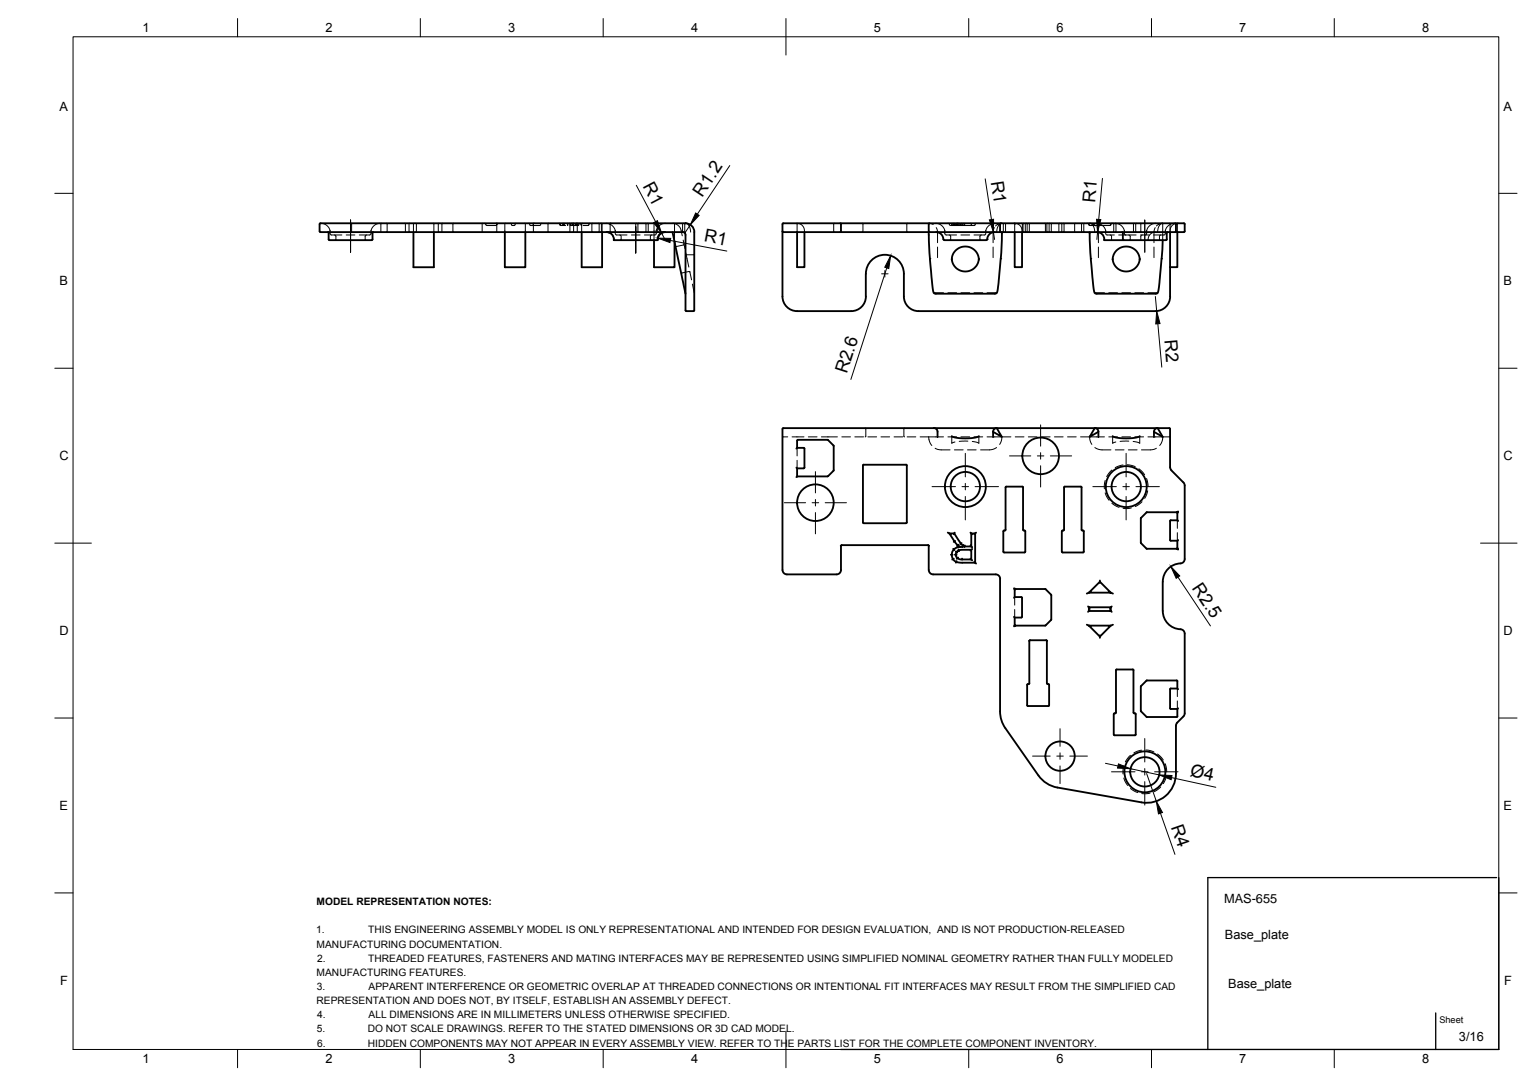
ISO-10303-21;
HEADER;
FILE_DESCRIPTION((''),'2;1');
FILE_NAME('Base_Plate.step','2026-10-09T11:34:15-07:00',(''),(''),'','','');
FILE_SCHEMA (('AUTOMOTIVE_DESIGN { 1 0 10303 214 3 1 1 }'));
ENDSEC;
DATA;
#10=MECHANICAL_DESIGN_GEOMETRIC_PRESENTATION_REPRESENTATION('',(#630),#117170);
#171=ELLIPSE('',#50166,0.169705627484765,0.12) ;
#172=ELLIPSE('',#50168,0.169705627484778,0.12) ;
#173=ELLIPSE('',#50175,0.249814202663062,0.12) ;
#174=ELLIPSE('',#50177,0.136899613896297,0.12) ;
#175=ELLIPSE('',#50182,0.169705627484765,0.12) ;
#176=ELLIPSE('',#50184,0.169705627484778,0.12) ;
#177=ELLIPSE('',#50186,0.169705627484765,0.12) ;
#178=ELLIPSE('',#50188,0.169705627484778,0.12) ;
#179=ELLIPSE('',#50195,0.169705627484765,0.12) ;
#180=ELLIPSE('',#50197,0.169705627484765,0.12) ;
#181=ELLIPSE('',#50201,0.169705627484779,0.12) ;
#182=ELLIPSE('',#50202,0.31357511157033,0.12) ;
#183=ELLIPSE('',#50204,0.313575111570327,0.12) ;
#184=ELLIPSE('',#50210,0.169705627484784,0.12) ;
#185=ELLIPSE('',#50211,0.169705627484784,0.12) ;
#186=ELLIPSE('',#50213,0.169705627484765,0.12) ;
#187=ELLIPSE('',#50215,0.169705627484753,0.12) ;
#188=ELLIPSE('',#50221,0.313575111570327,0.12) ;
#189=ELLIPSE('',#50222,0.169705627484779,0.12) ;
#190=ELLIPSE('',#50224,0.31357511157033,0.12) ;
#191=ELLIPSE('',#50230,0.249814202663065,0.12) ;
#192=ELLIPSE('',#50233,0.136899613896321,0.12) ;
#193=ELLIPSE('',#50235,0.169705627484778,0.12) ;
#194=ELLIPSE('',#50236,0.169705627484778,0.12) ;
#195=ELLIPSE('',#50238,0.169705627484765,0.12) ;
#196=ELLIPSE('',#50240,0.169705627484778,0.12) ;
#197=ELLIPSE('',#50250,1.73726470137952,1.7) ;
#198=ELLIPSE('',#50251,1.73726470137952,1.7) ;
#199=ELLIPSE('',#50254,1.73726470137952,1.7) ;
#200=ELLIPSE('',#50255,1.73726470137952,1.7) ;
#201=ELLIPSE('',#50326,0.313575111570335,0.12) ;
#202=ELLIPSE('',#50327,0.169705627484762,0.12) ;
#203=ELLIPSE('',#50329,0.313575111570314,0.12) ;
#204=ELLIPSE('',#50333,0.169705627484778,0.12) ;
#205=ELLIPSE('',#50334,0.169705627484778,0.12) ;
#206=ELLIPSE('',#50336,0.169705627484765,0.12) ;
#207=ELLIPSE('',#50338,0.169705627484778,0.12) ;
#208=ELLIPSE('',#50342,0.169705627484779,0.12) ;
#209=ELLIPSE('',#50343,0.313575111570343,0.12) ;
#210=ELLIPSE('',#50345,0.313575111570327,0.12) ;
#211=ELLIPSE('',#50371,1.73726470137952,1.7) ;
#212=ELLIPSE('',#50372,1.73726470137952,1.7) ;
#213=ELLIPSE('',#50373,1.73726470137952,1.7) ;
#214=ELLIPSE('',#50374,1.73726470137952,1.7) ;
#215=ELLIPSE('',#50520,4.854121959737,1.) ;
#216=ELLIPSE('',#50521,4.854121959737,1.) ;
#217=ELLIPSE('',#50535,4.854121959737,1.) ;
#218=ELLIPSE('',#50536,4.854121959737,1.) ;
#219=ELLIPSE('',#50561,8.2520073315529,1.7) ;
#220=ELLIPSE('',#50562,8.2520073315529,1.7) ;
#221=ELLIPSE('',#50563,8.2520073315529,1.7) ;
#222=ELLIPSE('',#50564,8.2520073315529,1.7) ;
#223=ELLIPSE('',#50565,0.707106781186556,0.5) ;
#224=ELLIPSE('',#50571,0.509901951359303,0.0999999999999979) ;
#225=ELLIPSE('',#50645,0.223606797749974,0.0999999999999979) ;
#226=ELLIPSE('',#50646,0.223606797749982,0.0999999999999979) ;
#227=ELLIPSE('',#50648,0.141421356237297,0.1) ;
#228=ELLIPSE('',#50651,0.223606797749982,0.100000000000002) ;
#229=ELLIPSE('',#50652,0.223606797749974,0.0999999999999979) ;
#230=ELLIPSE('',#50660,0.1414213562373,0.1) ;
#231=ELLIPSE('',#50779,0.223606797749974,0.0999999999999934) ;
#232=ELLIPSE('',#50780,0.223606797749982,0.0999999999999979) ;
#233=ELLIPSE('',#50783,0.223606797749982,0.0999999999999979) ;
#234=ELLIPSE('',#50784,0.223606797749974,0.100000000000002) ;
#235=ELLIPSE('',#51163,1.38924439894499,1.2) ;
#236=ELLIPSE('',#51164,1.38924439894499,1.2) ;
#237=ELLIPSE('',#51210,0.141421356237297,0.1) ;
#238=ELLIPSE('',#51222,0.141421356237292,0.1) ;
#239=ELLIPSE('',#51349,0.141421356237297,0.1) ;
#240=ELLIPSE('',#51361,0.141421356237292,0.1) ;
#241=ELLIPSE('',#51463,0.141421356237297,0.1) ;
#242=ELLIPSE('',#51475,0.141421356237292,0.1) ;
#243=ELLIPSE('',#51481,0.141421356237297,0.1) ;
#244=ELLIPSE('',#51631,1.38924439894499,1.2) ;
#245=ELLIPSE('',#51632,1.38924439894498,1.2) ;
#246=ELLIPSE('',#51634,1.38924439894498,1.2) ;
#247=ELLIPSE('',#51635,1.38924439894498,1.2) ;
#248=ELLIPSE('',#51636,1.38924439894499,1.2) ;
#249=ELLIPSE('',#51637,1.38924439894499,1.2) ;
#250=ELLIPSE('',#51639,1.38924439894499,1.2) ;
#251=ELLIPSE('',#51640,1.38924439894499,1.2) ;
#252=ELLIPSE('',#51641,1.38924439894498,1.2) ;
#253=ELLIPSE('',#51642,1.38924439894498,1.2) ;
#254=ELLIPSE('',#51644,1.38924439894498,1.20000000000001) ;
#255=ELLIPSE('',#51645,1.38924439894498,1.20000000000001) ;
#256=ELLIPSE('',#51650,0.614889130379839,0.499999999999998) ;
#257=ELLIPSE('',#51654,0.614889130379839,0.499999999999998) ;
#258=ELLIPSE('',#51660,0.614889130379839,0.499999999999998) ;
#259=ELLIPSE('',#51664,0.614889130379841,0.499999999999998) ;
#260=ELLIPSE('',#51673,4.7762432936358,0.499999999999998) ;
#261=ELLIPSE('',#51675,4.7762432936358,0.499999999999998) ;
#262=ELLIPSE('',#51683,4.7762432936358,0.499999999999998) ;
#263=ELLIPSE('',#51706,4.7762432936358,0.499999999999998) ;
#588=SHAPE_REPRESENTATION_RELATIONSHIP('SRR','None',#117243,#609) ;
#609=ADVANCED_BREP_SHAPE_REPRESENTATION('',(#651),#117151) ;
#630=STYLED_ITEM('',(#117355),#651) ;
#651=MANIFOLD_SOLID_BREP('Body1',#49059) ;
#679=FACE_BOUND('',#14322,.T.) ;
#680=FACE_BOUND('',#14408,.T.) ;
#681=FACE_BOUND('',#14409,.T.) ;
#682=FACE_BOUND('',#14410,.T.) ;
#683=FACE_BOUND('',#14411,.T.) ;
#684=FACE_BOUND('',#14412,.T.) ;
#685=FACE_BOUND('',#14413,.T.) ;
#686=FACE_BOUND('',#14414,.T.) ;
#687=FACE_BOUND('',#14415,.T.) ;
#688=FACE_BOUND('',#14416,.T.) ;
#689=FACE_BOUND('',#14417,.T.) ;
#690=FACE_BOUND('',#14418,.T.) ;
#691=FACE_BOUND('',#14419,.T.) ;
#692=FACE_BOUND('',#14420,.T.) ;
#693=FACE_BOUND('',#14421,.T.) ;
#694=FACE_BOUND('',#14422,.T.) ;
#695=FACE_BOUND('',#14423,.T.) ;
#696=FACE_BOUND('',#14424,.T.) ;
#697=FACE_BOUND('',#14425,.T.) ;
#698=FACE_BOUND('',#14447,.T.) ;
#699=FACE_BOUND('',#14453,.T.) ;
#700=FACE_BOUND('',#14454,.T.) ;
#701=FACE_BOUND('',#14455,.T.) ;
#702=FACE_BOUND('',#14456,.T.) ;
#703=FACE_BOUND('',#14457,.T.) ;
#704=FACE_BOUND('',#14458,.T.) ;
#705=FACE_BOUND('',#14459,.T.) ;
#706=FACE_BOUND('',#14460,.T.) ;
#707=FACE_BOUND('',#14461,.T.) ;
#708=FACE_BOUND('',#14462,.T.) ;
#709=FACE_BOUND('',#14463,.T.) ;
#710=FACE_BOUND('',#14464,.T.) ;
#711=FACE_BOUND('',#14465,.T.) ;
#712=FACE_BOUND('',#14466,.T.) ;
#713=FACE_BOUND('',#14496,.T.) ;
#714=FACE_BOUND('',#14502,.T.) ;
#715=FACE_BOUND('',#14505,.T.) ;
#716=FACE_BOUND('',#14509,.T.) ;
#717=FACE_BOUND('',#14512,.T.) ;
#718=FACE_BOUND('',#15017,.T.) ;
#719=FACE_BOUND('',#15025,.T.) ;
#720=FACE_BOUND('',#15032,.T.) ;
#721=FACE_BOUND('',#15038,.T.) ;
#998=B_SPLINE_CURVE_WITH_KNOTS('',3,(#79250,#79251,#79252,#79253,#79254,
#79255,#79256,#79257,#79258,#79259),.UNSPECIFIED.,.F.,.F.,(4,2,2,2,4),(-0.000984424941950333,
0.,0.0304393222729151,0.0604225486602068,0.0620633422654789),
 .UNSPECIFIED.) ;
#999=B_SPLINE_CURVE_WITH_KNOTS('',3,(#79261,#79262,#79263,#79264,#79265,
#79266,#79267,#79268,#79269,#79270,#79271,#79272,#79273,#79274),
 .UNSPECIFIED.,.F.,.F.,(4,2,2,2,2,2,4),(-8.82336995782881E-5,0.,0.00475115835790631,
0.00873436624242474,0.0121992039700031,0.0140206649989405,0.0158413354962278),
 .UNSPECIFIED.) ;
#1000=B_SPLINE_CURVE_WITH_KNOTS('',3,(#79276,#79277,#79278,#79279,#79280,
#79281,#79282,#79283,#79284,#79285,#79286,#79287,#79288,#79289,#79290,#79291,
#79292,#79293,#79294,#79295,#79296,#79297,#79298,#79299,#79300,#79301,#79302,
#79303,#79304,#79305,#79306,#79307,#79308,#79309),.UNSPECIFIED.,.F.,.F.,
(4,3,3,3,3,3,3,3,3,3,3,4),(-0.0604222015446389,-0.0550499926507643,-0.0493561418638026,
-0.0430468116754606,-0.0361516451437183,-0.0304393667102573,-0.0296323735440378,
-0.0222243385537494,-0.0158108328697019,-0.00982069491557987,-0.00433261667194647,
-2.33582884381498E-7),.UNSPECIFIED.) ;
#1001=B_SPLINE_CURVE_WITH_KNOTS('',3,(#79310,#79311,#79312,#79313,#79314,
#79315,#79316,#79317,#79318,#79319,#79320,#79321,#79322,#79323),
 .UNSPECIFIED.,.F.,.F.,(4,2,2,2,2,2,4),(-0.0211454388250223,-0.0210285224813978,
-0.0147156589259276,-0.00942919902689826,-0.00482563543048829,-0.00241277839740307,
0.),.UNSPECIFIED.) ;
#1002=B_SPLINE_CURVE_WITH_KNOTS('',3,(#79366,#79367,#79368,#79369,#79370,
#79371),.UNSPECIFIED.,.F.,.F.,(4,2,4),(-0.0604383125048107,-0.0340909276764841,
-5.87690718515846E-9),.UNSPECIFIED.) ;
#1003=B_SPLINE_CURVE_WITH_KNOTS('',3,(#79373,#79374,#79375,#79376,#79377,
#79378,#79379,#79380,#79381,#79382,#79383,#79384,#79385,#79386,#79387,#79388,
#79389,#79390,#79391,#79392,#79393,#79394,#79395,#79396,#79397),
 .UNSPECIFIED.,.F.,.F.,(4,3,3,3,3,3,3,3,4),(0.,0.142857141665404,0.284233095225632,
0.427830830943624,0.571428566661616,0.709082623356265,0.846526517857094,
0.983993345114335,1.00000000203212),.UNSPECIFIED.) ;
#1004=B_SPLINE_CURVE_WITH_KNOTS('',3,(#79399,#79400,#79401,#79402,#79403,
#79404,#79405,#79406),.UNSPECIFIED.,.F.,.F.,(4,2,2,4),(-6.37514627733282E-5,
0.0340909276764841,0.0604383336928468,0.061399226101535),.UNSPECIFIED.) ;
#1005=B_SPLINE_CURVE_WITH_KNOTS('',3,(#79407,#79408,#79409,#79410,#79411,
#79412,#79413,#79414,#79415,#79416,#79417,#79418,#79419,#79420),
 .UNSPECIFIED.,.F.,.F.,(4,2,2,2,2,2,4),(-0.0211453713160809,-0.0210284730514246,
-0.0147152918429848,-0.00942861499076061,-0.00482456947936517,-0.00241227801516162,
0.),.UNSPECIFIED.) ;
#1006=B_SPLINE_CURVE_WITH_KNOTS('',3,(#79472,#79473,#79474,#79475,#79476,
#79477,#79478,#79479,#79480,#79481),.UNSPECIFIED.,.F.,.F.,(4,2,2,2,4),(-0.0016406621045341,
0.,0.032656775096122,0.0751675585986371,0.0752925833074644),
 .UNSPECIFIED.) ;
#1007=B_SPLINE_CURVE_WITH_KNOTS('',3,(#79483,#79484,#79485,#79486,#79487,
#79488,#79489,#79490,#79491,#79492,#79493,#79494,#79495,#79496,#79497,#79498,
#79499,#79500,#79501,#79502,#79503,#79504,#79505,#79506),.UNSPECIFIED.,
 .F.,.F.,(4,2,2,2,2,2,2,2,2,2,2,4),(-0.0405465275427285,-0.0399836298810584,
-0.0342707961683927,-0.0296950430028694,-0.0224465576618196,-0.012906803650382,
-0.0107060635347755,-0.00880130672328058,-0.00614814155262501,-0.00435008553811397,
-0.00226833765470988,0.),.UNSPECIFIED.) ;
#1008=B_SPLINE_CURVE_WITH_KNOTS('',3,(#79507,#79508,#79509,#79510,#79511,
#79512,#79513,#79514,#79515,#79516,#79517,#79518,#79519,#79520,#79521,#79522,
#79523,#79524,#79525,#79526,#79527,#79528,#79529,#79530,#79531,#79532,#79533,
#79534,#79535,#79536,#79537,#79538,#79539,#79540),.UNSPECIFIED.,.F.,.F.,
(4,3,3,3,3,3,3,3,3,3,3,4),(-0.0751671270593557,-0.0670063003644427,-0.058330620968889,
-0.0493174041305417,-0.0396504587769834,-0.032656775096122,-0.0326552412924559,
-0.0240593424052777,-0.0160879007308648,-0.00858318314202981,-0.00158464448525019,
-1.06159176561375E-7),.UNSPECIFIED.) ;
#1009=B_SPLINE_CURVE_WITH_KNOTS('',3,(#79607,#79608,#79609,#79610,#79611,
#79612),.UNSPECIFIED.,.F.,.F.,(4,2,4),(-0.0457309983059805,-0.0235600635035843,
-3.22828420435411E-7),.UNSPECIFIED.) ;
#1010=B_SPLINE_CURVE_WITH_KNOTS('',3,(#79614,#79615,#79616,#79617,#79618,
#79619,#79620,#79621,#79622,#79623),.UNSPECIFIED.,.F.,.F.,(4,2,2,2,4),(-0.00096080851771424,
0.,0.0235600635035843,0.0457311162964727,0.0467303873666823),
 .UNSPECIFIED.) ;
#1011=B_SPLINE_CURVE_WITH_KNOTS('',3,(#79624,#79625,#79626,#79627,#79628,
#79629,#79630,#79631,#79632,#79633,#79634,#79635,#79636,#79637),
 .UNSPECIFIED.,.F.,.F.,(4,2,2,2,2,2,4),(-8.774851074935E-5,0.,0.00473869223690591,
0.00870703996733189,0.0121629886280889,0.0139740750814815,0.0157851260614204),
 .UNSPECIFIED.) ;
#1012=B_SPLINE_CURVE_WITH_KNOTS('',3,(#79688,#79689,#79690,#79691,#79692,
#79693,#79694,#79695,#79696,#79697,#79698,#79699,#79700,#79701,#79702,#79703,
#79704,#79705,#79706,#79707,#79708,#79709,#79710,#79711,#79712,#79713,#79714,
#79715),.UNSPECIFIED.,.F.,.F.,(4,3,3,3,3,3,3,3,3,4),(-0.0432143735368821,
-0.0386255934136773,-0.0334465535042506,-0.027720164402335,-0.0217199035575619,
-0.0210041587704275,-0.0147723605623817,-0.00929676450395368,-0.00452143288898869,
-8.08181800291421E-8),.UNSPECIFIED.) ;
#1013=B_SPLINE_CURVE_WITH_KNOTS('',3,(#79716,#79717,#79718,#79719,#79720,
#79721,#79722,#79723,#79724,#79725),.UNSPECIFIED.,.F.,.F.,(4,2,2,2,4),(-0.000999294135844071,
0.,0.0217198699392343,0.0432144526123464,0.0441989132427654),
 .UNSPECIFIED.) ;
#1014=B_SPLINE_CURVE_WITH_KNOTS('',3,(#79752,#79753,#79754,#79755,#79756,
#79757),.UNSPECIFIED.,.F.,.F.,(4,2,4),(1.8183290160026E-14,0.0307388136698783,
0.0544948017664183),.UNSPECIFIED.) ;
#1015=B_SPLINE_CURVE_WITH_KNOTS('',3,(#79763,#79764,#79765,#79766,#79767,
#79768,#79769,#79770),.UNSPECIFIED.,.F.,.F.,(4,2,2,4),(-0.000903812556791651,
0.,0.0126332411015006,0.0312371936251197),.UNSPECIFIED.) ;
#1016=B_SPLINE_CURVE_WITH_KNOTS('',3,(#79772,#79773,#79774,#79775,#79776,
#79777,#79778,#79779,#79780,#79781),.UNSPECIFIED.,.F.,.F.,(4,2,2,2,4),(-0.000668949496694549,
0.,0.0150950300818429,0.0294213468333971,0.0303251295908459),
 .UNSPECIFIED.) ;
#1017=B_SPLINE_CURVE_WITH_KNOTS('',3,(#79783,#79784,#79785,#79786,#79787,
#79788,#79789,#79790,#79791,#79792),.UNSPECIFIED.,.F.,.F.,(4,2,2,2,4),(-0.00020740379149845,
0.,0.0232646742763639,0.0410522705936588,0.041721226167804),
 .UNSPECIFIED.) ;
#1018=B_SPLINE_CURVE_WITH_KNOTS('',3,(#79794,#79795,#79796,#79797,#79798,
#79799,#79800,#79801),.UNSPECIFIED.,.F.,.F.,(4,2,2,4),(-4.75212523545475E-5,
0.0386336727204952,0.0678747004384468,0.0680821984481714),.UNSPECIFIED.) ;
#1019=B_SPLINE_CURVE_WITH_KNOTS('',3,(#79809,#79810,#79811,#79812,#79813,
#79814),.UNSPECIFIED.,.F.,.F.,(4,2,4),(0.000722157276979357,0.0318468005485353,
0.0667305959449343),.UNSPECIFIED.) ;
#1020=B_SPLINE_CURVE_WITH_KNOTS('',3,(#79816,#79817,#79818,#79819,#79820,
#79821,#79822,#79823),.UNSPECIFIED.,.F.,.F.,(4,2,2,4),(-0.0369647188766498,
0.,0.0196661092474417,0.0345442295414817),.UNSPECIFIED.) ;
#1021=B_SPLINE_CURVE_WITH_KNOTS('',3,(#79825,#79826,#79827,#79828,#79829,
#79830,#79831,#79832),.UNSPECIFIED.,.F.,.F.,(4,2,2,4),(0.00145417557171005,
0.0398009040484053,0.0884506599106943,0.125182168962163),.UNSPECIFIED.) ;
#1022=B_SPLINE_CURVE_WITH_KNOTS('',3,(#79834,#79835,#79836,#79837,#79838,
#79839,#79840,#79841),.UNSPECIFIED.,.F.,.F.,(4,1,2,1,4),(0.000848899917498889,
0.021868453247988,0.0364474220799808,0.0505556257289287,0.070263889237609),
 .UNSPECIFIED.) ;
#1023=B_SPLINE_CURVE_WITH_KNOTS('',3,(#79843,#79844,#79845,#79846,#79847,
#79848),.UNSPECIFIED.,.F.,.F.,(4,2,4),(0.000832214192100071,0.0289083223985083,
0.0574703491509667),.UNSPECIFIED.) ;
#1024=B_SPLINE_CURVE_WITH_KNOTS('',3,(#79850,#79851,#79852,#79853,#79854,
#79855,#79856,#79857),.UNSPECIFIED.,.F.,.F.,(4,1,2,1,4),(0.00109423153353252,
0.0104867604235457,0.0262169010588733,0.0371127510104888,0.052624276685899),
 .UNSPECIFIED.) ;
#1025=B_SPLINE_CURVE_WITH_KNOTS('',3,(#79859,#79860,#79861,#79862,#79863,
#79864),.UNSPECIFIED.,.F.,.F.,(4,2,4),(4.70742900094273E-5,0.0453812948763195,
0.0781603595086036),.UNSPECIFIED.) ;
#1026=B_SPLINE_CURVE_WITH_KNOTS('',3,(#79877,#79878,#79879,#79880,#79881,
#79882,#79883,#79884,#79885,#79886,#79887,#79888,#79889,#79890,#79891,#79892,
#79893,#79894,#79895,#79896,#79897,#79898),.UNSPECIFIED.,.F.,.F.,(4,2,2,
2,2,2,2,2,2,2,4),(-0.0189100268387207,-0.0188225261357837,-0.0160937127726661,
-0.0140628523915856,-0.0113357098457601,-0.010804126006901,-0.00937481072638454,
-0.00663134068272864,-0.00468727656071559,-0.00196623445923168,0.),
 .UNSPECIFIED.) ;
#1027=B_SPLINE_CURVE_WITH_KNOTS('',3,(#79905,#79906,#79907,#79908,#79909,
#79910,#79911,#79912,#79913,#79914,#79915,#79916,#79917,#79918,#79919,#79920,
#79921,#79922,#79923,#79924,#79925,#79926),.UNSPECIFIED.,.F.,.F.,(4,2,2,
2,2,2,2,2,2,2,4),(-0.0189091510353225,-0.0188216583950064,-0.0160930867214601,
-0.0140631747980082,-0.0113361362872527,-0.010803887239561,-0.00937541792678878,
-0.00663206984589378,-0.00468769926487486,-0.00196659271288638,0.),
 .UNSPECIFIED.) ;
#1028=B_SPLINE_CURVE_WITH_KNOTS('',3,(#79969,#79970,#79971,#79972,#79973,
#79974,#79975,#79976,#79977,#79978,#79979,#79980,#79981,#79982,#79983,#79984,
#79985,#79986,#79987,#79988,#79989,#79990,#79991,#79992,#79993,#79994,#79995,
#79996,#79997,#79998,#79999,#80000,#80001,#80002),.UNSPECIFIED.,.F.,.F.,
(4,3,3,3,3,3,3,3,3,3,3,4),(-0.0189104384936197,-0.0188229339990635,-0.0160940759188526,
-0.0140627008849462,-0.011335536637837,-0.0108042382537074,-0.00937452533081662,
-0.00663104829102613,-0.00468707787444879,-0.00196605255282242,-9.10972545172394E-5,
0.),.UNSPECIFIED.) ;
#1029=B_SPLINE_CURVE_WITH_KNOTS('',3,(#80003,#80004,#80005,#80006,#80007,
#80008),.UNSPECIFIED.,.F.,.F.,(4,2,4),(-0.0678747004384468,-0.0386336727204952,
9.931359662603E-16),.UNSPECIFIED.) ;
#1030=B_SPLINE_CURVE_WITH_KNOTS('',3,(#80060,#80061,#80062,#80063,#80064,
#80065,#80066,#80067,#80068,#80069,#80070,#80071,#80072,#80073,#80074,#80075,
#80076,#80077,#80078,#80079,#80080,#80081,#80082,#80083,#80084,#80085,#80086,
#80087,#80088,#80089,#80090,#80091,#80092,#80093),.UNSPECIFIED.,.F.,.F.,
(4,3,3,3,3,3,3,3,3,3,3,4),(-0.0189231987523393,-0.0188355768250839,-0.016103896315164,
-0.0140579962341654,-0.0113294935982673,-0.0108077177394999,-0.00936568511698275,
-0.00662104306256861,-0.00468092840563795,-0.00196078713666773,-0.000132076778823899,
0.),.UNSPECIFIED.) ;
#1031=B_SPLINE_CURVE_WITH_KNOTS('',3,(#80094,#80095,#80096,#80097,#80098,
#80099,#80100,#80101,#80102,#80103,#80104,#80105,#80106,#80107,#80108,#80109,
#80110,#80111,#80112,#80113,#80114,#80115,#80116,#80117,#80118),
 .UNSPECIFIED.,.F.,.F.,(4,3,3,3,3,3,3,3,4),(-0.041052254598462,-0.0353947710294345,
-0.0290069620103994,-0.0232649417665907,-0.0232646742763639,-0.0157599768214883,
-0.00879512539945639,-0.00239829329457513,-6.62284045196766E-9),
 .UNSPECIFIED.) ;
#1032=B_SPLINE_CURVE_WITH_KNOTS('',3,(#80151,#80152,#80153,#80154,#80155,
#80156),.UNSPECIFIED.,.F.,.F.,(4,2,4),(-0.0792555822118552,-0.0453812948763195,
2.08166817117217E-17),.UNSPECIFIED.) ;
#1033=B_SPLINE_CURVE_WITH_KNOTS('',3,(#80158,#80159,#80160,#80161,#80162,
#80163,#80164,#80165,#80166,#80167,#80168,#80169,#80170,#80171),
 .UNSPECIFIED.,.F.,.F.,(4,2,2,2,2,2,4),(-8.7816797165505E-5,0.,0.00473925006253047,
0.00870923522712718,0.0121658095680286,0.0139774248519991,0.0157888885985204),
 .UNSPECIFIED.) ;
#1034=B_SPLINE_CURVE_WITH_KNOTS('',3,(#80223,#80224,#80225,#80226,#80227,
#80228,#80229,#80230,#80231,#80232,#80233,#80234,#80235,#80236,#80237,#80238,
#80239,#80240,#80241,#80242,#80243,#80244,#80245,#80246,#80247,#80248,#80249,
#80250,#80251,#80252,#80253,#80254,#80255,#80256),.UNSPECIFIED.,.F.,.F.,
(4,3,3,3,3,3,3,3,3,3,3,4),(-8.77394398539964E-5,0.,0.00273498567989683,
0.00479398440821394,0.00752394270229122,0.00803717040806658,0.00949060351895224,
0.0122365053916693,0.0141734575442573,0.0168931630703535,0.0187358978034301,
0.0188493460956781),.UNSPECIFIED.) ;
#1035=B_SPLINE_CURVE_WITH_KNOTS('',3,(#80257,#80258,#80259,#80260,#80261,
#80262),.UNSPECIFIED.,.F.,.F.,(4,2,4),(-0.029421301615743,-0.0150950300818429,
-3.73770280713704E-8),.UNSPECIFIED.) ;
#1036=B_SPLINE_CURVE_WITH_KNOTS('',3,(#80309,#80310,#80311,#80312,#80313,
#80314,#80315,#80316,#80317,#80318,#80319,#80320,#80321,#80322,#80323,#80324,
#80325,#80326,#80327,#80328,#80329,#80330),.UNSPECIFIED.,.F.,.F.,(4,3,3,
3,3,3,3,4),(-0.0312400832992503,-0.0246244522927767,-0.0173572943526231,
-0.0126332423749213,-0.011908506553527,-0.00595425844831785,-0.000527709717726606,
-1.03431087073348E-8),.UNSPECIFIED.) ;
#1037=B_SPLINE_CURVE_WITH_KNOTS('',3,(#80386,#80387,#80388,#80389,#80390,
#80391,#80392,#80393),.UNSPECIFIED.,.F.,.F.,(4,1,2,1,4),(-0.0534565259379121,
-0.0371127510104888,-0.0262169010588733,-0.0104867604235457,6.07153216596483E-15),
 .UNSPECIFIED.) ;
#1038=B_SPLINE_CURVE_WITH_KNOTS('',3,(#80394,#80395,#80396,#80397,#80398,
#80399,#80400,#80401,#80402,#80403,#80404,#80405,#80406,#80407,#80408,#80409,
#80410,#80411,#80412,#80413,#80414,#80415,#80416,#80417,#80418,#80419,#80420,
#80421,#80422,#80423,#80424,#80425,#80426,#80427),.UNSPECIFIED.,.F.,.F.,
(4,3,3,3,3,3,3,3,3,3,3,4),(-0.0189309682305329,-0.0188432744075911,-0.0161088065138652,
-0.0140551360522483,-0.0113261441011701,-0.0108100283879569,-0.0108098271232967,
-0.00936033610026891,-0.00661505228534929,-0.00467721248496698,-0.00195726652153048,
0.),.UNSPECIFIED.) ;
#1039=B_SPLINE_CURVE_WITH_KNOTS('',3,(#80459,#80460,#80461,#80462,#80463,
#80464,#80465,#80466,#80467,#80468,#80469,#80470,#80471,#80472,#80473,#80474,
#80475,#80476,#80477,#80478,#80479,#80480,#80481,#80482,#80483,#80484,#80485,
#80486,#80487,#80488,#80489,#80490,#80491,#80492,#80493,#80494,#80495,#80496,
#80497,#80498),.UNSPECIFIED.,.F.,.F.,(4,3,3,3,3,3,3,3,3,3,3,3,3,4),(-0.0583191426684248,
-0.0515202234042521,-0.0455591618953523,-0.0399214617427771,-0.034414844098878,
-0.0316615352769285,-0.0302848808659537,-0.0294521489819769,-0.028908226454979,
-0.0238511390677379,-0.0185352795979771,-0.0127504766938683,-0.00631797168678906,
1.19054072156493E-14),.UNSPECIFIED.) ;
#1040=B_SPLINE_CURVE_WITH_KNOTS('',3,(#80499,#80500,#80501,#80502,#80503,
#80504,#80505,#80506,#80507,#80508,#80509,#80510,#80511,#80512,#80513,#80514,
#80515,#80516,#80517,#80518,#80519,#80520,#80521,#80522,#80523,#80524,#80525,
#80526,#80527,#80528,#80529,#80530,#80531,#80532),.UNSPECIFIED.,.F.,.F.,
(4,3,3,3,3,3,3,3,3,3,3,4),(-8.77110797273226E-5,0.,0.00273520643559201,
0.00478983254758793,0.00751988059915136,0.0080349187065388,0.00803514813958154,
0.00948541104957732,0.0122325784356822,0.0141688418023582,0.0168884919204612,
0.0188461231184326),.UNSPECIFIED.) ;
#1041=B_SPLINE_CURVE_WITH_KNOTS('',3,(#80574,#80575,#80576,#80577,#80578,
#80579,#80580,#80581),.UNSPECIFIED.,.F.,.F.,(4,1,2,1,4),(-0.0717179312023507,
-0.0505556257289287,-0.0364474220799808,-0.021868453247988,1.21551489931584E-15),
 .UNSPECIFIED.) ;
#1042=B_SPLINE_CURVE_WITH_KNOTS('',3,(#80582,#80583,#80584,#80585,#80586,
#80587,#80588,#80589,#80590,#80591,#80592,#80593,#80594,#80595,#80596,#80597,
#80598,#80599,#80600,#80601,#80602,#80603,#80604,#80605,#80606,#80607,#80608,
#80609,#80610,#80611,#80612,#80613,#80614,#80615,#80616,#80617,#80618),
 .UNSPECIFIED.,.F.,.F.,(4,3,3,3,3,3,3,3,3,3,3,3,4),(-0.0189757898193099,
-0.0188876825104194,-0.016141250710988,-0.0140385129384437,-0.0113059119834885,
-0.0108221873966673,-0.0108220365581979,-0.00932947344905913,-0.00658072601880498,
-0.00465582700007615,-0.00270420596151227,-0.00193828076950875,0.),
 .UNSPECIFIED.) ;
#1043=B_SPLINE_CURVE_WITH_KNOTS('',3,(#80668,#80669,#80670,#80671,#80672,
#80673),.UNSPECIFIED.,.F.,.F.,(4,2,4),(-0.0884477485126169,-0.0398009040484053,
3.34298561055327E-14),.UNSPECIFIED.) ;
#1044=B_SPLINE_CURVE_WITH_KNOTS('',3,(#80674,#80675,#80676,#80677,#80678,
#80679,#80680,#80681,#80682,#80683,#80684,#80685,#80686,#80687),
 .UNSPECIFIED.,.F.,.F.,(4,2,2,2,2,2,4),(-0.000257748868228079,0.,0.0227861491765853,
0.0430952613497541,0.0513731219354545,0.0545021507438859,0.0573049792139941),
 .UNSPECIFIED.) ;
#1045=B_SPLINE_CURVE_WITH_KNOTS('',3,(#80729,#80730,#80731,#80732,#80733,
#80734),.UNSPECIFIED.,.F.,.F.,(4,2,4),(-0.0352658770408685,-0.0196661092474417,
3.06681289893858E-7),.UNSPECIFIED.) ;
#1046=B_SPLINE_CURVE_WITH_KNOTS('',3,(#80735,#80736,#80737,#80738,#80739,
#80740,#80741,#80742,#80743,#80744,#80745,#80746,#80747,#80748,#80749,#80750,
#80751,#80752,#80753,#80754,#80755,#80756,#80757,#80758,#80759,#80760,#80761,
#80762,#80763,#80764,#80765),.UNSPECIFIED.,.F.,.F.,(4,3,3,3,3,3,3,3,3,3,
4),(-0.0189255450014105,-0.0188379011808369,-0.0161048586406479,-0.0140571373249443,
-0.0113284598467218,-0.010808352019202,-0.00936407769447349,-0.00661884257235523,
-0.00467981132905438,-0.00195973370921565,0.),.UNSPECIFIED.) ;
#1047=B_SPLINE_CURVE_WITH_KNOTS('',3,(#80796,#80797,#80798,#80799,#80800,
#80801,#80802,#80803,#80804,#80805,#80806,#80807,#80808,#80809,#80810,#80811,
#80812,#80813,#80814,#80815,#80816,#80817,#80818,#80819,#80820,#80821,#80822,
#80823,#80824,#80825,#80826,#80827,#80828,#80829),.UNSPECIFIED.,.F.,.F.,
(4,3,3,3,3,3,3,3,3,3,3,4),(-0.0669038356909525,-0.0556776653306576,-0.0448761350683132,
-0.0383614116366248,-0.0351040499207806,-0.0332964637419825,-0.0320905242267506,
-0.0318466882049363,-0.0219526243138846,-0.0116986697167936,-0.000861115342412766,
0.),.UNSPECIFIED.) ;
#1048=B_SPLINE_CURVE_WITH_KNOTS('',3,(#80843,#80844,#80845,#80846,#80847,
#80848),.UNSPECIFIED.,.F.,.F.,(4,2,4),(5.55111512312578E-17,0.0224201537133612,
0.0402049184529),.UNSPECIFIED.) ;
#1049=B_SPLINE_CURVE_WITH_KNOTS('',3,(#80862,#80863,#80864,#80865,#80866,
#80867),.UNSPECIFIED.,.F.,.F.,(4,2,4),(9.61380643681049E-9,0.033998052296077,
0.0714229819360441),.UNSPECIFIED.) ;
#1050=B_SPLINE_CURVE_WITH_KNOTS('',3,(#80892,#80893,#80894,#80895,#80896,
#80897),.UNSPECIFIED.,.F.,.F.,(4,2,4),(5.83560977318598E-15,0.0377278926030736,
0.066283338281117),.UNSPECIFIED.) ;
#1051=B_SPLINE_CURVE_WITH_KNOTS('',3,(#80910,#80911,#80912,#80913,#80914,
#80915),.UNSPECIFIED.,.F.,.F.,(4,2,4),(-2.77555756156289E-17,0.0199847249930681,
0.0352638829354677),.UNSPECIFIED.) ;
#1052=B_SPLINE_CURVE_WITH_KNOTS('',3,(#80928,#80929,#80930,#80931,#80932,
#80933,#80934,#80935,#80936,#80937,#80938,#80939,#80940,#80941,#80942,#80943,
#80944,#80945,#80946,#80947,#80948,#80949,#80950,#80951,#80952,#80953,#80954,
#80955,#80956,#80957,#80958,#80959,#80960,#80961),.UNSPECIFIED.,.F.,.F.,
(4,3,3,3,3,3,3,3,3,3,3,4),(-4.8815118613983E-15,0.0033937817965806,0.00647026806505026,
0.00922156932779166,0.0105972199591624,0.0112850452748477,0.0117100374865891,
0.0119728705905331,0.0145178026139032,0.0173664913107944,0.0204777162912316,
0.023335857822899),.UNSPECIFIED.) ;
#1053=B_SPLINE_CURVE_WITH_KNOTS('',3,(#80974,#80975,#80976,#80977,#80978,
#80979),.UNSPECIFIED.,.F.,.F.,(4,2,4),(-3.37568514807661E-14,0.0112807751130659,
0.0278959164324805),.UNSPECIFIED.) ;
#1054=B_SPLINE_CURVE_WITH_KNOTS('',3,(#81026,#81027,#81028,#81029,#81030,
#81031,#81032,#81033),.UNSPECIFIED.,.F.,.F.,(4,1,2,1,4),(-0.0331275497757554,
-0.0275093508272253,-0.0175825659440626,-0.0105495395664116,-0.000960732822002768),
 .UNSPECIFIED.) ;
#1055=B_SPLINE_CURVE_WITH_KNOTS('',3,(#81034,#81035,#81036,#81037,#81038,
#81039,#81040,#81041,#81042,#81043,#81044,#81045,#81046,#81047),
 .UNSPECIFIED.,.F.,.F.,(4,2,2,2,2,2,4),(-8.76821873054501E-5,0.,0.00473755893099621,
0.0087048318969467,0.0121603865659108,0.0139701425181185,0.0157799606242108),
 .UNSPECIFIED.) ;
#1056=B_SPLINE_CURVE_WITH_KNOTS('',3,(#81049,#81050,#81051,#81052,#81053,
#81054,#81055,#81056),.UNSPECIFIED.,.F.,.F.,(4,1,2,1,4),(-6.50365178378404E-14,
0.0105495395664116,0.0175825659440626,0.0275093508272253,0.0341272074160004),
 .UNSPECIFIED.) ;
#1057=B_SPLINE_CURVE_WITH_KNOTS('',3,(#81057,#81058,#81059,#81060,#81061,
#81062,#81063,#81064,#81065,#81066,#81067,#81068,#81069,#81070),
 .UNSPECIFIED.,.F.,.F.,(4,2,2,2,2,2,4),(-0.0211469908685138,-0.0210301208681755,
-0.0147166592526885,-0.00942972110677525,-0.00482452106724603,-0.00241229268713677,
0.),.UNSPECIFIED.) ;
#1058=B_SPLINE_CURVE_WITH_KNOTS('',3,(#81073,#81074,#81075,#81076,#81077,
#81078,#81079,#81080,#81081,#81082,#81083,#81084,#81085,#81086,#81087,#81088),
 .UNSPECIFIED.,.F.,.F.,(4,2,2,2,2,2,2,4),(0.,0.226168647000758,0.452278992039162,
0.678340117421019,0.90457233447104,1.13067979945043,1.35690435214638,1.57080531075693),
 .UNSPECIFIED.) ;
#1059=B_SPLINE_CURVE_WITH_KNOTS('',3,(#81096,#81097,#81098,#81099,#81100,
#81101,#81102,#81103,#81104,#81105,#81106,#81107,#81108,#81109,#81110,#81111,
#81112,#81113,#81114,#81115,#81116,#81117),.UNSPECIFIED.,.F.,.F.,(4,2,2,
2,2,2,2,2,2,2,4),(-0.018909573318621,-0.0188220768043535,-0.016093251639432,
-0.0140630190939924,-0.0113315789493842,-0.0108040023625357,-0.00937512502025987,
-0.006640358962904,-0.00468749542006272,-0.00270182786113088,0.),
 .UNSPECIFIED.) ;
#1060=B_SPLINE_CURVE_WITH_KNOTS('',3,(#81162,#81163,#81164,#81165,#81166,
#81167,#81168,#81169,#81170,#81171,#81172,#81173,#81174,#81175,#81176,#81177,
#81178,#81179,#81180,#81181,#81182,#81183,#81184,#81185,#81186,#81187,#81188,
#81189,#81190,#81191,#81192,#81193,#81194,#81195,#81196,#81197,#81198,#81199,
#81200,#81201,#81202,#81203,#81204),.UNSPECIFIED.,.F.,.F.,(4,3,3,3,3,3,
3,3,3,3,3,3,3,3,4),(-8.68229099727415E-16,0.00603095577270896,0.0112970853615661,
0.0160979596706912,0.0206419392505884,0.0248678312070903,0.0270954741281374,
0.0275760705491088,0.0325996412774412,0.0378159722742326,0.0426458767484477,
0.0483565421817521,0.054471144104918,0.0614210976336497,0.062393728839361),
 .UNSPECIFIED.) ;
#1061=B_SPLINE_CURVE_WITH_KNOTS('',3,(#81206,#81207,#81208,#81209,#81210,
#81211,#81212),.UNSPECIFIED.,.F.,.F.,(4,1,2,4),(-0.0622686948925872,-0.0412193079076597,
-0.0271030272865255,-0.00164197031784536),.UNSPECIFIED.) ;
#1062=B_SPLINE_CURVE_WITH_KNOTS('',3,(#81213,#81214,#81215,#81216,#81217,
#81218,#81219,#81220,#81221,#81222,#81223,#81224,#81225,#81226),
 .UNSPECIFIED.,.F.,.F.,(4,2,2,2,2,2,4),(-0.0264075038978238,-0.0262264477757636,
-0.0165688239045476,-0.00981534868988691,-0.00481983637094454,-0.0024018084974946,
0.),.UNSPECIFIED.) ;
#1063=B_SPLINE_CURVE_WITH_KNOTS('',3,(#81284,#81285,#81286,#81287,#81288,
#81289,#81290,#81291,#81292,#81293,#81294,#81295,#81296,#81297,#81298,#81299,
#81300,#81301,#81302,#81303,#81304,#81305,#81306,#81307,#81308,#81309,#81310,
#81311,#81312,#81313,#81314,#81315,#81316,#81317,#81318,#81319,#81320,#81321,
#81322,#81323,#81324,#81325,#81326,#81327,#81328,#81329,#81330,#81331,#81332,
#81333,#81334,#81335),.UNSPECIFIED.,.F.,.F.,(4,3,3,3,3,3,3,3,3,3,3,3,3,
3,3,3,3,4),(0.,0.00450947947892499,0.00841902259411946,0.00901895895784998,
0.0124006553358025,0.015294160794407,0.0180109586247333,0.0204951745201462,
0.0225457444696602,0.0225473973946249,0.0251046180458128,0.0269891467103356,
0.0296981883061816,0.0314308960260463,0.0349082131518329,0.0386648400573158,
0.0430428695384302,0.0447561439731784),.UNSPECIFIED.) ;
#1064=B_SPLINE_CURVE_WITH_KNOTS('',3,(#81337,#81338,#81339,#81340,#81341,
#81342,#81343,#81344,#81345),.UNSPECIFIED.,.F.,.F.,(4,1,1,2,1,4),(-0.043116371938142,
-0.0314308960260463,-0.0269891467103356,-0.0225473973946249,-0.00901895895784998,
-0.00098511887011706),.UNSPECIFIED.) ;
#1065=B_SPLINE_CURVE_WITH_KNOTS('',3,(#81346,#81347,#81348,#81349,#81350,
#81351,#81352,#81353,#81354,#81355,#81356,#81357,#81358,#81359,#81360,#81361,
#81362,#81363,#81364,#81365,#81366,#81367,#81368,#81369,#81370,#81371,#81372,
#81373,#81374,#81375,#81376,#81377,#81378,#81379,#81380,#81381,#81382,#81383,
#81384,#81385),.UNSPECIFIED.,.F.,.F.,(4,3,3,3,3,3,3,3,3,3,3,3,3,4),(-8.77879354781158E-5,
0.,0.00252798145936727,0.00273454309078326,0.00480081491969721,0.00753353483528674,
0.00804095404153383,0.00804321999015075,0.00949906978678616,0.0122336738715351,
0.0134513299663313,0.0141810106313358,0.0169048836436778,0.0188547055635755),
 .UNSPECIFIED.) ;
#1066=B_SPLINE_CURVE_WITH_KNOTS('',3,(#81426,#81427,#81428,#81429,#81430,
#81431,#81432,#81433,#81434,#81435,#81436,#81437,#81438,#81439,#81440,#81441,
#81442,#81443,#81444,#81445,#81446,#81447,#81448,#81449,#81450,#81451,#81452,
#81453,#81454,#81455,#81456,#81457,#81458,#81459,#81460,#81461,#81462,#81463,
#81464,#81465,#81466,#81467,#81468,#81469,#81470,#81471),.UNSPECIFIED.,
 .F.,.F.,(4,3,3,3,3,3,3,3,3,3,3,3,3,3,3,4),(-3.8936437845742E-15,0.00412980358625654,
0.0073953121092872,0.0102645357852797,0.0129835018205587,0.0147513580827983,
0.0156352862139181,0.0161055136169195,0.0164277850761292,0.0165192143450379,
0.0190242492168354,0.0217091716190259,0.024723772049841,0.0271062306444131,
0.0309150163721508,0.0328614318196219),.UNSPECIFIED.) ;
#1067=B_SPLINE_CURVE_WITH_KNOTS('',3,(#81472,#81473,#81474,#81475,#81476,
#81477,#81478,#81479),.UNSPECIFIED.,.F.,.F.,(4,1,2,1,4),(-0.0318767983081372,
-0.0263234394910323,-0.016516450998148,-0.00990987059888721,-0.0010005474151551),
 .UNSPECIFIED.) ;
#1068=B_SPLINE_CURVE_WITH_KNOTS('',3,(#81510,#81511,#81512,#81513,#81514,
#81515),.UNSPECIFIED.,.F.,.F.,(4,2,4),(-0.0535332247771704,-0.0307388136698783,
-6.37552332398931E-5),.UNSPECIFIED.) ;
#1069=B_SPLINE_CURVE_WITH_KNOTS('',3,(#81614,#81615,#81616,#81617,#81618,
#81619,#81620,#81621,#81622,#81623,#81624,#81625,#81626,#81627,#81628,#81629,
#81630,#81631,#81632,#81633),.UNSPECIFIED.,.F.,.F.,(4,2,2,2,2,2,2,2,2,4),
(-0.0576966986557776,-0.0574332020643026,-0.0527195345357808,-0.0451607359259123,
-0.0302726022898489,-0.0168228643688311,-0.0103578801382715,-0.00596969171523668,
-0.00327048355186457,0.),.UNSPECIFIED.) ;
#1070=B_SPLINE_CURVE_WITH_KNOTS('',3,(#81686,#81687,#81688,#81689,#81690,
#81691,#81692,#81693,#81694,#81695),.UNSPECIFIED.,.F.,.F.,(4,2,2,2,4),(-0.0715962154387296,
-0.0714230469344481,-0.033998052296077,0.,0.000721914453027042),
 .UNSPECIFIED.) ;
#1071=B_SPLINE_CURVE_WITH_KNOTS('',3,(#81696,#81697,#81698,#81699,#81700,
#81701,#81702,#81703,#81704,#81705,#81706,#81707,#81708,#81709,#81710,#81711,
#81712,#81713,#81714,#81715,#81716,#81717,#81718,#81719,#81720,#81721,#81722,
#81723,#81724,#81725,#81726,#81727,#81728,#81729),.UNSPECIFIED.,.F.,.F.,
(4,3,3,3,3,3,3,3,3,3,3,4),(-8.76499876818703E-5,0.,0.00273272879714876,
0.00478109970919887,0.00750990480829954,0.00803013500119809,0.00947451694969623,
0.0122195242547994,0.0141591392154495,0.0168794617448153,0.0187493114075714,
0.0188393055184181),.UNSPECIFIED.) ;
#1072=B_SPLINE_CURVE_WITH_KNOTS('',3,(#81771,#81772,#81773,#81774,#81775,
#81776),.UNSPECIFIED.,.F.,.F.,(4,2,4),(-0.0409268414934542,-0.0402049350827121,
-0.0322019631637999),.UNSPECIFIED.) ;
#1073=B_SPLINE_CURVE_WITH_KNOTS('',3,(#81777,#81778,#81779,#81780,#81781,
#81782,#81783,#81784,#81785,#81786,#81787,#81788,#81789,#81790),
 .UNSPECIFIED.,.F.,.F.,(4,2,2,2,2,2,4),(-0.0287724923583598,-0.0286527043683762,
-0.0151123592994182,-0.00653065970956893,-0.00288793000485767,-0.00137884937746232,
0.),.UNSPECIFIED.) ;
#1074=B_SPLINE_CURVE_WITH_KNOTS('',3,(#81838,#81839,#81840,#81841,#81842,
#81843,#81844,#81845),.UNSPECIFIED.,.F.,.F.,(4,2,2,4),(-0.0689415808684068,
-0.0452350077421772,0.,0.00145402880520905),.UNSPECIFIED.) ;
#1075=B_SPLINE_CURVE_WITH_KNOTS('',3,(#81847,#81848,#81849,#81850,#81851,
#81852,#81853,#81854,#81855,#81856,#81857,#81858,#81859,#81860),
 .UNSPECIFIED.,.F.,.F.,(4,2,2,2,2,2,4),(-8.81034153357365E-5,0.,0.00474653617288703,
0.00872474084759045,0.0121859542723517,0.0140038756503188,0.0158211901338128),
 .UNSPECIFIED.) ;
#1076=B_SPLINE_CURVE_WITH_KNOTS('',3,(#81861,#81862,#81863,#81864,#81865,
#81866),.UNSPECIFIED.,.F.,.F.,(4,2,4),(1.07296738594995E-7,0.0452350077421772,
0.100520135955306),.UNSPECIFIED.) ;
#1077=B_SPLINE_CURVE_WITH_KNOTS('',3,(#81918,#81919,#81920,#81921,#81922,
#81923,#81924,#81925,#81926,#81927),.UNSPECIFIED.,.F.,.F.,(4,2,2,2,4),(-0.0870620753300636,
-0.0856081292457083,-0.0435056845362515,0.,0.000848777061136591),
 .UNSPECIFIED.) ;
#1078=B_SPLINE_CURVE_WITH_KNOTS('',3,(#81929,#81930,#81931,#81932,#81933,
#81934,#81935,#81936,#81937,#81938,#81939,#81940,#81941,#81942,#81943,#81944,
#81945,#81946,#81947,#81948,#81949,#81950,#81951,#81952,#81953,#81954,#81955,
#81956,#81957,#81958,#81959,#81960,#81961,#81962),.UNSPECIFIED.,.F.,.F.,
(4,3,3,3,3,3,3,3,3,3,3,4),(-0.0189318067161962,-0.0188441055189667,-0.0161139390575287,
-0.0140548164804191,-0.0113247732297175,-0.0108100655848069,-0.00935972898436879,
-0.00661354647959299,-0.00467678954238819,-0.00195798115489982,-0.000183016470591954,
0.),.UNSPECIFIED.) ;
#1079=B_SPLINE_CURVE_WITH_KNOTS('',3,(#81963,#81964,#81965,#81966,#81967,
#81968),.UNSPECIFIED.,.F.,.F.,(4,2,4),(7.47511594064578E-8,0.0435056845362515,
0.0856079410889234),.UNSPECIFIED.) ;
#1080=B_SPLINE_CURVE_WITH_KNOTS('',3,(#82020,#82021,#82022,#82023,#82024,
#82025,#82026,#82027,#82028,#82029),.UNSPECIFIED.,.F.,.F.,(4,2,2,2,4),(-0.0691265383481362,
-0.0682776647009788,-0.0338448162467367,0.,0.000832239105180238),
 .UNSPECIFIED.) ;
#1081=B_SPLINE_CURVE_WITH_KNOTS('',3,(#82031,#82032,#82033,#82034,#82035,
#82036,#82037,#82038,#82039,#82040,#82041,#82042,#82043,#82044,#82045,#82046,
#82047,#82048,#82049,#82050,#82051,#82052,#82053,#82054,#82055,#82056,#82057,
#82058,#82059,#82060,#82061,#82062,#82063,#82064),.UNSPECIFIED.,.F.,.F.,
(4,3,3,3,3,3,3,3,3,3,3,4),(-8.7701944723502E-5,0.,0.00273259197152701,0.00478857188803212,
0.00751836784307051,0.00803421626080498,0.00948384878366692,0.0122297141375811,
0.0141674461840516,0.0168870659675853,0.0186680252920398,0.0188451300988223),
 .UNSPECIFIED.) ;
#1082=B_SPLINE_CURVE_WITH_KNOTS('',3,(#82065,#82066,#82067,#82068,#82069,
#82070),.UNSPECIFIED.,.F.,.F.,(4,2,4),(4.92710764161277E-8,0.0338448162467367,
0.0682776016463813),.UNSPECIFIED.) ;
#1083=B_SPLINE_CURVE_WITH_KNOTS('',3,(#82122,#82123,#82124,#82125,#82126,
#82127,#82128,#82129,#82130,#82131),.UNSPECIFIED.,.F.,.F.,(4,2,2,2,4),(-0.0663005130080268,
-0.065468485698588,-0.0321085924337593,0.,0.00109408852437443),
 .UNSPECIFIED.) ;
#1084=B_SPLINE_CURVE_WITH_KNOTS('',3,(#82133,#82134,#82135,#82136,#82137,
#82138,#82139,#82140,#82141,#82142,#82143,#82144,#82145,#82146),
 .UNSPECIFIED.,.F.,.F.,(4,2,2,2,2,2,4),(-0.02115345221426,-0.0210364437818934,
-0.0147219471919079,-0.0094328410561899,-0.0048279676271279,-0.00241386739955191,
0.),.UNSPECIFIED.) ;
#1085=B_SPLINE_CURVE_WITH_KNOTS('',3,(#82147,#82148,#82149,#82150,#82151,
#82152),.UNSPECIFIED.,.F.,.F.,(4,2,4),(2.55629243344565E-7,0.0321085924337593,
0.0654684152026825),.UNSPECIFIED.) ;
#1086=B_SPLINE_CURVE_WITH_KNOTS('',3,(#82194,#82195,#82196,#82197,#82198,
#82199,#82200,#82201),.UNSPECIFIED.,.F.,.F.,(4,2,2,4),(-0.0866902249621159,
-0.085595699976472,-0.0490110014082998,4.70756737529766E-5),
 .UNSPECIFIED.) ;
#1087=B_SPLINE_CURVE_WITH_KNOTS('',3,(#82203,#82204,#82205,#82206,#82207,
#82208,#82209,#82210,#82211,#82212,#82213,#82214,#82215,#82216,#82217,#82218,
#82219,#82220,#82221,#82222,#82223,#82224),.UNSPECIFIED.,.F.,.F.,(4,2,2,
2,2,2,2,2,2,2,4),(-0.0189091497005805,-0.0188216570693507,-0.0160930875609983,
-0.0140631752914572,-0.0113361432619141,-0.0108038868757659,-0.00937541885348054,
-0.0066320839853287,-0.00468769990948291,-0.00196658907698825,0.),
 .UNSPECIFIED.) ;
#1088=B_SPLINE_CURVE_WITH_KNOTS('',3,(#82225,#82226,#82227,#82228,#82229,
#82230,#82231,#82232,#82233,#82234,#82235,#82236,#82237,#82238,#82239,#82240,
#82241,#82242,#82243,#82244,#82245,#82246,#82247,#82248,#82249),
 .UNSPECIFIED.,.F.,.F.,(4,3,3,3,3,3,3,3,4),(1.57509957900154E-9,0.0132911426638058,
0.0269830849249619,0.0413877831821161,0.0490109714954551,0.0505389692183738,
0.0629605951743031,0.07447082612909,0.0855956752503445),.UNSPECIFIED.) ;
#1089=B_SPLINE_CURVE_WITH_KNOTS('',3,(#82306,#82307,#82308,#82309,#82310,
#82311),.UNSPECIFIED.,.F.,.F.,(4,2,4),(-0.0278988061061053,-0.0112807751130659,
-0.000904379645874189),.UNSPECIFIED.) ;
#1090=B_SPLINE_CURVE_WITH_KNOTS('',3,(#82312,#82313,#82314,#82315,#82316,
#82317,#82318,#82319,#82320,#82321,#82322,#82323,#82324,#82325),
 .UNSPECIFIED.,.F.,.F.,(4,2,2,2,2,2,4),(-0.0211430029019927,-0.0210263115451312,
-0.0147124541559798,-0.00942707088034509,-0.00482159977281412,-0.00241097745669264,
0.),.UNSPECIFIED.) ;
#1091=B_SPLINE_CURVE_WITH_KNOTS('',3,(#82359,#82360,#82361,#82362,#82363,
#82364),.UNSPECIFIED.,.F.,.F.,(4,2,4),(-0.0224313406438007,-0.0119728599231917,
-0.000668626710861112),.UNSPECIFIED.) ;
#1092=B_SPLINE_CURVE_WITH_KNOTS('',3,(#82365,#82366,#82367,#82368,#82369,
#82370,#82371,#82372,#82373,#82374,#82375,#82376,#82377,#82378,#82379,#82380,
#82381,#82382,#82383,#82384,#82385,#82386,#82387,#82388,#82389,#82390,#82391,
#82392,#82393,#82394,#82395),.UNSPECIFIED.,.F.,.F.,(4,3,3,3,3,3,3,3,3,3,
4),(-8.7628829834679E-5,0.,0.00273270250618685,0.00477794884587875,0.00750683894428588,
0.00802843590815977,0.00947056618272019,0.0122165071757717,0.0141556306430289,
0.0168758245379607,0.0188368670291837),.UNSPECIFIED.) ;
#1093=B_SPLINE_CURVE_WITH_KNOTS('',3,(#82427,#82428,#82429,#82430,#82431,
#82432),.UNSPECIFIED.,.F.,.F.,(4,2,4),(-0.0345946589883076,-0.0199847249930681,
-0.000207524979791521),.UNSPECIFIED.) ;
#1094=B_SPLINE_CURVE_WITH_KNOTS('',3,(#82433,#82434,#82435,#82436,#82437,
#82438,#82439,#82440,#82441,#82442,#82443,#82444,#82445,#82446,#82447,#82448,
#82449,#82450,#82451,#82452,#82453,#82454,#82455,#82456,#82457,#82458,#82459,
#82460,#82461,#82462,#82463),.UNSPECIFIED.,.F.,.F.,(4,3,3,3,3,3,3,3,3,3,
4),(-8.75050552364877E-5,0.,0.00272897052667188,0.00476026345104745,0.00748754551043703,
0.00801874653963784,0.00944846844817684,0.0121921607137149,0.0141359453584198,
0.0168569193374903,0.0188230526768059),.UNSPECIFIED.) ;
#1095=B_SPLINE_CURVE_WITH_KNOTS('',3,(#82494,#82495,#82496,#82497,#82498,
#82499),.UNSPECIFIED.,.F.,.F.,(4,2,4),(-0.0660759331217695,-0.0377278926030736,
-4.752274878301E-5),.UNSPECIFIED.) ;
#1096=B_SPLINE_CURVE_WITH_KNOTS('',3,(#83139,#83140,#83141,#83142,#83143,
#83144),.UNSPECIFIED.,.F.,.F.,(4,2,4),(-0.019402604569559,-0.0117562819132928,
0.),.UNSPECIFIED.) ;
#1097=B_SPLINE_CURVE_WITH_KNOTS('',3,(#83148,#83149,#83150,#83151,#83152,
#83153),.UNSPECIFIED.,.F.,.F.,(4,2,4),(-0.069955828573411,-0.0581995466601174,
-0.0505532240038506),.UNSPECIFIED.) ;
#1098=B_SPLINE_CURVE_WITH_KNOTS('',3,(#83283,#83284,#83285,#83286,#83287,
#83288),.UNSPECIFIED.,.F.,.F.,(4,2,4),(-0.069955828573407,-0.0581995466601109,
-0.05055322400384),.UNSPECIFIED.) ;
#1099=B_SPLINE_CURVE_WITH_KNOTS('',3,(#83307,#83308,#83309,#83310,#83311,
#83312),.UNSPECIFIED.,.F.,.F.,(4,2,4),(-0.0194026045695706,-0.0117562819132982,
3.46944695195361E-18),.UNSPECIFIED.) ;
#1100=B_SPLINE_CURVE_WITH_KNOTS('',3,(#83317,#83318,#83319,#83320,#83321,
#83322),.UNSPECIFIED.,.F.,.F.,(4,2,4),(-0.0699558285734111,-0.0581995466601248,
-0.0505532240038628),.UNSPECIFIED.) ;
#1101=B_SPLINE_CURVE_WITH_KNOTS('',3,(#83345,#83346,#83347,#83348,#83349,
#83350),.UNSPECIFIED.,.F.,.F.,(4,2,4),(-0.019402604569559,-0.0117562819132928,
0.),.UNSPECIFIED.) ;
#1102=B_SPLINE_CURVE_WITH_KNOTS('',3,(#83408,#83409,#83410,#83411,#83412,
#83413,#83414,#83415,#83416,#83417,#83418,#83419,#83420,#83421,#83422,#83423,
#83424,#83425),.UNSPECIFIED.,.T.,.F.,(4,1,1,1,1,1,1,1,1,1,1,1,1,1,1,4),
(-1.24903384766071,-1.07060044085204,-0.892167034043367,-0.713733627234693,
-0.53530022042602,-0.356866813617347,-0.178433406808673,0.0594778022695577,
0.118955604539115,0.178433406808673,0.356866813617347,0.53530022042602,
0.713733627234693,0.892167034043367,1.07060044085204,1.24903384766071),
 .UNSPECIFIED.) ;
#1103=B_SPLINE_CURVE_WITH_KNOTS('',3,(#83662,#83663,#83664,#83665,#83666),
 .UNSPECIFIED.,.F.,.F.,(4,1,4),(-1.,-0.571428571428571,0.),
 .UNSPECIFIED.) ;
#1104=B_SPLINE_CURVE_WITH_KNOTS('',3,(#83668,#83669,#83670,#83671,#83672,
#83673,#83674,#83675,#83676,#83677,#83678,#83679,#83680,#83681,#83682,#83683,
#83684,#83685),.UNSPECIFIED.,.F.,.F.,(4,1,1,1,1,1,1,1,1,1,1,1,1,1,1,4),
(-1.24887231172908,-1.07060044085204,-0.892167034043367,-0.713733627234693,
-0.53530022042602,-0.356866813617347,-0.178433406808673,-0.118955604539115,
-0.0594778022695577,0.178433406808673,0.356866813617347,0.53530022042602,
0.713733627234693,0.892167034043367,1.07060044085204,1.24854837899851),
 .UNSPECIFIED.) ;
#1105=B_SPLINE_CURVE_WITH_KNOTS('',3,(#83738,#83739,#83740,#83741,#83742),
 .UNSPECIFIED.,.F.,.F.,(4,1,4),(0.270884354171361,0.773477463983206,1.5707963267949),
 .UNSPECIFIED.) ;
#1106=B_SPLINE_CURVE_WITH_KNOTS('',3,(#83747,#83748,#83749,#83750,#83751),
 .UNSPECIFIED.,.F.,.F.,(4,1,4),(-1.57079632679489,-0.972068585273428,-0.27088435417137),
 .UNSPECIFIED.) ;
#1107=B_SPLINE_CURVE_WITH_KNOTS('',3,(#83787,#83788,#83789,#83790,#83791),
 .UNSPECIFIED.,.F.,.F.,(4,1,4),(-1.57079632679489,-0.972068585274832,-0.27088435417136),
 .UNSPECIFIED.) ;
#1108=B_SPLINE_CURVE_WITH_KNOTS('',3,(#83795,#83796,#83797,#83798,#83799),
 .UNSPECIFIED.,.F.,.F.,(4,1,4),(0.270884354171619,0.773477463983786,1.57079632679491),
 .UNSPECIFIED.) ;
#1109=B_SPLINE_CURVE_WITH_KNOTS('',3,(#83835,#83836,#83837,#83838,#83839,
#83840,#83841,#83842,#83843,#83844),.UNSPECIFIED.,.F.,.F.,(4,2,2,2,4),(0.,
0.00788303309691765,0.0119497367126136,0.015825892091812,0.0158931850550275),
 .UNSPECIFIED.) ;
#1110=B_SPLINE_CURVE_WITH_KNOTS('',3,(#83846,#83847,#83848,#83849,#83850,
#83851,#83852,#83853,#83854,#83855),.UNSPECIFIED.,.F.,.F.,(4,2,2,2,4),(-6.67745037823238E-5,
0.,0.00368652269857415,0.00752108608922011,0.0157260861811032),
 .UNSPECIFIED.) ;
#1111=B_SPLINE_CURVE_WITH_KNOTS('',3,(#83862,#83863,#83864,#83865,#83866,
#83867,#83868,#83869,#83870,#83871),.UNSPECIFIED.,.F.,.F.,(4,2,2,2,4),(0.,
0.00788283137687036,0.0119495587275004,0.0158257190872389,0.0158930122581911),
 .UNSPECIFIED.) ;
#1112=B_SPLINE_CURVE_WITH_KNOTS('',3,(#83873,#83874,#83875,#83876,#83877,
#83878,#83879,#83880,#83881,#83882),.UNSPECIFIED.,.F.,.F.,(4,2,2,2,4),(-6.70889521711013E-5,
0.,0.00367906803762835,0.00750255358812287,0.0157699191065211),
 .UNSPECIFIED.) ;
#1113=B_SPLINE_CURVE_WITH_KNOTS('',3,(#83899,#83900,#83901,#83902,#83903,
#83904,#83905,#83906,#83907,#83908,#83909,#83910,#83911,#83912,#83913,#83914,
#83915,#83916),.UNSPECIFIED.,.F.,.F.,(4,2,2,2,2,2,2,2,4),(0.,0.326127356006603,
0.557344647137824,0.584626694347595,0.59984323350605,0.617644550039615,
0.641541852563963,0.664074855441484,0.685580709784321),.UNSPECIFIED.) ;
#1114=B_SPLINE_CURVE_WITH_KNOTS('',3,(#83918,#83919,#83920,#83921,#83922,
#83923,#83924,#83925,#83926,#83927,#83928,#83929,#83930,#83931,#83932,#83933,
#83934,#83935),.UNSPECIFIED.,.F.,.F.,(4,2,2,2,2,2,2,2,4),(0.,0.0178986748860247,
0.030596894439968,0.0425739990891357,0.0508039795031799,0.0591630839826922,
0.0794036544378079,0.265037314904174,0.418714241056143),.UNSPECIFIED.) ;
#1115=B_SPLINE_CURVE_WITH_KNOTS('',3,(#83943,#83944,#83945,#83946,#83947,
#83948,#83949,#83950,#83951,#83952,#83953,#83954,#83955,#83956,#83957,#83958,
#83959,#83960),.UNSPECIFIED.,.F.,.F.,(4,2,2,2,2,2,2,2,4),(0.,0.326124834738013,
0.55734519302541,0.584627517143732,0.599844487527337,0.617646472342995,
0.641544788167125,0.664078789501966,0.685585439526425),.UNSPECIFIED.) ;
#1116=B_SPLINE_CURVE_WITH_KNOTS('',3,(#83962,#83963,#83964,#83965,#83966,
#83967,#83968,#83969,#83970,#83971,#83972,#83973,#83974,#83975,#83976,#83977,
#83978,#83979),.UNSPECIFIED.,.F.,.F.,(4,2,2,2,2,2,2,2,4),(0.,0.0178988264704468,
0.0305964768111414,0.0425728428045337,0.0508022993033077,0.0591609218800705,
0.0794005119967651,0.26502301977072,0.418693046005869),.UNSPECIFIED.) ;
#1117=B_SPLINE_CURVE_WITH_KNOTS('',3,(#83987,#83988,#83989,#83990),
 .UNSPECIFIED.,.F.,.F.,(4,4),(-0.400732539131533,-0.390705386116278),
 .UNSPECIFIED.) ;
#1118=B_SPLINE_CURVE_WITH_KNOTS('',3,(#83994,#83995,#83996,#83997,#83998),
 .UNSPECIFIED.,.F.,.F.,(4,1,4),(-0.0173570618196939,-0.00867853090984697,
0.),.UNSPECIFIED.) ;
#1119=B_SPLINE_CURVE_WITH_KNOTS('',3,(#84003,#84004,#84005,#84006,#84007,
#84008,#84009,#84010,#84011,#84012,#84013,#84014,#84015),.UNSPECIFIED.,
 .F.,.F.,(4,2,2,2,3,4),(-0.0524538649298037,-0.0454382448332118,-0.0301309134460882,
-0.0150654567230441,0.,0.00806831493386506),.UNSPECIFIED.) ;
#1120=B_SPLINE_CURVE_WITH_KNOTS('',3,(#84062,#84063,#84064,#84065,#84066,
#84067,#84068,#84069,#84070,#84071,#84072,#84073,#84074,#84075,#84076,#84077,
#84078,#84079,#84080),.UNSPECIFIED.,.F.,.F.,(4,3,3,3,3,3,4),(0.390705386116286,
0.392851683870094,0.394821897685454,0.396624148064999,0.39837845519803,
0.400094449296349,0.400732539131533),.UNSPECIFIED.) ;
#1121=B_SPLINE_CURVE_WITH_KNOTS('',3,(#84111,#84112,#84113,#84114,#84115),
 .UNSPECIFIED.,.F.,.F.,(4,1,4),(0.,0.00867853090984697,0.0173570618196939),
 .UNSPECIFIED.) ;
#1122=B_SPLINE_CURVE_WITH_KNOTS('',3,(#84138,#84139,#84140,#84141,#84142,
#84143,#84144,#84145,#84146,#84147,#84148,#84149),.UNSPECIFIED.,.F.,.F.,
(4,2,2,2,2,4),(-0.13141454633876,-0.123346231404894,-0.108280774681851,
-0.0932153179588078,-0.0779079865716814,-0.0708923664750809),
 .UNSPECIFIED.) ;
#1123=B_SPLINE_CURVE_WITH_KNOTS('',3,(#84151,#84152,#84153,#84154,#84155),
 .UNSPECIFIED.,.F.,.F.,(4,1,4),(0.276503853136672,0.620020769070722,1.),
 .UNSPECIFIED.) ;
#1124=B_SPLINE_CURVE_WITH_KNOTS('',3,(#86302,#86303,#86304,#86305,#86306),
 .UNSPECIFIED.,.F.,.F.,(4,1,4),(-1.,-0.622952086196121,-0.276501380066297),
 .UNSPECIFIED.) ;
#1125=B_SPLINE_CURVE_WITH_KNOTS('',3,(#86308,#86309,#86310,#86311,#86312),
 .UNSPECIFIED.,.F.,.F.,(4,1,4),(-1.,-0.622952086196224,-0.276501383761116),
 .UNSPECIFIED.) ;
#1126=B_SPLINE_CURVE_WITH_KNOTS('',3,(#86316,#86317,#86318,#86319,#86320),
 .UNSPECIFIED.,.F.,.F.,(4,1,4),(0.27650384808904,0.620020769070722,1.),
 .UNSPECIFIED.) ;
#1917=B_SPLINE_SURFACE_WITH_KNOTS('',3,3,((#79198,#79199,#79200,#79201,
#79202,#79203,#79204,#79205,#79206,#79207),(#79208,#79209,#79210,#79211,
#79212,#79213,#79214,#79215,#79216,#79217),(#79218,#79219,#79220,#79221,
#79222,#79223,#79224,#79225,#79226,#79227),(#79228,#79229,#79230,#79231,
#79232,#79233,#79234,#79235,#79236,#79237),(#79238,#79239,#79240,#79241,
#79242,#79243,#79244,#79245,#79246,#79247)),.UNSPECIFIED.,.F.,.F.,.F.,(4,
1,4),(4,2,2,2,4),(0.,0.571428571428571,1.),(-0.000984424941950333,0.,0.0304393222729151,
0.0604225486602068,0.0620633422654789),.UNSPECIFIED.) ;
#1918=B_SPLINE_SURFACE_WITH_KNOTS('',3,3,((#79324,#79325,#79326,#79327,
#79328,#79329,#79330,#79331),(#79332,#79333,#79334,#79335,#79336,#79337,
#79338,#79339),(#79340,#79341,#79342,#79343,#79344,#79345,#79346,#79347),
(#79348,#79349,#79350,#79351,#79352,#79353,#79354,#79355),(#79356,#79357,
#79358,#79359,#79360,#79361,#79362,#79363)),.UNSPECIFIED.,.F.,.F.,.F.,(4,
1,4),(4,2,2,4),(0.,0.571428571428571,1.),(-6.37514627733282E-5,0.0340909276764841,
0.0604383336928468,0.061399226101535),.UNSPECIFIED.) ;
#1919=B_SPLINE_SURFACE_WITH_KNOTS('',3,3,((#79421,#79422,#79423,#79424,
#79425,#79426,#79427,#79428,#79429,#79430),(#79431,#79432,#79433,#79434,
#79435,#79436,#79437,#79438,#79439,#79440),(#79441,#79442,#79443,#79444,
#79445,#79446,#79447,#79448,#79449,#79450),(#79451,#79452,#79453,#79454,
#79455,#79456,#79457,#79458,#79459,#79460),(#79461,#79462,#79463,#79464,
#79465,#79466,#79467,#79468,#79469,#79470)),.UNSPECIFIED.,.F.,.F.,.F.,(4,
1,4),(4,2,2,2,4),(0.,0.571428571428571,1.),(-0.0016406621045341,0.,0.032656775096122,
0.0751675585986371,0.0752925967203965),.UNSPECIFIED.) ;
#1920=B_SPLINE_SURFACE_WITH_KNOTS('',3,3,((#79556,#79557,#79558,#79559,
#79560,#79561,#79562,#79563,#79564,#79565),(#79566,#79567,#79568,#79569,
#79570,#79571,#79572,#79573,#79574,#79575),(#79576,#79577,#79578,#79579,
#79580,#79581,#79582,#79583,#79584,#79585),(#79586,#79587,#79588,#79589,
#79590,#79591,#79592,#79593,#79594,#79595),(#79596,#79597,#79598,#79599,
#79600,#79601,#79602,#79603,#79604,#79605)),.UNSPECIFIED.,.F.,.F.,.F.,(4,
1,4),(4,2,2,2,4),(0.,0.571428571428571,1.),(-0.00096080851771424,0.,0.0235600635035843,
0.0457311162964727,0.0467303873666823),.UNSPECIFIED.) ;
#1921=B_SPLINE_SURFACE_WITH_KNOTS('',3,3,((#79638,#79639,#79640,#79641,
#79642,#79643,#79644,#79645,#79646,#79647),(#79648,#79649,#79650,#79651,
#79652,#79653,#79654,#79655,#79656,#79657),(#79658,#79659,#79660,#79661,
#79662,#79663,#79664,#79665,#79666,#79667),(#79668,#79669,#79670,#79671,
#79672,#79673,#79674,#79675,#79676,#79677),(#79678,#79679,#79680,#79681,
#79682,#79683,#79684,#79685,#79686,#79687)),.UNSPECIFIED.,.F.,.F.,.F.,(4,
1,4),(4,2,2,2,4),(0.,0.571428571428571,1.),(-0.000999294135844071,0.,0.0217198699392343,
0.0432144526123464,0.0441989132427654),.UNSPECIFIED.) ;
#1922=B_SPLINE_SURFACE_WITH_KNOTS('',3,1,((#79740,#79741),(#79742,#79743),
(#79744,#79745),(#79746,#79747),(#79748,#79749)),.UNSPECIFIED.,.F.,.F.,
 .F.,(4,1,4),(2,2),(0.,0.0323852950215525,0.0574227556854303),(0.,0.0360000000000003),
 .UNSPECIFIED.) ;
#1923=B_SPLINE_SURFACE_WITH_KNOTS('',3,3,((#79928,#79929,#79930,#79931,
#79932,#79933,#79934,#79935),(#79936,#79937,#79938,#79939,#79940,#79941,
#79942,#79943),(#79944,#79945,#79946,#79947,#79948,#79949,#79950,#79951),
(#79952,#79953,#79954,#79955,#79956,#79957,#79958,#79959),(#79960,#79961,
#79962,#79963,#79964,#79965,#79966,#79967)),.UNSPECIFIED.,.F.,.F.,.F.,(4,
1,4),(4,2,2,4),(0.,0.571428571428571,1.),(-4.75219968878011E-5,0.0386336727204952,
0.0678747004384468,0.0680822294122733),.UNSPECIFIED.) ;
#1924=B_SPLINE_SURFACE_WITH_KNOTS('',3,3,((#80009,#80010,#80011,#80012,
#80013,#80014,#80015,#80016,#80017,#80018),(#80019,#80020,#80021,#80022,
#80023,#80024,#80025,#80026,#80027,#80028),(#80029,#80030,#80031,#80032,
#80033,#80034,#80035,#80036,#80037,#80038),(#80039,#80040,#80041,#80042,
#80043,#80044,#80045,#80046,#80047,#80048),(#80049,#80050,#80051,#80052,
#80053,#80054,#80055,#80056,#80057,#80058)),.UNSPECIFIED.,.F.,.F.,.F.,(4,
1,4),(4,2,2,2,4),(0.,0.571428571428571,1.),(-0.000207465766990066,0.,0.0232646742763639,
0.0410522705936588,0.041721226167804),.UNSPECIFIED.) ;
#1925=B_SPLINE_SURFACE_WITH_KNOTS('',3,3,((#80119,#80120,#80121,#80122,
#80123,#80124),(#80125,#80126,#80127,#80128,#80129,#80130),(#80131,#80132,
#80133,#80134,#80135,#80136),(#80137,#80138,#80139,#80140,#80141,#80142),
(#80143,#80144,#80145,#80146,#80147,#80148)),.UNSPECIFIED.,.F.,.F.,.F.,
(4,1,4),(4,2,4),(0.,0.571428571428571,1.),(-2.08166817117217E-17,0.0453812948763195,
0.0792555822118552),.UNSPECIFIED.) ;
#1926=B_SPLINE_SURFACE_WITH_KNOTS('',3,3,((#80172,#80173,#80174,#80175,
#80176,#80177,#80178,#80179,#80180,#80181),(#80182,#80183,#80184,#80185,
#80186,#80187,#80188,#80189,#80190,#80191),(#80192,#80193,#80194,#80195,
#80196,#80197,#80198,#80199,#80200,#80201),(#80202,#80203,#80204,#80205,
#80206,#80207,#80208,#80209,#80210,#80211),(#80212,#80213,#80214,#80215,
#80216,#80217,#80218,#80219,#80220,#80221)),.UNSPECIFIED.,.F.,.F.,.F.,(4,
1,4),(4,2,2,2,4),(0.,0.571428571428571,1.),(-0.000668949496694549,0.,0.0150950300818429,
0.0294213468333971,0.0303251295908459),.UNSPECIFIED.) ;
#1927=B_SPLINE_SURFACE_WITH_KNOTS('',3,3,((#80269,#80270,#80271,#80272,
#80273,#80274,#80275,#80276),(#80277,#80278,#80279,#80280,#80281,#80282,
#80283,#80284),(#80285,#80286,#80287,#80288,#80289,#80290,#80291,#80292),
(#80293,#80294,#80295,#80296,#80297,#80298,#80299,#80300),(#80301,#80302,
#80303,#80304,#80305,#80306,#80307,#80308)),.UNSPECIFIED.,.F.,.F.,.F.,(4,
1,4),(4,2,2,4),(0.,0.571428571428571,1.),(-0.000903812556791651,0.,0.0126332411015006,
0.0312404144905361),.UNSPECIFIED.) ;
#1928=B_SPLINE_SURFACE_WITH_KNOTS('',3,3,((#80345,#80346,#80347,#80348,
#80349,#80350,#80351,#80352),(#80353,#80354,#80355,#80356,#80357,#80358,
#80359,#80360),(#80361,#80362,#80363,#80364,#80365,#80366,#80367,#80368),
(#80369,#80370,#80371,#80372,#80373,#80374,#80375,#80376),(#80377,#80378,
#80379,#80380,#80381,#80382,#80383,#80384)),.UNSPECIFIED.,.F.,.F.,.F.,(4,
1,4),(4,1,2,1,4),(0.,0.571428571428571,1.),(-6.07153216596483E-15,0.0104867604235457,
0.0262169010588733,0.0371127510104888,0.0534565259379121),.UNSPECIFIED.) ;
#1929=B_SPLINE_SURFACE_WITH_KNOTS('',3,3,((#80428,#80429,#80430,#80431,
#80432,#80433),(#80434,#80435,#80436,#80437,#80438,#80439),(#80440,#80441,
#80442,#80443,#80444,#80445),(#80446,#80447,#80448,#80449,#80450,#80451),
(#80452,#80453,#80454,#80455,#80456,#80457)),.UNSPECIFIED.,.F.,.F.,.F.,
(4,1,4),(4,2,4),(0.,0.571428571428571,1.),(-1.19054072156493E-14,0.0289083223985083,
0.0583191426684248),.UNSPECIFIED.) ;
#1930=B_SPLINE_SURFACE_WITH_KNOTS('',3,3,((#80533,#80534,#80535,#80536,
#80537,#80538,#80539,#80540),(#80541,#80542,#80543,#80544,#80545,#80546,
#80547,#80548),(#80549,#80550,#80551,#80552,#80553,#80554,#80555,#80556),
(#80557,#80558,#80559,#80560,#80561,#80562,#80563,#80564),(#80565,#80566,
#80567,#80568,#80569,#80570,#80571,#80572)),.UNSPECIFIED.,.F.,.F.,.F.,(4,
1,4),(4,1,2,1,4),(0.,0.571428571428571,1.),(-1.21551489931584E-15,0.021868453247988,
0.0364474220799808,0.0505556257289287,0.0717179312023507),.UNSPECIFIED.) ;
#1931=B_SPLINE_SURFACE_WITH_KNOTS('',3,3,((#80619,#80620,#80621,#80622,
#80623,#80624,#80625,#80626),(#80627,#80628,#80629,#80630,#80631,#80632,
#80633,#80634),(#80635,#80636,#80637,#80638,#80639,#80640,#80641,#80642),
(#80643,#80644,#80645,#80646,#80647,#80648,#80649,#80650),(#80651,#80652,
#80653,#80654,#80655,#80656,#80657,#80658),(#80659,#80660,#80661,#80662,
#80663,#80664,#80665,#80666)),.UNSPECIFIED.,.F.,.F.,.F.,(4,1,1,4),(4,2,
2,4),(0.,0.142857142857143,0.571428571428571,1.),(-3.34298561055327E-14,
0.0398009040484053,0.0884506599106943,0.125182168962163),.UNSPECIFIED.) ;
#1932=B_SPLINE_SURFACE_WITH_KNOTS('',3,3,((#80688,#80689,#80690,#80691,
#80692,#80693,#80694,#80695),(#80696,#80697,#80698,#80699,#80700,#80701,
#80702,#80703),(#80704,#80705,#80706,#80707,#80708,#80709,#80710,#80711),
(#80712,#80713,#80714,#80715,#80716,#80717,#80718,#80719),(#80720,#80721,
#80722,#80723,#80724,#80725,#80726,#80727)),.UNSPECIFIED.,.F.,.F.,.F.,(4,
1,4),(4,2,2,4),(0.,0.571428571428571,1.),(-0.0369647188766498,0.,0.0196661092474417,
0.0352658770408685),.UNSPECIFIED.) ;
#1933=B_SPLINE_SURFACE_WITH_KNOTS('',3,3,((#80766,#80767,#80768,#80769,
#80770,#80771),(#80772,#80773,#80774,#80775,#80776,#80777),(#80778,#80779,
#80780,#80781,#80782,#80783),(#80784,#80785,#80786,#80787,#80788,#80789),
(#80790,#80791,#80792,#80793,#80794,#80795)),.UNSPECIFIED.,.F.,.F.,.F.,
(4,1,4),(4,2,4),(0.,0.571428571428571,1.),(0.,0.0318468005485353,0.0669038356909525),
 .UNSPECIFIED.) ;
#1934=B_SPLINE_SURFACE_WITH_KNOTS('',3,1,((#80830,#80831),(#80832,#80833),
(#80834,#80835),(#80836,#80837),(#80838,#80839)),.UNSPECIFIED.,.F.,.F.,
 .F.,(4,1,4),(2,2),(0.,0.0210301296927785,0.0377156586265697),(0.,0.0360000000000003),
 .UNSPECIFIED.) ;
#1935=B_SPLINE_SURFACE_WITH_KNOTS('',3,1,((#80850,#80851),(#80852,#80853),
(#80854,#80855),(#80856,#80857),(#80858,#80859)),.UNSPECIFIED.,.F.,.F.,
 .F.,(4,1,4),(2,2),(0.,0.0329095469988702,0.0691336974954879),(0.,0.0360000000000003),
 .UNSPECIFIED.) ;
#1936=B_SPLINE_SURFACE_WITH_KNOTS('',3,1,((#80880,#80881),(#80882,#80883),
(#80884,#80885),(#80886,#80887),(#80888,#80889)),.UNSPECIFIED.,.F.,.F.,
 .F.,(4,1,4),(2,2),(0.,0.0381782469542568,0.0670753371474822),(0.,0.0360000000000003),
 .UNSPECIFIED.) ;
#1937=B_SPLINE_SURFACE_WITH_KNOTS('',3,1,((#80898,#80899),(#80900,#80901),
(#80902,#80903),(#80904,#80905),(#80906,#80907)),.UNSPECIFIED.,.F.,.F.,
 .F.,(4,1,4),(2,2),(0.,0.0216058216755205,0.0381303842659523),(0.,0.0360000000000003),
 .UNSPECIFIED.) ;
#1938=B_SPLINE_SURFACE_WITH_KNOTS('',3,1,((#80916,#80917),(#80918,#80919),
(#80920,#80921),(#80922,#80923),(#80924,#80925)),.UNSPECIFIED.,.F.,.F.,
 .F.,(4,1,4),(2,2),(0.,0.0135228484064754,0.0263579081616444),(0.,0.0360000000000003),
 .UNSPECIFIED.) ;
#1939=B_SPLINE_SURFACE_WITH_KNOTS('',3,1,((#80962,#80963),(#80964,#80965),
(#80966,#80967),(#80968,#80969),(#80970,#80971)),.UNSPECIFIED.,.F.,.F.,
 .F.,(4,1,4),(2,2),(0.,0.011955158932918,0.0295605475166918),(0.,0.0360000000000003),
 .UNSPECIFIED.) ;
#1940=B_SPLINE_SURFACE_WITH_KNOTS('',3,3,((#80984,#80985,#80986,#80987,
#80988,#80989,#80990,#80991),(#80992,#80993,#80994,#80995,#80996,#80997,
#80998,#80999),(#81000,#81001,#81002,#81003,#81004,#81005,#81006,#81007),
(#81008,#81009,#81010,#81011,#81012,#81013,#81014,#81015),(#81016,#81017,
#81018,#81019,#81020,#81021,#81022,#81023)),.UNSPECIFIED.,.F.,.F.,.F.,(4,
1,4),(4,1,2,1,4),(0.,0.571428571428571,1.),(-6.50365178378404E-14,0.0105495395664116,
0.0175825659440626,0.0275093508272253,0.0341272074160004),.UNSPECIFIED.) ;
#1941=B_SPLINE_SURFACE_WITH_KNOTS('',3,3,((#81119,#81120,#81121,#81122,
#81123,#81124,#81125),(#81126,#81127,#81128,#81129,#81130,#81131,#81132),
(#81133,#81134,#81135,#81136,#81137,#81138,#81139),(#81140,#81141,#81142,
#81143,#81144,#81145,#81146),(#81147,#81148,#81149,#81150,#81151,#81152,
#81153),(#81154,#81155,#81156,#81157,#81158,#81159,#81160)),
 .UNSPECIFIED.,.F.,.F.,.F.,(4,1,1,4),(4,2,1,4),(0.,0.142857142857143,0.571428571428571,
1.),(-8.68229099727415E-16,0.0271030272865255,0.0412193079076597,0.062393728839361),
 .UNSPECIFIED.) ;
#1942=B_SPLINE_SURFACE_WITH_KNOTS('',3,3,((#81229,#81230,#81231,#81232,
#81233,#81234,#81235,#81236,#81237),(#81238,#81239,#81240,#81241,#81242,
#81243,#81244,#81245,#81246),(#81247,#81248,#81249,#81250,#81251,#81252,
#81253,#81254,#81255),(#81256,#81257,#81258,#81259,#81260,#81261,#81262,
#81263,#81264),(#81265,#81266,#81267,#81268,#81269,#81270,#81271,#81272,
#81273),(#81274,#81275,#81276,#81277,#81278,#81279,#81280,#81281,#81282)),
 .UNSPECIFIED.,.F.,.F.,.F.,(4,1,1,4),(4,1,2,1,1,4),(0.,0.285714285714286,
0.571428571428571,1.),(0.,0.00901895895784998,0.0225473973946249,0.0269891467103356,
0.0314308960260463,0.044761249451505),.UNSPECIFIED.) ;
#1943=B_SPLINE_SURFACE_WITH_KNOTS('',3,3,((#81386,#81387,#81388,#81389,
#81390,#81391,#81392,#81393),(#81394,#81395,#81396,#81397,#81398,#81399,
#81400,#81401),(#81402,#81403,#81404,#81405,#81406,#81407,#81408,#81409),
(#81410,#81411,#81412,#81413,#81414,#81415,#81416,#81417),(#81418,#81419,
#81420,#81421,#81422,#81423,#81424,#81425)),.UNSPECIFIED.,.F.,.F.,.F.,(4,
1,4),(4,1,2,1,4),(0.,0.571428571428571,1.),(-3.8936437845742E-15,0.00990987059888721,
0.016516450998148,0.0263234394910323,0.0328614318196219),.UNSPECIFIED.) ;
#1944=B_SPLINE_SURFACE_WITH_KNOTS('',3,3,((#81480,#81481,#81482,#81483,
#81484,#81485),(#81486,#81487,#81488,#81489,#81490,#81491),(#81492,#81493,
#81494,#81495,#81496,#81497),(#81498,#81499,#81500,#81501,#81502,#81503),
(#81504,#81505,#81506,#81507,#81508,#81509)),.UNSPECIFIED.,.F.,.F.,.F.,
(4,1,4),(4,2,4),(0.,0.571428571428571,1.),(-7.30609319335548E-6,0.0307388136698783,
0.0544948017664183),.UNSPECIFIED.) ;
#1945=B_SPLINE_SURFACE_WITH_KNOTS('',3,3,((#81635,#81636,#81637,#81638,
#81639,#81640,#81641,#81642,#81643,#81644),(#81645,#81646,#81647,#81648,
#81649,#81650,#81651,#81652,#81653,#81654),(#81655,#81656,#81657,#81658,
#81659,#81660,#81661,#81662,#81663,#81664),(#81665,#81666,#81667,#81668,
#81669,#81670,#81671,#81672,#81673,#81674),(#81675,#81676,#81677,#81678,
#81679,#81680,#81681,#81682,#81683,#81684)),.UNSPECIFIED.,.F.,.F.,.F.,(4,
1,4),(4,2,2,2,4),(0.,0.571428571428571,1.),(-0.000721914453027042,0.,0.033998052296077,
0.0714230469344481,0.0715962515154608),.UNSPECIFIED.) ;
#1946=B_SPLINE_SURFACE_WITH_KNOTS('',3,3,((#81730,#81731,#81732,#81733,
#81734,#81735,#81736,#81737),(#81738,#81739,#81740,#81741,#81742,#81743,
#81744,#81745),(#81746,#81747,#81748,#81749,#81750,#81751,#81752,#81753),
(#81754,#81755,#81756,#81757,#81758,#81759,#81760,#81761),(#81762,#81763,
#81764,#81765,#81766,#81767,#81768,#81769)),.UNSPECIFIED.,.F.,.F.,.F.,(4,
1,4),(4,2,2,4),(0.,0.571428571428571,1.),(5.55111512312578E-17,0.0224201537133612,
0.0402049350827121,0.0409268414934542),.UNSPECIFIED.) ;
#1947=B_SPLINE_SURFACE_WITH_KNOTS('',3,3,((#81797,#81798,#81799,#81800,
#81801,#81802,#81803,#81804),(#81805,#81806,#81807,#81808,#81809,#81810,
#81811,#81812),(#81813,#81814,#81815,#81816,#81817,#81818,#81819,#81820),
(#81821,#81822,#81823,#81824,#81825,#81826,#81827,#81828),(#81829,#81830,
#81831,#81832,#81833,#81834,#81835,#81836)),.UNSPECIFIED.,.F.,.F.,.F.,(4,
1,4),(4,2,2,4),(0.,0.571428571428571,1.),(-0.00145402880520905,0.,0.0452350077421772,
0.100520135955306),.UNSPECIFIED.) ;
#1948=B_SPLINE_SURFACE_WITH_KNOTS('',3,3,((#81867,#81868,#81869,#81870,
#81871,#81872,#81873,#81874,#81875,#81876),(#81877,#81878,#81879,#81880,
#81881,#81882,#81883,#81884,#81885,#81886),(#81887,#81888,#81889,#81890,
#81891,#81892,#81893,#81894,#81895,#81896),(#81897,#81898,#81899,#81900,
#81901,#81902,#81903,#81904,#81905,#81906),(#81907,#81908,#81909,#81910,
#81911,#81912,#81913,#81914,#81915,#81916)),.UNSPECIFIED.,.F.,.F.,.F.,(4,
1,4),(4,2,2,2,4),(0.,0.571428571428571,1.),(-0.000848777061136591,0.,0.0435056845362515,
0.0856081292457083,0.0870620753300636),.UNSPECIFIED.) ;
#1949=B_SPLINE_SURFACE_WITH_KNOTS('',3,3,((#81969,#81970,#81971,#81972,
#81973,#81974,#81975,#81976,#81977,#81978),(#81979,#81980,#81981,#81982,
#81983,#81984,#81985,#81986,#81987,#81988),(#81989,#81990,#81991,#81992,
#81993,#81994,#81995,#81996,#81997,#81998),(#81999,#82000,#82001,#82002,
#82003,#82004,#82005,#82006,#82007,#82008),(#82009,#82010,#82011,#82012,
#82013,#82014,#82015,#82016,#82017,#82018)),.UNSPECIFIED.,.F.,.F.,.F.,(4,
1,4),(4,2,2,2,4),(0.,0.571428571428571,1.),(-0.000832239105180238,0.,0.0338448162467367,
0.0682776647009788,0.0691265383481362),.UNSPECIFIED.) ;
#1950=B_SPLINE_SURFACE_WITH_KNOTS('',3,3,((#82071,#82072,#82073,#82074,
#82075,#82076,#82077,#82078,#82079,#82080),(#82081,#82082,#82083,#82084,
#82085,#82086,#82087,#82088,#82089,#82090),(#82091,#82092,#82093,#82094,
#82095,#82096,#82097,#82098,#82099,#82100),(#82101,#82102,#82103,#82104,
#82105,#82106,#82107,#82108,#82109,#82110),(#82111,#82112,#82113,#82114,
#82115,#82116,#82117,#82118,#82119,#82120)),.UNSPECIFIED.,.F.,.F.,.F.,(4,
1,4),(4,2,2,2,4),(0.,0.571428571428571,1.),(-0.00109408852437443,0.,0.0321085924337593,
0.065468485698588,0.0663005130080268),.UNSPECIFIED.) ;
#1951=B_SPLINE_SURFACE_WITH_KNOTS('',3,3,((#82153,#82154,#82155,#82156,
#82157,#82158,#82159,#82160),(#82161,#82162,#82163,#82164,#82165,#82166,
#82167,#82168),(#82169,#82170,#82171,#82172,#82173,#82174,#82175,#82176),
(#82177,#82178,#82179,#82180,#82181,#82182,#82183,#82184),(#82185,#82186,
#82187,#82188,#82189,#82190,#82191,#82192)),.UNSPECIFIED.,.F.,.F.,.F.,(4,
1,4),(4,2,2,4),(0.,0.571428571428571,1.),(-4.70756737529766E-5,0.0490110014082998,
0.085595699976472,0.0866902249621159),.UNSPECIFIED.) ;
#1952=B_SPLINE_SURFACE_WITH_KNOTS('',3,3,((#82273,#82274,#82275,#82276,
#82277,#82278),(#82279,#82280,#82281,#82282,#82283,#82284),(#82285,#82286,
#82287,#82288,#82289,#82290),(#82291,#82292,#82293,#82294,#82295,#82296),
(#82297,#82298,#82299,#82300,#82301,#82302)),.UNSPECIFIED.,.F.,.F.,.F.,
(4,1,4),(4,2,4),(0.,0.571428571428571,1.),(-3.37568514807661E-14,0.0112807751130659,
0.0278988061061053),.UNSPECIFIED.) ;
#1953=B_SPLINE_SURFACE_WITH_KNOTS('',3,3,((#82328,#82329,#82330,#82331,
#82332,#82333),(#82334,#82335,#82336,#82337,#82338,#82339),(#82340,#82341,
#82342,#82343,#82344,#82345),(#82346,#82347,#82348,#82349,#82350,#82351),
(#82352,#82353,#82354,#82355,#82356,#82357)),.UNSPECIFIED.,.F.,.F.,.F.,
(4,1,4),(4,2,4),(0.,0.571428571428571,1.),(-4.8815118613983E-15,0.0119728599231917,
0.023335857822899),.UNSPECIFIED.) ;
#1954=B_SPLINE_SURFACE_WITH_KNOTS('',3,3,((#82396,#82397,#82398,#82399,
#82400,#82401),(#82402,#82403,#82404,#82405,#82406,#82407),(#82408,#82409,
#82410,#82411,#82412,#82413),(#82414,#82415,#82416,#82417,#82418,#82419),
(#82420,#82421,#82422,#82423,#82424,#82425)),.UNSPECIFIED.,.F.,.F.,.F.,
(4,1,4),(4,2,4),(0.,0.571428571428571,1.),(-2.77555756156289E-17,0.0199847249930681,
0.0352638829354677),.UNSPECIFIED.) ;
#1955=B_SPLINE_SURFACE_WITH_KNOTS('',3,3,((#82464,#82465,#82466,#82467,
#82468,#82469),(#82470,#82471,#82472,#82473,#82474,#82475),(#82476,#82477,
#82478,#82479,#82480,#82481),(#82482,#82483,#82484,#82485,#82486,#82487),
(#82488,#82489,#82490,#82491,#82492,#82493)),.UNSPECIFIED.,.F.,.F.,.F.,
(4,1,4),(4,2,4),(-2.09809871143395E-6,0.571428571428571,1.00000209810189),
(-7.54436050495102E-6,0.0377278926030736,0.066283338281117),
 .UNSPECIFIED.) ;
#1956=B_SPLINE_SURFACE_WITH_KNOTS('',3,1,((#82502,#82503),(#82504,#82505),
(#82506,#82507),(#82508,#82509),(#82510,#82511)),.UNSPECIFIED.,.F.,.F.,
 .F.,(4,1,4),(2,2),(0.,0.0398228695438388,0.0783699334705556),(0.,0.0360000000000003),
 .UNSPECIFIED.) ;
#1957=B_SPLINE_SURFACE_WITH_KNOTS('',3,1,((#82514,#82515),(#82516,#82517),
(#82518,#82519),(#82520,#82521),(#82522,#82523)),.UNSPECIFIED.,.F.,.F.,
 .F.,(4,1,4),(2,2),(0.,0.0313133324080373,0.063168759987351),(0.,0.0360000000000003),
 .UNSPECIFIED.) ;
#1958=B_SPLINE_SURFACE_WITH_KNOTS('',3,1,((#82525,#82526),(#82527,#82528),
(#82529,#82530),(#82531,#82532),(#82533,#82534)),.UNSPECIFIED.,.F.,.F.,
 .F.,(4,1,4),(2,2),(0.,0.0290828541577381,0.0592932101613289),(0.,0.0360000000000003),
 .UNSPECIFIED.) ;
#1959=B_SPLINE_SURFACE_WITH_KNOTS('',3,1,((#82536,#82537),(#82538,#82539),
(#82540,#82541),(#82542,#82543),(#82544,#82545)),.UNSPECIFIED.,.F.,.F.,
 .F.,(4,1,4),(2,2),(0.,0.0471458586470647,0.0823534588635132),(0.,0.0360000000000003),
 .UNSPECIFIED.) ;
#1960=B_SPLINE_SURFACE_WITH_KNOTS('',3,1,((#82958,#82959),(#82960,#82961),
(#82962,#82963),(#82964,#82965),(#82966,#82967)),.UNSPECIFIED.,.F.,.F.,
 .F.,(4,1,4),(2,2),(0.,0.0298071351389365,0.0685496713495228),(0.,0.0360000000000003),
 .UNSPECIFIED.) ;
#1961=B_SPLINE_SURFACE_WITH_KNOTS('',3,1,((#82969,#82970),(#82971,#82972),
(#82973,#82974),(#82975,#82976),(#82977,#82978)),.UNSPECIFIED.,.F.,.F.,
 .F.,(4,1,4),(2,2),(0.,0.0263673128827931,0.0523427870633456),(0.,0.0360000000000003),
 .UNSPECIFIED.) ;
#1962=B_SPLINE_SURFACE_WITH_KNOTS('',3,1,((#82980,#82981),(#82982,#82983),
(#82984,#82985),(#82986,#82987),(#82988,#82989)),.UNSPECIFIED.,.F.,.F.,
 .F.,(4,1,4),(2,2),(0.,0.0190758281807941,0.0379545209982657),(0.,0.0360000000000003),
 .UNSPECIFIED.) ;
#1963=B_SPLINE_SURFACE_WITH_KNOTS('',3,1,((#82991,#82992),(#82993,#82994),
(#82995,#82996),(#82997,#82998),(#82999,#83000)),.UNSPECIFIED.,.F.,.F.,
 .F.,(4,1,4),(2,2),(0.,0.0205128997765721,0.0398218276255599),(0.,0.0360000000000003),
 .UNSPECIFIED.) ;
#1964=B_SPLINE_SURFACE_WITH_KNOTS('',3,1,((#83001,#83002),(#83003,#83004),
(#83005,#83006),(#83007,#83008),(#83009,#83010)),.UNSPECIFIED.,.F.,.F.,
 .F.,(4,1,4),(2,2),(0.,0.0424180496051088,0.0942055476140892),(0.,0.0360000000000003),
 .UNSPECIFIED.) ;
#1965=B_SPLINE_SURFACE_WITH_KNOTS('',3,3,((#83571,#83572,#83573,#83574,
#83575,#83576,#83577,#83578,#83579,#83580,#83581,#83582,#83583,#83584,#83585,
#83586,#83587,#83588),(#83589,#83590,#83591,#83592,#83593,#83594,#83595,
#83596,#83597,#83598,#83599,#83600,#83601,#83602,#83603,#83604,#83605,#83606),
(#83607,#83608,#83609,#83610,#83611,#83612,#83613,#83614,#83615,#83616,
#83617,#83618,#83619,#83620,#83621,#83622,#83623,#83624),(#83625,#83626,
#83627,#83628,#83629,#83630,#83631,#83632,#83633,#83634,#83635,#83636,#83637,
#83638,#83639,#83640,#83641,#83642),(#83643,#83644,#83645,#83646,#83647,
#83648,#83649,#83650,#83651,#83652,#83653,#83654,#83655,#83656,#83657,#83658,
#83659,#83660)),.UNSPECIFIED.,.F.,.T.,.F.,(4,1,4),(4,1,1,1,1,1,1,1,1,1,
1,1,1,1,1,4),(0.,0.571428571428571,1.),(-1.24903384766071,-1.07060044085204,
-0.892167034043367,-0.713733627234693,-0.53530022042602,-0.356866813617347,
-0.178433406808673,0.0594778022695577,0.118955604539115,0.178433406808673,
0.356866813617347,0.53530022042602,0.713733627234693,0.892167034043367,
1.07060044085204,1.24903384766071),.UNSPECIFIED.) ;
#1966=B_SPLINE_SURFACE_WITH_KNOTS('',3,3,((#84017,#84018,#84019,#84020),
(#84021,#84022,#84023,#84024),(#84025,#84026,#84027,#84028),(#84029,#84030,
#84031,#84032),(#84033,#84034,#84035,#84036)),.UNSPECIFIED.,.F.,.F.,.F.,
(4,1,4),(4,4),(0.,0.5,1.),(1.57079632679485,1.68822329689356),
 .UNSPECIFIED.) ;
#1967=B_SPLINE_SURFACE_WITH_KNOTS('',3,3,((#84040,#84041,#84042,#84043),
(#84044,#84045,#84046,#84047),(#84048,#84049,#84050,#84051),(#84052,#84053,
#84054,#84055),(#84056,#84057,#84058,#84059)),.UNSPECIFIED.,.F.,.F.,.F.,
(4,1,4),(4,4),(0.,0.5,1.00076388698133),(0.38994149913495,0.401496426112861),
 .UNSPECIFIED.) ;
#1968=B_SPLINE_SURFACE_WITH_KNOTS('',3,3,((#84085,#84086,#84087,#84088,
#84089),(#84090,#84091,#84092,#84093,#84094),(#84095,#84096,#84097,#84098,
#84099),(#84100,#84101,#84102,#84103,#84104),(#84105,#84106,#84107,#84108,
#84109)),.UNSPECIFIED.,.F.,.F.,.F.,(4,1,4),(4,1,4),(0.,0.5,1.),(0.,0.00867853090984697,
0.0173570618196939),.UNSPECIFIED.) ;
#1969=B_SPLINE_SURFACE_WITH_KNOTS('',3,3,((#84251,#84252,#84253,#84254),
(#84255,#84256,#84257,#84258),(#84259,#84260,#84261,#84262),(#84263,#84264,
#84265,#84266),(#84267,#84268,#84269,#84270)),.UNSPECIFIED.,.F.,.F.,.F.,
(4,1,4),(4,4),(0.,0.571428571428571,1.),(-1.11022302462516E-16,1.5707963267949),
 .UNSPECIFIED.) ;
#1970=B_SPLINE_SURFACE_WITH_KNOTS('',3,3,((#84279,#84280,#84281,#84282),
(#84283,#84284,#84285,#84286),(#84287,#84288,#84289,#84290),(#84291,#84292,
#84293,#84294),(#84295,#84296,#84297,#84298)),.UNSPECIFIED.,.F.,.F.,.F.,
(4,1,4),(4,4),(0.,0.571428571428571,1.),(-8.77933589643389E-15,1.5707963267949),
 .UNSPECIFIED.) ;
#1971=B_SPLINE_SURFACE_WITH_KNOTS('',3,3,((#84547,#84548,#84549,#84550),
(#84551,#84552,#84553,#84554),(#84555,#84556,#84557,#84558),(#84559,#84560,
#84561,#84562),(#84563,#84564,#84565,#84566)),.UNSPECIFIED.,.F.,.F.,.F.,
(4,1,4),(4,4),(0.,0.571428571428571,1.),(-6.90310534513333E-14,1.5707963267949),
 .UNSPECIFIED.) ;
#1972=B_SPLINE_SURFACE_WITH_KNOTS('',3,3,((#84575,#84576,#84577,#84578),
(#84579,#84580,#84581,#84582),(#84583,#84584,#84585,#84586),(#84587,#84588,
#84589,#84590),(#84591,#84592,#84593,#84594)),.UNSPECIFIED.,.F.,.F.,.F.,
(4,1,4),(4,4),(0.,0.571428571428571,1.),(-1.5707963267949,1.68448774068473E-13),
 .UNSPECIFIED.) ;
#1973=B_SPLINE_SURFACE_WITH_KNOTS('',3,3,((#85979,#85980,#85981,#85982,
#85983,#85984),(#85985,#85986,#85987,#85988,#85989,#85990),(#85991,#85992,
#85993,#85994,#85995,#85996),(#85997,#85998,#85999,#86000,#86001,#86002),
(#86003,#86004,#86005,#86006,#86007,#86008)),.UNSPECIFIED.,.F.,.F.,.F.,
(4,1,4),(4,1,1,4),(-0.000538086234182272,0.5,1.00053808622348),(-0.000538086234182344,
0.448798950512828,0.897597901025655,1.5707963267949),.UNSPECIFIED.) ;
#1974=B_SPLINE_SURFACE_WITH_KNOTS('',3,3,((#86013,#86014,#86015,#86016,
#86017),(#86018,#86019,#86020,#86021,#86022),(#86023,#86024,#86025,#86026,
#86027),(#86028,#86029,#86030,#86031,#86032),(#86033,#86034,#86035,#86036,
#86037)),.UNSPECIFIED.,.F.,.F.,.F.,(4,1,4),(4,1,4),(-0.00316978173158919,
0.5,1.00316978173188),(-0.00316978173188948,0.673198425769238,1.5707963267949),
 .UNSPECIFIED.) ;
#1975=B_SPLINE_SURFACE_WITH_KNOTS('',3,3,((#86046,#86047,#86048,#86049,
#86050),(#86051,#86052,#86053,#86054,#86055),(#86056,#86057,#86058,#86059,
#86060),(#86061,#86062,#86063,#86064,#86065),(#86066,#86067,#86068,#86069,
#86070)),.UNSPECIFIED.,.F.,.F.,.F.,(4,1,4),(4,1,4),(-0.00317101823526472,
0.5,1.00317101819783),(-0.00317101823526462,0.673198425769241,1.5707963267949),
 .UNSPECIFIED.) ;
#1976=B_SPLINE_SURFACE_WITH_KNOTS('',3,3,((#86079,#86080,#86081,#86082,
#86083),(#86084,#86085,#86086,#86087,#86088),(#86089,#86090,#86091,#86092,
#86093),(#86094,#86095,#86096,#86097,#86098),(#86099,#86100,#86101,#86102,
#86103)),.UNSPECIFIED.,.F.,.F.,.F.,(4,1,4),(4,1,4),(-0.00317180722397545,
0.5,1.00317180718751),(-0.00317180722396792,0.673198425769246,1.5707963267949),
 .UNSPECIFIED.) ;
#1977=B_SPLINE_SURFACE_WITH_KNOTS('',3,3,((#86113,#86114,#86115,#86116,
#86117,#86118),(#86119,#86120,#86121,#86122,#86123,#86124),(#86125,#86126,
#86127,#86128,#86129,#86130),(#86131,#86132,#86133,#86134,#86135,#86136),
(#86137,#86138,#86139,#86140,#86141,#86142)),.UNSPECIFIED.,.F.,.F.,.F.,
(4,1,4),(4,1,1,4),(0.,0.571428571428571,1.00028292742608),(-0.000282927426077196,
0.673198425769239,1.12199737628207,1.57107925422097),.UNSPECIFIED.) ;
#1978=B_SPLINE_SURFACE_WITH_KNOTS('',3,3,((#86147,#86148,#86149,#86150,
#86151),(#86152,#86153,#86154,#86155,#86156),(#86157,#86158,#86159,#86160,
#86161),(#86162,#86163,#86164,#86165,#86166),(#86167,#86168,#86169,#86170,
#86171)),.UNSPECIFIED.,.F.,.F.,.F.,(4,1,4),(4,1,4),(-0.000895493577093496,
0.571428571428571,1.00047285387642),(-1.57169182037199,-0.897597901025654,
0.000895493577097937),.UNSPECIFIED.) ;
#1979=B_SPLINE_SURFACE_WITH_KNOTS('',3,3,((#86182,#86183,#86184,#86185,
#86186,#86187),(#86188,#86189,#86190,#86191,#86192,#86193),(#86194,#86195,
#86196,#86197,#86198,#86199),(#86200,#86201,#86202,#86203,#86204,#86205),
(#86206,#86207,#86208,#86209,#86210,#86211)),.UNSPECIFIED.,.F.,.F.,.F.,
(4,1,4),(4,1,1,4),(0.,0.571428571428571,1.00028282366511),(-0.000282823665114463,
0.67319842576924,1.12199737628207,1.57107915046001),.UNSPECIFIED.) ;
#1980=B_SPLINE_SURFACE_WITH_KNOTS('',3,3,((#86216,#86217,#86218,#86219,
#86220),(#86221,#86222,#86223,#86224,#86225),(#86226,#86227,#86228,#86229,
#86230),(#86231,#86232,#86233,#86234,#86235),(#86236,#86237,#86238,#86239,
#86240)),.UNSPECIFIED.,.F.,.F.,.F.,(4,1,4),(4,1,4),(-0.00089808555193699,
0.571428571428571,1.00047258665151),(-1.57169441234684,-0.897597901025656,
0.000898085551936612),.UNSPECIFIED.) ;
#1981=B_SPLINE_SURFACE_WITH_KNOTS('',3,3,((#86321,#86322,#86323,#86324,
#86325),(#86326,#86327,#86328,#86329,#86330),(#86331,#86332,#86333,#86334,
#86335),(#86336,#86337,#86338,#86339,#86340),(#86341,#86342,#86343,#86344,
#86345)),.UNSPECIFIED.,.F.,.F.,.F.,(4,1,4),(4,1,4),(0.232659879271761,0.620020769070722,
1.),(0.173726017404586,0.773477463983206,1.5707963267949),.UNSPECIFIED.) ;
#1982=B_SPLINE_SURFACE_WITH_KNOTS('',3,3,((#86346,#86347,#86348,#86349,
#86350),(#86351,#86352,#86353,#86354,#86355),(#86356,#86357,#86358,#86359,
#86360),(#86361,#86362,#86363,#86364,#86365),(#86366,#86367,#86368,#86369,
#86370)),.UNSPECIFIED.,.F.,.F.,.F.,(4,1,4),(4,1,4),(0.229110535172741,0.622952086196121,
1.),(-1.57079632679489,-0.972068585274832,-0.173764929914751),
 .UNSPECIFIED.) ;
#1983=B_SPLINE_SURFACE_WITH_KNOTS('',3,3,((#86371,#86372,#86373,#86374,
#86375),(#86376,#86377,#86378,#86379,#86380),(#86381,#86382,#86383,#86384,
#86385),(#86386,#86387,#86388,#86389,#86390),(#86391,#86392,#86393,#86394,
#86395)),.UNSPECIFIED.,.F.,.F.,.F.,(4,1,4),(4,1,4),(0.2291096770137,0.622952086196224,
1.),(-1.57079632679489,-0.972068585273428,-0.173764929911475),
 .UNSPECIFIED.) ;
#1984=B_SPLINE_SURFACE_WITH_KNOTS('',3,3,((#86397,#86398,#86399,#86400,
#86401),(#86402,#86403,#86404,#86405,#86406),(#86407,#86408,#86409,#86410,
#86411),(#86412,#86413,#86414,#86415,#86416),(#86417,#86418,#86419,#86420,
#86421)),.UNSPECIFIED.,.F.,.F.,.F.,(4,1,4),(4,1,4),(0.232660620324116,0.620020769070722,
1.),(0.173725984876902,0.773477463983786,1.57079632679491),
 .UNSPECIFIED.) ;
#1985=B_SPLINE_SURFACE_WITH_KNOTS('',3,3,((#86423,#86424,#86425,#86426,
#86427,#86428),(#86429,#86430,#86431,#86432,#86433,#86434),(#86435,#86436,
#86437,#86438,#86439,#86440),(#86441,#86442,#86443,#86444,#86445,#86446),
(#86447,#86448,#86449,#86450,#86451,#86452)),.UNSPECIFIED.,.F.,.F.,.F.,
(4,1,4),(4,1,1,4),(-0.026021099187187,0.5,1.00149490139021),(-1.59681742598208,
-0.897597901025652,-0.448798950512825,0.0260210991871885),.UNSPECIFIED.) ;
#1986=B_SPLINE_SURFACE_WITH_KNOTS('',3,3,((#86454,#86455,#86456,#86457,
#86458),(#86459,#86460,#86461,#86462,#86463),(#86464,#86465,#86466,#86467,
#86468),(#86469,#86470,#86471,#86472,#86473),(#86474,#86475,#86476,#86477,
#86478)),.UNSPECIFIED.,.F.,.F.,.F.,(4,1,4),(4,1,4),(-0.0540331686418731,
0.5,1.00272533009723),(-0.0540331686418767,0.673198425769243,1.62482949543678),
 .UNSPECIFIED.) ;
#1987=B_SPLINE_SURFACE_WITH_KNOTS('',3,3,((#86479,#86480,#86481,#86482,
#86483,#86484),(#86485,#86486,#86487,#86488,#86489,#86490),(#86491,#86492,
#86493,#86494,#86495,#86496),(#86497,#86498,#86499,#86500,#86501,#86502),
(#86503,#86504,#86505,#86506,#86507,#86508)),.UNSPECIFIED.,.F.,.F.,.F.,
(4,1,4),(4,1,1,4),(-0.0260423511979298,0.5,1.00147848522175),(-0.0260423511979351,
0.448798950512826,0.897597901025657,1.59683867799283),.UNSPECIFIED.) ;
#1988=B_SPLINE_SURFACE_WITH_KNOTS('',3,3,((#86509,#86510,#86511,#86512,
#86513,#86514),(#86515,#86516,#86517,#86518,#86519,#86520),(#86521,#86522,
#86523,#86524,#86525,#86526),(#86527,#86528,#86529,#86530,#86531,#86532),
(#86533,#86534,#86535,#86536,#86537,#86538)),.UNSPECIFIED.,.F.,.F.,.F.,
(4,1,4),(4,1,1,4),(-0.0260371921793241,0.5,1.00148247115979),(-1.59683351897421,
-0.897597901025653,-0.448798950512826,0.0260371921793241),.UNSPECIFIED.) ;
#2176=SPHERICAL_SURFACE('',#50592,0.100000000000016) ;
#2177=SPHERICAL_SURFACE('',#50601,0.1) ;
#2178=SPHERICAL_SURFACE('',#50628,0.1) ;
#2179=SPHERICAL_SURFACE('',#50730,0.1) ;
#2180=SPHERICAL_SURFACE('',#50732,0.1) ;
#2181=SPHERICAL_SURFACE('',#50807,0.1) ;
#2182=SPHERICAL_SURFACE('',#50815,0.1) ;
#2183=SPHERICAL_SURFACE('',#50849,0.1) ;
#2184=SPHERICAL_SURFACE('',#50857,0.1) ;
#2185=SPHERICAL_SURFACE('',#50880,0.1) ;
#2186=SPHERICAL_SURFACE('',#50968,0.100000000000016) ;
#2187=SPHERICAL_SURFACE('',#50971,0.0999999999999979) ;
#2188=SPHERICAL_SURFACE('',#51016,0.0999999999999979) ;
#2189=SPHERICAL_SURFACE('',#51028,0.0999999999999979) ;
#2190=SPHERICAL_SURFACE('',#51263,0.0999999999999979) ;
#2191=SPHERICAL_SURFACE('',#51290,0.100000000000016) ;
#2277=PLANE('',#50170) ;
#2278=PLANE('',#50171) ;
#2279=PLANE('',#50172) ;
#2280=PLANE('',#50173) ;
#2281=PLANE('',#50190) ;
#2282=PLANE('',#50191) ;
#2283=PLANE('',#50192) ;
#2284=PLANE('',#50193) ;
#2285=PLANE('',#50199) ;
#2286=PLANE('',#50206) ;
#2287=PLANE('',#50207) ;
#2288=PLANE('',#50208) ;
#2289=PLANE('',#50217) ;
#2290=PLANE('',#50218) ;
#2291=PLANE('',#50219) ;
#2292=PLANE('',#50226) ;
#2293=PLANE('',#50227) ;
#2294=PLANE('',#50228) ;
#2295=PLANE('',#50245) ;
#2296=PLANE('',#50246) ;
#2297=PLANE('',#50247) ;
#2298=PLANE('',#50248) ;
#2299=PLANE('',#50249) ;
#2300=PLANE('',#50331) ;
#2301=PLANE('',#50340) ;
#2302=PLANE('',#50347) ;
#2303=PLANE('',#50348) ;
#2304=PLANE('',#50354) ;
#2305=PLANE('',#50366) ;
#2306=PLANE('',#50477) ;
#2307=PLANE('',#50481) ;
#2308=PLANE('',#50484) ;
#2309=PLANE('',#50487) ;
#2310=PLANE('',#50490) ;
#2311=PLANE('',#50493) ;
#2312=PLANE('',#50503) ;
#2313=PLANE('',#50519) ;
#2314=PLANE('',#50525) ;
#2315=PLANE('',#50534) ;
#2316=PLANE('',#50540) ;
#2317=PLANE('',#50555) ;
#2318=PLANE('',#50560) ;
#2319=PLANE('',#50633) ;
#2320=PLANE('',#50638) ;
#2321=PLANE('',#50649) ;
#2322=PLANE('',#50658) ;
#2323=PLANE('',#50678) ;
#2324=PLANE('',#50681) ;
#2325=PLANE('',#50684) ;
#2326=PLANE('',#50687) ;
#2327=PLANE('',#50690) ;
#2328=PLANE('',#50693) ;
#2329=PLANE('',#50736) ;
#2330=PLANE('',#50739) ;
#2331=PLANE('',#50742) ;
#2332=PLANE('',#50745) ;
#2333=PLANE('',#50787) ;
#2334=PLANE('',#50817) ;
#2335=PLANE('',#50820) ;
#2336=PLANE('',#50823) ;
#2337=PLANE('',#50826) ;
#2338=PLANE('',#50829) ;
#2339=PLANE('',#50859) ;
#2340=PLANE('',#50862) ;
#2341=PLANE('',#50865) ;
#2342=PLANE('',#50868) ;
#2343=PLANE('',#50871) ;
#2344=PLANE('',#50881) ;
#2345=PLANE('',#50886) ;
#2346=PLANE('',#50908) ;
#2347=PLANE('',#50911) ;
#2348=PLANE('',#50914) ;
#2349=PLANE('',#50917) ;
#2350=PLANE('',#50920) ;
#2351=PLANE('',#50926) ;
#2352=PLANE('',#50950) ;
#2353=PLANE('',#50960) ;
#2354=PLANE('',#51002) ;
#2355=PLANE('',#51012) ;
#2356=PLANE('',#51054) ;
#2357=PLANE('',#51165) ;
#2358=PLANE('',#51168) ;
#2359=PLANE('',#51173) ;
#2360=PLANE('',#51178) ;
#2361=PLANE('',#51181) ;
#2362=PLANE('',#51184) ;
#2363=PLANE('',#51187) ;
#2364=PLANE('',#51190) ;
#2365=PLANE('',#51193) ;
#2366=PLANE('',#51196) ;
#2367=PLANE('',#51199) ;
#2368=PLANE('',#51213) ;
#2369=PLANE('',#51214) ;
#2370=PLANE('',#51223) ;
#2371=PLANE('',#51261) ;
#2372=PLANE('',#51262) ;
#2373=PLANE('',#51303) ;
#2374=PLANE('',#51304) ;
#2375=PLANE('',#51313) ;
#2376=PLANE('',#51323) ;
#2377=PLANE('',#51352) ;
#2378=PLANE('',#51353) ;
#2379=PLANE('',#51362) ;
#2380=PLANE('',#51390) ;
#2381=PLANE('',#51391) ;
#2382=PLANE('',#51392) ;
#2383=PLANE('',#51393) ;
#2384=PLANE('',#51394) ;
#2385=PLANE('',#51396) ;
#2386=PLANE('',#51398) ;
#2387=PLANE('',#51443) ;
#2388=PLANE('',#51444) ;
#2389=PLANE('',#51445) ;
#2390=PLANE('',#51446) ;
#2391=PLANE('',#51464) ;
#2392=PLANE('',#51465) ;
#2393=PLANE('',#51467) ;
#2394=PLANE('',#51571) ;
#2395=PLANE('',#51594) ;
#2396=PLANE('',#51612) ;
#2397=PLANE('',#51622) ;
#2398=PLANE('',#51624) ;
#2399=PLANE('',#51626) ;
#2400=PLANE('',#51627) ;
#2401=PLANE('',#51628) ;
#2402=PLANE('',#51629) ;
#2403=PLANE('',#51630) ;
#2404=PLANE('',#51671) ;
#2405=PLANE('',#51676) ;
#2406=PLANE('',#51681) ;
#2407=PLANE('',#51684) ;
#2408=PLANE('',#51685) ;
#2409=PLANE('',#51686) ;
#2410=PLANE('',#51687) ;
#2411=PLANE('',#51688) ;
#2412=PLANE('',#51689) ;
#2413=PLANE('',#51690) ;
#2414=PLANE('',#51691) ;
#2415=PLANE('',#51692) ;
#2416=PLANE('',#51693) ;
#2417=PLANE('',#51694) ;
#2418=PLANE('',#51695) ;
#2419=PLANE('',#51696) ;
#2420=PLANE('',#51697) ;
#2421=PLANE('',#51698) ;
#2422=PLANE('',#51699) ;
#2423=PLANE('',#51700) ;
#2424=PLANE('',#51704) ;
#2425=PLANE('',#51705) ;
#2426=PLANE('',#51708) ;
#3323=LINE('',#79543,#6537) ;
#3324=LINE('',#79546,#6538) ;
#3325=LINE('',#79549,#6539) ;
#3326=LINE('',#79551,#6540) ;
#3327=LINE('',#79554,#6541) ;
#3328=LINE('',#79555,#6542) ;
#3329=LINE('',#79728,#6543) ;
#3330=LINE('',#79730,#6544) ;
#3331=LINE('',#79731,#6545) ;
#3332=LINE('',#79734,#6546) ;
#3333=LINE('',#79735,#6547) ;
#3334=LINE('',#79738,#6548) ;
#3335=LINE('',#79739,#6549) ;
#3336=LINE('',#79751,#6550) ;
#3337=LINE('',#79761,#6551) ;
#3338=LINE('',#79803,#6552) ;
#3339=LINE('',#79805,#6553) ;
#3340=LINE('',#79807,#6554) ;
#3341=LINE('',#79866,#6555) ;
#3342=LINE('',#79868,#6556) ;
#3343=LINE('',#79870,#6557) ;
#3344=LINE('',#79871,#6558) ;
#3345=LINE('',#79876,#6559) ;
#3346=LINE('',#79902,#6560) ;
#3347=LINE('',#79927,#6561) ;
#3348=LINE('',#80266,#6562) ;
#3349=LINE('',#80334,#6563) ;
#3350=LINE('',#80337,#6564) ;
#3351=LINE('',#80341,#6565) ;
#3352=LINE('',#80344,#6566) ;
#3353=LINE('',#80841,#6567) ;
#3354=LINE('',#80849,#6568) ;
#3355=LINE('',#80861,#6569) ;
#3356=LINE('',#80870,#6570) ;
#3357=LINE('',#80871,#6571) ;
#3358=LINE('',#80874,#6572) ;
#3359=LINE('',#80875,#6573) ;
#3360=LINE('',#80878,#6574) ;
#3361=LINE('',#80879,#6575) ;
#3362=LINE('',#80891,#6576) ;
#3363=LINE('',#80909,#6577) ;
#3364=LINE('',#80927,#6578) ;
#3365=LINE('',#80973,#6579) ;
#3366=LINE('',#80982,#6580) ;
#3367=LINE('',#80983,#6581) ;
#3368=LINE('',#81090,#6582) ;
#3369=LINE('',#81095,#6583) ;
#3370=LINE('',#81228,#6584) ;
#3371=LINE('',#81520,#6585) ;
#3372=LINE('',#81524,#6586) ;
#3373=LINE('',#81528,#6587) ;
#3374=LINE('',#81530,#6588) ;
#3375=LINE('',#81533,#6589) ;
#3376=LINE('',#81534,#6590) ;
#3377=LINE('',#81537,#6591) ;
#3378=LINE('',#81539,#6592) ;
#3379=LINE('',#81540,#6593) ;
#3380=LINE('',#81543,#6594) ;
#3381=LINE('',#81544,#6595) ;
#3382=LINE('',#81549,#6596) ;
#3383=LINE('',#81553,#6597) ;
#3384=LINE('',#81557,#6598) ;
#3385=LINE('',#81559,#6599) ;
#3386=LINE('',#81563,#6600) ;
#3387=LINE('',#81565,#6601) ;
#3388=LINE('',#81568,#6602) ;
#3389=LINE('',#81569,#6603) ;
#3390=LINE('',#81572,#6604) ;
#3391=LINE('',#81574,#6605) ;
#3392=LINE('',#81575,#6606) ;
#3393=LINE('',#81578,#6607) ;
#3394=LINE('',#81579,#6608) ;
#3395=LINE('',#81584,#6609) ;
#3396=LINE('',#81588,#6610) ;
#3397=LINE('',#81592,#6611) ;
#3398=LINE('',#81594,#6612) ;
#3399=LINE('',#81597,#6613) ;
#3400=LINE('',#81598,#6614) ;
#3401=LINE('',#81601,#6615) ;
#3402=LINE('',#81603,#6616) ;
#3403=LINE('',#81604,#6617) ;
#3404=LINE('',#81607,#6618) ;
#3405=LINE('',#81608,#6619) ;
#3406=LINE('',#81613,#6620) ;
#3407=LINE('',#81795,#6621) ;
#3408=LINE('',#82252,#6622) ;
#3409=LINE('',#82256,#6623) ;
#3410=LINE('',#82260,#6624) ;
#3411=LINE('',#82263,#6625) ;
#3412=LINE('',#82266,#6626) ;
#3413=LINE('',#82269,#6627) ;
#3414=LINE('',#82271,#6628) ;
#3415=LINE('',#82272,#6629) ;
#3416=LINE('',#82327,#6630) ;
#3417=LINE('',#82501,#6631) ;
#3418=LINE('',#82512,#6632) ;
#3419=LINE('',#82513,#6633) ;
#3420=LINE('',#82524,#6634) ;
#3421=LINE('',#82535,#6635) ;
#3422=LINE('',#82546,#6636) ;
#3423=LINE('',#82548,#6637) ;
#3424=LINE('',#82550,#6638) ;
#3425=LINE('',#82552,#6639) ;
#3426=LINE('',#82557,#6640) ;
#3427=LINE('',#82559,#6641) ;
#3428=LINE('',#82561,#6642) ;
#3429=LINE('',#82565,#6643) ;
#3430=LINE('',#82569,#6644) ;
#3431=LINE('',#82571,#6645) ;
#3432=LINE('',#82576,#6646) ;
#3433=LINE('',#82578,#6647) ;
#3434=LINE('',#82582,#6648) ;
#3435=LINE('',#82586,#6649) ;
#3436=LINE('',#82588,#6650) ;
#3437=LINE('',#82590,#6651) ;
#3438=LINE('',#82594,#6652) ;
#3439=LINE('',#82598,#6653) ;
#3440=LINE('',#82602,#6654) ;
#3441=LINE('',#82606,#6655) ;
#3442=LINE('',#82610,#6656) ;
#3443=LINE('',#82614,#6657) ;
#3444=LINE('',#82618,#6658) ;
#3445=LINE('',#82622,#6659) ;
#3446=LINE('',#82626,#6660) ;
#3447=LINE('',#82630,#6661) ;
#3448=LINE('',#82634,#6662) ;
#3449=LINE('',#82640,#6663) ;
#3450=LINE('',#82646,#6664) ;
#3451=LINE('',#82650,#6665) ;
#3452=LINE('',#82654,#6666) ;
#3453=LINE('',#82656,#6667) ;
#3454=LINE('',#82657,#6668) ;
#3455=LINE('',#82660,#6669) ;
#3456=LINE('',#82662,#6670) ;
#3457=LINE('',#82663,#6671) ;
#3458=LINE('',#82668,#6672) ;
#3459=LINE('',#82672,#6673) ;
#3460=LINE('',#82676,#6674) ;
#3461=LINE('',#82678,#6675) ;
#3462=LINE('',#82682,#6676) ;
#3463=LINE('',#82686,#6677) ;
#3464=LINE('',#82688,#6678) ;
#3465=LINE('',#82691,#6679) ;
#3466=LINE('',#82694,#6680) ;
#3467=LINE('',#82696,#6681) ;
#3468=LINE('',#82698,#6682) ;
#3469=LINE('',#82700,#6683) ;
#3470=LINE('',#82702,#6684) ;
#3471=LINE('',#82706,#6685) ;
#3472=LINE('',#82710,#6686) ;
#3473=LINE('',#82714,#6687) ;
#3474=LINE('',#82718,#6688) ;
#3475=LINE('',#82722,#6689) ;
#3476=LINE('',#82728,#6690) ;
#3477=LINE('',#82730,#6691) ;
#3478=LINE('',#82734,#6692) ;
#3479=LINE('',#82738,#6693) ;
#3480=LINE('',#82740,#6694) ;
#3481=LINE('',#82744,#6695) ;
#3482=LINE('',#82748,#6696) ;
#3483=LINE('',#82751,#6697) ;
#3484=LINE('',#82756,#6698) ;
#3485=LINE('',#82758,#6699) ;
#3486=LINE('',#82762,#6700) ;
#3487=LINE('',#82766,#6701) ;
#3488=LINE('',#82768,#6702) ;
#3489=LINE('',#82772,#6703) ;
#3490=LINE('',#82776,#6704) ;
#3491=LINE('',#82779,#6705) ;
#3492=LINE('',#82782,#6706) ;
#3493=LINE('',#82784,#6707) ;
#3494=LINE('',#82786,#6708) ;
#3495=LINE('',#82788,#6709) ;
#3496=LINE('',#82790,#6710) ;
#3497=LINE('',#82792,#6711) ;
#3498=LINE('',#82796,#6712) ;
#3499=LINE('',#82800,#6713) ;
#3500=LINE('',#82804,#6714) ;
#3501=LINE('',#82807,#6715) ;
#3502=LINE('',#82812,#6716) ;
#3503=LINE('',#82816,#6717) ;
#3504=LINE('',#82820,#6718) ;
#3505=LINE('',#82824,#6719) ;
#3506=LINE('',#82828,#6720) ;
#3507=LINE('',#82832,#6721) ;
#3508=LINE('',#82834,#6722) ;
#3509=LINE('',#82836,#6723) ;
#3510=LINE('',#82838,#6724) ;
#3511=LINE('',#82839,#6725) ;
#3512=LINE('',#82846,#6726) ;
#3513=LINE('',#82848,#6727) ;
#3514=LINE('',#82850,#6728) ;
#3515=LINE('',#82854,#6729) ;
#3516=LINE('',#82858,#6730) ;
#3517=LINE('',#82862,#6731) ;
#3518=LINE('',#82866,#6732) ;
#3519=LINE('',#82868,#6733) ;
#3520=LINE('',#82870,#6734) ;
#3521=LINE('',#82871,#6735) ;
#3522=LINE('',#82880,#6736) ;
#3523=LINE('',#82884,#6737) ;
#3524=LINE('',#82888,#6738) ;
#3525=LINE('',#82891,#6739) ;
#3526=LINE('',#82896,#6740) ;
#3527=LINE('',#82900,#6741) ;
#3528=LINE('',#82904,#6742) ;
#3529=LINE('',#82906,#6743) ;
#3530=LINE('',#82910,#6744) ;
#3531=LINE('',#82914,#6745) ;
#3532=LINE('',#82916,#6746) ;
#3533=LINE('',#82919,#6747) ;
#3534=LINE('',#82922,#6748) ;
#3535=LINE('',#82924,#6749) ;
#3536=LINE('',#82926,#6750) ;
#3537=LINE('',#82927,#6751) ;
#3538=LINE('',#82934,#6752) ;
#3539=LINE('',#82943,#6753) ;
#3540=LINE('',#82946,#6754) ;
#3541=LINE('',#82948,#6755) ;
#3542=LINE('',#82955,#6756) ;
#3543=LINE('',#82968,#6757) ;
#3544=LINE('',#82979,#6758) ;
#3545=LINE('',#82990,#6759) ;
#3546=LINE('',#83024,#6760) ;
#3547=LINE('',#83033,#6761) ;
#3548=LINE('',#83041,#6762) ;
#3549=LINE('',#83045,#6763) ;
#3550=LINE('',#83047,#6764) ;
#3551=LINE('',#83049,#6765) ;
#3552=LINE('',#83051,#6766) ;
#3553=LINE('',#83053,#6767) ;
#3554=LINE('',#83057,#6768) ;
#3555=LINE('',#83061,#6769) ;
#3556=LINE('',#83065,#6770) ;
#3557=LINE('',#83067,#6771) ;
#3558=LINE('',#83071,#6772) ;
#3559=LINE('',#83075,#6773) ;
#3560=LINE('',#83077,#6774) ;
#3561=LINE('',#83079,#6775) ;
#3562=LINE('',#83083,#6776) ;
#3563=LINE('',#83087,#6777) ;
#3564=LINE('',#83089,#6778) ;
#3565=LINE('',#83093,#6779) ;
#3566=LINE('',#83097,#6780) ;
#3567=LINE('',#83103,#6781) ;
#3568=LINE('',#83109,#6782) ;
#3569=LINE('',#83113,#6783) ;
#3570=LINE('',#83117,#6784) ;
#3571=LINE('',#83121,#6785) ;
#3572=LINE('',#83125,#6786) ;
#3573=LINE('',#83129,#6787) ;
#3574=LINE('',#83133,#6788) ;
#3575=LINE('',#83137,#6789) ;
#3576=LINE('',#83146,#6790) ;
#3577=LINE('',#83155,#6791) ;
#3578=LINE('',#83159,#6792) ;
#3579=LINE('',#83162,#6793) ;
#3580=LINE('',#83167,#6794) ;
#3581=LINE('',#83169,#6795) ;
#3582=LINE('',#83173,#6796) ;
#3583=LINE('',#83177,#6797) ;
#3584=LINE('',#83179,#6798) ;
#3585=LINE('',#83183,#6799) ;
#3586=LINE('',#83187,#6800) ;
#3587=LINE('',#83191,#6801) ;
#3588=LINE('',#83199,#6802) ;
#3589=LINE('',#83201,#6803) ;
#3590=LINE('',#83205,#6804) ;
#3591=LINE('',#83209,#6805) ;
#3592=LINE('',#83213,#6806) ;
#3593=LINE('',#83217,#6807) ;
#3594=LINE('',#83221,#6808) ;
#3595=LINE('',#83225,#6809) ;
#3596=LINE('',#83227,#6810) ;
#3597=LINE('',#83228,#6811) ;
#3598=LINE('',#83233,#6812) ;
#3599=LINE('',#83237,#6813) ;
#3600=LINE('',#83241,#6814) ;
#3601=LINE('',#83245,#6815) ;
#3602=LINE('',#83249,#6816) ;
#3603=LINE('',#83253,#6817) ;
#3604=LINE('',#83255,#6818) ;
#3605=LINE('',#83257,#6819) ;
#3606=LINE('',#83263,#6820) ;
#3607=LINE('',#83267,#6821) ;
#3608=LINE('',#83271,#6822) ;
#3609=LINE('',#83274,#6823) ;
#3610=LINE('',#83277,#6824) ;
#3611=LINE('',#83279,#6825) ;
#3612=LINE('',#83281,#6826) ;
#3613=LINE('',#83290,#6827) ;
#3614=LINE('',#83294,#6828) ;
#3615=LINE('',#83298,#6829) ;
#3616=LINE('',#83302,#6830) ;
#3617=LINE('',#83306,#6831) ;
#3618=LINE('',#83315,#6832) ;
#3619=LINE('',#83324,#6833) ;
#3620=LINE('',#83326,#6834) ;
#3621=LINE('',#83330,#6835) ;
#3622=LINE('',#83334,#6836) ;
#3623=LINE('',#83338,#6837) ;
#3624=LINE('',#83342,#6838) ;
#3625=LINE('',#83344,#6839) ;
#3626=LINE('',#83355,#6840) ;
#3627=LINE('',#83359,#6841) ;
#3628=LINE('',#83363,#6842) ;
#3629=LINE('',#83367,#6843) ;
#3630=LINE('',#83369,#6844) ;
#3631=LINE('',#83373,#6845) ;
#3632=LINE('',#83377,#6846) ;
#3633=LINE('',#83378,#6847) ;
#3634=LINE('',#83383,#6848) ;
#3635=LINE('',#83387,#6849) ;
#3636=LINE('',#83391,#6850) ;
#3637=LINE('',#83395,#6851) ;
#3638=LINE('',#83397,#6852) ;
#3639=LINE('',#83401,#6853) ;
#3640=LINE('',#83405,#6854) ;
#3641=LINE('',#83406,#6855) ;
#3642=LINE('',#83438,#6856) ;
#3643=LINE('',#83439,#6857) ;
#3644=LINE('',#83450,#6858) ;
#3645=LINE('',#83451,#6859) ;
#3646=LINE('',#83462,#6860) ;
#3647=LINE('',#83463,#6861) ;
#3648=LINE('',#83474,#6862) ;
#3649=LINE('',#83475,#6863) ;
#3650=LINE('',#83486,#6864) ;
#3651=LINE('',#83487,#6865) ;
#3652=LINE('',#83498,#6866) ;
#3653=LINE('',#83499,#6867) ;
#3654=LINE('',#83507,#6868) ;
#3655=LINE('',#83509,#6869) ;
#3656=LINE('',#83513,#6870) ;
#3657=LINE('',#83515,#6871) ;
#3658=LINE('',#83516,#6872) ;
#3659=LINE('',#83519,#6873) ;
#3660=LINE('',#83523,#6874) ;
#3661=LINE('',#83524,#6875) ;
#3662=LINE('',#83527,#6876) ;
#3663=LINE('',#83531,#6877) ;
#3664=LINE('',#83532,#6878) ;
#3665=LINE('',#83535,#6879) ;
#3666=LINE('',#83539,#6880) ;
#3667=LINE('',#83540,#6881) ;
#3668=LINE('',#83543,#6882) ;
#3669=LINE('',#83547,#6883) ;
#3670=LINE('',#83548,#6884) ;
#3671=LINE('',#83551,#6885) ;
#3672=LINE('',#83555,#6886) ;
#3673=LINE('',#83557,#6887) ;
#3674=LINE('',#83559,#6888) ;
#3675=LINE('',#83562,#6889) ;
#3676=LINE('',#83569,#6890) ;
#3677=LINE('',#83686,#6891) ;
#3678=LINE('',#83702,#6892) ;
#3679=LINE('',#83714,#6893) ;
#3680=LINE('',#83721,#6894) ;
#3681=LINE('',#83723,#6895) ;
#3682=LINE('',#83727,#6896) ;
#3683=LINE('',#83730,#6897) ;
#3684=LINE('',#83743,#6898) ;
#3685=LINE('',#83745,#6899) ;
#3686=LINE('',#83752,#6900) ;
#3687=LINE('',#83763,#6901) ;
#3688=LINE('',#83770,#6902) ;
#3689=LINE('',#83772,#6903) ;
#3690=LINE('',#83776,#6904) ;
#3691=LINE('',#83779,#6905) ;
#3692=LINE('',#83793,#6906) ;
#3693=LINE('',#83800,#6907) ;
#3694=LINE('',#83801,#6908) ;
#3695=LINE('',#83811,#6909) ;
#3696=LINE('',#83819,#6910) ;
#3697=LINE('',#83826,#6911) ;
#3698=LINE('',#83830,#6912) ;
#3699=LINE('',#83832,#6913) ;
#3700=LINE('',#83834,#6914) ;
#3701=LINE('',#83857,#6915) ;
#3702=LINE('',#83859,#6916) ;
#3703=LINE('',#83861,#6917) ;
#3704=LINE('',#83884,#6918) ;
#3705=LINE('',#83886,#6919) ;
#3706=LINE('',#83888,#6920) ;
#3707=LINE('',#83891,#6921) ;
#3708=LINE('',#83896,#6922) ;
#3709=LINE('',#83938,#6923) ;
#3710=LINE('',#83940,#6924) ;
#3711=LINE('',#83983,#6925) ;
#3712=LINE('',#83992,#6926) ;
#3713=LINE('',#83999,#6927) ;
#3714=LINE('',#84084,#6928) ;
#3715=LINE('',#84128,#6929) ;
#3716=LINE('',#84136,#6930) ;
#3717=LINE('',#84165,#6931) ;
#3718=LINE('',#84177,#6932) ;
#3719=LINE('',#84178,#6933) ;
#3720=LINE('',#84192,#6934) ;
#3721=LINE('',#84194,#6935) ;
#3722=LINE('',#84202,#6936) ;
#3723=LINE('',#84203,#6937) ;
#3724=LINE('',#84208,#6938) ;
#3725=LINE('',#84209,#6939) ;
#3726=LINE('',#84216,#6940) ;
#3727=LINE('',#84223,#6941) ;
#3728=LINE('',#84226,#6942) ;
#3729=LINE('',#84229,#6943) ;
#3730=LINE('',#84233,#6944) ;
#3731=LINE('',#84236,#6945) ;
#3732=LINE('',#84238,#6946) ;
#3733=LINE('',#84249,#6947) ;
#3734=LINE('',#84250,#6948) ;
#3735=LINE('',#84275,#6949) ;
#3736=LINE('',#84278,#6950) ;
#3737=LINE('',#84308,#6951) ;
#3738=LINE('',#84309,#6952) ;
#3739=LINE('',#84315,#6953) ;
#3740=LINE('',#84316,#6954) ;
#3741=LINE('',#84324,#6955) ;
#3742=LINE('',#84332,#6956) ;
#3743=LINE('',#84340,#6957) ;
#3744=LINE('',#84346,#6958) ;
#3745=LINE('',#84349,#6959) ;
#3746=LINE('',#84351,#6960) ;
#3747=LINE('',#84352,#6961) ;
#3748=LINE('',#84355,#6962) ;
#3749=LINE('',#84359,#6963) ;
#3750=LINE('',#84360,#6964) ;
#3751=LINE('',#84363,#6965) ;
#3752=LINE('',#84367,#6966) ;
#3753=LINE('',#84368,#6967) ;
#3754=LINE('',#84371,#6968) ;
#3755=LINE('',#84375,#6969) ;
#3756=LINE('',#84376,#6970) ;
#3757=LINE('',#84379,#6971) ;
#3758=LINE('',#84383,#6972) ;
#3759=LINE('',#84384,#6973) ;
#3760=LINE('',#84387,#6974) ;
#3761=LINE('',#84391,#6975) ;
#3762=LINE('',#84392,#6976) ;
#3763=LINE('',#84397,#6977) ;
#3764=LINE('',#84406,#6978) ;
#3765=LINE('',#84414,#6979) ;
#3766=LINE('',#84422,#6980) ;
#3767=LINE('',#84430,#6981) ;
#3768=LINE('',#84435,#6982) ;
#3769=LINE('',#84444,#6983) ;
#3770=LINE('',#84452,#6984) ;
#3771=LINE('',#84459,#6985) ;
#3772=LINE('',#84462,#6986) ;
#3773=LINE('',#84465,#6987) ;
#3774=LINE('',#84466,#6988) ;
#3775=LINE('',#84469,#6989) ;
#3776=LINE('',#84473,#6990) ;
#3777=LINE('',#84474,#6991) ;
#3778=LINE('',#84477,#6992) ;
#3779=LINE('',#84481,#6993) ;
#3780=LINE('',#84482,#6994) ;
#3781=LINE('',#84485,#6995) ;
#3782=LINE('',#84489,#6996) ;
#3783=LINE('',#84490,#6997) ;
#3784=LINE('',#84506,#6998) ;
#3785=LINE('',#84514,#6999) ;
#3786=LINE('',#84522,#7000) ;
#3787=LINE('',#84530,#7001) ;
#3788=LINE('',#84536,#7002) ;
#3789=LINE('',#84540,#7003) ;
#3790=LINE('',#84545,#7004) ;
#3791=LINE('',#84546,#7005) ;
#3792=LINE('',#84573,#7006) ;
#3793=LINE('',#84574,#7007) ;
#3794=LINE('',#84600,#7008) ;
#3795=LINE('',#84603,#7009) ;
#3796=LINE('',#84604,#7010) ;
#3797=LINE('',#84614,#7011) ;
#3798=LINE('',#84619,#7012) ;
#3799=LINE('',#84628,#7013) ;
#3800=LINE('',#84636,#7014) ;
#3801=LINE('',#84643,#7015) ;
#3802=LINE('',#84653,#7016) ;
#3803=LINE('',#84655,#7017) ;
#3804=LINE('',#84656,#7018) ;
#3805=LINE('',#84659,#7019) ;
#3806=LINE('',#84663,#7020) ;
#3807=LINE('',#84664,#7021) ;
#3808=LINE('',#84667,#7022) ;
#3809=LINE('',#84671,#7023) ;
#3810=LINE('',#84672,#7024) ;
#3811=LINE('',#84675,#7025) ;
#3812=LINE('',#84679,#7026) ;
#3813=LINE('',#84680,#7027) ;
#3814=LINE('',#84683,#7028) ;
#3815=LINE('',#84687,#7029) ;
#3816=LINE('',#84688,#7030) ;
#3817=LINE('',#84698,#7031) ;
#3818=LINE('',#84703,#7032) ;
#3819=LINE('',#84712,#7033) ;
#3820=LINE('',#84720,#7034) ;
#3821=LINE('',#84727,#7035) ;
#3822=LINE('',#84737,#7036) ;
#3823=LINE('',#84739,#7037) ;
#3824=LINE('',#84740,#7038) ;
#3825=LINE('',#84743,#7039) ;
#3826=LINE('',#84747,#7040) ;
#3827=LINE('',#84748,#7041) ;
#3828=LINE('',#84751,#7042) ;
#3829=LINE('',#84755,#7043) ;
#3830=LINE('',#84756,#7044) ;
#3831=LINE('',#84759,#7045) ;
#3832=LINE('',#84763,#7046) ;
#3833=LINE('',#84764,#7047) ;
#3834=LINE('',#84767,#7048) ;
#3835=LINE('',#84771,#7049) ;
#3836=LINE('',#84772,#7050) ;
#3837=LINE('',#84778,#7051) ;
#3838=LINE('',#84786,#7052) ;
#3839=LINE('',#84788,#7053) ;
#3840=LINE('',#84796,#7054) ;
#3841=LINE('',#84805,#7055) ;
#3842=LINE('',#84813,#7056) ;
#3843=LINE('',#84821,#7057) ;
#3844=LINE('',#84827,#7058) ;
#3845=LINE('',#84830,#7059) ;
#3846=LINE('',#84831,#7060) ;
#3847=LINE('',#84834,#7061) ;
#3848=LINE('',#84838,#7062) ;
#3849=LINE('',#84839,#7063) ;
#3850=LINE('',#84842,#7064) ;
#3851=LINE('',#84846,#7065) ;
#3852=LINE('',#84847,#7066) ;
#3853=LINE('',#84850,#7067) ;
#3854=LINE('',#84854,#7068) ;
#3855=LINE('',#84855,#7069) ;
#3856=LINE('',#84858,#7070) ;
#3857=LINE('',#84861,#7071) ;
#3858=LINE('',#84863,#7072) ;
#3859=LINE('',#84872,#7073) ;
#3860=LINE('',#84874,#7074) ;
#3861=LINE('',#84876,#7075) ;
#3862=LINE('',#84877,#7076) ;
#3863=LINE('',#84883,#7077) ;
#3864=LINE('',#84895,#7078) ;
#3865=LINE('',#84897,#7079) ;
#3866=LINE('',#84906,#7080) ;
#3867=LINE('',#84908,#7081) ;
#3868=LINE('',#84910,#7082) ;
#3869=LINE('',#84912,#7083) ;
#3870=LINE('',#84927,#7084) ;
#3871=LINE('',#84929,#7085) ;
#3872=LINE('',#84931,#7086) ;
#3873=LINE('',#84932,#7087) ;
#3874=LINE('',#84959,#7088) ;
#3875=LINE('',#84971,#7089) ;
#3876=LINE('',#84973,#7090) ;
#3877=LINE('',#84976,#7091) ;
#3878=LINE('',#84978,#7092) ;
#3879=LINE('',#84980,#7093) ;
#3880=LINE('',#84985,#7094) ;
#3881=LINE('',#85000,#7095) ;
#3882=LINE('',#85002,#7096) ;
#3883=LINE('',#85004,#7097) ;
#3884=LINE('',#85005,#7098) ;
#3885=LINE('',#85038,#7099) ;
#3886=LINE('',#85045,#7100) ;
#3887=LINE('',#85047,#7101) ;
#3888=LINE('',#85050,#7102) ;
#3889=LINE('',#85052,#7103) ;
#3890=LINE('',#85054,#7104) ;
#3891=LINE('',#85058,#7105) ;
#3892=LINE('',#85087,#7106) ;
#3893=LINE('',#85093,#7107) ;
#3894=LINE('',#85111,#7108) ;
#3895=LINE('',#85119,#7109) ;
#3896=LINE('',#85131,#7110) ;
#3897=LINE('',#85143,#7111) ;
#3898=LINE('',#85151,#7112) ;
#3899=LINE('',#85159,#7113) ;
#3900=LINE('',#85167,#7114) ;
#3901=LINE('',#85175,#7115) ;
#3902=LINE('',#85183,#7116) ;
#3903=LINE('',#85191,#7117) ;
#3904=LINE('',#85197,#7118) ;
#3905=LINE('',#85205,#7119) ;
#3906=LINE('',#85206,#7120) ;
#3907=LINE('',#85208,#7121) ;
#3908=LINE('',#85213,#7122) ;
#3909=LINE('',#85214,#7123) ;
#3910=LINE('',#85224,#7124) ;
#3911=LINE('',#85226,#7125) ;
#3912=LINE('',#85227,#7126) ;
#3913=LINE('',#85230,#7127) ;
#3914=LINE('',#85234,#7128) ;
#3915=LINE('',#85235,#7129) ;
#3916=LINE('',#85238,#7130) ;
#3917=LINE('',#85242,#7131) ;
#3918=LINE('',#85246,#7132) ;
#3919=LINE('',#85247,#7133) ;
#3920=LINE('',#85250,#7134) ;
#3921=LINE('',#85254,#7135) ;
#3922=LINE('',#85258,#7136) ;
#3923=LINE('',#85259,#7137) ;
#3924=LINE('',#85262,#7138) ;
#3925=LINE('',#85266,#7139) ;
#3926=LINE('',#85267,#7140) ;
#3927=LINE('',#85270,#7141) ;
#3928=LINE('',#85274,#7142) ;
#3929=LINE('',#85275,#7143) ;
#3930=LINE('',#85278,#7144) ;
#3931=LINE('',#85282,#7145) ;
#3932=LINE('',#85283,#7146) ;
#3933=LINE('',#85286,#7147) ;
#3934=LINE('',#85290,#7148) ;
#3935=LINE('',#85291,#7149) ;
#3936=LINE('',#85294,#7150) ;
#3937=LINE('',#85298,#7151) ;
#3938=LINE('',#85299,#7152) ;
#3939=LINE('',#85302,#7153) ;
#3940=LINE('',#85306,#7154) ;
#3941=LINE('',#85307,#7155) ;
#3942=LINE('',#85310,#7156) ;
#3943=LINE('',#85313,#7157) ;
#3944=LINE('',#85321,#7158) ;
#3945=LINE('',#85324,#7159) ;
#3946=LINE('',#85334,#7160) ;
#3947=LINE('',#85338,#7161) ;
#3948=LINE('',#85339,#7162) ;
#3949=LINE('',#85342,#7163) ;
#3950=LINE('',#85344,#7164) ;
#3951=LINE('',#85346,#7165) ;
#3952=LINE('',#85350,#7166) ;
#3953=LINE('',#85359,#7167) ;
#3954=LINE('',#85360,#7168) ;
#3955=LINE('',#85374,#7169) ;
#3956=LINE('',#85382,#7170) ;
#3957=LINE('',#85390,#7171) ;
#3958=LINE('',#85398,#7172) ;
#3959=LINE('',#85406,#7173) ;
#3960=LINE('',#85408,#7174) ;
#3961=LINE('',#85409,#7175) ;
#3962=LINE('',#85411,#7176) ;
#3963=LINE('',#85413,#7177) ;
#3964=LINE('',#85414,#7178) ;
#3965=LINE('',#85416,#7179) ;
#3966=LINE('',#85417,#7180) ;
#3967=LINE('',#85419,#7181) ;
#3968=LINE('',#85420,#7182) ;
#3969=LINE('',#85422,#7183) ;
#3970=LINE('',#85423,#7184) ;
#3971=LINE('',#85425,#7185) ;
#3972=LINE('',#85426,#7186) ;
#3973=LINE('',#85428,#7187) ;
#3974=LINE('',#85444,#7188) ;
#3975=LINE('',#85446,#7189) ;
#3976=LINE('',#85447,#7190) ;
#3977=LINE('',#85458,#7191) ;
#3978=LINE('',#85465,#7192) ;
#3979=LINE('',#85480,#7193) ;
#3980=LINE('',#85482,#7194) ;
#3981=LINE('',#85483,#7195) ;
#3982=LINE('',#85485,#7196) ;
#3983=LINE('',#85487,#7197) ;
#3984=LINE('',#85488,#7198) ;
#3985=LINE('',#85496,#7199) ;
#3986=LINE('',#85499,#7200) ;
#3987=LINE('',#85507,#7201) ;
#3988=LINE('',#85508,#7202) ;
#3989=LINE('',#85514,#7203) ;
#3990=LINE('',#85517,#7204) ;
#3991=LINE('',#85524,#7205) ;
#3992=LINE('',#85526,#7206) ;
#3993=LINE('',#85549,#7207) ;
#3994=LINE('',#85552,#7208) ;
#3995=LINE('',#85561,#7209) ;
#3996=LINE('',#85565,#7210) ;
#3997=LINE('',#85566,#7211) ;
#3998=LINE('',#85569,#7212) ;
#3999=LINE('',#85571,#7213) ;
#4000=LINE('',#85573,#7214) ;
#4001=LINE('',#85577,#7215) ;
#4002=LINE('',#85586,#7216) ;
#4003=LINE('',#85587,#7217) ;
#4004=LINE('',#85613,#7218) ;
#4005=LINE('',#85616,#7219) ;
#4006=LINE('',#85618,#7220) ;
#4007=LINE('',#85619,#7221) ;
#4008=LINE('',#85621,#7222) ;
#4009=LINE('',#85623,#7223) ;
#4010=LINE('',#85624,#7224) ;
#4011=LINE('',#85626,#7225) ;
#4012=LINE('',#85628,#7226) ;
#4013=LINE('',#85629,#7227) ;
#4014=LINE('',#85631,#7228) ;
#4015=LINE('',#85633,#7229) ;
#4016=LINE('',#85634,#7230) ;
#4017=LINE('',#85636,#7231) ;
#4018=LINE('',#85643,#7232) ;
#4019=LINE('',#85646,#7233) ;
#4020=LINE('',#85691,#7234) ;
#4021=LINE('',#85699,#7235) ;
#4022=LINE('',#85701,#7236) ;
#4023=LINE('',#85703,#7237) ;
#4024=LINE('',#85704,#7238) ;
#4025=LINE('',#85706,#7239) ;
#4026=LINE('',#85708,#7240) ;
#4027=LINE('',#85710,#7241) ;
#4028=LINE('',#85711,#7242) ;
#4029=LINE('',#85713,#7243) ;
#4030=LINE('',#85714,#7244) ;
#4031=LINE('',#85716,#7245) ;
#4032=LINE('',#85718,#7246) ;
#4033=LINE('',#85720,#7247) ;
#4034=LINE('',#85722,#7248) ;
#4035=LINE('',#85723,#7249) ;
#4036=LINE('',#85734,#7250) ;
#4037=LINE('',#85745,#7251) ;
#4038=LINE('',#85748,#7252) ;
#4039=LINE('',#85757,#7253) ;
#4040=LINE('',#85758,#7254) ;
#4041=LINE('',#85761,#7255) ;
#4042=LINE('',#85765,#7256) ;
#4043=LINE('',#85766,#7257) ;
#4044=LINE('',#85769,#7258) ;
#4045=LINE('',#85770,#7259) ;
#4046=LINE('',#85774,#7260) ;
#4047=LINE('',#85806,#7261) ;
#4048=LINE('',#85814,#7262) ;
#4049=LINE('',#85822,#7263) ;
#4050=LINE('',#85879,#7264) ;
#4051=LINE('',#85885,#7265) ;
#4052=LINE('',#85902,#7266) ;
#4053=LINE('',#85919,#7267) ;
#4054=LINE('',#85937,#7268) ;
#4055=LINE('',#85948,#7269) ;
#4056=LINE('',#85969,#7270) ;
#4057=LINE('',#85970,#7271) ;
#4058=LINE('',#85972,#7272) ;
#4059=LINE('',#86111,#7273) ;
#4060=LINE('',#86176,#7274) ;
#4061=LINE('',#86180,#7275) ;
#4062=LINE('',#86245,#7276) ;
#4063=LINE('',#86250,#7277) ;
#4064=LINE('',#86253,#7278) ;
#4065=LINE('',#86256,#7279) ;
#4066=LINE('',#86261,#7280) ;
#4067=LINE('',#86264,#7281) ;
#4068=LINE('',#86269,#7282) ;
#4069=LINE('',#86272,#7283) ;
#4070=LINE('',#86277,#7284) ;
#4071=LINE('',#86278,#7285) ;
#4072=LINE('',#86280,#7286) ;
#4073=LINE('',#86283,#7287) ;
#4074=LINE('',#86284,#7288) ;
#4075=LINE('',#86288,#7289) ;
#4076=LINE('',#86289,#7290) ;
#4077=LINE('',#86293,#7291) ;
#4078=LINE('',#86313,#7292) ;
#4079=LINE('',#86315,#7293) ;
#4080=LINE('',#86540,#7294) ;
#6537=VECTOR('',#57100,10.) ;
#6538=VECTOR('',#57103,10.) ;
#6539=VECTOR('',#57106,10.) ;
#6540=VECTOR('',#57107,10.) ;
#6541=VECTOR('',#57112,10.) ;
#6542=VECTOR('',#57113,10.) ;
#6543=VECTOR('',#57116,10.) ;
#6544=VECTOR('',#57117,10.) ;
#6545=VECTOR('',#57118,10.) ;
#6546=VECTOR('',#57121,10.) ;
#6547=VECTOR('',#57122,10.) ;
#6548=VECTOR('',#57125,10.) ;
#6549=VECTOR('',#57126,10.) ;
#6550=VECTOR('',#57127,10.) ;
#6551=VECTOR('',#57130,10.) ;
#6552=VECTOR('',#57131,10.) ;
#6553=VECTOR('',#57132,10.) ;
#6554=VECTOR('',#57133,10.) ;
#6555=VECTOR('',#57134,10.) ;
#6556=VECTOR('',#57135,10.) ;
#6557=VECTOR('',#57136,10.) ;
#6558=VECTOR('',#57137,10.) ;
#6559=VECTOR('',#57142,10.) ;
#6560=VECTOR('',#57147,10.) ;
#6561=VECTOR('',#57150,10.) ;
#6562=VECTOR('',#57155,10.) ;
#6563=VECTOR('',#57164,10.) ;
#6564=VECTOR('',#57167,10.) ;
#6565=VECTOR('',#57172,10.) ;
#6566=VECTOR('',#57177,10.) ;
#6567=VECTOR('',#57178,10.) ;
#6568=VECTOR('',#57179,10.) ;
#6569=VECTOR('',#57180,10.) ;
#6570=VECTOR('',#57183,10.) ;
#6571=VECTOR('',#57184,10.) ;
#6572=VECTOR('',#57187,10.) ;
#6573=VECTOR('',#57188,10.) ;
#6574=VECTOR('',#57191,10.) ;
#6575=VECTOR('',#57192,10.) ;
#6576=VECTOR('',#57193,10.) ;
#6577=VECTOR('',#57194,10.) ;
#6578=VECTOR('',#57195,10.) ;
#6579=VECTOR('',#57196,10.) ;
#6580=VECTOR('',#57199,10.) ;
#6581=VECTOR('',#57200,10.) ;
#6582=VECTOR('',#57203,10.) ;
#6583=VECTOR('',#57208,10.) ;
#6584=VECTOR('',#57213,10.) ;
#6585=VECTOR('',#57218,10.) ;
#6586=VECTOR('',#57221,10.) ;
#6587=VECTOR('',#57226,10.) ;
#6588=VECTOR('',#57227,10.) ;
#6589=VECTOR('',#57232,10.) ;
#6590=VECTOR('',#57233,10.) ;
#6591=VECTOR('',#57236,10.) ;
#6592=VECTOR('',#57237,10.) ;
#6593=VECTOR('',#57238,10.) ;
#6594=VECTOR('',#57241,10.) ;
#6595=VECTOR('',#57242,10.) ;
#6596=VECTOR('',#57247,10.) ;
#6597=VECTOR('',#57250,10.) ;
#6598=VECTOR('',#57255,10.) ;
#6599=VECTOR('',#57256,10.) ;
#6600=VECTOR('',#57261,10.) ;
#6601=VECTOR('',#57262,10.) ;
#6602=VECTOR('',#57267,10.) ;
#6603=VECTOR('',#57268,10.) ;
#6604=VECTOR('',#57271,10.) ;
#6605=VECTOR('',#57272,10.) ;
#6606=VECTOR('',#57273,10.) ;
#6607=VECTOR('',#57276,10.) ;
#6608=VECTOR('',#57277,10.) ;
#6609=VECTOR('',#57282,10.) ;
#6610=VECTOR('',#57285,10.) ;
#6611=VECTOR('',#57290,10.) ;
#6612=VECTOR('',#57291,10.) ;
#6613=VECTOR('',#57296,10.) ;
#6614=VECTOR('',#57297,10.) ;
#6615=VECTOR('',#57300,10.) ;
#6616=VECTOR('',#57301,10.) ;
#6617=VECTOR('',#57302,10.) ;
#6618=VECTOR('',#57305,10.) ;
#6619=VECTOR('',#57306,10.) ;
#6620=VECTOR('',#57311,10.) ;
#6621=VECTOR('',#57318,10.) ;
#6622=VECTOR('',#57323,10.) ;
#6623=VECTOR('',#57326,10.) ;
#6624=VECTOR('',#57331,10.) ;
#6625=VECTOR('',#57334,10.) ;
#6626=VECTOR('',#57337,10.) ;
#6627=VECTOR('',#57340,10.) ;
#6628=VECTOR('',#57343,10.) ;
#6629=VECTOR('',#57344,10.) ;
#6630=VECTOR('',#57349,10.) ;
#6631=VECTOR('',#57352,10.) ;
#6632=VECTOR('',#57353,10.) ;
#6633=VECTOR('',#57354,10.) ;
#6634=VECTOR('',#57355,10.) ;
#6635=VECTOR('',#57356,10.) ;
#6636=VECTOR('',#57357,10.) ;
#6637=VECTOR('',#57360,10.) ;
#6638=VECTOR('',#57363,10.) ;
#6639=VECTOR('',#57366,10.) ;
#6640=VECTOR('',#57371,10.) ;
#6641=VECTOR('',#57372,10.) ;
#6642=VECTOR('',#57373,10.) ;
#6643=VECTOR('',#57376,10.) ;
#6644=VECTOR('',#57379,10.) ;
#6645=VECTOR('',#57380,10.) ;
#6646=VECTOR('',#57385,10.) ;
#6647=VECTOR('',#57386,10.) ;
#6648=VECTOR('',#57389,10.) ;
#6649=VECTOR('',#57392,10.) ;
#6650=VECTOR('',#57393,10.) ;
#6651=VECTOR('',#57394,10.) ;
#6652=VECTOR('',#57397,10.) ;
#6653=VECTOR('',#57400,10.) ;
#6654=VECTOR('',#57403,10.) ;
#6655=VECTOR('',#57406,10.) ;
#6656=VECTOR('',#57409,10.) ;
#6657=VECTOR('',#57412,10.) ;
#6658=VECTOR('',#57415,10.) ;
#6659=VECTOR('',#57418,10.) ;
#6660=VECTOR('',#57421,10.) ;
#6661=VECTOR('',#57424,10.) ;
#6662=VECTOR('',#57427,10.) ;
#6663=VECTOR('',#57432,10.) ;
#6664=VECTOR('',#57437,10.) ;
#6665=VECTOR('',#57440,10.) ;
#6666=VECTOR('',#57443,10.) ;
#6667=VECTOR('',#57444,10.) ;
#6668=VECTOR('',#57445,10.) ;
#6669=VECTOR('',#57446,10.) ;
#6670=VECTOR('',#57447,10.) ;
#6671=VECTOR('',#57448,10.) ;
#6672=VECTOR('',#57451,10.) ;
#6673=VECTOR('',#57454,10.) ;
#6674=VECTOR('',#57457,10.) ;
#6675=VECTOR('',#57458,10.) ;
#6676=VECTOR('',#57461,10.) ;
#6677=VECTOR('',#57464,10.) ;
#6678=VECTOR('',#57465,10.) ;
#6679=VECTOR('',#57468,10.) ;
#6680=VECTOR('',#57469,10.) ;
#6681=VECTOR('',#57470,10.) ;
#6682=VECTOR('',#57471,10.) ;
#6683=VECTOR('',#57472,10.) ;
#6684=VECTOR('',#57473,10.) ;
#6685=VECTOR('',#57476,10.) ;
#6686=VECTOR('',#57479,10.) ;
#6687=VECTOR('',#57482,10.) ;
#6688=VECTOR('',#57485,10.) ;
#6689=VECTOR('',#57488,10.) ;
#6690=VECTOR('',#57493,10.) ;
#6691=VECTOR('',#57494,10.) ;
#6692=VECTOR('',#57497,10.) ;
#6693=VECTOR('',#57500,10.) ;
#6694=VECTOR('',#57501,10.) ;
#6695=VECTOR('',#57504,10.) ;
#6696=VECTOR('',#57507,10.) ;
#6697=VECTOR('',#57510,10.) ;
#6698=VECTOR('',#57513,10.) ;
#6699=VECTOR('',#57514,10.) ;
#6700=VECTOR('',#57517,10.) ;
#6701=VECTOR('',#57520,10.) ;
#6702=VECTOR('',#57521,10.) ;
#6703=VECTOR('',#57524,10.) ;
#6704=VECTOR('',#57527,10.) ;
#6705=VECTOR('',#57530,10.) ;
#6706=VECTOR('',#57531,10.) ;
#6707=VECTOR('',#57532,10.) ;
#6708=VECTOR('',#57533,10.) ;
#6709=VECTOR('',#57534,10.) ;
#6710=VECTOR('',#57535,10.) ;
#6711=VECTOR('',#57536,10.) ;
#6712=VECTOR('',#57539,10.) ;
#6713=VECTOR('',#57542,10.) ;
#6714=VECTOR('',#57545,10.) ;
#6715=VECTOR('',#57548,10.) ;
#6716=VECTOR('',#57551,10.) ;
#6717=VECTOR('',#57554,10.) ;
#6718=VECTOR('',#57557,10.) ;
#6719=VECTOR('',#57560,10.) ;
#6720=VECTOR('',#57563,10.) ;
#6721=VECTOR('',#57566,10.) ;
#6722=VECTOR('',#57567,10.) ;
#6723=VECTOR('',#57568,10.) ;
#6724=VECTOR('',#57569,10.) ;
#6725=VECTOR('',#57570,10.) ;
#6726=VECTOR('',#57575,10.) ;
#6727=VECTOR('',#57576,10.) ;
#6728=VECTOR('',#57577,10.) ;
#6729=VECTOR('',#57580,10.) ;
#6730=VECTOR('',#57583,10.) ;
#6731=VECTOR('',#57586,10.) ;
#6732=VECTOR('',#57589,10.) ;
#6733=VECTOR('',#57590,10.) ;
#6734=VECTOR('',#57591,10.) ;
#6735=VECTOR('',#57592,10.) ;
#6736=VECTOR('',#57599,10.) ;
#6737=VECTOR('',#57602,10.) ;
#6738=VECTOR('',#57605,10.) ;
#6739=VECTOR('',#57608,10.) ;
#6740=VECTOR('',#57611,10.) ;
#6741=VECTOR('',#57614,10.) ;
#6742=VECTOR('',#57617,10.) ;
#6743=VECTOR('',#57618,10.) ;
#6744=VECTOR('',#57621,10.) ;
#6745=VECTOR('',#57624,10.) ;
#6746=VECTOR('',#57625,10.) ;
#6747=VECTOR('',#57628,10.) ;
#6748=VECTOR('',#57629,10.) ;
#6749=VECTOR('',#57630,10.) ;
#6750=VECTOR('',#57631,10.) ;
#6751=VECTOR('',#57632,10.) ;
#6752=VECTOR('',#57645,10.) ;
#6753=VECTOR('',#57660,10.) ;
#6754=VECTOR('',#57665,10.) ;
#6755=VECTOR('',#57668,10.) ;
#6756=VECTOR('',#57681,10.) ;
#6757=VECTOR('',#57686,10.) ;
#6758=VECTOR('',#57687,10.) ;
#6759=VECTOR('',#57688,10.) ;
#6760=VECTOR('',#57705,2.) ;
#6761=VECTOR('',#57718,2.99999999999999) ;
#6762=VECTOR('',#57727,10.) ;
#6763=VECTOR('',#57730,10.) ;
#6764=VECTOR('',#57731,10.) ;
#6765=VECTOR('',#57732,10.) ;
#6766=VECTOR('',#57733,10.) ;
#6767=VECTOR('',#57734,10.) ;
#6768=VECTOR('',#57737,10.) ;
#6769=VECTOR('',#57740,10.) ;
#6770=VECTOR('',#57743,10.) ;
#6771=VECTOR('',#57744,10.) ;
#6772=VECTOR('',#57747,10.) ;
#6773=VECTOR('',#57750,10.) ;
#6774=VECTOR('',#57751,10.) ;
#6775=VECTOR('',#57752,10.) ;
#6776=VECTOR('',#57755,10.) ;
#6777=VECTOR('',#57758,10.) ;
#6778=VECTOR('',#57759,10.) ;
#6779=VECTOR('',#57762,10.) ;
#6780=VECTOR('',#57765,10.) ;
#6781=VECTOR('',#57770,10.) ;
#6782=VECTOR('',#57775,10.) ;
#6783=VECTOR('',#57778,10.) ;
#6784=VECTOR('',#57781,10.) ;
#6785=VECTOR('',#57784,10.) ;
#6786=VECTOR('',#57787,10.) ;
#6787=VECTOR('',#57790,10.) ;
#6788=VECTOR('',#57793,10.) ;
#6789=VECTOR('',#57796,10.) ;
#6790=VECTOR('',#57797,10.) ;
#6791=VECTOR('',#57798,10.) ;
#6792=VECTOR('',#57801,10.) ;
#6793=VECTOR('',#57804,10.) ;
#6794=VECTOR('',#57807,10.) ;
#6795=VECTOR('',#57808,10.) ;
#6796=VECTOR('',#57811,10.) ;
#6797=VECTOR('',#57814,10.) ;
#6798=VECTOR('',#57815,10.) ;
#6799=VECTOR('',#57818,10.) ;
#6800=VECTOR('',#57821,10.) ;
#6801=VECTOR('',#57824,10.) ;
#6802=VECTOR('',#57831,10.) ;
#6803=VECTOR('',#57832,10.) ;
#6804=VECTOR('',#57835,10.) ;
#6805=VECTOR('',#57838,10.) ;
#6806=VECTOR('',#57841,10.) ;
#6807=VECTOR('',#57844,10.) ;
#6808=VECTOR('',#57847,10.) ;
#6809=VECTOR('',#57850,10.) ;
#6810=VECTOR('',#57851,10.) ;
#6811=VECTOR('',#57852,10.) ;
#6812=VECTOR('',#57855,10.) ;
#6813=VECTOR('',#57858,10.) ;
#6814=VECTOR('',#57861,10.) ;
#6815=VECTOR('',#57864,10.) ;
#6816=VECTOR('',#57867,10.) ;
#6817=VECTOR('',#57870,10.) ;
#6818=VECTOR('',#57871,10.) ;
#6819=VECTOR('',#57872,10.) ;
#6820=VECTOR('',#57877,10.) ;
#6821=VECTOR('',#57880,10.) ;
#6822=VECTOR('',#57883,10.) ;
#6823=VECTOR('',#57886,10.) ;
#6824=VECTOR('',#57887,10.) ;
#6825=VECTOR('',#57888,10.) ;
#6826=VECTOR('',#57889,10.) ;
#6827=VECTOR('',#57890,10.) ;
#6828=VECTOR('',#57893,10.) ;
#6829=VECTOR('',#57896,10.) ;
#6830=VECTOR('',#57899,10.) ;
#6831=VECTOR('',#57902,10.) ;
#6832=VECTOR('',#57903,10.) ;
#6833=VECTOR('',#57904,10.) ;
#6834=VECTOR('',#57905,10.) ;
#6835=VECTOR('',#57908,10.) ;
#6836=VECTOR('',#57911,10.) ;
#6837=VECTOR('',#57914,10.) ;
#6838=VECTOR('',#57917,10.) ;
#6839=VECTOR('',#57918,10.) ;
#6840=VECTOR('',#57921,10.) ;
#6841=VECTOR('',#57924,10.) ;
#6842=VECTOR('',#57927,10.) ;
#6843=VECTOR('',#57930,10.) ;
#6844=VECTOR('',#57931,10.) ;
#6845=VECTOR('',#57934,10.) ;
#6846=VECTOR('',#57937,10.) ;
#6847=VECTOR('',#57938,10.) ;
#6848=VECTOR('',#57941,10.) ;
#6849=VECTOR('',#57944,10.) ;
#6850=VECTOR('',#57947,10.) ;
#6851=VECTOR('',#57950,10.) ;
#6852=VECTOR('',#57951,10.) ;
#6853=VECTOR('',#57954,10.) ;
#6854=VECTOR('',#57957,10.) ;
#6855=VECTOR('',#57958,10.) ;
#6856=VECTOR('',#57973,10.) ;
#6857=VECTOR('',#57974,10.) ;
#6858=VECTOR('',#57987,10.) ;
#6859=VECTOR('',#57988,10.) ;
#6860=VECTOR('',#58001,10.) ;
#6861=VECTOR('',#58002,10.) ;
#6862=VECTOR('',#58015,10.) ;
#6863=VECTOR('',#58016,10.) ;
#6864=VECTOR('',#58029,10.) ;
#6865=VECTOR('',#58030,10.) ;
#6866=VECTOR('',#58043,10.) ;
#6867=VECTOR('',#58044,10.) ;
#6868=VECTOR('',#58055,10.) ;
#6869=VECTOR('',#58056,10.) ;
#6870=VECTOR('',#58059,10.) ;
#6871=VECTOR('',#58060,10.) ;
#6872=VECTOR('',#58061,10.) ;
#6873=VECTOR('',#58064,10.) ;
#6874=VECTOR('',#58069,10.) ;
#6875=VECTOR('',#58070,10.) ;
#6876=VECTOR('',#58073,10.) ;
#6877=VECTOR('',#58078,10.) ;
#6878=VECTOR('',#58079,10.) ;
#6879=VECTOR('',#58082,10.) ;
#6880=VECTOR('',#58087,10.) ;
#6881=VECTOR('',#58088,10.) ;
#6882=VECTOR('',#58091,10.) ;
#6883=VECTOR('',#58096,10.) ;
#6884=VECTOR('',#58097,10.) ;
#6885=VECTOR('',#58100,10.) ;
#6886=VECTOR('',#58105,10.) ;
#6887=VECTOR('',#58106,10.) ;
#6888=VECTOR('',#58107,10.) ;
#6889=VECTOR('',#58110,10.) ;
#6890=VECTOR('',#58119,3.) ;
#6891=VECTOR('',#58122,10.) ;
#6892=VECTOR('',#58143,2.) ;
#6893=VECTOR('',#58158,1.85) ;
#6894=VECTOR('',#58165,10.) ;
#6895=VECTOR('',#58166,10.) ;
#6896=VECTOR('',#58169,10.) ;
#6897=VECTOR('',#58172,10.) ;
#6898=VECTOR('',#58181,10.) ;
#6899=VECTOR('',#58182,10.) ;
#6900=VECTOR('',#58183,10.) ;
#6901=VECTOR('',#58196,1.85) ;
#6902=VECTOR('',#58203,10.) ;
#6903=VECTOR('',#58204,10.) ;
#6904=VECTOR('',#58207,10.) ;
#6905=VECTOR('',#58210,10.) ;
#6906=VECTOR('',#58219,10.) ;
#6907=VECTOR('',#58220,10.) ;
#6908=VECTOR('',#58221,10.) ;
#6909=VECTOR('',#58234,10.) ;
#6910=VECTOR('',#58245,10.) ;
#6911=VECTOR('',#58254,10.) ;
#6912=VECTOR('',#58257,10.) ;
#6913=VECTOR('',#58258,10.) ;
#6914=VECTOR('',#58259,10.) ;
#6915=VECTOR('',#58260,10.) ;
#6916=VECTOR('',#58261,10.) ;
#6917=VECTOR('',#58262,10.) ;
#6918=VECTOR('',#58263,10.) ;
#6919=VECTOR('',#58264,10.) ;
#6920=VECTOR('',#58265,10.) ;
#6921=VECTOR('',#58268,10.) ;
#6922=VECTOR('',#58275,10.) ;
#6923=VECTOR('',#58280,10.) ;
#6924=VECTOR('',#58281,10.) ;
#6925=VECTOR('',#58286,10.) ;
#6926=VECTOR('',#58289,10.) ;
#6927=VECTOR('',#58290,10.) ;
#6928=VECTOR('',#58309,10.) ;
#6929=VECTOR('',#58330,10.) ;
#6930=VECTOR('',#58341,10.) ;
#6931=VECTOR('',#58358,10.) ;
#6932=VECTOR('',#58375,10.) ;
#6933=VECTOR('',#58376,10.) ;
#6934=VECTOR('',#58395,10.) ;
#6935=VECTOR('',#58398,10.) ;
#6936=VECTOR('',#58409,10.) ;
#6937=VECTOR('',#58410,10.) ;
#6938=VECTOR('',#58415,10.) ;
#6939=VECTOR('',#58416,10.) ;
#6940=VECTOR('',#58427,10.) ;
#6941=VECTOR('',#58436,10.) ;
#6942=VECTOR('',#58441,10.) ;
#6943=VECTOR('',#58444,10.) ;
#6944=VECTOR('',#58449,10.) ;
#6945=VECTOR('',#58452,10.) ;
#6946=VECTOR('',#58455,10.) ;
#6947=VECTOR('',#58468,10.) ;
#6948=VECTOR('',#58469,10.) ;
#6949=VECTOR('',#58476,10.) ;
#6950=VECTOR('',#58481,10.) ;
#6951=VECTOR('',#58492,10.) ;
#6952=VECTOR('',#58493,10.) ;
#6953=VECTOR('',#58502,10.) ;
#6954=VECTOR('',#58503,10.) ;
#6955=VECTOR('',#58514,10.) ;
#6956=VECTOR('',#58525,10.) ;
#6957=VECTOR('',#58536,10.) ;
#6958=VECTOR('',#58545,10.) ;
#6959=VECTOR('',#58548,10.) ;
#6960=VECTOR('',#58549,10.) ;
#6961=VECTOR('',#58550,10.) ;
#6962=VECTOR('',#58553,10.) ;
#6963=VECTOR('',#58558,10.) ;
#6964=VECTOR('',#58559,10.) ;
#6965=VECTOR('',#58562,10.) ;
#6966=VECTOR('',#58567,10.) ;
#6967=VECTOR('',#58568,10.) ;
#6968=VECTOR('',#58571,10.) ;
#6969=VECTOR('',#58576,10.) ;
#6970=VECTOR('',#58577,10.) ;
#6971=VECTOR('',#58580,10.) ;
#6972=VECTOR('',#58585,10.) ;
#6973=VECTOR('',#58586,10.) ;
#6974=VECTOR('',#58589,10.) ;
#6975=VECTOR('',#58594,10.) ;
#6976=VECTOR('',#58595,10.) ;
#6977=VECTOR('',#58600,10.) ;
#6978=VECTOR('',#58613,10.) ;
#6979=VECTOR('',#58624,10.) ;
#6980=VECTOR('',#58635,10.) ;
#6981=VECTOR('',#58646,10.) ;
#6982=VECTOR('',#58651,10.) ;
#6983=VECTOR('',#58664,10.) ;
#6984=VECTOR('',#58675,10.) ;
#6985=VECTOR('',#58686,10.) ;
#6986=VECTOR('',#58689,10.) ;
#6987=VECTOR('',#58692,10.) ;
#6988=VECTOR('',#58693,10.) ;
#6989=VECTOR('',#58696,10.) ;
#6990=VECTOR('',#58701,10.) ;
#6991=VECTOR('',#58702,10.) ;
#6992=VECTOR('',#58705,10.) ;
#6993=VECTOR('',#58710,10.) ;
#6994=VECTOR('',#58711,10.) ;
#6995=VECTOR('',#58714,10.) ;
#6996=VECTOR('',#58719,10.) ;
#6997=VECTOR('',#58720,10.) ;
#6998=VECTOR('',#58741,10.) ;
#6999=VECTOR('',#58752,10.) ;
#7000=VECTOR('',#58763,10.) ;
#7001=VECTOR('',#58774,10.) ;
#7002=VECTOR('',#58783,10.) ;
#7003=VECTOR('',#58788,10.) ;
#7004=VECTOR('',#58793,10.) ;
#7005=VECTOR('',#58794,10.) ;
#7006=VECTOR('',#58803,10.) ;
#7007=VECTOR('',#58804,10.) ;
#7008=VECTOR('',#58813,10.) ;
#7009=VECTOR('',#58816,10.) ;
#7010=VECTOR('',#58817,10.) ;
#7011=VECTOR('',#58830,10.) ;
#7012=VECTOR('',#58835,10.) ;
#7013=VECTOR('',#58848,10.) ;
#7014=VECTOR('',#58859,10.) ;
#7015=VECTOR('',#58868,10.) ;
#7016=VECTOR('',#58883,10.) ;
#7017=VECTOR('',#58884,10.) ;
#7018=VECTOR('',#58885,10.) ;
#7019=VECTOR('',#58888,10.) ;
#7020=VECTOR('',#58893,10.) ;
#7021=VECTOR('',#58894,10.) ;
#7022=VECTOR('',#58897,10.) ;
#7023=VECTOR('',#58902,10.) ;
#7024=VECTOR('',#58903,10.) ;
#7025=VECTOR('',#58906,10.) ;
#7026=VECTOR('',#58911,10.) ;
#7027=VECTOR('',#58912,10.) ;
#7028=VECTOR('',#58915,10.) ;
#7029=VECTOR('',#58920,10.) ;
#7030=VECTOR('',#58921,10.) ;
#7031=VECTOR('',#58934,10.) ;
#7032=VECTOR('',#58939,10.) ;
#7033=VECTOR('',#58952,10.) ;
#7034=VECTOR('',#58963,10.) ;
#7035=VECTOR('',#58972,10.) ;
#7036=VECTOR('',#58987,10.) ;
#7037=VECTOR('',#58988,10.) ;
#7038=VECTOR('',#58989,10.) ;
#7039=VECTOR('',#58992,10.) ;
#7040=VECTOR('',#58997,10.) ;
#7041=VECTOR('',#58998,10.) ;
#7042=VECTOR('',#59001,10.) ;
#7043=VECTOR('',#59006,10.) ;
#7044=VECTOR('',#59007,10.) ;
#7045=VECTOR('',#59010,10.) ;
#7046=VECTOR('',#59015,10.) ;
#7047=VECTOR('',#59016,10.) ;
#7048=VECTOR('',#59019,10.) ;
#7049=VECTOR('',#59024,10.) ;
#7050=VECTOR('',#59025,10.) ;
#7051=VECTOR('',#59034,10.) ;
#7052=VECTOR('',#59047,10.) ;
#7053=VECTOR('',#59050,10.) ;
#7054=VECTOR('',#59061,10.) ;
#7055=VECTOR('',#59074,10.) ;
#7056=VECTOR('',#59085,10.) ;
#7057=VECTOR('',#59096,10.) ;
#7058=VECTOR('',#59105,10.) ;
#7059=VECTOR('',#59108,10.) ;
#7060=VECTOR('',#59109,10.) ;
#7061=VECTOR('',#59112,10.) ;
#7062=VECTOR('',#59117,10.) ;
#7063=VECTOR('',#59118,10.) ;
#7064=VECTOR('',#59121,10.) ;
#7065=VECTOR('',#59126,10.) ;
#7066=VECTOR('',#59127,10.) ;
#7067=VECTOR('',#59130,10.) ;
#7068=VECTOR('',#59135,10.) ;
#7069=VECTOR('',#59136,10.) ;
#7070=VECTOR('',#59139,10.) ;
#7071=VECTOR('',#59144,10.) ;
#7072=VECTOR('',#59147,10.) ;
#7073=VECTOR('',#59158,10.) ;
#7074=VECTOR('',#59159,10.) ;
#7075=VECTOR('',#59160,10.) ;
#7076=VECTOR('',#59161,10.) ;
#7077=VECTOR('',#59170,10.) ;
#7078=VECTOR('',#59189,10.) ;
#7079=VECTOR('',#59192,10.) ;
#7080=VECTOR('',#59207,10.) ;
#7081=VECTOR('',#59210,10.) ;
#7082=VECTOR('',#59213,10.) ;
#7083=VECTOR('',#59216,10.) ;
#7084=VECTOR('',#59237,10.) ;
#7085=VECTOR('',#59238,10.) ;
#7086=VECTOR('',#59239,10.) ;
#7087=VECTOR('',#59240,10.) ;
#7088=VECTOR('',#59289,10.) ;
#7089=VECTOR('',#59308,10.) ;
#7090=VECTOR('',#59311,10.) ;
#7091=VECTOR('',#59316,10.) ;
#7092=VECTOR('',#59319,10.) ;
#7093=VECTOR('',#59322,10.) ;
#7094=VECTOR('',#59331,10.) ;
#7095=VECTOR('',#59352,10.) ;
#7096=VECTOR('',#59353,10.) ;
#7097=VECTOR('',#59354,10.) ;
#7098=VECTOR('',#59355,10.) ;
#7099=VECTOR('',#59414,10.) ;
#7100=VECTOR('',#59425,10.) ;
#7101=VECTOR('',#59428,10.) ;
#7102=VECTOR('',#59433,10.) ;
#7103=VECTOR('',#59436,10.) ;
#7104=VECTOR('',#59439,10.) ;
#7105=VECTOR('',#59446,10.) ;
#7106=VECTOR('',#59491,10.) ;
#7107=VECTOR('',#59500,10.) ;
#7108=VECTOR('',#59531,10.) ;
#7109=VECTOR('',#59542,10.) ;
#7110=VECTOR('',#59559,10.) ;
#7111=VECTOR('',#59576,10.) ;
#7112=VECTOR('',#59587,10.) ;
#7113=VECTOR('',#59598,10.) ;
#7114=VECTOR('',#59609,10.) ;
#7115=VECTOR('',#59620,10.) ;
#7116=VECTOR('',#59631,10.) ;
#7117=VECTOR('',#59642,10.) ;
#7118=VECTOR('',#59651,10.) ;
#7119=VECTOR('',#59662,10.) ;
#7120=VECTOR('',#59663,10.) ;
#7121=VECTOR('',#59666,10.) ;
#7122=VECTOR('',#59671,10.) ;
#7123=VECTOR('',#59672,10.) ;
#7124=VECTOR('',#59687,10.) ;
#7125=VECTOR('',#59688,10.) ;
#7126=VECTOR('',#59689,10.) ;
#7127=VECTOR('',#59692,10.) ;
#7128=VECTOR('',#59697,0.600000000000005) ;
#7129=VECTOR('',#59698,10.) ;
#7130=VECTOR('',#59701,0.600000000000005) ;
#7131=VECTOR('',#59706,10.) ;
#7132=VECTOR('',#59711,10.) ;
#7133=VECTOR('',#59712,10.) ;
#7134=VECTOR('',#59715,0.600000000000023) ;
#7135=VECTOR('',#59720,0.600000000000023) ;
#7136=VECTOR('',#59725,10.) ;
#7137=VECTOR('',#59726,10.) ;
#7138=VECTOR('',#59729,10.) ;
#7139=VECTOR('',#59734,10.) ;
#7140=VECTOR('',#59735,10.) ;
#7141=VECTOR('',#59738,10.) ;
#7142=VECTOR('',#59743,10.) ;
#7143=VECTOR('',#59744,10.) ;
#7144=VECTOR('',#59747,10.) ;
#7145=VECTOR('',#59752,10.) ;
#7146=VECTOR('',#59753,10.) ;
#7147=VECTOR('',#59756,10.) ;
#7148=VECTOR('',#59761,10.) ;
#7149=VECTOR('',#59762,10.) ;
#7150=VECTOR('',#59765,10.) ;
#7151=VECTOR('',#59770,10.) ;
#7152=VECTOR('',#59771,10.) ;
#7153=VECTOR('',#59774,10.) ;
#7154=VECTOR('',#59779,10.) ;
#7155=VECTOR('',#59780,10.) ;
#7156=VECTOR('',#59783,10.) ;
#7157=VECTOR('',#59788,10.) ;
#7158=VECTOR('',#59797,10.) ;
#7159=VECTOR('',#59800,10.) ;
#7160=VECTOR('',#59815,10.) ;
#7161=VECTOR('',#59820,10.) ;
#7162=VECTOR('',#59821,10.) ;
#7163=VECTOR('',#59824,10.) ;
#7164=VECTOR('',#59825,10.) ;
#7165=VECTOR('',#59826,10.) ;
#7166=VECTOR('',#59831,10.) ;
#7167=VECTOR('',#59846,10.) ;
#7168=VECTOR('',#59847,10.) ;
#7169=VECTOR('',#59866,10.) ;
#7170=VECTOR('',#59877,10.) ;
#7171=VECTOR('',#59888,10.) ;
#7172=VECTOR('',#59899,10.) ;
#7173=VECTOR('',#59910,10.) ;
#7174=VECTOR('',#59913,10.) ;
#7175=VECTOR('',#59914,10.) ;
#7176=VECTOR('',#59917,10.) ;
#7177=VECTOR('',#59920,10.) ;
#7178=VECTOR('',#59921,10.) ;
#7179=VECTOR('',#59924,10.) ;
#7180=VECTOR('',#59925,10.) ;
#7181=VECTOR('',#59928,10.) ;
#7182=VECTOR('',#59929,10.) ;
#7183=VECTOR('',#59932,10.) ;
#7184=VECTOR('',#59933,10.) ;
#7185=VECTOR('',#59936,10.) ;
#7186=VECTOR('',#59937,10.) ;
#7187=VECTOR('',#59940,10.) ;
#7188=VECTOR('',#59963,10.) ;
#7189=VECTOR('',#59966,10.) ;
#7190=VECTOR('',#59967,10.) ;
#7191=VECTOR('',#59984,10.) ;
#7192=VECTOR('',#59995,10.) ;
#7193=VECTOR('',#60024,10.) ;
#7194=VECTOR('',#60027,10.) ;
#7195=VECTOR('',#60028,10.) ;
#7196=VECTOR('',#60031,10.) ;
#7197=VECTOR('',#60034,10.) ;
#7198=VECTOR('',#60035,10.) ;
#7199=VECTOR('',#60044,10.) ;
#7200=VECTOR('',#60047,10.) ;
#7201=VECTOR('',#60060,10.) ;
#7202=VECTOR('',#60061,10.) ;
#7203=VECTOR('',#60066,10.) ;
#7204=VECTOR('',#60069,10.) ;
#7205=VECTOR('',#60082,10.) ;
#7206=VECTOR('',#60085,10.) ;
#7207=VECTOR('',#60124,10.) ;
#7208=VECTOR('',#60127,10.) ;
#7209=VECTOR('',#60142,10.) ;
#7210=VECTOR('',#60147,10.) ;
#7211=VECTOR('',#60148,10.) ;
#7212=VECTOR('',#60151,10.) ;
#7213=VECTOR('',#60152,10.) ;
#7214=VECTOR('',#60153,10.) ;
#7215=VECTOR('',#60158,10.) ;
#7216=VECTOR('',#60173,10.) ;
#7217=VECTOR('',#60174,10.) ;
#7218=VECTOR('',#60209,10.) ;
#7219=VECTOR('',#60214,10.) ;
#7220=VECTOR('',#60217,10.) ;
#7221=VECTOR('',#60218,10.) ;
#7222=VECTOR('',#60221,10.) ;
#7223=VECTOR('',#60224,10.) ;
#7224=VECTOR('',#60225,10.) ;
#7225=VECTOR('',#60228,10.) ;
#7226=VECTOR('',#60231,10.) ;
#7227=VECTOR('',#60232,10.) ;
#7228=VECTOR('',#60235,10.) ;
#7229=VECTOR('',#60238,10.) ;
#7230=VECTOR('',#60239,10.) ;
#7231=VECTOR('',#60242,10.) ;
#7232=VECTOR('',#60255,10.) ;
#7233=VECTOR('',#60260,10.) ;
#7234=VECTOR('',#60321,10.) ;
#7235=VECTOR('',#60332,10.) ;
#7236=VECTOR('',#60335,10.) ;
#7237=VECTOR('',#60338,10.) ;
#7238=VECTOR('',#60339,10.) ;
#7239=VECTOR('',#60342,10.) ;
#7240=VECTOR('',#60345,10.) ;
#7241=VECTOR('',#60348,10.) ;
#7242=VECTOR('',#60349,10.) ;
#7243=VECTOR('',#60352,10.) ;
#7244=VECTOR('',#60353,10.) ;
#7245=VECTOR('',#60356,10.) ;
#7246=VECTOR('',#60359,10.) ;
#7247=VECTOR('',#60362,10.) ;
#7248=VECTOR('',#60365,10.) ;
#7249=VECTOR('',#60366,10.) ;
#7250=VECTOR('',#60383,2.5) ;
#7251=VECTOR('',#60396,10.) ;
#7252=VECTOR('',#60399,10.) ;
#7253=VECTOR('',#60414,10.) ;
#7254=VECTOR('',#60415,10.) ;
#7255=VECTOR('',#60418,10.) ;
#7256=VECTOR('',#60421,10.) ;
#7257=VECTOR('',#60422,10.) ;
#7258=VECTOR('',#60425,10.) ;
#7259=VECTOR('',#60426,10.) ;
#7260=VECTOR('',#60431,10.) ;
#7261=VECTOR('',#60492,10.) ;
#7262=VECTOR('',#60503,2.5) ;
#7263=VECTOR('',#60514,2.) ;
#7264=VECTOR('',#60623,10.) ;
#7265=VECTOR('',#60632,10.) ;
#7266=VECTOR('',#60655,2.8) ;
#7267=VECTOR('',#60676,2.8) ;
#7268=VECTOR('',#60701,2.) ;
#7269=VECTOR('',#60714,2.79999999999999) ;
#7270=VECTOR('',#60749,10.) ;
#7271=VECTOR('',#60750,10.) ;
#7272=VECTOR('',#60753,10.) ;
#7273=VECTOR('',#60800,10.) ;
#7274=VECTOR('',#60817,10.) ;
#7275=VECTOR('',#60822,10.) ;
#7276=VECTOR('',#60839,10.) ;
#7277=VECTOR('',#60846,10.) ;
#7278=VECTOR('',#60849,10.) ;
#7279=VECTOR('',#60854,10.) ;
#7280=VECTOR('',#60861,10.) ;
#7281=VECTOR('',#60866,10.) ;
#7282=VECTOR('',#60873,10.) ;
#7283=VECTOR('',#60878,10.) ;
#7284=VECTOR('',#60885,10.) ;
#7285=VECTOR('',#60886,10.) ;
#7286=VECTOR('',#60889,10.) ;
#7287=VECTOR('',#60894,10.) ;
#7288=VECTOR('',#60895,10.) ;
#7289=VECTOR('',#60902,10.) ;
#7290=VECTOR('',#60903,10.) ;
#7291=VECTOR('',#60910,10.) ;
#7292=VECTOR('',#60929,10.) ;
#7293=VECTOR('',#60932,10.) ;
#7294=VECTOR('',#60941,10.) ;
#9592=CYLINDRICAL_SURFACE('',#50165,0.12) ;
#9593=CYLINDRICAL_SURFACE('',#50167,0.12) ;
#9594=CYLINDRICAL_SURFACE('',#50169,0.12) ;
#9595=CYLINDRICAL_SURFACE('',#50174,0.12) ;
#9596=CYLINDRICAL_SURFACE('',#50176,0.12) ;
#9597=CYLINDRICAL_SURFACE('',#50178,0.12) ;
#9598=CYLINDRICAL_SURFACE('',#50180,0.12) ;
#9599=CYLINDRICAL_SURFACE('',#50183,0.12) ;
#9600=CYLINDRICAL_SURFACE('',#50185,0.12) ;
#9601=CYLINDRICAL_SURFACE('',#50187,0.12) ;
#9602=CYLINDRICAL_SURFACE('',#50189,0.12) ;
#9603=CYLINDRICAL_SURFACE('',#50194,0.12) ;
#9604=CYLINDRICAL_SURFACE('',#50196,0.12) ;
#9605=CYLINDRICAL_SURFACE('',#50198,0.12) ;
#9606=CYLINDRICAL_SURFACE('',#50200,0.12) ;
#9607=CYLINDRICAL_SURFACE('',#50203,0.12) ;
#9608=CYLINDRICAL_SURFACE('',#50205,0.12) ;
#9609=CYLINDRICAL_SURFACE('',#50209,0.12) ;
#9610=CYLINDRICAL_SURFACE('',#50212,0.12) ;
#9611=CYLINDRICAL_SURFACE('',#50214,0.12) ;
#9612=CYLINDRICAL_SURFACE('',#50216,0.12) ;
#9613=CYLINDRICAL_SURFACE('',#50220,0.12) ;
#9614=CYLINDRICAL_SURFACE('',#50223,0.12) ;
#9615=CYLINDRICAL_SURFACE('',#50225,0.12) ;
#9616=CYLINDRICAL_SURFACE('',#50229,0.12) ;
#9617=CYLINDRICAL_SURFACE('',#50231,0.12) ;
#9618=CYLINDRICAL_SURFACE('',#50234,0.12) ;
#9619=CYLINDRICAL_SURFACE('',#50237,0.12) ;
#9620=CYLINDRICAL_SURFACE('',#50239,0.12) ;
#9621=CYLINDRICAL_SURFACE('',#50241,0.12) ;
#9622=CYLINDRICAL_SURFACE('',#50243,0.12) ;
#9623=CYLINDRICAL_SURFACE('',#50244,0.12) ;
#9624=CYLINDRICAL_SURFACE('',#50325,0.12) ;
#9625=CYLINDRICAL_SURFACE('',#50328,0.12) ;
#9626=CYLINDRICAL_SURFACE('',#50330,0.12) ;
#9627=CYLINDRICAL_SURFACE('',#50332,0.12) ;
#9628=CYLINDRICAL_SURFACE('',#50335,0.12) ;
#9629=CYLINDRICAL_SURFACE('',#50337,0.12) ;
#9630=CYLINDRICAL_SURFACE('',#50339,0.12) ;
#9631=CYLINDRICAL_SURFACE('',#50341,0.12) ;
#9632=CYLINDRICAL_SURFACE('',#50344,0.12) ;
#9633=CYLINDRICAL_SURFACE('',#50346,0.12) ;
#9634=CYLINDRICAL_SURFACE('',#50356,2.) ;
#9635=CYLINDRICAL_SURFACE('',#50361,2.99999999999999) ;
#9636=CYLINDRICAL_SURFACE('',#50441,0.1) ;
#9637=CYLINDRICAL_SURFACE('',#50447,0.1) ;
#9638=CYLINDRICAL_SURFACE('',#50453,0.1) ;
#9639=CYLINDRICAL_SURFACE('',#50459,0.1) ;
#9640=CYLINDRICAL_SURFACE('',#50465,0.1) ;
#9641=CYLINDRICAL_SURFACE('',#50471,0.1) ;
#9642=CYLINDRICAL_SURFACE('',#50479,2.) ;
#9643=CYLINDRICAL_SURFACE('',#50482,2.) ;
#9644=CYLINDRICAL_SURFACE('',#50485,2.6) ;
#9645=CYLINDRICAL_SURFACE('',#50488,2.) ;
#9646=CYLINDRICAL_SURFACE('',#50491,2.) ;
#9647=CYLINDRICAL_SURFACE('',#50498,3.) ;
#9648=CYLINDRICAL_SURFACE('',#50509,2.) ;
#9649=CYLINDRICAL_SURFACE('',#50516,1.85) ;
#9650=CYLINDRICAL_SURFACE('',#50531,1.85) ;
#9651=CYLINDRICAL_SURFACE('',#50545,0.1) ;
#9652=CYLINDRICAL_SURFACE('',#50550,0.1) ;
#9653=CYLINDRICAL_SURFACE('',#50558,0.1) ;
#9654=CYLINDRICAL_SURFACE('',#50566,0.1) ;
#9655=CYLINDRICAL_SURFACE('',#50568,0.4) ;
#9656=CYLINDRICAL_SURFACE('',#50573,0.4) ;
#9657=CYLINDRICAL_SURFACE('',#50576,0.4) ;
#9658=CYLINDRICAL_SURFACE('',#50577,0.1) ;
#9659=CYLINDRICAL_SURFACE('',#50583,0.1) ;
#9660=CYLINDRICAL_SURFACE('',#50588,0.1) ;
#9661=CYLINDRICAL_SURFACE('',#50590,0.4) ;
#9662=CYLINDRICAL_SURFACE('',#50591,1.7) ;
#9663=CYLINDRICAL_SURFACE('',#50596,0.1) ;
#9664=CYLINDRICAL_SURFACE('',#50605,0.1) ;
#9665=CYLINDRICAL_SURFACE('',#50614,0.1) ;
#9666=CYLINDRICAL_SURFACE('',#50615,0.1) ;
#9667=CYLINDRICAL_SURFACE('',#50620,0.1) ;
#9668=CYLINDRICAL_SURFACE('',#50621,0.1) ;
#9669=CYLINDRICAL_SURFACE('',#50626,0.1) ;
#9670=CYLINDRICAL_SURFACE('',#50631,0.1) ;
#9671=CYLINDRICAL_SURFACE('',#50634,0.1) ;
#9672=CYLINDRICAL_SURFACE('',#50636,0.1) ;
#9673=CYLINDRICAL_SURFACE('',#50643,0.1) ;
#9674=CYLINDRICAL_SURFACE('',#50647,0.1) ;
#9675=CYLINDRICAL_SURFACE('',#50653,0.1) ;
#9676=CYLINDRICAL_SURFACE('',#50659,0.1) ;
#9677=CYLINDRICAL_SURFACE('',#50661,0.1) ;
#9678=CYLINDRICAL_SURFACE('',#50667,0.1) ;
#9679=CYLINDRICAL_SURFACE('',#50672,0.1) ;
#9680=CYLINDRICAL_SURFACE('',#50676,0.1) ;
#9681=CYLINDRICAL_SURFACE('',#50679,0.1) ;
#9682=CYLINDRICAL_SURFACE('',#50682,0.1) ;
#9683=CYLINDRICAL_SURFACE('',#50685,0.1) ;
#9684=CYLINDRICAL_SURFACE('',#50688,0.1) ;
#9685=CYLINDRICAL_SURFACE('',#50691,0.1) ;
#9686=CYLINDRICAL_SURFACE('',#50694,0.1) ;
#9687=CYLINDRICAL_SURFACE('',#50700,0.1) ;
#9688=CYLINDRICAL_SURFACE('',#50705,0.1) ;
#9689=CYLINDRICAL_SURFACE('',#50710,0.1) ;
#9690=CYLINDRICAL_SURFACE('',#50715,0.1) ;
#9691=CYLINDRICAL_SURFACE('',#50717,0.1) ;
#9692=CYLINDRICAL_SURFACE('',#50723,0.1) ;
#9693=CYLINDRICAL_SURFACE('',#50728,0.1) ;
#9694=CYLINDRICAL_SURFACE('',#50734,0.1) ;
#9695=CYLINDRICAL_SURFACE('',#50737,0.1) ;
#9696=CYLINDRICAL_SURFACE('',#50740,0.1) ;
#9697=CYLINDRICAL_SURFACE('',#50743,0.1) ;
#9698=CYLINDRICAL_SURFACE('',#50754,0.1) ;
#9699=CYLINDRICAL_SURFACE('',#50759,0.1) ;
#9700=CYLINDRICAL_SURFACE('',#50764,0.1) ;
#9701=CYLINDRICAL_SURFACE('',#50769,0.1) ;
#9702=CYLINDRICAL_SURFACE('',#50774,0.1) ;
#9703=CYLINDRICAL_SURFACE('',#50775,0.1) ;
#9704=CYLINDRICAL_SURFACE('',#50777,0.1) ;
#9705=CYLINDRICAL_SURFACE('',#50781,0.1) ;
#9706=CYLINDRICAL_SURFACE('',#50785,0.1) ;
#9707=CYLINDRICAL_SURFACE('',#50792,0.1) ;
#9708=CYLINDRICAL_SURFACE('',#50794,0.1) ;
#9709=CYLINDRICAL_SURFACE('',#50800,0.1) ;
#9710=CYLINDRICAL_SURFACE('',#50805,0.1) ;
#9711=CYLINDRICAL_SURFACE('',#50809,0.1) ;
#9712=CYLINDRICAL_SURFACE('',#50818,0.1) ;
#9713=CYLINDRICAL_SURFACE('',#50821,0.1) ;
#9714=CYLINDRICAL_SURFACE('',#50824,0.1) ;
#9715=CYLINDRICAL_SURFACE('',#50827,0.1) ;
#9716=CYLINDRICAL_SURFACE('',#50834,0.1) ;
#9717=CYLINDRICAL_SURFACE('',#50836,0.1) ;
#9718=CYLINDRICAL_SURFACE('',#50842,0.1) ;
#9719=CYLINDRICAL_SURFACE('',#50847,0.1) ;
#9720=CYLINDRICAL_SURFACE('',#50851,0.1) ;
#9721=CYLINDRICAL_SURFACE('',#50860,0.1) ;
#9722=CYLINDRICAL_SURFACE('',#50863,0.1) ;
#9723=CYLINDRICAL_SURFACE('',#50866,0.1) ;
#9724=CYLINDRICAL_SURFACE('',#50869,0.1) ;
#9725=CYLINDRICAL_SURFACE('',#50872,0.1) ;
#9726=CYLINDRICAL_SURFACE('',#50874,0.1) ;
#9727=CYLINDRICAL_SURFACE('',#50882,0.1) ;
#9728=CYLINDRICAL_SURFACE('',#50887,0.1) ;
#9729=CYLINDRICAL_SURFACE('',#50892,0.1) ;
#9730=CYLINDRICAL_SURFACE('',#50897,0.1) ;
#9731=CYLINDRICAL_SURFACE('',#50902,0.1) ;
#9732=CYLINDRICAL_SURFACE('',#50907,0.1) ;
#9733=CYLINDRICAL_SURFACE('',#50909,0.1) ;
#9734=CYLINDRICAL_SURFACE('',#50912,0.1) ;
#9735=CYLINDRICAL_SURFACE('',#50915,0.1) ;
#9736=CYLINDRICAL_SURFACE('',#50918,0.1) ;
#9737=CYLINDRICAL_SURFACE('',#50921,0.1) ;
#9738=CYLINDRICAL_SURFACE('',#50930,0.1) ;
#9739=CYLINDRICAL_SURFACE('',#50939,0.1) ;
#9740=CYLINDRICAL_SURFACE('',#50940,0.1) ;
#9741=CYLINDRICAL_SURFACE('',#50941,0.1) ;
#9742=CYLINDRICAL_SURFACE('',#50946,0.1) ;
#9743=CYLINDRICAL_SURFACE('',#50947,0.1) ;
#9744=CYLINDRICAL_SURFACE('',#50948,0.1) ;
#9745=CYLINDRICAL_SURFACE('',#50949,0.1) ;
#9746=CYLINDRICAL_SURFACE('',#50951,0.1) ;
#9747=CYLINDRICAL_SURFACE('',#50967,0.1) ;
#9748=CYLINDRICAL_SURFACE('',#50974,0.1) ;
#9749=CYLINDRICAL_SURFACE('',#50983,0.1) ;
#9750=CYLINDRICAL_SURFACE('',#50984,0.1) ;
#9751=CYLINDRICAL_SURFACE('',#50993,0.1) ;
#9752=CYLINDRICAL_SURFACE('',#50994,0.1) ;
#9753=CYLINDRICAL_SURFACE('',#50995,0.1) ;
#9754=CYLINDRICAL_SURFACE('',#50996,0.1) ;
#9755=CYLINDRICAL_SURFACE('',#50997,0.1) ;
#9756=CYLINDRICAL_SURFACE('',#50998,0.1) ;
#9757=CYLINDRICAL_SURFACE('',#50999,0.1) ;
#9758=CYLINDRICAL_SURFACE('',#51000,0.1) ;
#9759=CYLINDRICAL_SURFACE('',#51001,0.1) ;
#9760=CYLINDRICAL_SURFACE('',#51003,0.1) ;
#9761=CYLINDRICAL_SURFACE('',#51019,0.1) ;
#9762=CYLINDRICAL_SURFACE('',#51023,0.1) ;
#9763=CYLINDRICAL_SURFACE('',#51031,0.1) ;
#9764=CYLINDRICAL_SURFACE('',#51040,0.1) ;
#9765=CYLINDRICAL_SURFACE('',#51041,0.1) ;
#9766=CYLINDRICAL_SURFACE('',#51046,0.1) ;
#9767=CYLINDRICAL_SURFACE('',#51047,0.1) ;
#9768=CYLINDRICAL_SURFACE('',#51048,0.1) ;
#9769=CYLINDRICAL_SURFACE('',#51049,0.1) ;
#9770=CYLINDRICAL_SURFACE('',#51050,0.1) ;
#9771=CYLINDRICAL_SURFACE('',#51051,0.1) ;
#9772=CYLINDRICAL_SURFACE('',#51052,0.1) ;
#9773=CYLINDRICAL_SURFACE('',#51053,0.1) ;
#9774=CYLINDRICAL_SURFACE('',#51055,0.1) ;
#9775=CYLINDRICAL_SURFACE('',#51064,0.1) ;
#9776=CYLINDRICAL_SURFACE('',#51070,0.1) ;
#9777=CYLINDRICAL_SURFACE('',#51075,0.1) ;
#9778=CYLINDRICAL_SURFACE('',#51080,0.1) ;
#9779=CYLINDRICAL_SURFACE('',#51084,0.1) ;
#9780=CYLINDRICAL_SURFACE('',#51089,0.1) ;
#9781=CYLINDRICAL_SURFACE('',#51094,0.1) ;
#9782=CYLINDRICAL_SURFACE('',#51099,0.1) ;
#9783=CYLINDRICAL_SURFACE('',#51107,0.1) ;
#9784=CYLINDRICAL_SURFACE('',#51115,0.1) ;
#9785=CYLINDRICAL_SURFACE('',#51120,0.1) ;
#9786=CYLINDRICAL_SURFACE('',#51125,0.1) ;
#9787=CYLINDRICAL_SURFACE('',#51130,0.1) ;
#9788=CYLINDRICAL_SURFACE('',#51135,0.1) ;
#9789=CYLINDRICAL_SURFACE('',#51140,0.1) ;
#9790=CYLINDRICAL_SURFACE('',#51145,0.1) ;
#9791=CYLINDRICAL_SURFACE('',#51150,0.1) ;
#9792=CYLINDRICAL_SURFACE('',#51155,0.1) ;
#9793=CYLINDRICAL_SURFACE('',#51156,0.1) ;
#9794=CYLINDRICAL_SURFACE('',#51157,0.1) ;
#9795=CYLINDRICAL_SURFACE('',#51162,1.2) ;
#9796=CYLINDRICAL_SURFACE('',#51166,0.6) ;
#9797=CYLINDRICAL_SURFACE('',#51169,0.600000000000005) ;
#9798=CYLINDRICAL_SURFACE('',#51171,2.49999999999996) ;
#9799=CYLINDRICAL_SURFACE('',#51174,2.49999999999999) ;
#9800=CYLINDRICAL_SURFACE('',#51176,0.600000000000023) ;
#9801=CYLINDRICAL_SURFACE('',#51179,0.6) ;
#9802=CYLINDRICAL_SURFACE('',#51182,0.6) ;
#9803=CYLINDRICAL_SURFACE('',#51185,4.) ;
#9804=CYLINDRICAL_SURFACE('',#51188,4.) ;
#9805=CYLINDRICAL_SURFACE('',#51191,4.) ;
#9806=CYLINDRICAL_SURFACE('',#51194,0.6) ;
#9807=CYLINDRICAL_SURFACE('',#51197,0.6) ;
#9808=CYLINDRICAL_SURFACE('',#51200,0.1) ;
#9809=CYLINDRICAL_SURFACE('',#51202,0.1) ;
#9810=CYLINDRICAL_SURFACE('',#51209,0.1) ;
#9811=CYLINDRICAL_SURFACE('',#51211,1.) ;
#9812=CYLINDRICAL_SURFACE('',#51216,0.1) ;
#9813=CYLINDRICAL_SURFACE('',#51221,0.1) ;
#9814=CYLINDRICAL_SURFACE('',#51232,0.1) ;
#9815=CYLINDRICAL_SURFACE('',#51237,0.1) ;
#9816=CYLINDRICAL_SURFACE('',#51242,0.1) ;
#9817=CYLINDRICAL_SURFACE('',#51247,0.1) ;
#9818=CYLINDRICAL_SURFACE('',#51252,0.1) ;
#9819=CYLINDRICAL_SURFACE('',#51253,0.1) ;
#9820=CYLINDRICAL_SURFACE('',#51254,0.1) ;
#9821=CYLINDRICAL_SURFACE('',#51255,0.1) ;
#9822=CYLINDRICAL_SURFACE('',#51256,0.1) ;
#9823=CYLINDRICAL_SURFACE('',#51257,0.1) ;
#9824=CYLINDRICAL_SURFACE('',#51258,0.1) ;
#9825=CYLINDRICAL_SURFACE('',#51259,0.1) ;
#9826=CYLINDRICAL_SURFACE('',#51260,0.1) ;
#9827=CYLINDRICAL_SURFACE('',#51271,0.1) ;
#9828=CYLINDRICAL_SURFACE('',#51272,0.1) ;
#9829=CYLINDRICAL_SURFACE('',#51280,0.1) ;
#9830=CYLINDRICAL_SURFACE('',#51285,0.1) ;
#9831=CYLINDRICAL_SURFACE('',#51289,0.1) ;
#9832=CYLINDRICAL_SURFACE('',#51296,0.1) ;
#9833=CYLINDRICAL_SURFACE('',#51297,0.1) ;
#9834=CYLINDRICAL_SURFACE('',#51298,0.1) ;
#9835=CYLINDRICAL_SURFACE('',#51299,0.1) ;
#9836=CYLINDRICAL_SURFACE('',#51300,0.1) ;
#9837=CYLINDRICAL_SURFACE('',#51301,0.1) ;
#9838=CYLINDRICAL_SURFACE('',#51302,0.1) ;
#9839=CYLINDRICAL_SURFACE('',#51305,0.1) ;
#9840=CYLINDRICAL_SURFACE('',#51312,0.1) ;
#9841=CYLINDRICAL_SURFACE('',#51314,0.1) ;
#9842=CYLINDRICAL_SURFACE('',#51321,0.1) ;
#9843=CYLINDRICAL_SURFACE('',#51322,1.) ;
#9844=CYLINDRICAL_SURFACE('',#51327,0.1) ;
#9845=CYLINDRICAL_SURFACE('',#51331,0.1) ;
#9846=CYLINDRICAL_SURFACE('',#51335,0.1) ;
#9847=CYLINDRICAL_SURFACE('',#51339,0.1) ;
#9848=CYLINDRICAL_SURFACE('',#51340,0.1) ;
#9849=CYLINDRICAL_SURFACE('',#51341,0.1) ;
#9850=CYLINDRICAL_SURFACE('',#51348,0.1) ;
#9851=CYLINDRICAL_SURFACE('',#51350,1.) ;
#9852=CYLINDRICAL_SURFACE('',#51355,0.1) ;
#9853=CYLINDRICAL_SURFACE('',#51360,0.1) ;
#9854=CYLINDRICAL_SURFACE('',#51379,0.1) ;
#9855=CYLINDRICAL_SURFACE('',#51380,0.1) ;
#9856=CYLINDRICAL_SURFACE('',#51381,0.1) ;
#9857=CYLINDRICAL_SURFACE('',#51382,0.1) ;
#9858=CYLINDRICAL_SURFACE('',#51383,0.1) ;
#9859=CYLINDRICAL_SURFACE('',#51384,0.1) ;
#9860=CYLINDRICAL_SURFACE('',#51385,0.1) ;
#9861=CYLINDRICAL_SURFACE('',#51386,0.1) ;
#9862=CYLINDRICAL_SURFACE('',#51387,0.1) ;
#9863=CYLINDRICAL_SURFACE('',#51388,0.1) ;
#9864=CYLINDRICAL_SURFACE('',#51389,0.1) ;
#9865=CYLINDRICAL_SURFACE('',#51395,0.1) ;
#9866=CYLINDRICAL_SURFACE('',#51397,0.1) ;
#9867=CYLINDRICAL_SURFACE('',#51427,0.1) ;
#9868=CYLINDRICAL_SURFACE('',#51432,0.1) ;
#9869=CYLINDRICAL_SURFACE('',#51433,0.1) ;
#9870=CYLINDRICAL_SURFACE('',#51434,0.1) ;
#9871=CYLINDRICAL_SURFACE('',#51435,0.1) ;
#9872=CYLINDRICAL_SURFACE('',#51436,0.1) ;
#9873=CYLINDRICAL_SURFACE('',#51437,0.1) ;
#9874=CYLINDRICAL_SURFACE('',#51438,0.1) ;
#9875=CYLINDRICAL_SURFACE('',#51439,0.1) ;
#9876=CYLINDRICAL_SURFACE('',#51440,0.1) ;
#9877=CYLINDRICAL_SURFACE('',#51441,0.1) ;
#9878=CYLINDRICAL_SURFACE('',#51442,0.1) ;
#9879=CYLINDRICAL_SURFACE('',#51450,2.5) ;
#9880=CYLINDRICAL_SURFACE('',#51455,0.1) ;
#9881=CYLINDRICAL_SURFACE('',#51462,0.1) ;
#9882=CYLINDRICAL_SURFACE('',#51468,0.1) ;
#9883=CYLINDRICAL_SURFACE('',#51474,0.1) ;
#9884=CYLINDRICAL_SURFACE('',#51476,1.) ;
#9885=CYLINDRICAL_SURFACE('',#51480,0.1) ;
#9886=CYLINDRICAL_SURFACE('',#51485,0.1) ;
#9887=CYLINDRICAL_SURFACE('',#51489,0.1) ;
#9888=CYLINDRICAL_SURFACE('',#51493,0.1) ;
#9889=CYLINDRICAL_SURFACE('',#51497,0.1) ;
#9890=CYLINDRICAL_SURFACE('',#51498,0.1) ;
#9891=CYLINDRICAL_SURFACE('',#51499,0.1) ;
#9892=CYLINDRICAL_SURFACE('',#51504,2.5) ;
#9893=CYLINDRICAL_SURFACE('',#51509,2.) ;
#9894=CYLINDRICAL_SURFACE('',#51510,0.1) ;
#9895=CYLINDRICAL_SURFACE('',#51515,0.1) ;
#9896=CYLINDRICAL_SURFACE('',#51519,0.1) ;
#9897=CYLINDRICAL_SURFACE('',#51525,0.1) ;
#9898=CYLINDRICAL_SURFACE('',#51531,0.1) ;
#9899=CYLINDRICAL_SURFACE('',#51535,0.1) ;
#9900=CYLINDRICAL_SURFACE('',#51539,0.1) ;
#9901=CYLINDRICAL_SURFACE('',#51543,0.1) ;
#9902=CYLINDRICAL_SURFACE('',#51547,0.1) ;
#9903=CYLINDRICAL_SURFACE('',#51551,0.1) ;
#9904=CYLINDRICAL_SURFACE('',#51555,0.1) ;
#9905=CYLINDRICAL_SURFACE('',#51558,0.6) ;
#9906=CYLINDRICAL_SURFACE('',#51562,0.1) ;
#9907=CYLINDRICAL_SURFACE('',#51567,0.1) ;
#9908=CYLINDRICAL_SURFACE('',#51577,2.8) ;
#9909=CYLINDRICAL_SURFACE('',#51588,2.8) ;
#9910=CYLINDRICAL_SURFACE('',#51599,2.) ;
#9911=CYLINDRICAL_SURFACE('',#51606,2.79999999999999) ;
#9912=CYLINDRICAL_SURFACE('',#51623,0.6) ;
#9913=CYLINDRICAL_SURFACE('',#51625,0.6) ;
#9914=CYLINDRICAL_SURFACE('',#51647,1.2) ;
#9915=CYLINDRICAL_SURFACE('',#51651,1.2) ;
#9916=CYLINDRICAL_SURFACE('',#51655,1.2) ;
#9917=CYLINDRICAL_SURFACE('',#51656,1.2) ;
#9918=CYLINDRICAL_SURFACE('',#51657,1.2) ;
#9919=CYLINDRICAL_SURFACE('',#51661,1.2) ;
#9920=CYLINDRICAL_SURFACE('',#51665,1.2) ;
#9921=CYLINDRICAL_SURFACE('',#51666,1.2) ;
#9922=CYLINDRICAL_SURFACE('',#51667,0.5) ;
#9923=CYLINDRICAL_SURFACE('',#51669,0.5) ;
#9924=CYLINDRICAL_SURFACE('',#51672,0.5) ;
#9925=CYLINDRICAL_SURFACE('',#51674,0.5) ;
#9926=CYLINDRICAL_SURFACE('',#51677,0.5) ;
#9927=CYLINDRICAL_SURFACE('',#51679,0.5) ;
#9928=CYLINDRICAL_SURFACE('',#51682,0.5) ;
#9929=CYLINDRICAL_SURFACE('',#51701,1.7) ;
#9930=CYLINDRICAL_SURFACE('',#51702,1.7) ;
#9931=CYLINDRICAL_SURFACE('',#51703,1.7) ;
#9932=CYLINDRICAL_SURFACE('',#51707,0.5) ;
#11208=FACE_OUTER_BOUND('',#14309,.T.) ;
#11209=FACE_OUTER_BOUND('',#14310,.T.) ;
#11210=FACE_OUTER_BOUND('',#14311,.T.) ;
#11211=FACE_OUTER_BOUND('',#14312,.T.) ;
#11212=FACE_OUTER_BOUND('',#14313,.T.) ;
#11213=FACE_OUTER_BOUND('',#14314,.T.) ;
#11214=FACE_OUTER_BOUND('',#14315,.T.) ;
#11215=FACE_OUTER_BOUND('',#14316,.T.) ;
#11216=FACE_OUTER_BOUND('',#14317,.T.) ;
#11217=FACE_OUTER_BOUND('',#14318,.T.) ;
#11218=FACE_OUTER_BOUND('',#14319,.T.) ;
#11219=FACE_OUTER_BOUND('',#14320,.T.) ;
#11220=FACE_OUTER_BOUND('',#14321,.T.) ;
#11221=FACE_OUTER_BOUND('',#14323,.T.) ;
#11222=FACE_OUTER_BOUND('',#14324,.T.) ;
#11223=FACE_OUTER_BOUND('',#14325,.T.) ;
#11224=FACE_OUTER_BOUND('',#14326,.T.) ;
#11225=FACE_OUTER_BOUND('',#14327,.T.) ;
#11226=FACE_OUTER_BOUND('',#14328,.T.) ;
#11227=FACE_OUTER_BOUND('',#14329,.T.) ;
#11228=FACE_OUTER_BOUND('',#14330,.T.) ;
#11229=FACE_OUTER_BOUND('',#14331,.T.) ;
#11230=FACE_OUTER_BOUND('',#14332,.T.) ;
#11231=FACE_OUTER_BOUND('',#14333,.T.) ;
#11232=FACE_OUTER_BOUND('',#14334,.T.) ;
#11233=FACE_OUTER_BOUND('',#14335,.T.) ;
#11234=FACE_OUTER_BOUND('',#14336,.T.) ;
#11235=FACE_OUTER_BOUND('',#14337,.T.) ;
#11236=FACE_OUTER_BOUND('',#14338,.T.) ;
#11237=FACE_OUTER_BOUND('',#14339,.T.) ;
#11238=FACE_OUTER_BOUND('',#14340,.T.) ;
#11239=FACE_OUTER_BOUND('',#14341,.T.) ;
#11240=FACE_OUTER_BOUND('',#14342,.T.) ;
#11241=FACE_OUTER_BOUND('',#14343,.T.) ;
#11242=FACE_OUTER_BOUND('',#14344,.T.) ;
#11243=FACE_OUTER_BOUND('',#14345,.T.) ;
#11244=FACE_OUTER_BOUND('',#14346,.T.) ;
#11245=FACE_OUTER_BOUND('',#14347,.T.) ;
#11246=FACE_OUTER_BOUND('',#14348,.T.) ;
#11247=FACE_OUTER_BOUND('',#14349,.T.) ;
#11248=FACE_OUTER_BOUND('',#14350,.T.) ;
#11249=FACE_OUTER_BOUND('',#14351,.T.) ;
#11250=FACE_OUTER_BOUND('',#14352,.T.) ;
#11251=FACE_OUTER_BOUND('',#14353,.T.) ;
#11252=FACE_OUTER_BOUND('',#14354,.T.) ;
#11253=FACE_OUTER_BOUND('',#14355,.T.) ;
#11254=FACE_OUTER_BOUND('',#14356,.T.) ;
#11255=FACE_OUTER_BOUND('',#14357,.T.) ;
#11256=FACE_OUTER_BOUND('',#14358,.T.) ;
#11257=FACE_OUTER_BOUND('',#14359,.T.) ;
#11258=FACE_OUTER_BOUND('',#14360,.T.) ;
#11259=FACE_OUTER_BOUND('',#14361,.T.) ;
#11260=FACE_OUTER_BOUND('',#14362,.T.) ;
#11261=FACE_OUTER_BOUND('',#14363,.T.) ;
#11262=FACE_OUTER_BOUND('',#14364,.T.) ;
#11263=FACE_OUTER_BOUND('',#14365,.T.) ;
#11264=FACE_OUTER_BOUND('',#14366,.T.) ;
#11265=FACE_OUTER_BOUND('',#14367,.T.) ;
#11266=FACE_OUTER_BOUND('',#14368,.T.) ;
#11267=FACE_OUTER_BOUND('',#14369,.T.) ;
#11268=FACE_OUTER_BOUND('',#14370,.T.) ;
#11269=FACE_OUTER_BOUND('',#14371,.T.) ;
#11270=FACE_OUTER_BOUND('',#14372,.T.) ;
#11271=FACE_OUTER_BOUND('',#14373,.T.) ;
#11272=FACE_OUTER_BOUND('',#14374,.T.) ;
#11273=FACE_OUTER_BOUND('',#14375,.T.) ;
#11274=FACE_OUTER_BOUND('',#14376,.T.) ;
#11275=FACE_OUTER_BOUND('',#14377,.T.) ;
#11276=FACE_OUTER_BOUND('',#14378,.T.) ;
#11277=FACE_OUTER_BOUND('',#14379,.T.) ;
#11278=FACE_OUTER_BOUND('',#14380,.T.) ;
#11279=FACE_OUTER_BOUND('',#14381,.T.) ;
#11280=FACE_OUTER_BOUND('',#14382,.T.) ;
#11281=FACE_OUTER_BOUND('',#14383,.T.) ;
#11282=FACE_OUTER_BOUND('',#14384,.T.) ;
#11283=FACE_OUTER_BOUND('',#14385,.T.) ;
#11284=FACE_OUTER_BOUND('',#14386,.T.) ;
#11285=FACE_OUTER_BOUND('',#14387,.T.) ;
#11286=FACE_OUTER_BOUND('',#14388,.T.) ;
#11287=FACE_OUTER_BOUND('',#14389,.T.) ;
#11288=FACE_OUTER_BOUND('',#14390,.T.) ;
#11289=FACE_OUTER_BOUND('',#14391,.T.) ;
#11290=FACE_OUTER_BOUND('',#14392,.T.) ;
#11291=FACE_OUTER_BOUND('',#14393,.T.) ;
#11292=FACE_OUTER_BOUND('',#14394,.T.) ;
#11293=FACE_OUTER_BOUND('',#14395,.T.) ;
#11294=FACE_OUTER_BOUND('',#14396,.T.) ;
#11295=FACE_OUTER_BOUND('',#14397,.T.) ;
#11296=FACE_OUTER_BOUND('',#14398,.T.) ;
#11297=FACE_OUTER_BOUND('',#14399,.T.) ;
#11298=FACE_OUTER_BOUND('',#14400,.T.) ;
#11299=FACE_OUTER_BOUND('',#14401,.T.) ;
#11300=FACE_OUTER_BOUND('',#14402,.T.) ;
#11301=FACE_OUTER_BOUND('',#14403,.T.) ;
#11302=FACE_OUTER_BOUND('',#14404,.T.) ;
#11303=FACE_OUTER_BOUND('',#14405,.T.) ;
#11304=FACE_OUTER_BOUND('',#14406,.T.) ;
#11305=FACE_OUTER_BOUND('',#14407,.T.) ;
#11306=FACE_OUTER_BOUND('',#14426,.T.) ;
#11307=FACE_OUTER_BOUND('',#14427,.T.) ;
#11308=FACE_OUTER_BOUND('',#14428,.T.) ;
#11309=FACE_OUTER_BOUND('',#14429,.T.) ;
#11310=FACE_OUTER_BOUND('',#14430,.T.) ;
#11311=FACE_OUTER_BOUND('',#14431,.T.) ;
#11312=FACE_OUTER_BOUND('',#14432,.T.) ;
#11313=FACE_OUTER_BOUND('',#14433,.T.) ;
#11314=FACE_OUTER_BOUND('',#14434,.T.) ;
#11315=FACE_OUTER_BOUND('',#14435,.T.) ;
#11316=FACE_OUTER_BOUND('',#14436,.T.) ;
#11317=FACE_OUTER_BOUND('',#14437,.T.) ;
#11318=FACE_OUTER_BOUND('',#14438,.T.) ;
#11319=FACE_OUTER_BOUND('',#14439,.T.) ;
#11320=FACE_OUTER_BOUND('',#14440,.T.) ;
#11321=FACE_OUTER_BOUND('',#14441,.T.) ;
#11322=FACE_OUTER_BOUND('',#14442,.T.) ;
#11323=FACE_OUTER_BOUND('',#14443,.T.) ;
#11324=FACE_OUTER_BOUND('',#14444,.T.) ;
#11325=FACE_OUTER_BOUND('',#14445,.T.) ;
#11326=FACE_OUTER_BOUND('',#14446,.T.) ;
#11327=FACE_OUTER_BOUND('',#14448,.T.) ;
#11328=FACE_OUTER_BOUND('',#14449,.T.) ;
#11329=FACE_OUTER_BOUND('',#14450,.T.) ;
#11330=FACE_OUTER_BOUND('',#14451,.T.) ;
#11331=FACE_OUTER_BOUND('',#14452,.T.) ;
#11332=FACE_OUTER_BOUND('',#14467,.T.) ;
#11333=FACE_OUTER_BOUND('',#14468,.T.) ;
#11334=FACE_OUTER_BOUND('',#14469,.T.) ;
#11335=FACE_OUTER_BOUND('',#14470,.T.) ;
#11336=FACE_OUTER_BOUND('',#14471,.T.) ;
#11337=FACE_OUTER_BOUND('',#14472,.T.) ;
#11338=FACE_OUTER_BOUND('',#14473,.T.) ;
#11339=FACE_OUTER_BOUND('',#14474,.T.) ;
#11340=FACE_OUTER_BOUND('',#14475,.T.) ;
#11341=FACE_OUTER_BOUND('',#14476,.T.) ;
#11342=FACE_OUTER_BOUND('',#14477,.T.) ;
#11343=FACE_OUTER_BOUND('',#14478,.T.) ;
#11344=FACE_OUTER_BOUND('',#14479,.T.) ;
#11345=FACE_OUTER_BOUND('',#14480,.T.) ;
#11346=FACE_OUTER_BOUND('',#14481,.T.) ;
#11347=FACE_OUTER_BOUND('',#14482,.T.) ;
#11348=FACE_OUTER_BOUND('',#14483,.T.) ;
#11349=FACE_OUTER_BOUND('',#14484,.T.) ;
#11350=FACE_OUTER_BOUND('',#14485,.T.) ;
#11351=FACE_OUTER_BOUND('',#14486,.T.) ;
#11352=FACE_OUTER_BOUND('',#14487,.T.) ;
#11353=FACE_OUTER_BOUND('',#14488,.T.) ;
#11354=FACE_OUTER_BOUND('',#14489,.T.) ;
#11355=FACE_OUTER_BOUND('',#14490,.T.) ;
#11356=FACE_OUTER_BOUND('',#14491,.T.) ;
#11357=FACE_OUTER_BOUND('',#14492,.T.) ;
#11358=FACE_OUTER_BOUND('',#14493,.T.) ;
#11359=FACE_OUTER_BOUND('',#14494,.T.) ;
#11360=FACE_OUTER_BOUND('',#14495,.T.) ;
#11361=FACE_OUTER_BOUND('',#14497,.T.) ;
#11362=FACE_OUTER_BOUND('',#14498,.T.) ;
#11363=FACE_OUTER_BOUND('',#14499,.T.) ;
#11364=FACE_OUTER_BOUND('',#14500,.T.) ;
#11365=FACE_OUTER_BOUND('',#14501,.T.) ;
#11366=FACE_OUTER_BOUND('',#14503,.T.) ;
#11367=FACE_OUTER_BOUND('',#14504,.T.) ;
#11368=FACE_OUTER_BOUND('',#14506,.T.) ;
#11369=FACE_OUTER_BOUND('',#14507,.T.) ;
#11370=FACE_OUTER_BOUND('',#14508,.T.) ;
#11371=FACE_OUTER_BOUND('',#14510,.T.) ;
#11372=FACE_OUTER_BOUND('',#14511,.T.) ;
#11373=FACE_OUTER_BOUND('',#14513,.T.) ;
#11374=FACE_OUTER_BOUND('',#14514,.T.) ;
#11375=FACE_OUTER_BOUND('',#14515,.T.) ;
#11376=FACE_OUTER_BOUND('',#14516,.T.) ;
#11377=FACE_OUTER_BOUND('',#14517,.T.) ;
#11378=FACE_OUTER_BOUND('',#14518,.T.) ;
#11379=FACE_OUTER_BOUND('',#14519,.T.) ;
#11380=FACE_OUTER_BOUND('',#14520,.T.) ;
#11381=FACE_OUTER_BOUND('',#14521,.T.) ;
#11382=FACE_OUTER_BOUND('',#14522,.T.) ;
#11383=FACE_OUTER_BOUND('',#14523,.T.) ;
#11384=FACE_OUTER_BOUND('',#14524,.T.) ;
#11385=FACE_OUTER_BOUND('',#14525,.T.) ;
#11386=FACE_OUTER_BOUND('',#14526,.T.) ;
#11387=FACE_OUTER_BOUND('',#14527,.T.) ;
#11388=FACE_OUTER_BOUND('',#14528,.T.) ;
#11389=FACE_OUTER_BOUND('',#14529,.T.) ;
#11390=FACE_OUTER_BOUND('',#14530,.T.) ;
#11391=FACE_OUTER_BOUND('',#14531,.T.) ;
#11392=FACE_OUTER_BOUND('',#14532,.T.) ;
#11393=FACE_OUTER_BOUND('',#14533,.T.) ;
#11394=FACE_OUTER_BOUND('',#14534,.T.) ;
#11395=FACE_OUTER_BOUND('',#14535,.T.) ;
#11396=FACE_OUTER_BOUND('',#14536,.T.) ;
#11397=FACE_OUTER_BOUND('',#14537,.T.) ;
#11398=FACE_OUTER_BOUND('',#14538,.T.) ;
#11399=FACE_OUTER_BOUND('',#14539,.T.) ;
#11400=FACE_OUTER_BOUND('',#14540,.T.) ;
#11401=FACE_OUTER_BOUND('',#14541,.T.) ;
#11402=FACE_OUTER_BOUND('',#14542,.T.) ;
#11403=FACE_OUTER_BOUND('',#14543,.T.) ;
#11404=FACE_OUTER_BOUND('',#14544,.T.) ;
#11405=FACE_OUTER_BOUND('',#14545,.T.) ;
#11406=FACE_OUTER_BOUND('',#14546,.T.) ;
#11407=FACE_OUTER_BOUND('',#14547,.T.) ;
#11408=FACE_OUTER_BOUND('',#14548,.T.) ;
#11409=FACE_OUTER_BOUND('',#14549,.T.) ;
#11410=FACE_OUTER_BOUND('',#14550,.T.) ;
#11411=FACE_OUTER_BOUND('',#14551,.T.) ;
#11412=FACE_OUTER_BOUND('',#14552,.T.) ;
#11413=FACE_OUTER_BOUND('',#14553,.T.) ;
#11414=FACE_OUTER_BOUND('',#14554,.T.) ;
#11415=FACE_OUTER_BOUND('',#14555,.T.) ;
#11416=FACE_OUTER_BOUND('',#14556,.T.) ;
#11417=FACE_OUTER_BOUND('',#14557,.T.) ;
#11418=FACE_OUTER_BOUND('',#14558,.T.) ;
#11419=FACE_OUTER_BOUND('',#14559,.T.) ;
#11420=FACE_OUTER_BOUND('',#14560,.T.) ;
#11421=FACE_OUTER_BOUND('',#14561,.T.) ;
#11422=FACE_OUTER_BOUND('',#14562,.T.) ;
#11423=FACE_OUTER_BOUND('',#14563,.T.) ;
#11424=FACE_OUTER_BOUND('',#14564,.T.) ;
#11425=FACE_OUTER_BOUND('',#14565,.T.) ;
#11426=FACE_OUTER_BOUND('',#14566,.T.) ;
#11427=FACE_OUTER_BOUND('',#14567,.T.) ;
#11428=FACE_OUTER_BOUND('',#14568,.T.) ;
#11429=FACE_OUTER_BOUND('',#14569,.T.) ;
#11430=FACE_OUTER_BOUND('',#14570,.T.) ;
#11431=FACE_OUTER_BOUND('',#14571,.T.) ;
#11432=FACE_OUTER_BOUND('',#14572,.T.) ;
#11433=FACE_OUTER_BOUND('',#14573,.T.) ;
#11434=FACE_OUTER_BOUND('',#14574,.T.) ;
#11435=FACE_OUTER_BOUND('',#14575,.T.) ;
#11436=FACE_OUTER_BOUND('',#14576,.T.) ;
#11437=FACE_OUTER_BOUND('',#14577,.T.) ;
#11438=FACE_OUTER_BOUND('',#14578,.T.) ;
#11439=FACE_OUTER_BOUND('',#14579,.T.) ;
#11440=FACE_OUTER_BOUND('',#14580,.T.) ;
#11441=FACE_OUTER_BOUND('',#14581,.T.) ;
#11442=FACE_OUTER_BOUND('',#14582,.T.) ;
#11443=FACE_OUTER_BOUND('',#14583,.T.) ;
#11444=FACE_OUTER_BOUND('',#14584,.T.) ;
#11445=FACE_OUTER_BOUND('',#14585,.T.) ;
#11446=FACE_OUTER_BOUND('',#14586,.T.) ;
#11447=FACE_OUTER_BOUND('',#14587,.T.) ;
#11448=FACE_OUTER_BOUND('',#14588,.T.) ;
#11449=FACE_OUTER_BOUND('',#14589,.T.) ;
#11450=FACE_OUTER_BOUND('',#14590,.T.) ;
#11451=FACE_OUTER_BOUND('',#14591,.T.) ;
#11452=FACE_OUTER_BOUND('',#14592,.T.) ;
#11453=FACE_OUTER_BOUND('',#14593,.T.) ;
#11454=FACE_OUTER_BOUND('',#14594,.T.) ;
#11455=FACE_OUTER_BOUND('',#14595,.T.) ;
#11456=FACE_OUTER_BOUND('',#14596,.T.) ;
#11457=FACE_OUTER_BOUND('',#14597,.T.) ;
#11458=FACE_OUTER_BOUND('',#14598,.T.) ;
#11459=FACE_OUTER_BOUND('',#14599,.T.) ;
#11460=FACE_OUTER_BOUND('',#14600,.T.) ;
#11461=FACE_OUTER_BOUND('',#14601,.T.) ;
#11462=FACE_OUTER_BOUND('',#14602,.T.) ;
#11463=FACE_OUTER_BOUND('',#14603,.T.) ;
#11464=FACE_OUTER_BOUND('',#14604,.T.) ;
#11465=FACE_OUTER_BOUND('',#14605,.T.) ;
#11466=FACE_OUTER_BOUND('',#14606,.T.) ;
#11467=FACE_OUTER_BOUND('',#14607,.T.) ;
#11468=FACE_OUTER_BOUND('',#14608,.T.) ;
#11469=FACE_OUTER_BOUND('',#14609,.T.) ;
#11470=FACE_OUTER_BOUND('',#14610,.T.) ;
#11471=FACE_OUTER_BOUND('',#14611,.T.) ;
#11472=FACE_OUTER_BOUND('',#14612,.T.) ;
#11473=FACE_OUTER_BOUND('',#14613,.T.) ;
#11474=FACE_OUTER_BOUND('',#14614,.T.) ;
#11475=FACE_OUTER_BOUND('',#14615,.T.) ;
#11476=FACE_OUTER_BOUND('',#14616,.T.) ;
#11477=FACE_OUTER_BOUND('',#14617,.T.) ;
#11478=FACE_OUTER_BOUND('',#14618,.T.) ;
#11479=FACE_OUTER_BOUND('',#14619,.T.) ;
#11480=FACE_OUTER_BOUND('',#14620,.T.) ;
#11481=FACE_OUTER_BOUND('',#14621,.T.) ;
#11482=FACE_OUTER_BOUND('',#14622,.T.) ;
#11483=FACE_OUTER_BOUND('',#14623,.T.) ;
#11484=FACE_OUTER_BOUND('',#14624,.T.) ;
#11485=FACE_OUTER_BOUND('',#14625,.T.) ;
#11486=FACE_OUTER_BOUND('',#14626,.T.) ;
#11487=FACE_OUTER_BOUND('',#14627,.T.) ;
#11488=FACE_OUTER_BOUND('',#14628,.T.) ;
#11489=FACE_OUTER_BOUND('',#14629,.T.) ;
#11490=FACE_OUTER_BOUND('',#14630,.T.) ;
#11491=FACE_OUTER_BOUND('',#14631,.T.) ;
#11492=FACE_OUTER_BOUND('',#14632,.T.) ;
#11493=FACE_OUTER_BOUND('',#14633,.T.) ;
#11494=FACE_OUTER_BOUND('',#14634,.T.) ;
#11495=FACE_OUTER_BOUND('',#14635,.T.) ;
#11496=FACE_OUTER_BOUND('',#14636,.T.) ;
#11497=FACE_OUTER_BOUND('',#14637,.T.) ;
#11498=FACE_OUTER_BOUND('',#14638,.T.) ;
#11499=FACE_OUTER_BOUND('',#14639,.T.) ;
#11500=FACE_OUTER_BOUND('',#14640,.T.) ;
#11501=FACE_OUTER_BOUND('',#14641,.T.) ;
#11502=FACE_OUTER_BOUND('',#14642,.T.) ;
#11503=FACE_OUTER_BOUND('',#14643,.T.) ;
#11504=FACE_OUTER_BOUND('',#14644,.T.) ;
#11505=FACE_OUTER_BOUND('',#14645,.T.) ;
#11506=FACE_OUTER_BOUND('',#14646,.T.) ;
#11507=FACE_OUTER_BOUND('',#14647,.T.) ;
#11508=FACE_OUTER_BOUND('',#14648,.T.) ;
#11509=FACE_OUTER_BOUND('',#14649,.T.) ;
#11510=FACE_OUTER_BOUND('',#14650,.T.) ;
#11511=FACE_OUTER_BOUND('',#14651,.T.) ;
#11512=FACE_OUTER_BOUND('',#14652,.T.) ;
#11513=FACE_OUTER_BOUND('',#14653,.T.) ;
#11514=FACE_OUTER_BOUND('',#14654,.T.) ;
#11515=FACE_OUTER_BOUND('',#14655,.T.) ;
#11516=FACE_OUTER_BOUND('',#14656,.T.) ;
#11517=FACE_OUTER_BOUND('',#14657,.T.) ;
#11518=FACE_OUTER_BOUND('',#14658,.T.) ;
#11519=FACE_OUTER_BOUND('',#14659,.T.) ;
#11520=FACE_OUTER_BOUND('',#14660,.T.) ;
#11521=FACE_OUTER_BOUND('',#14661,.T.) ;
#11522=FACE_OUTER_BOUND('',#14662,.T.) ;
#11523=FACE_OUTER_BOUND('',#14663,.T.) ;
#11524=FACE_OUTER_BOUND('',#14664,.T.) ;
#11525=FACE_OUTER_BOUND('',#14665,.T.) ;
#11526=FACE_OUTER_BOUND('',#14666,.T.) ;
#11527=FACE_OUTER_BOUND('',#14667,.T.) ;
#11528=FACE_OUTER_BOUND('',#14668,.T.) ;
#11529=FACE_OUTER_BOUND('',#14669,.T.) ;
#11530=FACE_OUTER_BOUND('',#14670,.T.) ;
#11531=FACE_OUTER_BOUND('',#14671,.T.) ;
#11532=FACE_OUTER_BOUND('',#14672,.T.) ;
#11533=FACE_OUTER_BOUND('',#14673,.T.) ;
#11534=FACE_OUTER_BOUND('',#14674,.T.) ;
#11535=FACE_OUTER_BOUND('',#14675,.T.) ;
#11536=FACE_OUTER_BOUND('',#14676,.T.) ;
#11537=FACE_OUTER_BOUND('',#14677,.T.) ;
#11538=FACE_OUTER_BOUND('',#14678,.T.) ;
#11539=FACE_OUTER_BOUND('',#14679,.T.) ;
#11540=FACE_OUTER_BOUND('',#14680,.T.) ;
#11541=FACE_OUTER_BOUND('',#14681,.T.) ;
#11542=FACE_OUTER_BOUND('',#14682,.T.) ;
#11543=FACE_OUTER_BOUND('',#14683,.T.) ;
#11544=FACE_OUTER_BOUND('',#14684,.T.) ;
#11545=FACE_OUTER_BOUND('',#14685,.T.) ;
#11546=FACE_OUTER_BOUND('',#14686,.T.) ;
#11547=FACE_OUTER_BOUND('',#14687,.T.) ;
#11548=FACE_OUTER_BOUND('',#14688,.T.) ;
#11549=FACE_OUTER_BOUND('',#14689,.T.) ;
#11550=FACE_OUTER_BOUND('',#14690,.T.) ;
#11551=FACE_OUTER_BOUND('',#14691,.T.) ;
#11552=FACE_OUTER_BOUND('',#14692,.T.) ;
#11553=FACE_OUTER_BOUND('',#14693,.T.) ;
#11554=FACE_OUTER_BOUND('',#14694,.T.) ;
#11555=FACE_OUTER_BOUND('',#14695,.T.) ;
#11556=FACE_OUTER_BOUND('',#14696,.T.) ;
#11557=FACE_OUTER_BOUND('',#14697,.T.) ;
#11558=FACE_OUTER_BOUND('',#14698,.T.) ;
#11559=FACE_OUTER_BOUND('',#14699,.T.) ;
#11560=FACE_OUTER_BOUND('',#14700,.T.) ;
#11561=FACE_OUTER_BOUND('',#14701,.T.) ;
#11562=FACE_OUTER_BOUND('',#14702,.T.) ;
#11563=FACE_OUTER_BOUND('',#14703,.T.) ;
#11564=FACE_OUTER_BOUND('',#14704,.T.) ;
#11565=FACE_OUTER_BOUND('',#14705,.T.) ;
#11566=FACE_OUTER_BOUND('',#14706,.T.) ;
#11567=FACE_OUTER_BOUND('',#14707,.T.) ;
#11568=FACE_OUTER_BOUND('',#14708,.T.) ;
#11569=FACE_OUTER_BOUND('',#14709,.T.) ;
#11570=FACE_OUTER_BOUND('',#14710,.T.) ;
#11571=FACE_OUTER_BOUND('',#14711,.T.) ;
#11572=FACE_OUTER_BOUND('',#14712,.T.) ;
#11573=FACE_OUTER_BOUND('',#14713,.T.) ;
#11574=FACE_OUTER_BOUND('',#14714,.T.) ;
#11575=FACE_OUTER_BOUND('',#14715,.T.) ;
#11576=FACE_OUTER_BOUND('',#14716,.T.) ;
#11577=FACE_OUTER_BOUND('',#14717,.T.) ;
#11578=FACE_OUTER_BOUND('',#14718,.T.) ;
#11579=FACE_OUTER_BOUND('',#14719,.T.) ;
#11580=FACE_OUTER_BOUND('',#14720,.T.) ;
#11581=FACE_OUTER_BOUND('',#14721,.T.) ;
#11582=FACE_OUTER_BOUND('',#14722,.T.) ;
#11583=FACE_OUTER_BOUND('',#14723,.T.) ;
#11584=FACE_OUTER_BOUND('',#14724,.T.) ;
#11585=FACE_OUTER_BOUND('',#14725,.T.) ;
#11586=FACE_OUTER_BOUND('',#14726,.T.) ;
#11587=FACE_OUTER_BOUND('',#14727,.T.) ;
#11588=FACE_OUTER_BOUND('',#14728,.T.) ;
#11589=FACE_OUTER_BOUND('',#14729,.T.) ;
#11590=FACE_OUTER_BOUND('',#14730,.T.) ;
#11591=FACE_OUTER_BOUND('',#14731,.T.) ;
#11592=FACE_OUTER_BOUND('',#14732,.T.) ;
#11593=FACE_OUTER_BOUND('',#14733,.T.) ;
#11594=FACE_OUTER_BOUND('',#14734,.T.) ;
#11595=FACE_OUTER_BOUND('',#14735,.T.) ;
#11596=FACE_OUTER_BOUND('',#14736,.T.) ;
#11597=FACE_OUTER_BOUND('',#14737,.T.) ;
#11598=FACE_OUTER_BOUND('',#14738,.T.) ;
#11599=FACE_OUTER_BOUND('',#14739,.T.) ;
#11600=FACE_OUTER_BOUND('',#14740,.T.) ;
#11601=FACE_OUTER_BOUND('',#14741,.T.) ;
#11602=FACE_OUTER_BOUND('',#14742,.T.) ;
#11603=FACE_OUTER_BOUND('',#14743,.T.) ;
#11604=FACE_OUTER_BOUND('',#14744,.T.) ;
#11605=FACE_OUTER_BOUND('',#14745,.T.) ;
#11606=FACE_OUTER_BOUND('',#14746,.T.) ;
#11607=FACE_OUTER_BOUND('',#14747,.T.) ;
#11608=FACE_OUTER_BOUND('',#14748,.T.) ;
#11609=FACE_OUTER_BOUND('',#14749,.T.) ;
#11610=FACE_OUTER_BOUND('',#14750,.T.) ;
#11611=FACE_OUTER_BOUND('',#14751,.T.) ;
#11612=FACE_OUTER_BOUND('',#14752,.T.) ;
#11613=FACE_OUTER_BOUND('',#14753,.T.) ;
#11614=FACE_OUTER_BOUND('',#14754,.T.) ;
#11615=FACE_OUTER_BOUND('',#14755,.T.) ;
#11616=FACE_OUTER_BOUND('',#14756,.T.) ;
#11617=FACE_OUTER_BOUND('',#14757,.T.) ;
#11618=FACE_OUTER_BOUND('',#14758,.T.) ;
#11619=FACE_OUTER_BOUND('',#14759,.T.) ;
#11620=FACE_OUTER_BOUND('',#14760,.T.) ;
#11621=FACE_OUTER_BOUND('',#14761,.T.) ;
#11622=FACE_OUTER_BOUND('',#14762,.T.) ;
#11623=FACE_OUTER_BOUND('',#14763,.T.) ;
#11624=FACE_OUTER_BOUND('',#14764,.T.) ;
#11625=FACE_OUTER_BOUND('',#14765,.T.) ;
#11626=FACE_OUTER_BOUND('',#14766,.T.) ;
#11627=FACE_OUTER_BOUND('',#14767,.T.) ;
#11628=FACE_OUTER_BOUND('',#14768,.T.) ;
#11629=FACE_OUTER_BOUND('',#14769,.T.) ;
#11630=FACE_OUTER_BOUND('',#14770,.T.) ;
#11631=FACE_OUTER_BOUND('',#14771,.T.) ;
#11632=FACE_OUTER_BOUND('',#14772,.T.) ;
#11633=FACE_OUTER_BOUND('',#14773,.T.) ;
#11634=FACE_OUTER_BOUND('',#14774,.T.) ;
#11635=FACE_OUTER_BOUND('',#14775,.T.) ;
#11636=FACE_OUTER_BOUND('',#14776,.T.) ;
#11637=FACE_OUTER_BOUND('',#14777,.T.) ;
#11638=FACE_OUTER_BOUND('',#14778,.T.) ;
#11639=FACE_OUTER_BOUND('',#14779,.T.) ;
#11640=FACE_OUTER_BOUND('',#14780,.T.) ;
#11641=FACE_OUTER_BOUND('',#14781,.T.) ;
#11642=FACE_OUTER_BOUND('',#14782,.T.) ;
#11643=FACE_OUTER_BOUND('',#14783,.T.) ;
#11644=FACE_OUTER_BOUND('',#14784,.T.) ;
#11645=FACE_OUTER_BOUND('',#14785,.T.) ;
#11646=FACE_OUTER_BOUND('',#14786,.T.) ;
#11647=FACE_OUTER_BOUND('',#14787,.T.) ;
#11648=FACE_OUTER_BOUND('',#14788,.T.) ;
#11649=FACE_OUTER_BOUND('',#14789,.T.) ;
#11650=FACE_OUTER_BOUND('',#14790,.T.) ;
#11651=FACE_OUTER_BOUND('',#14791,.T.) ;
#11652=FACE_OUTER_BOUND('',#14792,.T.) ;
#11653=FACE_OUTER_BOUND('',#14793,.T.) ;
#11654=FACE_OUTER_BOUND('',#14794,.T.) ;
#11655=FACE_OUTER_BOUND('',#14795,.T.) ;
#11656=FACE_OUTER_BOUND('',#14796,.T.) ;
#11657=FACE_OUTER_BOUND('',#14797,.T.) ;
#11658=FACE_OUTER_BOUND('',#14798,.T.) ;
#11659=FACE_OUTER_BOUND('',#14799,.T.) ;
#11660=FACE_OUTER_BOUND('',#14800,.T.) ;
#11661=FACE_OUTER_BOUND('',#14801,.T.) ;
#11662=FACE_OUTER_BOUND('',#14802,.T.) ;
#11663=FACE_OUTER_BOUND('',#14803,.T.) ;
#11664=FACE_OUTER_BOUND('',#14804,.T.) ;
#11665=FACE_OUTER_BOUND('',#14805,.T.) ;
#11666=FACE_OUTER_BOUND('',#14806,.T.) ;
#11667=FACE_OUTER_BOUND('',#14807,.T.) ;
#11668=FACE_OUTER_BOUND('',#14808,.T.) ;
#11669=FACE_OUTER_BOUND('',#14809,.T.) ;
#11670=FACE_OUTER_BOUND('',#14810,.T.) ;
#11671=FACE_OUTER_BOUND('',#14811,.T.) ;
#11672=FACE_OUTER_BOUND('',#14812,.T.) ;
#11673=FACE_OUTER_BOUND('',#14813,.T.) ;
#11674=FACE_OUTER_BOUND('',#14814,.T.) ;
#11675=FACE_OUTER_BOUND('',#14815,.T.) ;
#11676=FACE_OUTER_BOUND('',#14816,.T.) ;
#11677=FACE_OUTER_BOUND('',#14817,.T.) ;
#11678=FACE_OUTER_BOUND('',#14818,.T.) ;
#11679=FACE_OUTER_BOUND('',#14819,.T.) ;
#11680=FACE_OUTER_BOUND('',#14820,.T.) ;
#11681=FACE_OUTER_BOUND('',#14821,.T.) ;
#11682=FACE_OUTER_BOUND('',#14822,.T.) ;
#11683=FACE_OUTER_BOUND('',#14823,.T.) ;
#11684=FACE_OUTER_BOUND('',#14824,.T.) ;
#11685=FACE_OUTER_BOUND('',#14825,.T.) ;
#11686=FACE_OUTER_BOUND('',#14826,.T.) ;
#11687=FACE_OUTER_BOUND('',#14827,.T.) ;
#11688=FACE_OUTER_BOUND('',#14828,.T.) ;
#11689=FACE_OUTER_BOUND('',#14829,.T.) ;
#11690=FACE_OUTER_BOUND('',#14830,.T.) ;
#11691=FACE_OUTER_BOUND('',#14831,.T.) ;
#11692=FACE_OUTER_BOUND('',#14832,.T.) ;
#11693=FACE_OUTER_BOUND('',#14833,.T.) ;
#11694=FACE_OUTER_BOUND('',#14834,.T.) ;
#11695=FACE_OUTER_BOUND('',#14835,.T.) ;
#11696=FACE_OUTER_BOUND('',#14836,.T.) ;
#11697=FACE_OUTER_BOUND('',#14837,.T.) ;
#11698=FACE_OUTER_BOUND('',#14838,.T.) ;
#11699=FACE_OUTER_BOUND('',#14839,.T.) ;
#11700=FACE_OUTER_BOUND('',#14840,.T.) ;
#11701=FACE_OUTER_BOUND('',#14841,.T.) ;
#11702=FACE_OUTER_BOUND('',#14842,.T.) ;
#11703=FACE_OUTER_BOUND('',#14843,.T.) ;
#11704=FACE_OUTER_BOUND('',#14844,.T.) ;
#11705=FACE_OUTER_BOUND('',#14845,.T.) ;
#11706=FACE_OUTER_BOUND('',#14846,.T.) ;
#11707=FACE_OUTER_BOUND('',#14847,.T.) ;
#11708=FACE_OUTER_BOUND('',#14848,.T.) ;
#11709=FACE_OUTER_BOUND('',#14849,.T.) ;
#11710=FACE_OUTER_BOUND('',#14850,.T.) ;
#11711=FACE_OUTER_BOUND('',#14851,.T.) ;
#11712=FACE_OUTER_BOUND('',#14852,.T.) ;
#11713=FACE_OUTER_BOUND('',#14853,.T.) ;
#11714=FACE_OUTER_BOUND('',#14854,.T.) ;
#11715=FACE_OUTER_BOUND('',#14855,.T.) ;
#11716=FACE_OUTER_BOUND('',#14856,.T.) ;
#11717=FACE_OUTER_BOUND('',#14857,.T.) ;
#11718=FACE_OUTER_BOUND('',#14858,.T.) ;
#11719=FACE_OUTER_BOUND('',#14859,.T.) ;
#11720=FACE_OUTER_BOUND('',#14860,.T.) ;
#11721=FACE_OUTER_BOUND('',#14861,.T.) ;
#11722=FACE_OUTER_BOUND('',#14862,.T.) ;
#11723=FACE_OUTER_BOUND('',#14863,.T.) ;
#11724=FACE_OUTER_BOUND('',#14864,.T.) ;
#11725=FACE_OUTER_BOUND('',#14865,.T.) ;
#11726=FACE_OUTER_BOUND('',#14866,.T.) ;
#11727=FACE_OUTER_BOUND('',#14867,.T.) ;
#11728=FACE_OUTER_BOUND('',#14868,.T.) ;
#11729=FACE_OUTER_BOUND('',#14869,.T.) ;
#11730=FACE_OUTER_BOUND('',#14870,.T.) ;
#11731=FACE_OUTER_BOUND('',#14871,.T.) ;
#11732=FACE_OUTER_BOUND('',#14872,.T.) ;
#11733=FACE_OUTER_BOUND('',#14873,.T.) ;
#11734=FACE_OUTER_BOUND('',#14874,.T.) ;
#11735=FACE_OUTER_BOUND('',#14875,.T.) ;
#11736=FACE_OUTER_BOUND('',#14876,.T.) ;
#11737=FACE_OUTER_BOUND('',#14877,.T.) ;
#11738=FACE_OUTER_BOUND('',#14878,.T.) ;
#11739=FACE_OUTER_BOUND('',#14879,.T.) ;
#11740=FACE_OUTER_BOUND('',#14880,.T.) ;
#11741=FACE_OUTER_BOUND('',#14881,.T.) ;
#11742=FACE_OUTER_BOUND('',#14882,.T.) ;
#11743=FACE_OUTER_BOUND('',#14883,.T.) ;
#11744=FACE_OUTER_BOUND('',#14884,.T.) ;
#11745=FACE_OUTER_BOUND('',#14885,.T.) ;
#11746=FACE_OUTER_BOUND('',#14886,.T.) ;
#11747=FACE_OUTER_BOUND('',#14887,.T.) ;
#11748=FACE_OUTER_BOUND('',#14888,.T.) ;
#11749=FACE_OUTER_BOUND('',#14889,.T.) ;
#11750=FACE_OUTER_BOUND('',#14890,.T.) ;
#11751=FACE_OUTER_BOUND('',#14891,.T.) ;
#11752=FACE_OUTER_BOUND('',#14892,.T.) ;
#11753=FACE_OUTER_BOUND('',#14893,.T.) ;
#11754=FACE_OUTER_BOUND('',#14894,.T.) ;
#11755=FACE_OUTER_BOUND('',#14895,.T.) ;
#11756=FACE_OUTER_BOUND('',#14896,.T.) ;
#11757=FACE_OUTER_BOUND('',#14897,.T.) ;
#11758=FACE_OUTER_BOUND('',#14898,.T.) ;
#11759=FACE_OUTER_BOUND('',#14899,.T.) ;
#11760=FACE_OUTER_BOUND('',#14900,.T.) ;
#11761=FACE_OUTER_BOUND('',#14901,.T.) ;
#11762=FACE_OUTER_BOUND('',#14902,.T.) ;
#11763=FACE_OUTER_BOUND('',#14903,.T.) ;
#11764=FACE_OUTER_BOUND('',#14904,.T.) ;
#11765=FACE_OUTER_BOUND('',#14905,.T.) ;
#11766=FACE_OUTER_BOUND('',#14906,.T.) ;
#11767=FACE_OUTER_BOUND('',#14907,.T.) ;
#11768=FACE_OUTER_BOUND('',#14908,.T.) ;
#11769=FACE_OUTER_BOUND('',#14909,.T.) ;
#11770=FACE_OUTER_BOUND('',#14910,.T.) ;
#11771=FACE_OUTER_BOUND('',#14911,.T.) ;
#11772=FACE_OUTER_BOUND('',#14912,.T.) ;
#11773=FACE_OUTER_BOUND('',#14913,.T.) ;
#11774=FACE_OUTER_BOUND('',#14914,.T.) ;
#11775=FACE_OUTER_BOUND('',#14915,.T.) ;
#11776=FACE_OUTER_BOUND('',#14916,.T.) ;
#11777=FACE_OUTER_BOUND('',#14917,.T.) ;
#11778=FACE_OUTER_BOUND('',#14918,.T.) ;
#11779=FACE_OUTER_BOUND('',#14919,.T.) ;
#11780=FACE_OUTER_BOUND('',#14920,.T.) ;
#11781=FACE_OUTER_BOUND('',#14921,.T.) ;
#11782=FACE_OUTER_BOUND('',#14922,.T.) ;
#11783=FACE_OUTER_BOUND('',#14923,.T.) ;
#11784=FACE_OUTER_BOUND('',#14924,.T.) ;
#11785=FACE_OUTER_BOUND('',#14925,.T.) ;
#11786=FACE_OUTER_BOUND('',#14926,.T.) ;
#11787=FACE_OUTER_BOUND('',#14927,.T.) ;
#11788=FACE_OUTER_BOUND('',#14928,.T.) ;
#11789=FACE_OUTER_BOUND('',#14929,.T.) ;
#11790=FACE_OUTER_BOUND('',#14930,.T.) ;
#11791=FACE_OUTER_BOUND('',#14931,.T.) ;
#11792=FACE_OUTER_BOUND('',#14932,.T.) ;
#11793=FACE_OUTER_BOUND('',#14933,.T.) ;
#11794=FACE_OUTER_BOUND('',#14934,.T.) ;
#11795=FACE_OUTER_BOUND('',#14935,.T.) ;
#11796=FACE_OUTER_BOUND('',#14936,.T.) ;
#11797=FACE_OUTER_BOUND('',#14937,.T.) ;
#11798=FACE_OUTER_BOUND('',#14938,.T.) ;
#11799=FACE_OUTER_BOUND('',#14939,.T.) ;
#11800=FACE_OUTER_BOUND('',#14940,.T.) ;
#11801=FACE_OUTER_BOUND('',#14941,.T.) ;
#11802=FACE_OUTER_BOUND('',#14942,.T.) ;
#11803=FACE_OUTER_BOUND('',#14943,.T.) ;
#11804=FACE_OUTER_BOUND('',#14944,.T.) ;
#11805=FACE_OUTER_BOUND('',#14945,.T.) ;
#11806=FACE_OUTER_BOUND('',#14946,.T.) ;
#11807=FACE_OUTER_BOUND('',#14947,.T.) ;
#11808=FACE_OUTER_BOUND('',#14948,.T.) ;
#11809=FACE_OUTER_BOUND('',#14949,.T.) ;
#11810=FACE_OUTER_BOUND('',#14950,.T.) ;
#11811=FACE_OUTER_BOUND('',#14951,.T.) ;
#11812=FACE_OUTER_BOUND('',#14952,.T.) ;
#11813=FACE_OUTER_BOUND('',#14953,.T.) ;
#11814=FACE_OUTER_BOUND('',#14954,.T.) ;
#11815=FACE_OUTER_BOUND('',#14955,.T.) ;
#11816=FACE_OUTER_BOUND('',#14956,.T.) ;
#11817=FACE_OUTER_BOUND('',#14957,.T.) ;
#11818=FACE_OUTER_BOUND('',#14958,.T.) ;
#11819=FACE_OUTER_BOUND('',#14959,.T.) ;
#11820=FACE_OUTER_BOUND('',#14960,.T.) ;
#11821=FACE_OUTER_BOUND('',#14961,.T.) ;
#11822=FACE_OUTER_BOUND('',#14962,.T.) ;
#11823=FACE_OUTER_BOUND('',#14963,.T.) ;
#11824=FACE_OUTER_BOUND('',#14964,.T.) ;
#11825=FACE_OUTER_BOUND('',#14965,.T.) ;
#11826=FACE_OUTER_BOUND('',#14966,.T.) ;
#11827=FACE_OUTER_BOUND('',#14967,.T.) ;
#11828=FACE_OUTER_BOUND('',#14968,.T.) ;
#11829=FACE_OUTER_BOUND('',#14969,.T.) ;
#11830=FACE_OUTER_BOUND('',#14970,.T.) ;
#11831=FACE_OUTER_BOUND('',#14971,.T.) ;
#11832=FACE_OUTER_BOUND('',#14972,.T.) ;
#11833=FACE_OUTER_BOUND('',#14973,.T.) ;
#11834=FACE_OUTER_BOUND('',#14974,.T.) ;
#11835=FACE_OUTER_BOUND('',#14975,.T.) ;
#11836=FACE_OUTER_BOUND('',#14976,.T.) ;
#11837=FACE_OUTER_BOUND('',#14977,.T.) ;
#11838=FACE_OUTER_BOUND('',#14978,.T.) ;
#11839=FACE_OUTER_BOUND('',#14979,.T.) ;
#11840=FACE_OUTER_BOUND('',#14980,.T.) ;
#11841=FACE_OUTER_BOUND('',#14981,.T.) ;
#11842=FACE_OUTER_BOUND('',#14982,.T.) ;
#11843=FACE_OUTER_BOUND('',#14983,.T.) ;
#11844=FACE_OUTER_BOUND('',#14984,.T.) ;
#11845=FACE_OUTER_BOUND('',#14985,.T.) ;
#11846=FACE_OUTER_BOUND('',#14986,.T.) ;
#11847=FACE_OUTER_BOUND('',#14987,.T.) ;
#11848=FACE_OUTER_BOUND('',#14988,.T.) ;
#11849=FACE_OUTER_BOUND('',#14989,.T.) ;
#11850=FACE_OUTER_BOUND('',#14990,.T.) ;
#11851=FACE_OUTER_BOUND('',#14991,.T.) ;
#11852=FACE_OUTER_BOUND('',#14992,.T.) ;
#11853=FACE_OUTER_BOUND('',#14993,.T.) ;
#11854=FACE_OUTER_BOUND('',#14994,.T.) ;
#11855=FACE_OUTER_BOUND('',#14995,.T.) ;
#11856=FACE_OUTER_BOUND('',#14996,.T.) ;
#11857=FACE_OUTER_BOUND('',#14997,.T.) ;
#11858=FACE_OUTER_BOUND('',#14998,.T.) ;
#11859=FACE_OUTER_BOUND('',#14999,.T.) ;
#11860=FACE_OUTER_BOUND('',#15000,.T.) ;
#11861=FACE_OUTER_BOUND('',#15001,.T.) ;
#11862=FACE_OUTER_BOUND('',#15002,.T.) ;
#11863=FACE_OUTER_BOUND('',#15003,.T.) ;
#11864=FACE_OUTER_BOUND('',#15004,.T.) ;
#11865=FACE_OUTER_BOUND('',#15005,.T.) ;
#11866=FACE_OUTER_BOUND('',#15006,.T.) ;
#11867=FACE_OUTER_BOUND('',#15007,.T.) ;
#11868=FACE_OUTER_BOUND('',#15008,.T.) ;
#11869=FACE_OUTER_BOUND('',#15009,.T.) ;
#11870=FACE_OUTER_BOUND('',#15010,.T.) ;
#11871=FACE_OUTER_BOUND('',#15011,.T.) ;
#11872=FACE_OUTER_BOUND('',#15012,.T.) ;
#11873=FACE_OUTER_BOUND('',#15013,.T.) ;
#11874=FACE_OUTER_BOUND('',#15014,.T.) ;
#11875=FACE_OUTER_BOUND('',#15015,.T.) ;
#11876=FACE_OUTER_BOUND('',#15016,.T.) ;
#11877=FACE_OUTER_BOUND('',#15018,.T.) ;
#11878=FACE_OUTER_BOUND('',#15019,.T.) ;
#11879=FACE_OUTER_BOUND('',#15020,.T.) ;
#11880=FACE_OUTER_BOUND('',#15021,.T.) ;
#11881=FACE_OUTER_BOUND('',#15022,.T.) ;
#11882=FACE_OUTER_BOUND('',#15023,.T.) ;
#11883=FACE_OUTER_BOUND('',#15024,.T.) ;
#11884=FACE_OUTER_BOUND('',#15026,.T.) ;
#11885=FACE_OUTER_BOUND('',#15027,.T.) ;
#11886=FACE_OUTER_BOUND('',#15028,.T.) ;
#11887=FACE_OUTER_BOUND('',#15029,.T.) ;
#11888=FACE_OUTER_BOUND('',#15030,.T.) ;
#11889=FACE_OUTER_BOUND('',#15031,.T.) ;
#11890=FACE_OUTER_BOUND('',#15033,.T.) ;
#11891=FACE_OUTER_BOUND('',#15034,.T.) ;
#11892=FACE_OUTER_BOUND('',#15035,.T.) ;
#11893=FACE_OUTER_BOUND('',#15036,.T.) ;
#11894=FACE_OUTER_BOUND('',#15037,.T.) ;
#11895=FACE_OUTER_BOUND('',#15039,.T.) ;
#11896=FACE_OUTER_BOUND('',#15040,.T.) ;
#11897=FACE_OUTER_BOUND('',#15041,.T.) ;
#11898=FACE_OUTER_BOUND('',#15042,.T.) ;
#11899=FACE_OUTER_BOUND('',#15043,.T.) ;
#11900=FACE_OUTER_BOUND('',#15044,.T.) ;
#11901=FACE_OUTER_BOUND('',#15045,.T.) ;
#11902=FACE_OUTER_BOUND('',#15046,.T.) ;
#11903=FACE_OUTER_BOUND('',#15047,.T.) ;
#11904=FACE_OUTER_BOUND('',#15048,.T.) ;
#11905=FACE_OUTER_BOUND('',#15049,.T.) ;
#11906=FACE_OUTER_BOUND('',#15050,.T.) ;
#11907=FACE_OUTER_BOUND('',#15051,.T.) ;
#11908=FACE_OUTER_BOUND('',#15052,.T.) ;
#11909=FACE_OUTER_BOUND('',#15053,.T.) ;
#11910=FACE_OUTER_BOUND('',#15054,.T.) ;
#11911=FACE_OUTER_BOUND('',#15055,.T.) ;
#11912=FACE_OUTER_BOUND('',#15056,.T.) ;
#11913=FACE_OUTER_BOUND('',#15057,.T.) ;
#11914=FACE_OUTER_BOUND('',#15058,.T.) ;
#11915=FACE_OUTER_BOUND('',#15059,.T.) ;
#11916=FACE_OUTER_BOUND('',#15060,.T.) ;
#11917=FACE_OUTER_BOUND('',#15061,.T.) ;
#11918=FACE_OUTER_BOUND('',#15062,.T.) ;
#11919=FACE_OUTER_BOUND('',#15063,.T.) ;
#11920=FACE_OUTER_BOUND('',#15064,.T.) ;
#11921=FACE_OUTER_BOUND('',#15065,.T.) ;
#11922=FACE_OUTER_BOUND('',#15066,.T.) ;
#11923=FACE_OUTER_BOUND('',#15067,.T.) ;
#11924=FACE_OUTER_BOUND('',#15068,.T.) ;
#11925=FACE_OUTER_BOUND('',#15069,.T.) ;
#11926=FACE_OUTER_BOUND('',#15070,.T.) ;
#11927=FACE_OUTER_BOUND('',#15071,.T.) ;
#11928=FACE_OUTER_BOUND('',#15072,.T.) ;
#11929=FACE_OUTER_BOUND('',#15073,.T.) ;
#11930=FACE_OUTER_BOUND('',#15074,.T.) ;
#11931=FACE_OUTER_BOUND('',#15075,.T.) ;
#11932=FACE_OUTER_BOUND('',#15076,.T.) ;
#11933=FACE_OUTER_BOUND('',#15077,.T.) ;
#11934=FACE_OUTER_BOUND('',#15078,.T.) ;
#11935=FACE_OUTER_BOUND('',#15079,.T.) ;
#11936=FACE_OUTER_BOUND('',#15080,.T.) ;
#11937=FACE_OUTER_BOUND('',#15081,.T.) ;
#11938=FACE_OUTER_BOUND('',#15082,.T.) ;
#11939=FACE_OUTER_BOUND('',#15083,.T.) ;
#11940=FACE_OUTER_BOUND('',#15084,.T.) ;
#11941=FACE_OUTER_BOUND('',#15085,.T.) ;
#11942=FACE_OUTER_BOUND('',#15086,.T.) ;
#11943=FACE_OUTER_BOUND('',#15087,.T.) ;
#11944=FACE_OUTER_BOUND('',#15088,.T.) ;
#11945=FACE_OUTER_BOUND('',#15089,.T.) ;
#11946=FACE_OUTER_BOUND('',#15090,.T.) ;
#11947=FACE_OUTER_BOUND('',#15091,.T.) ;
#11948=FACE_OUTER_BOUND('',#15092,.T.) ;
#11949=FACE_OUTER_BOUND('',#15093,.T.) ;
#11950=FACE_OUTER_BOUND('',#15094,.T.) ;
#11951=FACE_OUTER_BOUND('',#15095,.T.) ;
#11952=FACE_OUTER_BOUND('',#15096,.T.) ;
#11953=FACE_OUTER_BOUND('',#15097,.T.) ;
#11954=FACE_OUTER_BOUND('',#15098,.T.) ;
#11955=FACE_OUTER_BOUND('',#15099,.T.) ;
#11956=FACE_OUTER_BOUND('',#15100,.T.) ;
#11957=FACE_OUTER_BOUND('',#15101,.T.) ;
#11958=FACE_OUTER_BOUND('',#15102,.T.) ;
#11959=FACE_OUTER_BOUND('',#15103,.T.) ;
#11960=FACE_OUTER_BOUND('',#15104,.T.) ;
#14309=EDGE_LOOP('',(#33100,#33101,#33102,#33103)) ;
#14310=EDGE_LOOP('',(#33104,#33105,#33106,#33107)) ;
#14311=EDGE_LOOP('',(#33108,#33109,#33110,#33111)) ;
#14312=EDGE_LOOP('',(#33112,#33113,#33114,#33115)) ;
#14313=EDGE_LOOP('',(#33116,#33117,#33118,#33119)) ;
#14314=EDGE_LOOP('',(#33120,#33121,#33122,#33123)) ;
#14315=EDGE_LOOP('',(#33124,#33125,#33126,#33127)) ;
#14316=EDGE_LOOP('',(#33128,#33129,#33130,#33131)) ;
#14317=EDGE_LOOP('',(#33132,#33133,#33134,#33135)) ;
#14318=EDGE_LOOP('',(#33136,#33137,#33138,#33139)) ;
#14319=EDGE_LOOP('',(#33140,#33141,#33142,#33143)) ;
#14320=EDGE_LOOP('',(#33144,#33145,#33146,#33147)) ;
#14321=EDGE_LOOP('',(#33148,#33149,#33150,#33151,#33152,#33153,#33154,#33155,
#33156,#33157,#33158,#33159,#33160,#33161,#33162,#33163,#33164,#33165,#33166)) ;
#14322=EDGE_LOOP('',(#33167,#33168,#33169,#33170,#33171,#33172,#33173,#33174)) ;
#14323=EDGE_LOOP('',(#33175,#33176,#33177,#33178)) ;
#14324=EDGE_LOOP('',(#33179,#33180,#33181,#33182)) ;
#14325=EDGE_LOOP('',(#33183,#33184,#33185,#33186)) ;
#14326=EDGE_LOOP('',(#33187,#33188,#33189,#33190)) ;
#14327=EDGE_LOOP('',(#33191,#33192,#33193,#33194)) ;
#14328=EDGE_LOOP('',(#33195,#33196,#33197,#33198)) ;
#14329=EDGE_LOOP('',(#33199,#33200,#33201,#33202)) ;
#14330=EDGE_LOOP('',(#33203,#33204,#33205,#33206)) ;
#14331=EDGE_LOOP('',(#33207,#33208,#33209,#33210)) ;
#14332=EDGE_LOOP('',(#33211,#33212,#33213,#33214)) ;
#14333=EDGE_LOOP('',(#33215,#33216,#33217,#33218)) ;
#14334=EDGE_LOOP('',(#33219,#33220,#33221,#33222)) ;
#14335=EDGE_LOOP('',(#33223,#33224,#33225,#33226)) ;
#14336=EDGE_LOOP('',(#33227,#33228,#33229,#33230)) ;
#14337=EDGE_LOOP('',(#33231,#33232,#33233,#33234)) ;
#14338=EDGE_LOOP('',(#33235,#33236,#33237,#33238)) ;
#14339=EDGE_LOOP('',(#33239,#33240,#33241,#33242)) ;
#14340=EDGE_LOOP('',(#33243,#33244,#33245,#33246)) ;
#14341=EDGE_LOOP('',(#33247,#33248,#33249,#33250)) ;
#14342=EDGE_LOOP('',(#33251,#33252,#33253,#33254)) ;
#14343=EDGE_LOOP('',(#33255,#33256,#33257,#33258)) ;
#14344=EDGE_LOOP('',(#33259,#33260,#33261,#33262)) ;
#14345=EDGE_LOOP('',(#33263,#33264,#33265,#33266)) ;
#14346=EDGE_LOOP('',(#33267,#33268,#33269,#33270)) ;
#14347=EDGE_LOOP('',(#33271,#33272,#33273,#33274)) ;
#14348=EDGE_LOOP('',(#33275,#33276,#33277,#33278)) ;
#14349=EDGE_LOOP('',(#33279,#33280,#33281,#33282)) ;
#14350=EDGE_LOOP('',(#33283,#33284,#33285,#33286)) ;
#14351=EDGE_LOOP('',(#33287,#33288,#33289,#33290)) ;
#14352=EDGE_LOOP('',(#33291,#33292,#33293,#33294)) ;
#14353=EDGE_LOOP('',(#33295,#33296,#33297,#33298)) ;
#14354=EDGE_LOOP('',(#33299,#33300,#33301,#33302)) ;
#14355=EDGE_LOOP('',(#33303,#33304,#33305,#33306)) ;
#14356=EDGE_LOOP('',(#33307,#33308,#33309,#33310)) ;
#14357=EDGE_LOOP('',(#33311,#33312,#33313,#33314)) ;
#14358=EDGE_LOOP('',(#33315,#33316,#33317,#33318)) ;
#14359=EDGE_LOOP('',(#33319,#33320,#33321,#33322)) ;
#14360=EDGE_LOOP('',(#33323,#33324,#33325,#33326,#33327,#33328,#33329,#33330)) ;
#14361=EDGE_LOOP('',(#33331,#33332,#33333,#33334)) ;
#14362=EDGE_LOOP('',(#33335,#33336,#33337,#33338)) ;
#14363=EDGE_LOOP('',(#33339,#33340,#33341,#33342)) ;
#14364=EDGE_LOOP('',(#33343,#33344,#33345,#33346)) ;
#14365=EDGE_LOOP('',(#33347,#33348,#33349,#33350)) ;
#14366=EDGE_LOOP('',(#33351,#33352,#33353)) ;
#14367=EDGE_LOOP('',(#33354,#33355,#33356,#33357)) ;
#14368=EDGE_LOOP('',(#33358,#33359,#33360,#33361)) ;
#14369=EDGE_LOOP('',(#33362,#33363,#33364,#33365)) ;
#14370=EDGE_LOOP('',(#33366,#33367,#33368,#33369)) ;
#14371=EDGE_LOOP('',(#33370,#33371,#33372,#33373)) ;
#14372=EDGE_LOOP('',(#33374,#33375,#33376,#33377)) ;
#14373=EDGE_LOOP('',(#33378,#33379,#33380,#33381)) ;
#14374=EDGE_LOOP('',(#33382,#33383,#33384,#33385)) ;
#14375=EDGE_LOOP('',(#33386,#33387,#33388,#33389)) ;
#14376=EDGE_LOOP('',(#33390,#33391,#33392,#33393)) ;
#14377=EDGE_LOOP('',(#33394,#33395,#33396,#33397)) ;
#14378=EDGE_LOOP('',(#33398,#33399,#33400,#33401)) ;
#14379=EDGE_LOOP('',(#33402,#33403,#33404)) ;
#14380=EDGE_LOOP('',(#33405,#33406,#33407,#33408)) ;
#14381=EDGE_LOOP('',(#33409,#33410,#33411,#33412)) ;
#14382=EDGE_LOOP('',(#33413,#33414,#33415,#33416)) ;
#14383=EDGE_LOOP('',(#33417,#33418,#33419,#33420)) ;
#14384=EDGE_LOOP('',(#33421,#33422,#33423,#33424)) ;
#14385=EDGE_LOOP('',(#33425,#33426,#33427,#33428)) ;
#14386=EDGE_LOOP('',(#33429,#33430,#33431,#33432)) ;
#14387=EDGE_LOOP('',(#33433,#33434,#33435,#33436)) ;
#14388=EDGE_LOOP('',(#33437,#33438,#33439,#33440)) ;
#14389=EDGE_LOOP('',(#33441,#33442,#33443,#33444)) ;
#14390=EDGE_LOOP('',(#33445,#33446,#33447,#33448)) ;
#14391=EDGE_LOOP('',(#33449,#33450,#33451,#33452)) ;
#14392=EDGE_LOOP('',(#33453,#33454,#33455,#33456)) ;
#14393=EDGE_LOOP('',(#33457,#33458,#33459,#33460)) ;
#14394=EDGE_LOOP('',(#33461,#33462,#33463,#33464)) ;
#14395=EDGE_LOOP('',(#33465,#33466,#33467,#33468)) ;
#14396=EDGE_LOOP('',(#33469,#33470,#33471,#33472)) ;
#14397=EDGE_LOOP('',(#33473,#33474,#33475,#33476)) ;
#14398=EDGE_LOOP('',(#33477,#33478,#33479,#33480)) ;
#14399=EDGE_LOOP('',(#33481,#33482,#33483,#33484)) ;
#14400=EDGE_LOOP('',(#33485,#33486,#33487,#33488)) ;
#14401=EDGE_LOOP('',(#33489,#33490,#33491,#33492)) ;
#14402=EDGE_LOOP('',(#33493,#33494,#33495,#33496)) ;
#14403=EDGE_LOOP('',(#33497,#33498,#33499,#33500)) ;
#14404=EDGE_LOOP('',(#33501,#33502,#33503,#33504)) ;
#14405=EDGE_LOOP('',(#33505,#33506,#33507,#33508)) ;
#14406=EDGE_LOOP('',(#33509,#33510,#33511,#33512)) ;
#14407=EDGE_LOOP('',(#33513,#33514,#33515,#33516,#33517,#33518,#33519,#33520,
#33521,#33522,#33523,#33524,#33525,#33526,#33527,#33528,#33529,#33530,#33531,
#33532,#33533,#33534,#33535,#33536,#33537,#33538,#33539,#33540,#33541,#33542,
#33543,#33544,#33545,#33546,#33547,#33548,#33549,#33550,#33551,#33552,#33553,
#33554,#33555,#33556,#33557,#33558,#33559,#33560,#33561)) ;
#14408=EDGE_LOOP('',(#33562,#33563,#33564)) ;
#14409=EDGE_LOOP('',(#33565,#33566,#33567)) ;
#14410=EDGE_LOOP('',(#33568,#33569,#33570,#33571,#33572,#33573,#33574,#33575,
#33576,#33577,#33578,#33579,#33580,#33581)) ;
#14411=EDGE_LOOP('',(#33582,#33583,#33584,#33585,#33586,#33587,#33588,#33589,
#33590,#33591,#33592,#33593,#33594,#33595,#33596,#33597)) ;
#14412=EDGE_LOOP('',(#33598,#33599,#33600,#33601,#33602,#33603,#33604,#33605,
#33606,#33607,#33608,#33609,#33610,#33611)) ;
#14413=EDGE_LOOP('',(#33612,#33613,#33614,#33615,#33616,#33617,#33618,#33619,
#33620,#33621,#33622,#33623,#33624,#33625)) ;
#14414=EDGE_LOOP('',(#33626,#33627,#33628,#33629,#33630,#33631,#33632,#33633,
#33634,#33635,#33636,#33637,#33638,#33639)) ;
#14415=EDGE_LOOP('',(#33640)) ;
#14416=EDGE_LOOP('',(#33641,#33642,#33643,#33644,#33645,#33646,#33647,#33648,
#33649,#33650,#33651,#33652,#33653,#33654,#33655)) ;
#14417=EDGE_LOOP('',(#33656)) ;
#14418=EDGE_LOOP('',(#33657)) ;
#14419=EDGE_LOOP('',(#33658,#33659,#33660,#33661,#33662,#33663,#33664,#33665,
#33666,#33667,#33668,#33669,#33670,#33671)) ;
#14420=EDGE_LOOP('',(#33672)) ;
#14421=EDGE_LOOP('',(#33673)) ;
#14422=EDGE_LOOP('',(#33674,#33675,#33676,#33677,#33678,#33679,#33680,#33681)) ;
#14423=EDGE_LOOP('',(#33682,#33683,#33684,#33685,#33686,#33687,#33688,#33689,
#33690,#33691,#33692,#33693,#33694,#33695)) ;
#14424=EDGE_LOOP('',(#33696,#33697,#33698,#33699)) ;
#14425=EDGE_LOOP('',(#33700,#33701,#33702,#33703,#33704,#33705,#33706,#33707,
#33708,#33709,#33710,#33711,#33712,#33713,#33714,#33715,#33716,#33717,#33718)) ;
#14426=EDGE_LOOP('',(#33719,#33720,#33721,#33722)) ;
#14427=EDGE_LOOP('',(#33723,#33724,#33725,#33726)) ;
#14428=EDGE_LOOP('',(#33727,#33728,#33729,#33730)) ;
#14429=EDGE_LOOP('',(#33731,#33732,#33733,#33734)) ;
#14430=EDGE_LOOP('',(#33735,#33736,#33737,#33738)) ;
#14431=EDGE_LOOP('',(#33739,#33740,#33741,#33742)) ;
#14432=EDGE_LOOP('',(#33743,#33744,#33745,#33746)) ;
#14433=EDGE_LOOP('',(#33747,#33748,#33749,#33750)) ;
#14434=EDGE_LOOP('',(#33751,#33752,#33753,#33754)) ;
#14435=EDGE_LOOP('',(#33755,#33756,#33757,#33758)) ;
#14436=EDGE_LOOP('',(#33759,#33760,#33761,#33762)) ;
#14437=EDGE_LOOP('',(#33763,#33764,#33765,#33766)) ;
#14438=EDGE_LOOP('',(#33767,#33768,#33769,#33770)) ;
#14439=EDGE_LOOP('',(#33771,#33772,#33773,#33774)) ;
#14440=EDGE_LOOP('',(#33775,#33776,#33777,#33778)) ;
#14441=EDGE_LOOP('',(#33779,#33780,#33781,#33782)) ;
#14442=EDGE_LOOP('',(#33783,#33784,#33785,#33786)) ;
#14443=EDGE_LOOP('',(#33787,#33788,#33789,#33790)) ;
#14444=EDGE_LOOP('',(#33791,#33792,#33793,#33794)) ;
#14445=EDGE_LOOP('',(#33795,#33796,#33797,#33798,#33799)) ;
#14446=EDGE_LOOP('',(#33800)) ;
#14447=EDGE_LOOP('',(#33801)) ;
#14448=EDGE_LOOP('',(#33802,#33803,#33804,#33805,#33806)) ;
#14449=EDGE_LOOP('',(#33807,#33808,#33809,#33810)) ;
#14450=EDGE_LOOP('',(#33811,#33812,#33813,#33814)) ;
#14451=EDGE_LOOP('',(#33815,#33816,#33817,#33818)) ;
#14452=EDGE_LOOP('',(#33819,#33820,#33821,#33822,#33823,#33824,#33825,#33826,
#33827,#33828,#33829,#33830,#33831,#33832,#33833,#33834,#33835,#33836,#33837,
#33838,#33839,#33840,#33841,#33842,#33843,#33844,#33845,#33846,#33847,#33848,
#33849,#33850,#33851,#33852,#33853,#33854,#33855,#33856,#33857,#33858,#33859,
#33860,#33861,#33862,#33863,#33864,#33865,#33866,#33867,#33868,#33869,#33870,
#33871,#33872,#33873,#33874,#33875)) ;
#14453=EDGE_LOOP('',(#33876)) ;
#14454=EDGE_LOOP('',(#33877,#33878,#33879,#33880,#33881,#33882,#33883,#33884,
#33885,#33886,#33887,#33888,#33889,#33890)) ;
#14455=EDGE_LOOP('',(#33891)) ;
#14456=EDGE_LOOP('',(#33892)) ;
#14457=EDGE_LOOP('',(#33893,#33894,#33895,#33896,#33897,#33898,#33899,#33900,
#33901,#33902,#33903,#33904,#33905,#33906,#33907,#33908)) ;
#14458=EDGE_LOOP('',(#33909)) ;
#14459=EDGE_LOOP('',(#33910,#33911,#33912,#33913,#33914,#33915,#33916,#33917,
#33918,#33919,#33920,#33921,#33922,#33923)) ;
#14460=EDGE_LOOP('',(#33924,#33925,#33926,#33927,#33928,#33929,#33930,#33931)) ;
#14461=EDGE_LOOP('',(#33932,#33933,#33934,#33935,#33936,#33937,#33938,#33939,
#33940,#33941,#33942,#33943,#33944,#33945)) ;
#14462=EDGE_LOOP('',(#33946,#33947,#33948,#33949,#33950,#33951,#33952,#33953,
#33954,#33955,#33956,#33957,#33958,#33959)) ;
#14463=EDGE_LOOP('',(#33960,#33961,#33962,#33963,#33964,#33965,#33966,#33967,
#33968,#33969,#33970,#33971,#33972,#33973)) ;
#14464=EDGE_LOOP('',(#33974,#33975,#33976,#33977,#33978,#33979,#33980,#33981,
#33982,#33983,#33984,#33985,#33986,#33987)) ;
#14465=EDGE_LOOP('',(#33988)) ;
#14466=EDGE_LOOP('',(#33989)) ;
#14467=EDGE_LOOP('',(#33990,#33991,#33992,#33993)) ;
#14468=EDGE_LOOP('',(#33994,#33995,#33996,#33997)) ;
#14469=EDGE_LOOP('',(#33998,#33999,#34000,#34001)) ;
#14470=EDGE_LOOP('',(#34002,#34003,#34004,#34005)) ;
#14471=EDGE_LOOP('',(#34006,#34007,#34008,#34009)) ;
#14472=EDGE_LOOP('',(#34010,#34011,#34012,#34013)) ;
#14473=EDGE_LOOP('',(#34014,#34015,#34016,#34017)) ;
#14474=EDGE_LOOP('',(#34018,#34019,#34020,#34021)) ;
#14475=EDGE_LOOP('',(#34022,#34023,#34024,#34025)) ;
#14476=EDGE_LOOP('',(#34026,#34027,#34028,#34029)) ;
#14477=EDGE_LOOP('',(#34030,#34031,#34032,#34033)) ;
#14478=EDGE_LOOP('',(#34034,#34035,#34036,#34037)) ;
#14479=EDGE_LOOP('',(#34038,#34039,#34040,#34041)) ;
#14480=EDGE_LOOP('',(#34042,#34043,#34044,#34045,#34046,#34047,#34048,#34049)) ;
#14481=EDGE_LOOP('',(#34050,#34051,#34052,#34053)) ;
#14482=EDGE_LOOP('',(#34054,#34055,#34056,#34057)) ;
#14483=EDGE_LOOP('',(#34058,#34059,#34060,#34061)) ;
#14484=EDGE_LOOP('',(#34062,#34063,#34064,#34065)) ;
#14485=EDGE_LOOP('',(#34066,#34067,#34068,#34069)) ;
#14486=EDGE_LOOP('',(#34070,#34071,#34072,#34073)) ;
#14487=EDGE_LOOP('',(#34074,#34075,#34076,#34077)) ;
#14488=EDGE_LOOP('',(#34078,#34079,#34080,#34081)) ;
#14489=EDGE_LOOP('',(#34082,#34083,#34084,#34085)) ;
#14490=EDGE_LOOP('',(#34086,#34087,#34088,#34089,#34090,#34091,#34092,#34093)) ;
#14491=EDGE_LOOP('',(#34094,#34095,#34096,#34097)) ;
#14492=EDGE_LOOP('',(#34098,#34099,#34100,#34101)) ;
#14493=EDGE_LOOP('',(#34102,#34103,#34104,#34105,#34106)) ;
#14494=EDGE_LOOP('',(#34107,#34108,#34109,#34110,#34111)) ;
#14495=EDGE_LOOP('',(#34112)) ;
#14496=EDGE_LOOP('',(#34113)) ;
#14497=EDGE_LOOP('',(#34114,#34115,#34116,#34117,#34118)) ;
#14498=EDGE_LOOP('',(#34119,#34120,#34121,#34122,#34123)) ;
#14499=EDGE_LOOP('',(#34124,#34125,#34126,#34127,#34128)) ;
#14500=EDGE_LOOP('',(#34129,#34130,#34131,#34132,#34133,#34134)) ;
#14501=EDGE_LOOP('',(#34135,#34136,#34137,#34138,#34139,#34140)) ;
#14502=EDGE_LOOP('',(#34141)) ;
#14503=EDGE_LOOP('',(#34142,#34143,#34144,#34145,#34146)) ;
#14504=EDGE_LOOP('',(#34147,#34148,#34149,#34150,#34151,#34152)) ;
#14505=EDGE_LOOP('',(#34153)) ;
#14506=EDGE_LOOP('',(#34154,#34155,#34156,#34157,#34158)) ;
#14507=EDGE_LOOP('',(#34159,#34160,#34161,#34162,#34163,#34164)) ;
#14508=EDGE_LOOP('',(#34165,#34166,#34167,#34168,#34169,#34170)) ;
#14509=EDGE_LOOP('',(#34171)) ;
#14510=EDGE_LOOP('',(#34172,#34173,#34174,#34175,#34176)) ;
#14511=EDGE_LOOP('',(#34177,#34178,#34179,#34180,#34181,#34182)) ;
#14512=EDGE_LOOP('',(#34183)) ;
#14513=EDGE_LOOP('',(#34184,#34185,#34186,#34187)) ;
#14514=EDGE_LOOP('',(#34188,#34189,#34190,#34191)) ;
#14515=EDGE_LOOP('',(#34192,#34193,#34194,#34195)) ;
#14516=EDGE_LOOP('',(#34196,#34197,#34198,#34199)) ;
#14517=EDGE_LOOP('',(#34200,#34201,#34202,#34203)) ;
#14518=EDGE_LOOP('',(#34204,#34205,#34206,#34207,#34208,#34209,#34210,#34211,
#34212,#34213,#34214,#34215,#34216,#34217,#34218,#34219,#34220,#34221,#34222,
#34223,#34224,#34225,#34226,#34227)) ;
#14519=EDGE_LOOP('',(#34228,#34229,#34230,#34231)) ;
#14520=EDGE_LOOP('',(#34232,#34233,#34234,#34235,#34236,#34237,#34238,#34239,
#34240,#34241,#34242,#34243,#34244,#34245,#34246,#34247,#34248,#34249,#34250,
#34251,#34252,#34253,#34254,#34255,#34256,#34257,#34258,#34259,#34260,#34261,
#34262)) ;
#14521=EDGE_LOOP('',(#34263,#34264,#34265,#34266)) ;
#14522=EDGE_LOOP('',(#34267,#34268,#34269,#34270)) ;
#14523=EDGE_LOOP('',(#34271,#34272,#34273,#34274)) ;
#14524=EDGE_LOOP('',(#34275,#34276,#34277,#34278)) ;
#14525=EDGE_LOOP('',(#34279,#34280,#34281,#34282)) ;
#14526=EDGE_LOOP('',(#34283,#34284,#34285,#34286)) ;
#14527=EDGE_LOOP('',(#34287,#34288,#34289,#34290)) ;
#14528=EDGE_LOOP('',(#34291,#34292,#34293,#34294)) ;
#14529=EDGE_LOOP('',(#34295,#34296,#34297,#34298,#34299)) ;
#14530=EDGE_LOOP('',(#34300,#34301,#34302,#34303)) ;
#14531=EDGE_LOOP('',(#34304,#34305,#34306,#34307)) ;
#14532=EDGE_LOOP('',(#34308,#34309,#34310,#34311,#34312)) ;
#14533=EDGE_LOOP('',(#34313,#34314,#34315,#34316)) ;
#14534=EDGE_LOOP('',(#34317,#34318,#34319,#34320,#34321)) ;
#14535=EDGE_LOOP('',(#34322,#34323,#34324)) ;
#14536=EDGE_LOOP('',(#34325,#34326,#34327,#34328)) ;
#14537=EDGE_LOOP('',(#34329,#34330,#34331,#34332)) ;
#14538=EDGE_LOOP('',(#34333,#34334,#34335)) ;
#14539=EDGE_LOOP('',(#34336,#34337,#34338,#34339)) ;
#14540=EDGE_LOOP('',(#34340,#34341,#34342,#34343)) ;
#14541=EDGE_LOOP('',(#34344,#34345,#34346,#34347)) ;
#14542=EDGE_LOOP('',(#34348,#34349,#34350,#34351)) ;
#14543=EDGE_LOOP('',(#34352,#34353,#34354,#34355)) ;
#14544=EDGE_LOOP('',(#34356,#34357,#34358,#34359)) ;
#14545=EDGE_LOOP('',(#34360,#34361,#34362,#34363)) ;
#14546=EDGE_LOOP('',(#34364,#34365,#34366,#34367)) ;
#14547=EDGE_LOOP('',(#34368,#34369,#34370,#34371)) ;
#14548=EDGE_LOOP('',(#34372,#34373,#34374,#34375)) ;
#14549=EDGE_LOOP('',(#34376,#34377,#34378)) ;
#14550=EDGE_LOOP('',(#34379,#34380,#34381,#34382)) ;
#14551=EDGE_LOOP('',(#34383,#34384,#34385,#34386)) ;
#14552=EDGE_LOOP('',(#34387,#34388,#34389,#34390)) ;
#14553=EDGE_LOOP('',(#34391,#34392,#34393,#34394)) ;
#14554=EDGE_LOOP('',(#34395,#34396,#34397,#34398)) ;
#14555=EDGE_LOOP('',(#34399,#34400,#34401,#34402)) ;
#14556=EDGE_LOOP('',(#34403,#34404,#34405,#34406)) ;
#14557=EDGE_LOOP('',(#34407,#34408,#34409)) ;
#14558=EDGE_LOOP('',(#34410,#34411,#34412,#34413)) ;
#14559=EDGE_LOOP('',(#34414,#34415,#34416,#34417,#34418)) ;
#14560=EDGE_LOOP('',(#34419,#34420,#34421)) ;
#14561=EDGE_LOOP('',(#34422,#34423,#34424,#34425)) ;
#14562=EDGE_LOOP('',(#34426,#34427,#34428,#34429)) ;
#14563=EDGE_LOOP('',(#34430,#34431,#34432,#34433,#34434)) ;
#14564=EDGE_LOOP('',(#34435,#34436,#34437,#34438)) ;
#14565=EDGE_LOOP('',(#34439,#34440,#34441,#34442)) ;
#14566=EDGE_LOOP('',(#34443,#34444,#34445,#34446)) ;
#14567=EDGE_LOOP('',(#34447,#34448,#34449,#34450)) ;
#14568=EDGE_LOOP('',(#34451,#34452,#34453,#34454)) ;
#14569=EDGE_LOOP('',(#34455,#34456,#34457,#34458)) ;
#14570=EDGE_LOOP('',(#34459,#34460,#34461,#34462)) ;
#14571=EDGE_LOOP('',(#34463,#34464,#34465,#34466)) ;
#14572=EDGE_LOOP('',(#34467,#34468,#34469,#34470)) ;
#14573=EDGE_LOOP('',(#34471,#34472,#34473,#34474)) ;
#14574=EDGE_LOOP('',(#34475,#34476,#34477,#34478)) ;
#14575=EDGE_LOOP('',(#34479,#34480,#34481,#34482)) ;
#14576=EDGE_LOOP('',(#34483,#34484,#34485,#34486)) ;
#14577=EDGE_LOOP('',(#34487,#34488,#34489,#34490)) ;
#14578=EDGE_LOOP('',(#34491,#34492,#34493,#34494)) ;
#14579=EDGE_LOOP('',(#34495,#34496,#34497,#34498)) ;
#14580=EDGE_LOOP('',(#34499,#34500,#34501,#34502)) ;
#14581=EDGE_LOOP('',(#34503,#34504,#34505,#34506)) ;
#14582=EDGE_LOOP('',(#34507,#34508,#34509,#34510)) ;
#14583=EDGE_LOOP('',(#34511,#34512,#34513,#34514)) ;
#14584=EDGE_LOOP('',(#34515,#34516,#34517,#34518)) ;
#14585=EDGE_LOOP('',(#34519,#34520,#34521,#34522)) ;
#14586=EDGE_LOOP('',(#34523,#34524,#34525,#34526)) ;
#14587=EDGE_LOOP('',(#34527,#34528,#34529,#34530)) ;
#14588=EDGE_LOOP('',(#34531,#34532,#34533,#34534)) ;
#14589=EDGE_LOOP('',(#34535,#34536,#34537,#34538)) ;
#14590=EDGE_LOOP('',(#34539,#34540,#34541,#34542)) ;
#14591=EDGE_LOOP('',(#34543,#34544,#34545,#34546)) ;
#14592=EDGE_LOOP('',(#34547,#34548,#34549,#34550)) ;
#14593=EDGE_LOOP('',(#34551,#34552,#34553,#34554)) ;
#14594=EDGE_LOOP('',(#34555,#34556,#34557,#34558)) ;
#14595=EDGE_LOOP('',(#34559,#34560,#34561,#34562)) ;
#14596=EDGE_LOOP('',(#34563,#34564,#34565,#34566)) ;
#14597=EDGE_LOOP('',(#34567,#34568,#34569)) ;
#14598=EDGE_LOOP('',(#34570,#34571,#34572)) ;
#14599=EDGE_LOOP('',(#34573,#34574,#34575,#34576)) ;
#14600=EDGE_LOOP('',(#34577,#34578,#34579,#34580)) ;
#14601=EDGE_LOOP('',(#34581,#34582,#34583,#34584)) ;
#14602=EDGE_LOOP('',(#34585,#34586,#34587,#34588)) ;
#14603=EDGE_LOOP('',(#34589,#34590,#34591,#34592)) ;
#14604=EDGE_LOOP('',(#34593,#34594,#34595,#34596)) ;
#14605=EDGE_LOOP('',(#34597,#34598,#34599,#34600)) ;
#14606=EDGE_LOOP('',(#34601,#34602,#34603,#34604)) ;
#14607=EDGE_LOOP('',(#34605,#34606,#34607,#34608)) ;
#14608=EDGE_LOOP('',(#34609,#34610,#34611,#34612)) ;
#14609=EDGE_LOOP('',(#34613,#34614,#34615,#34616)) ;
#14610=EDGE_LOOP('',(#34617,#34618,#34619,#34620)) ;
#14611=EDGE_LOOP('',(#34621,#34622,#34623,#34624)) ;
#14612=EDGE_LOOP('',(#34625,#34626,#34627,#34628)) ;
#14613=EDGE_LOOP('',(#34629,#34630,#34631,#34632)) ;
#14614=EDGE_LOOP('',(#34633,#34634,#34635,#34636)) ;
#14615=EDGE_LOOP('',(#34637,#34638,#34639,#34640)) ;
#14616=EDGE_LOOP('',(#34641,#34642,#34643,#34644)) ;
#14617=EDGE_LOOP('',(#34645,#34646,#34647,#34648)) ;
#14618=EDGE_LOOP('',(#34649,#34650,#34651,#34652)) ;
#14619=EDGE_LOOP('',(#34653,#34654,#34655,#34656)) ;
#14620=EDGE_LOOP('',(#34657,#34658,#34659)) ;
#14621=EDGE_LOOP('',(#34660,#34661,#34662,#34663)) ;
#14622=EDGE_LOOP('',(#34664,#34665,#34666)) ;
#14623=EDGE_LOOP('',(#34667,#34668,#34669,#34670)) ;
#14624=EDGE_LOOP('',(#34671,#34672,#34673,#34674)) ;
#14625=EDGE_LOOP('',(#34675,#34676,#34677,#34678)) ;
#14626=EDGE_LOOP('',(#34679,#34680,#34681,#34682)) ;
#14627=EDGE_LOOP('',(#34683,#34684,#34685,#34686)) ;
#14628=EDGE_LOOP('',(#34687,#34688,#34689,#34690)) ;
#14629=EDGE_LOOP('',(#34691,#34692,#34693,#34694)) ;
#14630=EDGE_LOOP('',(#34695,#34696,#34697,#34698)) ;
#14631=EDGE_LOOP('',(#34699,#34700,#34701,#34702)) ;
#14632=EDGE_LOOP('',(#34703,#34704,#34705)) ;
#14633=EDGE_LOOP('',(#34706,#34707,#34708,#34709)) ;
#14634=EDGE_LOOP('',(#34710,#34711,#34712,#34713)) ;
#14635=EDGE_LOOP('',(#34714,#34715,#34716)) ;
#14636=EDGE_LOOP('',(#34717,#34718,#34719,#34720)) ;
#14637=EDGE_LOOP('',(#34721,#34722,#34723,#34724)) ;
#14638=EDGE_LOOP('',(#34725,#34726,#34727,#34728)) ;
#14639=EDGE_LOOP('',(#34729,#34730,#34731,#34732)) ;
#14640=EDGE_LOOP('',(#34733,#34734,#34735,#34736)) ;
#14641=EDGE_LOOP('',(#34737,#34738,#34739,#34740)) ;
#14642=EDGE_LOOP('',(#34741,#34742,#34743,#34744)) ;
#14643=EDGE_LOOP('',(#34745,#34746,#34747,#34748)) ;
#14644=EDGE_LOOP('',(#34749,#34750,#34751,#34752)) ;
#14645=EDGE_LOOP('',(#34753,#34754,#34755,#34756)) ;
#14646=EDGE_LOOP('',(#34757,#34758,#34759,#34760)) ;
#14647=EDGE_LOOP('',(#34761,#34762,#34763,#34764)) ;
#14648=EDGE_LOOP('',(#34765,#34766,#34767,#34768)) ;
#14649=EDGE_LOOP('',(#34769,#34770,#34771,#34772)) ;
#14650=EDGE_LOOP('',(#34773,#34774,#34775,#34776)) ;
#14651=EDGE_LOOP('',(#34777,#34778,#34779,#34780)) ;
#14652=EDGE_LOOP('',(#34781,#34782,#34783)) ;
#14653=EDGE_LOOP('',(#34784,#34785,#34786,#34787)) ;
#14654=EDGE_LOOP('',(#34788,#34789,#34790,#34791)) ;
#14655=EDGE_LOOP('',(#34792,#34793,#34794)) ;
#14656=EDGE_LOOP('',(#34795,#34796,#34797,#34798)) ;
#14657=EDGE_LOOP('',(#34799,#34800,#34801,#34802)) ;
#14658=EDGE_LOOP('',(#34803,#34804,#34805,#34806)) ;
#14659=EDGE_LOOP('',(#34807,#34808,#34809,#34810)) ;
#14660=EDGE_LOOP('',(#34811,#34812,#34813,#34814)) ;
#14661=EDGE_LOOP('',(#34815,#34816,#34817,#34818)) ;
#14662=EDGE_LOOP('',(#34819,#34820,#34821,#34822)) ;
#14663=EDGE_LOOP('',(#34823,#34824,#34825,#34826)) ;
#14664=EDGE_LOOP('',(#34827,#34828,#34829,#34830)) ;
#14665=EDGE_LOOP('',(#34831,#34832,#34833,#34834)) ;
#14666=EDGE_LOOP('',(#34835,#34836,#34837,#34838)) ;
#14667=EDGE_LOOP('',(#34839,#34840,#34841,#34842)) ;
#14668=EDGE_LOOP('',(#34843,#34844,#34845)) ;
#14669=EDGE_LOOP('',(#34846,#34847,#34848,#34849)) ;
#14670=EDGE_LOOP('',(#34850,#34851,#34852,#34853)) ;
#14671=EDGE_LOOP('',(#34854,#34855,#34856,#34857)) ;
#14672=EDGE_LOOP('',(#34858,#34859,#34860,#34861)) ;
#14673=EDGE_LOOP('',(#34862,#34863,#34864,#34865)) ;
#14674=EDGE_LOOP('',(#34866,#34867,#34868,#34869)) ;
#14675=EDGE_LOOP('',(#34870,#34871,#34872,#34873)) ;
#14676=EDGE_LOOP('',(#34874,#34875,#34876,#34877)) ;
#14677=EDGE_LOOP('',(#34878,#34879,#34880,#34881)) ;
#14678=EDGE_LOOP('',(#34882,#34883,#34884,#34885)) ;
#14679=EDGE_LOOP('',(#34886,#34887,#34888,#34889)) ;
#14680=EDGE_LOOP('',(#34890,#34891,#34892,#34893)) ;
#14681=EDGE_LOOP('',(#34894,#34895,#34896,#34897)) ;
#14682=EDGE_LOOP('',(#34898,#34899,#34900,#34901)) ;
#14683=EDGE_LOOP('',(#34902,#34903,#34904,#34905)) ;
#14684=EDGE_LOOP('',(#34906,#34907,#34908,#34909)) ;
#14685=EDGE_LOOP('',(#34910,#34911,#34912,#34913)) ;
#14686=EDGE_LOOP('',(#34914,#34915,#34916,#34917)) ;
#14687=EDGE_LOOP('',(#34918,#34919,#34920,#34921)) ;
#14688=EDGE_LOOP('',(#34922,#34923,#34924,#34925)) ;
#14689=EDGE_LOOP('',(#34926,#34927,#34928,#34929)) ;
#14690=EDGE_LOOP('',(#34930,#34931,#34932,#34933)) ;
#14691=EDGE_LOOP('',(#34934,#34935,#34936,#34937)) ;
#14692=EDGE_LOOP('',(#34938,#34939,#34940,#34941)) ;
#14693=EDGE_LOOP('',(#34942,#34943,#34944,#34945)) ;
#14694=EDGE_LOOP('',(#34946,#34947,#34948,#34949)) ;
#14695=EDGE_LOOP('',(#34950,#34951,#34952,#34953)) ;
#14696=EDGE_LOOP('',(#34954,#34955,#34956,#34957)) ;
#14697=EDGE_LOOP('',(#34958,#34959,#34960,#34961)) ;
#14698=EDGE_LOOP('',(#34962,#34963,#34964,#34965)) ;
#14699=EDGE_LOOP('',(#34966,#34967,#34968,#34969)) ;
#14700=EDGE_LOOP('',(#34970,#34971,#34972,#34973)) ;
#14701=EDGE_LOOP('',(#34974,#34975,#34976,#34977)) ;
#14702=EDGE_LOOP('',(#34978,#34979,#34980,#34981)) ;
#14703=EDGE_LOOP('',(#34982,#34983,#34984,#34985)) ;
#14704=EDGE_LOOP('',(#34986,#34987,#34988,#34989)) ;
#14705=EDGE_LOOP('',(#34990,#34991,#34992,#34993)) ;
#14706=EDGE_LOOP('',(#34994,#34995,#34996,#34997)) ;
#14707=EDGE_LOOP('',(#34998,#34999,#35000,#35001)) ;
#14708=EDGE_LOOP('',(#35002,#35003,#35004,#35005)) ;
#14709=EDGE_LOOP('',(#35006,#35007,#35008,#35009)) ;
#14710=EDGE_LOOP('',(#35010,#35011,#35012,#35013)) ;
#14711=EDGE_LOOP('',(#35014,#35015,#35016,#35017)) ;
#14712=EDGE_LOOP('',(#35018,#35019,#35020,#35021)) ;
#14713=EDGE_LOOP('',(#35022,#35023,#35024,#35025)) ;
#14714=EDGE_LOOP('',(#35026,#35027,#35028)) ;
#14715=EDGE_LOOP('',(#35029,#35030,#35031)) ;
#14716=EDGE_LOOP('',(#35032,#35033,#35034,#35035)) ;
#14717=EDGE_LOOP('',(#35036,#35037,#35038,#35039)) ;
#14718=EDGE_LOOP('',(#35040,#35041,#35042,#35043)) ;
#14719=EDGE_LOOP('',(#35044,#35045,#35046,#35047)) ;
#14720=EDGE_LOOP('',(#35048,#35049,#35050,#35051)) ;
#14721=EDGE_LOOP('',(#35052,#35053,#35054,#35055)) ;
#14722=EDGE_LOOP('',(#35056,#35057,#35058,#35059)) ;
#14723=EDGE_LOOP('',(#35060,#35061,#35062,#35063)) ;
#14724=EDGE_LOOP('',(#35064,#35065,#35066,#35067)) ;
#14725=EDGE_LOOP('',(#35068,#35069,#35070,#35071)) ;
#14726=EDGE_LOOP('',(#35072,#35073,#35074,#35075)) ;
#14727=EDGE_LOOP('',(#35076,#35077,#35078,#35079)) ;
#14728=EDGE_LOOP('',(#35080,#35081,#35082,#35083)) ;
#14729=EDGE_LOOP('',(#35084,#35085,#35086,#35087)) ;
#14730=EDGE_LOOP('',(#35088,#35089,#35090,#35091)) ;
#14731=EDGE_LOOP('',(#35092,#35093,#35094,#35095)) ;
#14732=EDGE_LOOP('',(#35096,#35097,#35098,#35099)) ;
#14733=EDGE_LOOP('',(#35100,#35101,#35102,#35103)) ;
#14734=EDGE_LOOP('',(#35104,#35105,#35106,#35107)) ;
#14735=EDGE_LOOP('',(#35108,#35109,#35110,#35111)) ;
#14736=EDGE_LOOP('',(#35112,#35113,#35114,#35115)) ;
#14737=EDGE_LOOP('',(#35116,#35117,#35118,#35119)) ;
#14738=EDGE_LOOP('',(#35120,#35121,#35122)) ;
#14739=EDGE_LOOP('',(#35123,#35124,#35125,#35126)) ;
#14740=EDGE_LOOP('',(#35127,#35128,#35129,#35130)) ;
#14741=EDGE_LOOP('',(#35131,#35132,#35133,#35134)) ;
#14742=EDGE_LOOP('',(#35135,#35136,#35137,#35138)) ;
#14743=EDGE_LOOP('',(#35139,#35140,#35141)) ;
#14744=EDGE_LOOP('',(#35142,#35143,#35144,#35145)) ;
#14745=EDGE_LOOP('',(#35146,#35147,#35148,#35149)) ;
#14746=EDGE_LOOP('',(#35150,#35151,#35152,#35153)) ;
#14747=EDGE_LOOP('',(#35154,#35155,#35156,#35157)) ;
#14748=EDGE_LOOP('',(#35158,#35159,#35160,#35161)) ;
#14749=EDGE_LOOP('',(#35162,#35163,#35164,#35165)) ;
#14750=EDGE_LOOP('',(#35166,#35167,#35168,#35169)) ;
#14751=EDGE_LOOP('',(#35170,#35171,#35172,#35173)) ;
#14752=EDGE_LOOP('',(#35174,#35175,#35176,#35177)) ;
#14753=EDGE_LOOP('',(#35178,#35179,#35180,#35181)) ;
#14754=EDGE_LOOP('',(#35182,#35183,#35184,#35185)) ;
#14755=EDGE_LOOP('',(#35186,#35187,#35188,#35189)) ;
#14756=EDGE_LOOP('',(#35190,#35191,#35192,#35193)) ;
#14757=EDGE_LOOP('',(#35194,#35195,#35196,#35197)) ;
#14758=EDGE_LOOP('',(#35198,#35199,#35200,#35201)) ;
#14759=EDGE_LOOP('',(#35202,#35203,#35204,#35205)) ;
#14760=EDGE_LOOP('',(#35206,#35207,#35208,#35209)) ;
#14761=EDGE_LOOP('',(#35210,#35211,#35212,#35213)) ;
#14762=EDGE_LOOP('',(#35214,#35215,#35216,#35217)) ;
#14763=EDGE_LOOP('',(#35218,#35219,#35220,#35221)) ;
#14764=EDGE_LOOP('',(#35222,#35223,#35224,#35225)) ;
#14765=EDGE_LOOP('',(#35226,#35227,#35228,#35229)) ;
#14766=EDGE_LOOP('',(#35230,#35231,#35232,#35233)) ;
#14767=EDGE_LOOP('',(#35234,#35235,#35236,#35237)) ;
#14768=EDGE_LOOP('',(#35238,#35239,#35240,#35241)) ;
#14769=EDGE_LOOP('',(#35242,#35243,#35244,#35245)) ;
#14770=EDGE_LOOP('',(#35246,#35247,#35248,#35249)) ;
#14771=EDGE_LOOP('',(#35250,#35251,#35252,#35253)) ;
#14772=EDGE_LOOP('',(#35254,#35255,#35256,#35257)) ;
#14773=EDGE_LOOP('',(#35258,#35259,#35260,#35261)) ;
#14774=EDGE_LOOP('',(#35262,#35263,#35264,#35265)) ;
#14775=EDGE_LOOP('',(#35266,#35267,#35268,#35269)) ;
#14776=EDGE_LOOP('',(#35270,#35271,#35272,#35273)) ;
#14777=EDGE_LOOP('',(#35274,#35275,#35276,#35277)) ;
#14778=EDGE_LOOP('',(#35278,#35279,#35280,#35281)) ;
#14779=EDGE_LOOP('',(#35282,#35283,#35284,#35285)) ;
#14780=EDGE_LOOP('',(#35286,#35287,#35288,#35289)) ;
#14781=EDGE_LOOP('',(#35290,#35291,#35292,#35293)) ;
#14782=EDGE_LOOP('',(#35294,#35295,#35296,#35297)) ;
#14783=EDGE_LOOP('',(#35298,#35299,#35300,#35301)) ;
#14784=EDGE_LOOP('',(#35302,#35303,#35304,#35305)) ;
#14785=EDGE_LOOP('',(#35306,#35307,#35308,#35309)) ;
#14786=EDGE_LOOP('',(#35310,#35311,#35312,#35313)) ;
#14787=EDGE_LOOP('',(#35314,#35315,#35316,#35317)) ;
#14788=EDGE_LOOP('',(#35318,#35319,#35320,#35321)) ;
#14789=EDGE_LOOP('',(#35322,#35323,#35324,#35325)) ;
#14790=EDGE_LOOP('',(#35326,#35327,#35328,#35329)) ;
#14791=EDGE_LOOP('',(#35330,#35331,#35332,#35333)) ;
#14792=EDGE_LOOP('',(#35334,#35335,#35336,#35337)) ;
#14793=EDGE_LOOP('',(#35338,#35339,#35340,#35341)) ;
#14794=EDGE_LOOP('',(#35342,#35343,#35344,#35345)) ;
#14795=EDGE_LOOP('',(#35346,#35347,#35348,#35349)) ;
#14796=EDGE_LOOP('',(#35350,#35351,#35352,#35353)) ;
#14797=EDGE_LOOP('',(#35354,#35355,#35356,#35357)) ;
#14798=EDGE_LOOP('',(#35358,#35359,#35360,#35361)) ;
#14799=EDGE_LOOP('',(#35362,#35363,#35364,#35365)) ;
#14800=EDGE_LOOP('',(#35366,#35367,#35368,#35369)) ;
#14801=EDGE_LOOP('',(#35370,#35371,#35372,#35373)) ;
#14802=EDGE_LOOP('',(#35374,#35375,#35376,#35377)) ;
#14803=EDGE_LOOP('',(#35378,#35379,#35380,#35381,#35382)) ;
#14804=EDGE_LOOP('',(#35383,#35384,#35385,#35386)) ;
#14805=EDGE_LOOP('',(#35387,#35388,#35389,#35390)) ;
#14806=EDGE_LOOP('',(#35391,#35392,#35393,#35394)) ;
#14807=EDGE_LOOP('',(#35395,#35396,#35397,#35398)) ;
#14808=EDGE_LOOP('',(#35399,#35400,#35401,#35402)) ;
#14809=EDGE_LOOP('',(#35403,#35404,#35405,#35406)) ;
#14810=EDGE_LOOP('',(#35407,#35408,#35409,#35410)) ;
#14811=EDGE_LOOP('',(#35411,#35412,#35413,#35414)) ;
#14812=EDGE_LOOP('',(#35415,#35416,#35417,#35418)) ;
#14813=EDGE_LOOP('',(#35419,#35420,#35421,#35422)) ;
#14814=EDGE_LOOP('',(#35423,#35424,#35425,#35426)) ;
#14815=EDGE_LOOP('',(#35427,#35428,#35429,#35430)) ;
#14816=EDGE_LOOP('',(#35431,#35432,#35433,#35434)) ;
#14817=EDGE_LOOP('',(#35435,#35436,#35437,#35438)) ;
#14818=EDGE_LOOP('',(#35439,#35440,#35441,#35442)) ;
#14819=EDGE_LOOP('',(#35443,#35444,#35445,#35446)) ;
#14820=EDGE_LOOP('',(#35447,#35448,#35449,#35450)) ;
#14821=EDGE_LOOP('',(#35451,#35452,#35453,#35454)) ;
#14822=EDGE_LOOP('',(#35455,#35456,#35457,#35458)) ;
#14823=EDGE_LOOP('',(#35459,#35460,#35461,#35462)) ;
#14824=EDGE_LOOP('',(#35463,#35464,#35465,#35466)) ;
#14825=EDGE_LOOP('',(#35467,#35468,#35469,#35470)) ;
#14826=EDGE_LOOP('',(#35471,#35472,#35473,#35474)) ;
#14827=EDGE_LOOP('',(#35475,#35476,#35477,#35478)) ;
#14828=EDGE_LOOP('',(#35479,#35480,#35481,#35482)) ;
#14829=EDGE_LOOP('',(#35483,#35484,#35485,#35486)) ;
#14830=EDGE_LOOP('',(#35487,#35488,#35489)) ;
#14831=EDGE_LOOP('',(#35490,#35491,#35492,#35493)) ;
#14832=EDGE_LOOP('',(#35494,#35495,#35496,#35497)) ;
#14833=EDGE_LOOP('',(#35498,#35499,#35500,#35501,#35502,#35503)) ;
#14834=EDGE_LOOP('',(#35504,#35505,#35506,#35507)) ;
#14835=EDGE_LOOP('',(#35508,#35509,#35510,#35511)) ;
#14836=EDGE_LOOP('',(#35512,#35513,#35514)) ;
#14837=EDGE_LOOP('',(#35515,#35516,#35517,#35518,#35519)) ;
#14838=EDGE_LOOP('',(#35520,#35521,#35522,#35523)) ;
#14839=EDGE_LOOP('',(#35524,#35525,#35526,#35527)) ;
#14840=EDGE_LOOP('',(#35528,#35529,#35530,#35531)) ;
#14841=EDGE_LOOP('',(#35532,#35533,#35534,#35535)) ;
#14842=EDGE_LOOP('',(#35536,#35537,#35538,#35539)) ;
#14843=EDGE_LOOP('',(#35540,#35541,#35542,#35543)) ;
#14844=EDGE_LOOP('',(#35544,#35545,#35546,#35547)) ;
#14845=EDGE_LOOP('',(#35548,#35549,#35550,#35551)) ;
#14846=EDGE_LOOP('',(#35552,#35553,#35554,#35555)) ;
#14847=EDGE_LOOP('',(#35556,#35557,#35558,#35559)) ;
#14848=EDGE_LOOP('',(#35560,#35561,#35562,#35563)) ;
#14849=EDGE_LOOP('',(#35564,#35565,#35566,#35567)) ;
#14850=EDGE_LOOP('',(#35568,#35569,#35570,#35571)) ;
#14851=EDGE_LOOP('',(#35572,#35573,#35574,#35575)) ;
#14852=EDGE_LOOP('',(#35576,#35577,#35578,#35579)) ;
#14853=EDGE_LOOP('',(#35580,#35581,#35582,#35583)) ;
#14854=EDGE_LOOP('',(#35584,#35585,#35586,#35587)) ;
#14855=EDGE_LOOP('',(#35588,#35589,#35590,#35591)) ;
#14856=EDGE_LOOP('',(#35592,#35593,#35594,#35595)) ;
#14857=EDGE_LOOP('',(#35596,#35597,#35598,#35599)) ;
#14858=EDGE_LOOP('',(#35600,#35601,#35602,#35603)) ;
#14859=EDGE_LOOP('',(#35604,#35605,#35606)) ;
#14860=EDGE_LOOP('',(#35607,#35608,#35609,#35610)) ;
#14861=EDGE_LOOP('',(#35611,#35612,#35613,#35614)) ;
#14862=EDGE_LOOP('',(#35615,#35616,#35617,#35618)) ;
#14863=EDGE_LOOP('',(#35619,#35620,#35621,#35622)) ;
#14864=EDGE_LOOP('',(#35623,#35624,#35625,#35626)) ;
#14865=EDGE_LOOP('',(#35627,#35628,#35629,#35630)) ;
#14866=EDGE_LOOP('',(#35631,#35632,#35633,#35634)) ;
#14867=EDGE_LOOP('',(#35635,#35636,#35637,#35638)) ;
#14868=EDGE_LOOP('',(#35639,#35640,#35641,#35642)) ;
#14869=EDGE_LOOP('',(#35643,#35644,#35645,#35646)) ;
#14870=EDGE_LOOP('',(#35647,#35648,#35649)) ;
#14871=EDGE_LOOP('',(#35650,#35651,#35652,#35653)) ;
#14872=EDGE_LOOP('',(#35654,#35655,#35656,#35657)) ;
#14873=EDGE_LOOP('',(#35658,#35659,#35660,#35661)) ;
#14874=EDGE_LOOP('',(#35662,#35663,#35664,#35665)) ;
#14875=EDGE_LOOP('',(#35666,#35667,#35668,#35669)) ;
#14876=EDGE_LOOP('',(#35670,#35671,#35672,#35673)) ;
#14877=EDGE_LOOP('',(#35674,#35675,#35676,#35677)) ;
#14878=EDGE_LOOP('',(#35678,#35679,#35680,#35681)) ;
#14879=EDGE_LOOP('',(#35682,#35683,#35684,#35685)) ;
#14880=EDGE_LOOP('',(#35686,#35687,#35688,#35689)) ;
#14881=EDGE_LOOP('',(#35690,#35691,#35692,#35693)) ;
#14882=EDGE_LOOP('',(#35694,#35695,#35696,#35697)) ;
#14883=EDGE_LOOP('',(#35698,#35699,#35700)) ;
#14884=EDGE_LOOP('',(#35701,#35702,#35703,#35704,#35705)) ;
#14885=EDGE_LOOP('',(#35706,#35707,#35708,#35709)) ;
#14886=EDGE_LOOP('',(#35710,#35711,#35712,#35713)) ;
#14887=EDGE_LOOP('',(#35714,#35715,#35716)) ;
#14888=EDGE_LOOP('',(#35717,#35718,#35719,#35720)) ;
#14889=EDGE_LOOP('',(#35721,#35722,#35723,#35724)) ;
#14890=EDGE_LOOP('',(#35725,#35726,#35727,#35728)) ;
#14891=EDGE_LOOP('',(#35729,#35730,#35731,#35732)) ;
#14892=EDGE_LOOP('',(#35733,#35734,#35735,#35736)) ;
#14893=EDGE_LOOP('',(#35737,#35738,#35739,#35740)) ;
#14894=EDGE_LOOP('',(#35741,#35742,#35743,#35744)) ;
#14895=EDGE_LOOP('',(#35745,#35746,#35747,#35748)) ;
#14896=EDGE_LOOP('',(#35749,#35750,#35751,#35752)) ;
#14897=EDGE_LOOP('',(#35753,#35754,#35755,#35756)) ;
#14898=EDGE_LOOP('',(#35757,#35758,#35759,#35760)) ;
#14899=EDGE_LOOP('',(#35761,#35762,#35763,#35764)) ;
#14900=EDGE_LOOP('',(#35765,#35766,#35767,#35768)) ;
#14901=EDGE_LOOP('',(#35769,#35770,#35771)) ;
#14902=EDGE_LOOP('',(#35772,#35773,#35774,#35775)) ;
#14903=EDGE_LOOP('',(#35776,#35777,#35778,#35779)) ;
#14904=EDGE_LOOP('',(#35780,#35781,#35782,#35783,#35784,#35785)) ;
#14905=EDGE_LOOP('',(#35786,#35787,#35788,#35789)) ;
#14906=EDGE_LOOP('',(#35790,#35791,#35792,#35793)) ;
#14907=EDGE_LOOP('',(#35794,#35795,#35796)) ;
#14908=EDGE_LOOP('',(#35797,#35798,#35799,#35800,#35801,#35802,#35803)) ;
#14909=EDGE_LOOP('',(#35804,#35805,#35806,#35807)) ;
#14910=EDGE_LOOP('',(#35808,#35809,#35810,#35811)) ;
#14911=EDGE_LOOP('',(#35812,#35813,#35814,#35815)) ;
#14912=EDGE_LOOP('',(#35816,#35817,#35818,#35819)) ;
#14913=EDGE_LOOP('',(#35820,#35821,#35822,#35823)) ;
#14914=EDGE_LOOP('',(#35824,#35825,#35826,#35827)) ;
#14915=EDGE_LOOP('',(#35828,#35829,#35830,#35831)) ;
#14916=EDGE_LOOP('',(#35832,#35833,#35834,#35835)) ;
#14917=EDGE_LOOP('',(#35836,#35837,#35838,#35839)) ;
#14918=EDGE_LOOP('',(#35840,#35841,#35842,#35843)) ;
#14919=EDGE_LOOP('',(#35844,#35845,#35846,#35847)) ;
#14920=EDGE_LOOP('',(#35848,#35849,#35850,#35851)) ;
#14921=EDGE_LOOP('',(#35852,#35853,#35854,#35855)) ;
#14922=EDGE_LOOP('',(#35856,#35857,#35858,#35859)) ;
#14923=EDGE_LOOP('',(#35860,#35861,#35862,#35863)) ;
#14924=EDGE_LOOP('',(#35864,#35865,#35866,#35867)) ;
#14925=EDGE_LOOP('',(#35868,#35869,#35870,#35871)) ;
#14926=EDGE_LOOP('',(#35872,#35873,#35874,#35875)) ;
#14927=EDGE_LOOP('',(#35876,#35877,#35878,#35879)) ;
#14928=EDGE_LOOP('',(#35880,#35881,#35882,#35883)) ;
#14929=EDGE_LOOP('',(#35884,#35885,#35886,#35887)) ;
#14930=EDGE_LOOP('',(#35888,#35889,#35890,#35891)) ;
#14931=EDGE_LOOP('',(#35892,#35893,#35894,#35895)) ;
#14932=EDGE_LOOP('',(#35896,#35897,#35898,#35899)) ;
#14933=EDGE_LOOP('',(#35900,#35901,#35902,#35903)) ;
#14934=EDGE_LOOP('',(#35904,#35905,#35906,#35907)) ;
#14935=EDGE_LOOP('',(#35908,#35909,#35910,#35911)) ;
#14936=EDGE_LOOP('',(#35912,#35913,#35914,#35915)) ;
#14937=EDGE_LOOP('',(#35916,#35917,#35918,#35919)) ;
#14938=EDGE_LOOP('',(#35920,#35921,#35922,#35923)) ;
#14939=EDGE_LOOP('',(#35924,#35925,#35926,#35927)) ;
#14940=EDGE_LOOP('',(#35928,#35929,#35930,#35931)) ;
#14941=EDGE_LOOP('',(#35932,#35933,#35934,#35935)) ;
#14942=EDGE_LOOP('',(#35936,#35937,#35938,#35939)) ;
#14943=EDGE_LOOP('',(#35940,#35941,#35942,#35943)) ;
#14944=EDGE_LOOP('',(#35944,#35945,#35946,#35947)) ;
#14945=EDGE_LOOP('',(#35948,#35949,#35950,#35951)) ;
#14946=EDGE_LOOP('',(#35952,#35953,#35954,#35955)) ;
#14947=EDGE_LOOP('',(#35956,#35957,#35958,#35959)) ;
#14948=EDGE_LOOP('',(#35960,#35961,#35962,#35963)) ;
#14949=EDGE_LOOP('',(#35964,#35965,#35966,#35967)) ;
#14950=EDGE_LOOP('',(#35968,#35969,#35970,#35971)) ;
#14951=EDGE_LOOP('',(#35972,#35973,#35974,#35975)) ;
#14952=EDGE_LOOP('',(#35976,#35977,#35978,#35979)) ;
#14953=EDGE_LOOP('',(#35980,#35981,#35982,#35983)) ;
#14954=EDGE_LOOP('',(#35984,#35985,#35986,#35987)) ;
#14955=EDGE_LOOP('',(#35988,#35989,#35990,#35991)) ;
#14956=EDGE_LOOP('',(#35992,#35993,#35994,#35995)) ;
#14957=EDGE_LOOP('',(#35996,#35997,#35998,#35999)) ;
#14958=EDGE_LOOP('',(#36000,#36001,#36002,#36003,#36004)) ;
#14959=EDGE_LOOP('',(#36005,#36006,#36007,#36008,#36009)) ;
#14960=EDGE_LOOP('',(#36010,#36011,#36012,#36013)) ;
#14961=EDGE_LOOP('',(#36014,#36015,#36016,#36017)) ;
#14962=EDGE_LOOP('',(#36018,#36019,#36020)) ;
#14963=EDGE_LOOP('',(#36021,#36022,#36023,#36024,#36025,#36026,#36027)) ;
#14964=EDGE_LOOP('',(#36028,#36029,#36030,#36031,#36032,#36033)) ;
#14965=EDGE_LOOP('',(#36034,#36035,#36036,#36037)) ;
#14966=EDGE_LOOP('',(#36038,#36039,#36040,#36041)) ;
#14967=EDGE_LOOP('',(#36042,#36043,#36044,#36045)) ;
#14968=EDGE_LOOP('',(#36046,#36047,#36048)) ;
#14969=EDGE_LOOP('',(#36049,#36050,#36051,#36052)) ;
#14970=EDGE_LOOP('',(#36053,#36054,#36055,#36056)) ;
#14971=EDGE_LOOP('',(#36057,#36058,#36059,#36060)) ;
#14972=EDGE_LOOP('',(#36061,#36062,#36063,#36064)) ;
#14973=EDGE_LOOP('',(#36065,#36066,#36067,#36068)) ;
#14974=EDGE_LOOP('',(#36069,#36070,#36071,#36072)) ;
#14975=EDGE_LOOP('',(#36073,#36074,#36075,#36076)) ;
#14976=EDGE_LOOP('',(#36077,#36078,#36079,#36080)) ;
#14977=EDGE_LOOP('',(#36081,#36082,#36083,#36084)) ;
#14978=EDGE_LOOP('',(#36085,#36086,#36087,#36088)) ;
#14979=EDGE_LOOP('',(#36089,#36090,#36091,#36092)) ;
#14980=EDGE_LOOP('',(#36093,#36094,#36095,#36096)) ;
#14981=EDGE_LOOP('',(#36097,#36098,#36099,#36100)) ;
#14982=EDGE_LOOP('',(#36101,#36102,#36103,#36104,#36105,#36106)) ;
#14983=EDGE_LOOP('',(#36107,#36108,#36109,#36110,#36111)) ;
#14984=EDGE_LOOP('',(#36112,#36113,#36114,#36115,#36116)) ;
#14985=EDGE_LOOP('',(#36117,#36118,#36119,#36120,#36121)) ;
#14986=EDGE_LOOP('',(#36122,#36123,#36124,#36125)) ;
#14987=EDGE_LOOP('',(#36126,#36127,#36128,#36129)) ;
#14988=EDGE_LOOP('',(#36130,#36131,#36132,#36133)) ;
#14989=EDGE_LOOP('',(#36134,#36135,#36136,#36137)) ;
#14990=EDGE_LOOP('',(#36138,#36139,#36140,#36141)) ;
#14991=EDGE_LOOP('',(#36142,#36143,#36144,#36145)) ;
#14992=EDGE_LOOP('',(#36146,#36147,#36148,#36149)) ;
#14993=EDGE_LOOP('',(#36150,#36151,#36152,#36153)) ;
#14994=EDGE_LOOP('',(#36154,#36155,#36156,#36157)) ;
#14995=EDGE_LOOP('',(#36158,#36159,#36160,#36161)) ;
#14996=EDGE_LOOP('',(#36162,#36163,#36164,#36165)) ;
#14997=EDGE_LOOP('',(#36166,#36167,#36168,#36169)) ;
#14998=EDGE_LOOP('',(#36170,#36171,#36172,#36173)) ;
#14999=EDGE_LOOP('',(#36174,#36175,#36176,#36177)) ;
#15000=EDGE_LOOP('',(#36178,#36179,#36180,#36181)) ;
#15001=EDGE_LOOP('',(#36182,#36183,#36184,#36185)) ;
#15002=EDGE_LOOP('',(#36186,#36187,#36188,#36189)) ;
#15003=EDGE_LOOP('',(#36190,#36191,#36192,#36193)) ;
#15004=EDGE_LOOP('',(#36194,#36195,#36196,#36197)) ;
#15005=EDGE_LOOP('',(#36198,#36199,#36200,#36201)) ;
#15006=EDGE_LOOP('',(#36202,#36203,#36204,#36205)) ;
#15007=EDGE_LOOP('',(#36206,#36207,#36208,#36209)) ;
#15008=EDGE_LOOP('',(#36210,#36211,#36212,#36213)) ;
#15009=EDGE_LOOP('',(#36214,#36215,#36216,#36217)) ;
#15010=EDGE_LOOP('',(#36218,#36219,#36220,#36221)) ;
#15011=EDGE_LOOP('',(#36222,#36223,#36224,#36225)) ;
#15012=EDGE_LOOP('',(#36226,#36227,#36228,#36229)) ;
#15013=EDGE_LOOP('',(#36230,#36231,#36232,#36233)) ;
#15014=EDGE_LOOP('',(#36234,#36235,#36236,#36237)) ;
#15015=EDGE_LOOP('',(#36238,#36239,#36240,#36241)) ;
#15016=EDGE_LOOP('',(#36242)) ;
#15017=EDGE_LOOP('',(#36243)) ;
#15018=EDGE_LOOP('',(#36244,#36245,#36246,#36247,#36248)) ;
#15019=EDGE_LOOP('',(#36249,#36250,#36251,#36252,#36253)) ;
#15020=EDGE_LOOP('',(#36254,#36255,#36256,#36257,#36258)) ;
#15021=EDGE_LOOP('',(#36259,#36260,#36261,#36262,#36263)) ;
#15022=EDGE_LOOP('',(#36264,#36265,#36266,#36267,#36268)) ;
#15023=EDGE_LOOP('',(#36269,#36270,#36271,#36272,#36273)) ;
#15024=EDGE_LOOP('',(#36274)) ;
#15025=EDGE_LOOP('',(#36275)) ;
#15026=EDGE_LOOP('',(#36276,#36277,#36278,#36279)) ;
#15027=EDGE_LOOP('',(#36280,#36281,#36282,#36283)) ;
#15028=EDGE_LOOP('',(#36284,#36285,#36286,#36287,#36288)) ;
#15029=EDGE_LOOP('',(#36289,#36290,#36291,#36292,#36293)) ;
#15030=EDGE_LOOP('',(#36294,#36295,#36296,#36297)) ;
#15031=EDGE_LOOP('',(#36298)) ;
#15032=EDGE_LOOP('',(#36299)) ;
#15033=EDGE_LOOP('',(#36300,#36301,#36302,#36303,#36304)) ;
#15034=EDGE_LOOP('',(#36305,#36306,#36307,#36308,#36309)) ;
#15035=EDGE_LOOP('',(#36310,#36311,#36312,#36313,#36314)) ;
#15036=EDGE_LOOP('',(#36315,#36316,#36317,#36318,#36319)) ;
#15037=EDGE_LOOP('',(#36320)) ;
#15038=EDGE_LOOP('',(#36321)) ;
#15039=EDGE_LOOP('',(#36322,#36323,#36324,#36325)) ;
#15040=EDGE_LOOP('',(#36326,#36327,#36328,#36329)) ;
#15041=EDGE_LOOP('',(#36330,#36331,#36332,#36333)) ;
#15042=EDGE_LOOP('',(#36334,#36335,#36336,#36337)) ;
#15043=EDGE_LOOP('',(#36338,#36339,#36340,#36341)) ;
#15044=EDGE_LOOP('',(#36342,#36343,#36344,#36345)) ;
#15045=EDGE_LOOP('',(#36346,#36347,#36348,#36349)) ;
#15046=EDGE_LOOP('',(#36350,#36351,#36352,#36353)) ;
#15047=EDGE_LOOP('',(#36354,#36355,#36356)) ;
#15048=EDGE_LOOP('',(#36357,#36358,#36359,#36360,#36361)) ;
#15049=EDGE_LOOP('',(#36362,#36363,#36364,#36365,#36366)) ;
#15050=EDGE_LOOP('',(#36367,#36368,#36369,#36370,#36371)) ;
#15051=EDGE_LOOP('',(#36372,#36373,#36374,#36375,#36376)) ;
#15052=EDGE_LOOP('',(#36377,#36378,#36379,#36380)) ;
#15053=EDGE_LOOP('',(#36381,#36382,#36383,#36384)) ;
#15054=EDGE_LOOP('',(#36385,#36386,#36387,#36388)) ;
#15055=EDGE_LOOP('',(#36389,#36390,#36391,#36392,#36393)) ;
#15056=EDGE_LOOP('',(#36394,#36395,#36396,#36397,#36398,#36399,#36400)) ;
#15057=EDGE_LOOP('',(#36401,#36402,#36403,#36404,#36405)) ;
#15058=EDGE_LOOP('',(#36406,#36407,#36408,#36409)) ;
#15059=EDGE_LOOP('',(#36410,#36411,#36412,#36413)) ;
#15060=EDGE_LOOP('',(#36414,#36415,#36416,#36417)) ;
#15061=EDGE_LOOP('',(#36418,#36419,#36420,#36421)) ;
#15062=EDGE_LOOP('',(#36422,#36423,#36424,#36425)) ;
#15063=EDGE_LOOP('',(#36426,#36427,#36428,#36429)) ;
#15064=EDGE_LOOP('',(#36430,#36431,#36432,#36433)) ;
#15065=EDGE_LOOP('',(#36434,#36435,#36436)) ;
#15066=EDGE_LOOP('',(#36437,#36438,#36439,#36440)) ;
#15067=EDGE_LOOP('',(#36441,#36442,#36443,#36444)) ;
#15068=EDGE_LOOP('',(#36445,#36446,#36447)) ;
#15069=EDGE_LOOP('',(#36448,#36449,#36450,#36451)) ;
#15070=EDGE_LOOP('',(#36452,#36453,#36454,#36455)) ;
#15071=EDGE_LOOP('',(#36456,#36457,#36458)) ;
#15072=EDGE_LOOP('',(#36459,#36460,#36461,#36462)) ;
#15073=EDGE_LOOP('',(#36463,#36464,#36465,#36466,#36467)) ;
#15074=EDGE_LOOP('',(#36468,#36469,#36470,#36471)) ;
#15075=EDGE_LOOP('',(#36472,#36473,#36474,#36475,#36476,#36477)) ;
#15076=EDGE_LOOP('',(#36478,#36479,#36480,#36481,#36482)) ;
#15077=EDGE_LOOP('',(#36483,#36484,#36485,#36486)) ;
#15078=EDGE_LOOP('',(#36487,#36488,#36489,#36490,#36491)) ;
#15079=EDGE_LOOP('',(#36492,#36493,#36494,#36495,#36496)) ;
#15080=EDGE_LOOP('',(#36497,#36498,#36499,#36500)) ;
#15081=EDGE_LOOP('',(#36501,#36502,#36503,#36504)) ;
#15082=EDGE_LOOP('',(#36505,#36506,#36507,#36508,#36509,#36510,#36511)) ;
#15083=EDGE_LOOP('',(#36512,#36513,#36514,#36515)) ;
#15084=EDGE_LOOP('',(#36516,#36517,#36518,#36519,#36520,#36521)) ;
#15085=EDGE_LOOP('',(#36522,#36523,#36524,#36525)) ;
#15086=EDGE_LOOP('',(#36526,#36527,#36528,#36529)) ;
#15087=EDGE_LOOP('',(#36530,#36531,#36532,#36533)) ;
#15088=EDGE_LOOP('',(#36534,#36535,#36536,#36537,#36538,#36539)) ;
#15089=EDGE_LOOP('',(#36540,#36541,#36542,#36543)) ;
#15090=EDGE_LOOP('',(#36544,#36545,#36546,#36547,#36548)) ;
#15091=EDGE_LOOP('',(#36549,#36550,#36551,#36552,#36553)) ;
#15092=EDGE_LOOP('',(#36554,#36555,#36556,#36557,#36558)) ;
#15093=EDGE_LOOP('',(#36559,#36560,#36561)) ;
#15094=EDGE_LOOP('',(#36562,#36563,#36564)) ;
#15095=EDGE_LOOP('',(#36565,#36566,#36567)) ;
#15096=EDGE_LOOP('',(#36568,#36569,#36570)) ;
#15097=EDGE_LOOP('',(#36571,#36572,#36573)) ;
#15098=EDGE_LOOP('',(#36574,#36575,#36576)) ;
#15099=EDGE_LOOP('',(#36577,#36578,#36579,#36580)) ;
#15100=EDGE_LOOP('',(#36581,#36582,#36583,#36584)) ;
#15101=EDGE_LOOP('',(#36585,#36586,#36587,#36588)) ;
#15102=EDGE_LOOP('',(#36589,#36590,#36591,#36592)) ;
#15103=EDGE_LOOP('',(#36593,#36594,#36595,#36596)) ;
#15104=EDGE_LOOP('',(#36597,#36598,#36599)) ;
#17504=CIRCLE('',#50179,0.119999488241585) ;
#17505=CIRCLE('',#50181,0.120001966232961) ;
#17506=CIRCLE('',#50232,0.120002766430327) ;
#17507=CIRCLE('',#50242,0.119999998071627) ;
#17508=CIRCLE('',#50252,2.6) ;
#17509=CIRCLE('',#50253,2.6) ;
#17510=CIRCLE('',#50256,0.5) ;
#17511=CIRCLE('',#50257,0.5) ;
#17512=CIRCLE('',#50258,0.200000000000031) ;
#17513=CIRCLE('',#50259,0.199999999999996) ;
#17514=CIRCLE('',#50260,0.5) ;
#17515=CIRCLE('',#50261,0.7) ;
#17516=CIRCLE('',#50262,3.9) ;
#17517=CIRCLE('',#50263,3.9) ;
#17518=CIRCLE('',#50264,3.9) ;
#17519=CIRCLE('',#50265,0.7) ;
#17520=CIRCLE('',#50266,0.5) ;
#17521=CIRCLE('',#50267,0.500000000000023) ;
#17522=CIRCLE('',#50268,2.59999999999999) ;
#17523=CIRCLE('',#50269,2.59999999999996) ;
#17524=CIRCLE('',#50270,0.500000000000005) ;
#17525=CIRCLE('',#50271,0.5) ;
#17526=CIRCLE('',#50272,0.7) ;
#17527=CIRCLE('',#50273,0.200000000000031) ;
#17528=CIRCLE('',#50274,0.199999999999996) ;
#17529=CIRCLE('',#50275,0.200000000000031) ;
#17530=CIRCLE('',#50276,0.200000000000031) ;
#17531=CIRCLE('',#50277,0.199999999999996) ;
#17532=CIRCLE('',#50278,0.199999999999996) ;
#17533=CIRCLE('',#50279,0.200000000000031) ;
#17534=CIRCLE('',#50280,0.199999999999969) ;
#17535=CIRCLE('',#50281,0.199999999999978) ;
#17536=CIRCLE('',#50282,0.199999999999969) ;
#17537=CIRCLE('',#50283,0.200000000000031) ;
#17538=CIRCLE('',#50284,0.199999999999996) ;
#17539=CIRCLE('',#50285,0.200000000000031) ;
#17540=CIRCLE('',#50286,0.200000000000031) ;
#17541=CIRCLE('',#50287,0.199999999999996) ;
#17542=CIRCLE('',#50288,0.199999999999996) ;
#17543=CIRCLE('',#50289,0.200000000000031) ;
#17544=CIRCLE('',#50290,0.199999999999996) ;
#17545=CIRCLE('',#50291,0.2) ;
#17546=CIRCLE('',#50292,0.200000000000031) ;
#17547=CIRCLE('',#50293,0.199999999999996) ;
#17548=CIRCLE('',#50294,0.199999999999996) ;
#17549=CIRCLE('',#50295,0.200000000000031) ;
#17550=CIRCLE('',#50296,0.199999999999996) ;
#17551=CIRCLE('',#50297,0.200000000000001) ;
#17552=CIRCLE('',#50298,0.199999999999996) ;
#17553=CIRCLE('',#50299,0.199999999999969) ;
#17554=CIRCLE('',#50300,0.200000000000031) ;
#17555=CIRCLE('',#50301,2.6) ;
#17556=CIRCLE('',#50302,0.200000000000031) ;
#17557=CIRCLE('',#50303,0.199999999999929) ;
#17558=CIRCLE('',#50304,0.199999999999973) ;
#17559=CIRCLE('',#50305,0.199999999999966) ;
#17560=CIRCLE('',#50306,0.200000000000031) ;
#17561=CIRCLE('',#50307,4.06491106406736) ;
#17562=CIRCLE('',#50308,4.06491106406735) ;
#17563=CIRCLE('',#50309,0.199999999999957) ;
#17564=CIRCLE('',#50310,0.199999999999969) ;
#17565=CIRCLE('',#50311,0.199999999999969) ;
#17566=CIRCLE('',#50312,0.199999999999996) ;
#17567=CIRCLE('',#50313,4.06491106406736) ;
#17568=CIRCLE('',#50314,2.1) ;
#17569=CIRCLE('',#50315,0.200000000000031) ;
#17570=CIRCLE('',#50316,0.199999999999996) ;
#17571=CIRCLE('',#50317,0.200000000000031) ;
#17572=CIRCLE('',#50318,0.199999999999996) ;
#17573=CIRCLE('',#50319,0.200000000000031) ;
#17574=CIRCLE('',#50320,0.199999999999996) ;
#17575=CIRCLE('',#50321,0.200000000000031) ;
#17576=CIRCLE('',#50322,0.200000000000031) ;
#17577=CIRCLE('',#50323,0.199999999999996) ;
#17578=CIRCLE('',#50324,0.199999999999996) ;
#17579=CIRCLE('',#50350,2.) ;
#17580=CIRCLE('',#50351,0.1) ;
#17581=CIRCLE('',#50352,2.1) ;
#17582=CIRCLE('',#50353,2.) ;
#17583=CIRCLE('',#50355,2.89999999999999) ;
#17584=CIRCLE('',#50357,2.) ;
#17585=CIRCLE('',#50359,2.99999999999999) ;
#17586=CIRCLE('',#50360,0.1) ;
#17587=CIRCLE('',#50362,2.99999999999999) ;
#17588=CIRCLE('',#50364,3.09999999999999) ;
#17589=CIRCLE('',#50365,0.1) ;
#17590=CIRCLE('',#50367,0.2) ;
#17591=CIRCLE('',#50368,0.2) ;
#17592=CIRCLE('',#50369,0.2) ;
#17593=CIRCLE('',#50370,0.2) ;
#17594=CIRCLE('',#50375,0.7) ;
#17595=CIRCLE('',#50376,0.5) ;
#17596=CIRCLE('',#50377,0.500000000000005) ;
#17597=CIRCLE('',#50378,2.59999999999996) ;
#17598=CIRCLE('',#50379,2.59999999999999) ;
#17599=CIRCLE('',#50380,0.500000000000023) ;
#17600=CIRCLE('',#50381,0.5) ;
#17601=CIRCLE('',#50382,0.7) ;
#17602=CIRCLE('',#50383,3.9) ;
#17603=CIRCLE('',#50384,3.9) ;
#17604=CIRCLE('',#50385,3.9) ;
#17605=CIRCLE('',#50386,0.7) ;
#17606=CIRCLE('',#50387,0.5) ;
#17607=CIRCLE('',#50388,0.5) ;
#17608=CIRCLE('',#50389,0.5) ;
#17609=CIRCLE('',#50390,4.) ;
#17610=CIRCLE('',#50391,0.2) ;
#17611=CIRCLE('',#50392,0.2) ;
#17612=CIRCLE('',#50393,0.2) ;
#17613=CIRCLE('',#50394,0.2) ;
#17614=CIRCLE('',#50395,0.2) ;
#17615=CIRCLE('',#50396,0.2) ;
#17616=CIRCLE('',#50397,2.6) ;
#17617=CIRCLE('',#50398,2.5) ;
#17618=CIRCLE('',#50399,0.200000000000067) ;
#17619=CIRCLE('',#50400,0.2) ;
#17620=CIRCLE('',#50401,0.2) ;
#17621=CIRCLE('',#50402,0.2) ;
#17622=CIRCLE('',#50403,0.2) ;
#17623=CIRCLE('',#50404,0.199999999999996) ;
#17624=CIRCLE('',#50405,2.) ;
#17625=CIRCLE('',#50406,0.1) ;
#17626=CIRCLE('',#50407,0.1) ;
#17627=CIRCLE('',#50408,0.1) ;
#17628=CIRCLE('',#50409,0.1) ;
#17629=CIRCLE('',#50410,0.1) ;
#17630=CIRCLE('',#50411,0.1) ;
#17631=CIRCLE('',#50412,0.199999999999991) ;
#17632=CIRCLE('',#50413,0.200000000000031) ;
#17633=CIRCLE('',#50414,0.199999999999996) ;
#17634=CIRCLE('',#50415,0.200000000000031) ;
#17635=CIRCLE('',#50416,0.2) ;
#17636=CIRCLE('',#50417,0.2) ;
#17637=CIRCLE('',#50418,0.2) ;
#17638=CIRCLE('',#50419,0.2) ;
#17639=CIRCLE('',#50420,0.2) ;
#17640=CIRCLE('',#50421,0.200000000000067) ;
#17641=CIRCLE('',#50422,0.2) ;
#17642=CIRCLE('',#50423,0.2) ;
#17643=CIRCLE('',#50424,0.2) ;
#17644=CIRCLE('',#50425,0.2) ;
#17645=CIRCLE('',#50426,0.2) ;
#17646=CIRCLE('',#50427,0.2) ;
#17647=CIRCLE('',#50428,0.2) ;
#17648=CIRCLE('',#50429,0.2) ;
#17649=CIRCLE('',#50430,0.2) ;
#17650=CIRCLE('',#50431,0.2) ;
#17651=CIRCLE('',#50432,0.2) ;
#17652=CIRCLE('',#50433,0.2) ;
#17653=CIRCLE('',#50434,0.2) ;
#17654=CIRCLE('',#50435,0.2) ;
#17655=CIRCLE('',#50437,0.0999999999999934) ;
#17656=CIRCLE('',#50438,0.399999999999996) ;
#17657=CIRCLE('',#50439,0.1) ;
#17658=CIRCLE('',#50440,0.5) ;
#17659=CIRCLE('',#50442,0.100000000000002) ;
#17660=CIRCLE('',#50444,0.100000000000005) ;
#17661=CIRCLE('',#50445,1.9) ;
#17662=CIRCLE('',#50446,2.) ;
#17663=CIRCLE('',#50448,0.0999999999999979) ;
#17664=CIRCLE('',#50450,0.0999999999999979) ;
#17665=CIRCLE('',#50451,1.9) ;
#17666=CIRCLE('',#50452,2.) ;
#17667=CIRCLE('',#50454,0.100000000000002) ;
#17668=CIRCLE('',#50456,0.100000000000007) ;
#17669=CIRCLE('',#50457,2.7) ;
#17670=CIRCLE('',#50458,2.6) ;
#17671=CIRCLE('',#50460,0.0999999999999979) ;
#17672=CIRCLE('',#50462,0.0999999999999979) ;
#17673=CIRCLE('',#50463,1.9) ;
#17674=CIRCLE('',#50464,2.) ;
#17675=CIRCLE('',#50466,0.0999999999999956) ;
#17676=CIRCLE('',#50468,0.0999999999999979) ;
#17677=CIRCLE('',#50469,1.9) ;
#17678=CIRCLE('',#50470,2.) ;
#17679=CIRCLE('',#50472,0.0999999999999979) ;
#17680=CIRCLE('',#50474,0.5) ;
#17681=CIRCLE('',#50475,0.1) ;
#17682=CIRCLE('',#50476,0.400000000000027) ;
#17683=CIRCLE('',#50478,1.1) ;
#17684=CIRCLE('',#50480,2.) ;
#17685=CIRCLE('',#50483,2.) ;
#17686=CIRCLE('',#50486,2.6) ;
#17687=CIRCLE('',#50489,2.) ;
#17688=CIRCLE('',#50492,2.) ;
#17689=CIRCLE('',#50494,1.1) ;
#17690=CIRCLE('',#50496,1.) ;
#17691=CIRCLE('',#50497,3.) ;
#17692=CIRCLE('',#50499,3.) ;
#17693=CIRCLE('',#50501,0.12) ;
#17694=CIRCLE('',#50502,2.88) ;
#17695=CIRCLE('',#50504,2.12) ;
#17696=CIRCLE('',#50506,2.) ;
#17697=CIRCLE('',#50507,0.12) ;
#17698=CIRCLE('',#50508,2.) ;
#17699=CIRCLE('',#50510,2.) ;
#17700=CIRCLE('',#50512,1.97000000000001) ;
#17701=CIRCLE('',#50513,0.12) ;
#17702=CIRCLE('',#50514,1.85) ;
#17703=CIRCLE('',#50515,1.85) ;
#17704=CIRCLE('',#50517,1.85) ;
#17705=CIRCLE('',#50518,1.85) ;
#17706=CIRCLE('',#50523,1.97000000000001) ;
#17707=CIRCLE('',#50524,0.12) ;
#17708=CIRCLE('',#50527,1.97) ;
#17709=CIRCLE('',#50528,0.12) ;
#17710=CIRCLE('',#50529,1.85) ;
#17711=CIRCLE('',#50530,1.85) ;
#17712=CIRCLE('',#50532,1.85) ;
#17713=CIRCLE('',#50533,1.85) ;
#17714=CIRCLE('',#50538,1.97) ;
#17715=CIRCLE('',#50539,0.12) ;
#17716=CIRCLE('',#50542,0.100000000000002) ;
#17717=CIRCLE('',#50543,1.9) ;
#17718=CIRCLE('',#50544,0.100000000000016) ;
#17719=CIRCLE('',#50546,0.100000000000051) ;
#17720=CIRCLE('',#50548,0.100000000000016) ;
#17721=CIRCLE('',#50549,2.7) ;
#17722=CIRCLE('',#50551,0.100000000000051) ;
#17723=CIRCLE('',#50553,0.100000000000016) ;
#17724=CIRCLE('',#50554,1.9) ;
#17725=CIRCLE('',#50556,1.9) ;
#17726=CIRCLE('',#50557,1.9) ;
#17727=CIRCLE('',#50559,0.100000000000016) ;
#17728=CIRCLE('',#50567,0.100000000000016) ;
#17729=CIRCLE('',#50569,0.4) ;
#17730=CIRCLE('',#50570,0.400000000000023) ;
#17731=CIRCLE('',#50572,0.399999999999998) ;
#17732=CIRCLE('',#50574,0.399999999999988) ;
#17733=CIRCLE('',#50575,0.4) ;
#17734=CIRCLE('',#50578,0.0999999999999979) ;
#17735=CIRCLE('',#50580,0.100000000000016) ;
#17736=CIRCLE('',#50581,0.1) ;
#17737=CIRCLE('',#50582,0.100000000000002) ;
#17738=CIRCLE('',#50584,0.0999999999999801) ;
#17739=CIRCLE('',#50586,0.0999999999999785) ;
#17740=CIRCLE('',#50587,0.1) ;
#17741=CIRCLE('',#50589,0.1) ;
#17742=CIRCLE('',#50593,0.0999999999999979) ;
#17743=CIRCLE('',#50594,0.100000000000016) ;
#17744=CIRCLE('',#50595,0.0999999999999979) ;
#17745=CIRCLE('',#50597,0.0999999999999979) ;
#17746=CIRCLE('',#50599,0.1) ;
#17747=CIRCLE('',#50600,0.100000000000016) ;
#17748=CIRCLE('',#50602,0.0999999999999979) ;
#17749=CIRCLE('',#50603,0.0999999999999973) ;
#17750=CIRCLE('',#50604,0.0999999999999973) ;
#17751=CIRCLE('',#50607,0.100000000000016) ;
#17752=CIRCLE('',#50608,0.0999999999999979) ;
#17753=CIRCLE('',#50609,0.0999999999999934) ;
#17754=CIRCLE('',#50611,0.100000000000016) ;
#17755=CIRCLE('',#50612,0.0999999999999934) ;
#17756=CIRCLE('',#50613,0.0999999999999979) ;
#17757=CIRCLE('',#50617,0.100000000000016) ;
#17758=CIRCLE('',#50618,0.1) ;
#17759=CIRCLE('',#50619,0.2) ;
#17760=CIRCLE('',#50622,0.0999999999999801) ;
#17761=CIRCLE('',#50624,0.1) ;
#17762=CIRCLE('',#50625,0.2) ;
#17763=CIRCLE('',#50627,0.0999999999999979) ;
#17764=CIRCLE('',#50629,0.0999999999999973) ;
#17765=CIRCLE('',#50630,0.0999999999999973) ;
#17766=CIRCLE('',#50632,0.100000000000016) ;
#17767=CIRCLE('',#50635,0.100000000000016) ;
#17768=CIRCLE('',#50637,0.0999999999999973) ;
#17769=CIRCLE('',#50640,0.0999999999999979) ;
#17770=CIRCLE('',#50641,0.1) ;
#17771=CIRCLE('',#50642,0.2) ;
#17772=CIRCLE('',#50644,0.0999999999999979) ;
#17773=CIRCLE('',#50650,0.0999999999999979) ;
#17774=CIRCLE('',#50654,0.100000000000007) ;
#17775=CIRCLE('',#50656,0.1) ;
#17776=CIRCLE('',#50657,0.2) ;
#17777=CIRCLE('',#50662,0.100000000000016) ;
#17778=CIRCLE('',#50663,0.1) ;
#17779=CIRCLE('',#50665,0.100000000000026) ;
#17780=CIRCLE('',#50666,0.1) ;
#17781=CIRCLE('',#50668,0.0999999999999973) ;
#17782=CIRCLE('',#50670,0.100000000000002) ;
#17783=CIRCLE('',#50671,0.1) ;
#17784=CIRCLE('',#50673,0.0999999999999934) ;
#17785=CIRCLE('',#50675,0.1) ;
#17786=CIRCLE('',#50677,0.1) ;
#17787=CIRCLE('',#50680,0.100000000000016) ;
#17788=CIRCLE('',#50683,0.0999999999999753) ;
#17789=CIRCLE('',#50686,0.0999999999999979) ;
#17790=CIRCLE('',#50689,0.099999999999991) ;
#17791=CIRCLE('',#50692,0.100000000000016) ;
#17792=CIRCLE('',#50695,0.0999999999999979) ;
#17793=CIRCLE('',#50696,0.100000000000016) ;
#17794=CIRCLE('',#50698,0.0999999999999934) ;
#17795=CIRCLE('',#50699,0.1) ;
#17796=CIRCLE('',#50701,0.0999999999999934) ;
#17797=CIRCLE('',#50703,0.0999999999999934) ;
#17798=CIRCLE('',#50704,0.1) ;
#17799=CIRCLE('',#50706,0.0999999999999979) ;
#17800=CIRCLE('',#50708,0.0999999999999934) ;
#17801=CIRCLE('',#50709,0.1) ;
#17802=CIRCLE('',#50711,0.0999999999999934) ;
#17803=CIRCLE('',#50713,0.0999999999999934) ;
#17804=CIRCLE('',#50714,0.1) ;
#17805=CIRCLE('',#50716,0.0999999999999979) ;
#17806=CIRCLE('',#50718,0.0999999999999934) ;
#17807=CIRCLE('',#50719,0.0999999999999979) ;
#17808=CIRCLE('',#50721,0.0999999999999934) ;
#17809=CIRCLE('',#50722,0.1) ;
#17810=CIRCLE('',#50724,0.0999999999999979) ;
#17811=CIRCLE('',#50726,0.0999999999999934) ;
#17812=CIRCLE('',#50727,0.1) ;
#17813=CIRCLE('',#50729,0.0999999999999934) ;
#17814=CIRCLE('',#50731,0.0999999999999973) ;
#17815=CIRCLE('',#50733,0.100000000000004) ;
#17816=CIRCLE('',#50735,0.100000000000016) ;
#17817=CIRCLE('',#50738,0.0999999999999979) ;
#17818=CIRCLE('',#50741,0.100000000000016) ;
#17819=CIRCLE('',#50744,0.0999999999999979) ;
#17820=CIRCLE('',#50747,0.100000000000016) ;
#17821=CIRCLE('',#50748,0.0999999999999979) ;
#17822=CIRCLE('',#50749,0.0999999999999934) ;
#17823=CIRCLE('',#50751,0.100000000000051) ;
#17824=CIRCLE('',#50752,0.100000000000002) ;
#17825=CIRCLE('',#50753,0.0999999999999979) ;
#17826=CIRCLE('',#50755,0.100000000000016) ;
#17827=CIRCLE('',#50757,0.100000000000029) ;
#17828=CIRCLE('',#50758,0.1) ;
#17829=CIRCLE('',#50760,0.099999999999991) ;
#17830=CIRCLE('',#50762,0.100000000000007) ;
#17831=CIRCLE('',#50763,0.1) ;
#17832=CIRCLE('',#50765,0.100000000000007) ;
#17833=CIRCLE('',#50767,0.100000000000022) ;
#17834=CIRCLE('',#50768,0.1) ;
#17835=CIRCLE('',#50770,0.099999999999991) ;
#17836=CIRCLE('',#50772,0.0999999999999801) ;
#17837=CIRCLE('',#50773,0.1) ;
#17838=CIRCLE('',#50776,0.1) ;
#17839=CIRCLE('',#50778,0.0999999999999979) ;
#17840=CIRCLE('',#50782,0.100000000000016) ;
#17841=CIRCLE('',#50786,0.1) ;
#17842=CIRCLE('',#50789,0.0999999999999979) ;
#17843=CIRCLE('',#50790,0.100000000000016) ;
#17844=CIRCLE('',#50791,0.1) ;
#17845=CIRCLE('',#50793,0.0999999999999979) ;
#17846=CIRCLE('',#50795,0.0999999999999979) ;
#17847=CIRCLE('',#50796,0.0999999999999979) ;
#17848=CIRCLE('',#50798,0.0999999999999979) ;
#17849=CIRCLE('',#50799,0.1) ;
#17850=CIRCLE('',#50801,0.0999999999999979) ;
#17851=CIRCLE('',#50803,0.0999999999999979) ;
#17852=CIRCLE('',#50804,0.1) ;
#17853=CIRCLE('',#50806,0.0999999999999979) ;
#17854=CIRCLE('',#50808,0.0999999999999973) ;
#17855=CIRCLE('',#50810,0.0999999999999979) ;
#17856=CIRCLE('',#50811,0.100000000000016) ;
#17857=CIRCLE('',#50813,0.1) ;
#17858=CIRCLE('',#50814,0.100000000000051) ;
#17859=CIRCLE('',#50816,0.100000000000004) ;
#17860=CIRCLE('',#50819,0.0999999999999979) ;
#17861=CIRCLE('',#50822,0.100000000000016) ;
#17862=CIRCLE('',#50825,0.0999999999999979) ;
#17863=CIRCLE('',#50828,0.100000000000016) ;
#17864=CIRCLE('',#50831,0.0999999999999979) ;
#17865=CIRCLE('',#50832,0.100000000000016) ;
#17866=CIRCLE('',#50833,0.1) ;
#17867=CIRCLE('',#50835,0.0999999999999979) ;
#17868=CIRCLE('',#50837,0.0999999999999979) ;
#17869=CIRCLE('',#50838,0.0999999999999979) ;
#17870=CIRCLE('',#50840,0.0999999999999979) ;
#17871=CIRCLE('',#50841,0.1) ;
#17872=CIRCLE('',#50843,0.0999999999999979) ;
#17873=CIRCLE('',#50845,0.0999999999999979) ;
#17874=CIRCLE('',#50846,0.1) ;
#17875=CIRCLE('',#50848,0.0999999999999979) ;
#17876=CIRCLE('',#50850,0.0999999999999973) ;
#17877=CIRCLE('',#50852,0.0999999999999979) ;
#17878=CIRCLE('',#50853,0.100000000000016) ;
#17879=CIRCLE('',#50855,0.1) ;
#17880=CIRCLE('',#50856,0.100000000000051) ;
#17881=CIRCLE('',#50858,0.0999999999999973) ;
#17882=CIRCLE('',#50861,0.0999999999999979) ;
#17883=CIRCLE('',#50864,0.100000000000016) ;
#17884=CIRCLE('',#50867,0.0999999999999979) ;
#17885=CIRCLE('',#50870,0.100000000000016) ;
#17886=CIRCLE('',#50873,0.100000000000002) ;
#17887=CIRCLE('',#50875,0.100000000000002) ;
#17888=CIRCLE('',#50876,0.100000000000016) ;
#17889=CIRCLE('',#50878,0.1) ;
#17890=CIRCLE('',#50879,0.100000000000051) ;
#17891=CIRCLE('',#50884,0.100000000000016) ;
#17892=CIRCLE('',#50885,0.1) ;
#17893=CIRCLE('',#50888,0.100000000000016) ;
#17894=CIRCLE('',#50890,0.100000000000022) ;
#17895=CIRCLE('',#50891,0.1) ;
#17896=CIRCLE('',#50893,0.0999999999999785) ;
#17897=CIRCLE('',#50895,0.100000000000007) ;
#17898=CIRCLE('',#50896,0.1) ;
#17899=CIRCLE('',#50898,0.0999999999999979) ;
#17900=CIRCLE('',#50900,0.0999999999999973) ;
#17901=CIRCLE('',#50901,0.1) ;
#17902=CIRCLE('',#50903,0.099999999999991) ;
#17903=CIRCLE('',#50905,0.0999999999999801) ;
#17904=CIRCLE('',#50906,0.1) ;
#17905=CIRCLE('',#50910,0.0999999999999722) ;
#17906=CIRCLE('',#50913,0.0999999999999979) ;
#17907=CIRCLE('',#50916,0.099999999999991) ;
#17908=CIRCLE('',#50919,0.100000000000016) ;
#17909=CIRCLE('',#50923,0.100000000000016) ;
#17910=CIRCLE('',#50924,0.100000000000016) ;
#17911=CIRCLE('',#50925,0.1) ;
#17912=CIRCLE('',#50928,0.0999999999999979) ;
#17913=CIRCLE('',#50929,0.0999999999999934) ;
#17914=CIRCLE('',#50932,0.100000000000016) ;
#17915=CIRCLE('',#50933,0.0999999999999979) ;
#17916=CIRCLE('',#50934,0.0999999999999979) ;
#17917=CIRCLE('',#50936,0.0999999999999979) ;
#17918=CIRCLE('',#50937,0.100000000000016) ;
#17919=CIRCLE('',#50938,0.0999999999999979) ;
#17920=CIRCLE('',#50943,0.100000000000051) ;
#17921=CIRCLE('',#50944,0.0999999999999979) ;
#17922=CIRCLE('',#50945,0.0999999999999979) ;
#17923=CIRCLE('',#50953,0.0999999999999801) ;
#17924=CIRCLE('',#50954,0.1) ;
#17925=CIRCLE('',#50955,0.100000000000051) ;
#17926=CIRCLE('',#50957,0.100000000000016) ;
#17927=CIRCLE('',#50958,0.100000000000016) ;
#17928=CIRCLE('',#50959,0.1) ;
#17929=CIRCLE('',#50962,0.0999999999999979) ;
#17930=CIRCLE('',#50963,0.0999999999999979) ;
#17931=CIRCLE('',#50965,0.100000000000016) ;
#17932=CIRCLE('',#50966,0.0999999999999979) ;
#17933=CIRCLE('',#50969,0.0999999999999979) ;
#17934=CIRCLE('',#50970,0.100000000000016) ;
#17935=CIRCLE('',#50972,0.0999999999999979) ;
#17936=CIRCLE('',#50973,0.0999999999999979) ;
#17937=CIRCLE('',#50976,0.0999999999999979) ;
#17938=CIRCLE('',#50977,0.100000000000016) ;
#17939=CIRCLE('',#50978,0.0999999999999979) ;
#17940=CIRCLE('',#50980,0.100000000000016) ;
#17941=CIRCLE('',#50981,0.0999999999999979) ;
#17942=CIRCLE('',#50982,0.0999999999999979) ;
#17943=CIRCLE('',#50986,0.100000000000016) ;
#17944=CIRCLE('',#50987,0.0999999999999979) ;
#17945=CIRCLE('',#50988,0.0999999999999979) ;
#17946=CIRCLE('',#50990,0.0999999999999979) ;
#17947=CIRCLE('',#50991,0.100000000000016) ;
#17948=CIRCLE('',#50992,0.0999999999999979) ;
#17949=CIRCLE('',#51005,0.0999999999999801) ;
#17950=CIRCLE('',#51006,0.1) ;
#17951=CIRCLE('',#51007,0.100000000000051) ;
#17952=CIRCLE('',#51009,0.100000000000016) ;
#17953=CIRCLE('',#51010,0.100000000000016) ;
#17954=CIRCLE('',#51011,0.1) ;
#17955=CIRCLE('',#51014,0.0999999999999979) ;
#17956=CIRCLE('',#51015,0.0999999999999979) ;
#17957=CIRCLE('',#51017,0.0999999999999979) ;
#17958=CIRCLE('',#51018,0.100000000000016) ;
#17959=CIRCLE('',#51021,0.100000000000016) ;
#17960=CIRCLE('',#51022,0.0999999999999979) ;
#17961=CIRCLE('',#51025,0.0999999999999979) ;
#17962=CIRCLE('',#51026,0.100000000000016) ;
#17963=CIRCLE('',#51027,0.0999999999999979) ;
#17964=CIRCLE('',#51029,0.0999999999999979) ;
#17965=CIRCLE('',#51030,0.0999999999999979) ;
#17966=CIRCLE('',#51033,0.100000000000016) ;
#17967=CIRCLE('',#51034,0.0999999999999979) ;
#17968=CIRCLE('',#51035,0.0999999999999979) ;
#17969=CIRCLE('',#51037,0.100000000000016) ;
#17970=CIRCLE('',#51038,0.0999999999999979) ;
#17971=CIRCLE('',#51039,0.0999999999999979) ;
#17972=CIRCLE('',#51043,0.0999999999999979) ;
#17973=CIRCLE('',#51044,0.100000000000016) ;
#17974=CIRCLE('',#51045,0.0999999999999979) ;
#17975=CIRCLE('',#51057,0.100000000000016) ;
#17976=CIRCLE('',#51058,0.0999999999999979) ;
#17977=CIRCLE('',#51059,0.0999999999999979) ;
#17978=CIRCLE('',#51061,0.0999999999999979) ;
#17979=CIRCLE('',#51062,0.100000000000016) ;
#17980=CIRCLE('',#51063,0.0999999999999979) ;
#17981=CIRCLE('',#51065,0.100000000000051) ;
#17982=CIRCLE('',#51066,0.0999999999999979) ;
#17983=CIRCLE('',#51068,0.0999999999999979) ;
#17984=CIRCLE('',#51069,1.2) ;
#17985=CIRCLE('',#51071,0.0999999999999934) ;
#17986=CIRCLE('',#51073,0.0999999999999801) ;
#17987=CIRCLE('',#51074,0.6) ;
#17988=CIRCLE('',#51076,0.100000000000016) ;
#17989=CIRCLE('',#51078,0.100000000000002) ;
#17990=CIRCLE('',#51079,0.6) ;
#17991=CIRCLE('',#51083,0.100000000000016) ;
#17992=CIRCLE('',#51085,0.100000000000016) ;
#17993=CIRCLE('',#51087,0.100000000000002) ;
#17994=CIRCLE('',#51088,1.2) ;
#17995=CIRCLE('',#51090,0.100000000000002) ;
#17996=CIRCLE('',#51092,0.100000000000002) ;
#17997=CIRCLE('',#51093,0.6) ;
#17998=CIRCLE('',#51095,0.100000000000002) ;
#17999=CIRCLE('',#51097,0.100000000000002) ;
#18000=CIRCLE('',#51098,0.6) ;
#18001=CIRCLE('',#51100,0.100000000000002) ;
#18002=CIRCLE('',#51102,0.100000000000002) ;
#18003=CIRCLE('',#51103,0.600000000000005) ;
#18004=CIRCLE('',#51105,0.100000000000002) ;
#18005=CIRCLE('',#51106,2.49999999999996) ;
#18006=CIRCLE('',#51108,0.0999999999999979) ;
#18007=CIRCLE('',#51110,0.100000000000002) ;
#18008=CIRCLE('',#51111,2.49999999999999) ;
#18009=CIRCLE('',#51113,0.100000000000002) ;
#18010=CIRCLE('',#51114,0.600000000000023) ;
#18011=CIRCLE('',#51116,0.100000000000002) ;
#18012=CIRCLE('',#51118,0.100000000000002) ;
#18013=CIRCLE('',#51119,0.6) ;
#18014=CIRCLE('',#51121,0.100000000000002) ;
#18015=CIRCLE('',#51123,0.100000000000002) ;
#18016=CIRCLE('',#51124,0.6) ;
#18017=CIRCLE('',#51126,0.100000000000002) ;
#18018=CIRCLE('',#51128,0.100000000000002) ;
#18019=CIRCLE('',#51129,4.) ;
#18020=CIRCLE('',#51131,0.0999999999999934) ;
#18021=CIRCLE('',#51133,0.0999999999999979) ;
#18022=CIRCLE('',#51134,4.) ;
#18023=CIRCLE('',#51136,0.0999999999999979) ;
#18024=CIRCLE('',#51138,0.0999999999999979) ;
#18025=CIRCLE('',#51139,4.) ;
#18026=CIRCLE('',#51141,0.0999999999999979) ;
#18027=CIRCLE('',#51143,0.0999999999999979) ;
#18028=CIRCLE('',#51144,0.6) ;
#18029=CIRCLE('',#51146,0.100000000000002) ;
#18030=CIRCLE('',#51148,0.100000000000002) ;
#18031=CIRCLE('',#51149,0.6) ;
#18032=CIRCLE('',#51152,0.1000000000003) ;
#18033=CIRCLE('',#51153,0.1) ;
#18034=CIRCLE('',#51154,0.2) ;
#18035=CIRCLE('',#51158,0.0999999999999801) ;
#18036=CIRCLE('',#51160,0.1) ;
#18037=CIRCLE('',#51161,0.2) ;
#18038=CIRCLE('',#51167,0.6) ;
#18039=CIRCLE('',#51170,0.600000000000005) ;
#18040=CIRCLE('',#51172,2.49999999999996) ;
#18041=CIRCLE('',#51175,2.49999999999999) ;
#18042=CIRCLE('',#51177,0.600000000000023) ;
#18043=CIRCLE('',#51180,0.6) ;
#18044=CIRCLE('',#51183,0.6) ;
#18045=CIRCLE('',#51186,4.) ;
#18046=CIRCLE('',#51189,4.) ;
#18047=CIRCLE('',#51192,4.) ;
#18048=CIRCLE('',#51195,0.6) ;
#18049=CIRCLE('',#51198,0.6) ;
#18050=CIRCLE('',#51201,0.099999999999989) ;
#18051=CIRCLE('',#51203,0.1) ;
#18052=CIRCLE('',#51204,0.0999999999999979) ;
#18053=CIRCLE('',#51206,0.100000000000002) ;
#18054=CIRCLE('',#51207,0.9) ;
#18055=CIRCLE('',#51208,1.) ;
#18056=CIRCLE('',#51212,1.) ;
#18057=CIRCLE('',#51215,0.1) ;
#18058=CIRCLE('',#51217,0.100000000000016) ;
#18059=CIRCLE('',#51219,0.100000000000016) ;
#18060=CIRCLE('',#51220,0.9) ;
#18061=CIRCLE('',#51225,0.100000000000016) ;
#18062=CIRCLE('',#51226,0.0999999999999979) ;
#18063=CIRCLE('',#51227,0.100000000000002) ;
#18064=CIRCLE('',#51229,0.100000000000016) ;
#18065=CIRCLE('',#51230,0.0999999999999934) ;
#18066=CIRCLE('',#51231,0.0999999999999785) ;
#18067=CIRCLE('',#51234,0.0999999999999847) ;
#18068=CIRCLE('',#51235,0.0999999999999979) ;
#18069=CIRCLE('',#51236,0.0999999999999979) ;
#18070=CIRCLE('',#51239,0.0999999999999979) ;
#18071=CIRCLE('',#51240,0.100000000000002) ;
#18072=CIRCLE('',#51241,0.0999999999999847) ;
#18073=CIRCLE('',#51244,0.099999999999991) ;
#18074=CIRCLE('',#51245,0.0999999999999934) ;
#18075=CIRCLE('',#51246,0.100000000000016) ;
#18076=CIRCLE('',#51249,0.0999999999999979) ;
#18077=CIRCLE('',#51250,0.100000000000016) ;
#18078=CIRCLE('',#51251,0.0999999999999979) ;
#18079=CIRCLE('',#51264,0.0999999999999979) ;
#18080=CIRCLE('',#51265,0.0999999999999979) ;
#18081=CIRCLE('',#51266,0.100000000000016) ;
#18082=CIRCLE('',#51268,0.100000000000016) ;
#18083=CIRCLE('',#51269,0.0999999999999979) ;
#18084=CIRCLE('',#51270,0.100000000000002) ;
#18085=CIRCLE('',#51274,0.100000000000016) ;
#18086=CIRCLE('',#51275,0.0999999999999979) ;
#18087=CIRCLE('',#51276,0.100000000000002) ;
#18088=CIRCLE('',#51278,0.0999999999999979) ;
#18089=CIRCLE('',#51279,0.0999999999999979) ;
#18090=CIRCLE('',#51282,0.100000000000016) ;
#18091=CIRCLE('',#51283,0.0999999999999979) ;
#18092=CIRCLE('',#51284,0.0999999999999979) ;
#18093=CIRCLE('',#51287,0.100000000000016) ;
#18094=CIRCLE('',#51288,0.100000000000002) ;
#18095=CIRCLE('',#51291,0.100000000000002) ;
#18096=CIRCLE('',#51292,0.100000000000016) ;
#18097=CIRCLE('',#51294,0.0999999999999979) ;
#18098=CIRCLE('',#51295,0.0999999999999979) ;
#18099=CIRCLE('',#51306,0.1) ;
#18100=CIRCLE('',#51307,0.100000000000016) ;
#18101=CIRCLE('',#51309,0.100000000000016) ;
#18102=CIRCLE('',#51310,1.) ;
#18103=CIRCLE('',#51311,0.9) ;
#18104=CIRCLE('',#51315,0.1) ;
#18105=CIRCLE('',#51316,0.0999999999999979) ;
#18106=CIRCLE('',#51318,0.100000000000002) ;
#18107=CIRCLE('',#51319,0.900000000000001) ;
#18108=CIRCLE('',#51320,1.) ;
#18109=CIRCLE('',#51325,0.0999999999999979) ;
#18110=CIRCLE('',#51326,0.0999999999999785) ;
#18111=CIRCLE('',#51329,0.0999999999999979) ;
#18112=CIRCLE('',#51330,0.0999999999999979) ;
#18113=CIRCLE('',#51333,0.0999999999999934) ;
#18114=CIRCLE('',#51334,0.099999999999991) ;
#18115=CIRCLE('',#51337,0.0999999999999979) ;
#18116=CIRCLE('',#51338,0.100000000000016) ;
#18117=CIRCLE('',#51342,0.1) ;
#18118=CIRCLE('',#51343,0.0999999999999979) ;
#18119=CIRCLE('',#51345,0.100000000000007) ;
#18120=CIRCLE('',#51346,0.9) ;
#18121=CIRCLE('',#51347,1.) ;
#18122=CIRCLE('',#51351,1.) ;
#18123=CIRCLE('',#51354,0.1) ;
#18124=CIRCLE('',#51356,0.100000000000016) ;
#18125=CIRCLE('',#51358,0.100000000000016) ;
#18126=CIRCLE('',#51359,0.9) ;
#18127=CIRCLE('',#51364,0.0999999999999847) ;
#18128=CIRCLE('',#51365,0.0999999999999979) ;
#18129=CIRCLE('',#51366,0.100000000000016) ;
#18130=CIRCLE('',#51368,0.0999999999999979) ;
#18131=CIRCLE('',#51369,0.100000000000002) ;
#18132=CIRCLE('',#51370,0.099999999999991) ;
#18133=CIRCLE('',#51372,0.0999999999999847) ;
#18134=CIRCLE('',#51373,0.0999999999999934) ;
#18135=CIRCLE('',#51374,0.0999999999999979) ;
#18136=CIRCLE('',#51376,0.100000000000016) ;
#18137=CIRCLE('',#51377,0.0999999999999934) ;
#18138=CIRCLE('',#51378,0.0999999999999847) ;
#18139=CIRCLE('',#51400,0.0999999999999979) ;
#18140=CIRCLE('',#51401,0.100000000000016) ;
#18141=CIRCLE('',#51402,0.0999999999999979) ;
#18142=CIRCLE('',#51404,0.0999999999999979) ;
#18143=CIRCLE('',#51405,0.0999999999999934) ;
#18144=CIRCLE('',#51406,0.100000000000016) ;
#18145=CIRCLE('',#51408,0.100000000000016) ;
#18146=CIRCLE('',#51409,0.0999999999999979) ;
#18147=CIRCLE('',#51410,0.0999999999999979) ;
#18148=CIRCLE('',#51412,0.0999999999999979) ;
#18149=CIRCLE('',#51413,0.0999999999999934) ;
#18150=CIRCLE('',#51414,0.100000000000016) ;
#18151=CIRCLE('',#51416,0.0999999999999979) ;
#18152=CIRCLE('',#51417,0.100000000000016) ;
#18153=CIRCLE('',#51418,0.0999999999999934) ;
#18154=CIRCLE('',#51420,0.100000000000016) ;
#18155=CIRCLE('',#51421,0.0999999999999934) ;
#18156=CIRCLE('',#51422,0.0999999999999979) ;
#18157=CIRCLE('',#51424,0.0999999999999979) ;
#18158=CIRCLE('',#51425,0.100000000000016) ;
#18159=CIRCLE('',#51426,0.0999999999999979) ;
#18160=CIRCLE('',#51429,0.0999999999999934) ;
#18161=CIRCLE('',#51430,0.0999999999999979) ;
#18162=CIRCLE('',#51431,0.100000000000016) ;
#18163=CIRCLE('',#51448,0.1) ;
#18164=CIRCLE('',#51449,2.5) ;
#18165=CIRCLE('',#51451,2.5) ;
#18166=CIRCLE('',#51452,2.5) ;
#18167=CIRCLE('',#51454,0.1) ;
#18168=CIRCLE('',#51456,0.1) ;
#18169=CIRCLE('',#51457,0.100000000000016) ;
#18170=CIRCLE('',#51459,0.100000000000016) ;
#18171=CIRCLE('',#51460,1.) ;
#18172=CIRCLE('',#51461,0.900000000000001) ;
#18173=CIRCLE('',#51466,0.1) ;
#18174=CIRCLE('',#51469,0.0999999999999979) ;
#18175=CIRCLE('',#51471,0.0999999999999934) ;
#18176=CIRCLE('',#51472,0.9) ;
#18177=CIRCLE('',#51473,1.) ;
#18178=CIRCLE('',#51478,0.100000000000002) ;
#18179=CIRCLE('',#51479,0.099999999999991) ;
#18180=CIRCLE('',#51483,0.0999999999999979) ;
#18181=CIRCLE('',#51484,0.0999999999999979) ;
#18182=CIRCLE('',#51487,0.0999999999999979) ;
#18183=CIRCLE('',#51488,0.0999999999999847) ;
#18184=CIRCLE('',#51491,0.0999999999999979) ;
#18185=CIRCLE('',#51492,0.100000000000016) ;
#18186=CIRCLE('',#51495,0.100000000000002) ;
#18187=CIRCLE('',#51496,0.0999999999999979) ;
#18188=CIRCLE('',#51501,0.1) ;
#18189=CIRCLE('',#51502,2.5) ;
#18190=CIRCLE('',#51503,2.5) ;
#18191=CIRCLE('',#51506,0.1) ;
#18192=CIRCLE('',#51507,2.) ;
#18193=CIRCLE('',#51508,2.) ;
#18194=CIRCLE('',#51511,0.0999999999999979) ;
#18195=CIRCLE('',#51513,0.0999999999999847) ;
#18196=CIRCLE('',#51514,0.6) ;
#18197=CIRCLE('',#51516,0.0999999999999847) ;
#18198=CIRCLE('',#51518,0.100000000000016) ;
#18199=CIRCLE('',#51520,0.0999999999999979) ;
#18200=CIRCLE('',#51522,0.0999999999999938) ;
#18201=CIRCLE('',#51524,0.0999999999999979) ;
#18202=CIRCLE('',#51526,0.099999999999989) ;
#18203=CIRCLE('',#51528,0.100000000000029) ;
#18204=CIRCLE('',#51530,0.0999999999999979) ;
#18205=CIRCLE('',#51532,0.0999999999999979) ;
#18206=CIRCLE('',#51534,0.0999999999999847) ;
#18207=CIRCLE('',#51536,0.0999999999999847) ;
#18208=CIRCLE('',#51538,0.099999999999989) ;
#18209=CIRCLE('',#51540,0.0999999999999979) ;
#18210=CIRCLE('',#51542,0.100000000000006) ;
#18211=CIRCLE('',#51544,0.100000000000006) ;
#18212=CIRCLE('',#51546,0.100000000000022) ;
#18213=CIRCLE('',#51548,0.1) ;
#18214=CIRCLE('',#51550,0.100000000000007) ;
#18215=CIRCLE('',#51552,0.0999999999999979) ;
#18216=CIRCLE('',#51554,0.0999999999999801) ;
#18217=CIRCLE('',#51556,0.0999999999999801) ;
#18218=CIRCLE('',#51560,0.100000000000002) ;
#18219=CIRCLE('',#51561,0.6) ;
#18220=CIRCLE('',#51563,0.0999999999999934) ;
#18221=CIRCLE('',#51565,0.0999999999999979) ;
#18222=CIRCLE('',#51566,0.6) ;
#18223=CIRCLE('',#51569,0.2) ;
#18224=CIRCLE('',#51570,2.2) ;
#18225=CIRCLE('',#51572,2.6) ;
#18226=CIRCLE('',#51574,2.8) ;
#18227=CIRCLE('',#51575,0.2) ;
#18228=CIRCLE('',#51576,2.8) ;
#18229=CIRCLE('',#51578,2.8) ;
#18230=CIRCLE('',#51580,0.2) ;
#18231=CIRCLE('',#51581,2.80637980653322) ;
#18232=CIRCLE('',#51582,2.80637980653322) ;
#18233=CIRCLE('',#51584,2.8) ;
#18234=CIRCLE('',#51585,0.2) ;
#18235=CIRCLE('',#51586,2.80637980653322) ;
#18236=CIRCLE('',#51587,2.80637980653322) ;
#18237=CIRCLE('',#51589,2.8) ;
#18238=CIRCLE('',#51590,2.8) ;
#18239=CIRCLE('',#51592,0.2) ;
#18240=CIRCLE('',#51593,2.6) ;
#18241=CIRCLE('',#51595,2.2) ;
#18242=CIRCLE('',#51597,2.) ;
#18243=CIRCLE('',#51598,0.2) ;
#18244=CIRCLE('',#51600,2.) ;
#18245=CIRCLE('',#51602,2.79999999999999) ;
#18246=CIRCLE('',#51603,0.2) ;
#18247=CIRCLE('',#51604,2.80637980653321) ;
#18248=CIRCLE('',#51605,2.80637980653321) ;
#18249=CIRCLE('',#51607,2.79999999999999) ;
#18250=CIRCLE('',#51608,2.79999999999999) ;
#18251=CIRCLE('',#51610,0.2) ;
#18252=CIRCLE('',#51611,2.2) ;
#18253=CIRCLE('',#51613,2.59999999999999) ;
#18254=CIRCLE('',#51615,0.2) ;
#18255=CIRCLE('',#51617,1.3) ;
#18256=CIRCLE('',#51619,1.3) ;
#18257=CIRCLE('',#51621,1.3) ;
#18258=CIRCLE('',#51633,0.499999999999998) ;
#18259=CIRCLE('',#51638,0.500000000000007) ;
#18260=CIRCLE('',#51643,0.499999999999998) ;
#18261=CIRCLE('',#51646,0.500000000000007) ;
#18262=CIRCLE('',#51648,1.2) ;
#18263=CIRCLE('',#51649,1.20000000000002) ;
#18264=CIRCLE('',#51652,1.20000000000002) ;
#18265=CIRCLE('',#51653,1.19999999999999) ;
#18266=CIRCLE('',#51658,1.2) ;
#18267=CIRCLE('',#51659,1.20000000000002) ;
#18268=CIRCLE('',#51662,1.20000000000002) ;
#18269=CIRCLE('',#51663,1.2) ;
#18270=CIRCLE('',#51668,0.499999999999994) ;
#18271=CIRCLE('',#51670,0.499999999999998) ;
#18272=CIRCLE('',#51678,0.499999999999994) ;
#18273=CIRCLE('',#51680,0.499999999999989) ;
#20162=VERTEX_POINT('',#79248) ;
#20163=VERTEX_POINT('',#79249) ;
#20164=VERTEX_POINT('',#79260) ;
#20165=VERTEX_POINT('',#79275) ;
#20166=VERTEX_POINT('',#79364) ;
#20167=VERTEX_POINT('',#79365) ;
#20168=VERTEX_POINT('',#79372) ;
#20169=VERTEX_POINT('',#79398) ;
#20170=VERTEX_POINT('',#79471) ;
#20171=VERTEX_POINT('',#79482) ;
#20172=VERTEX_POINT('',#79542) ;
#20173=VERTEX_POINT('',#79544) ;
#20174=VERTEX_POINT('',#79548) ;
#20175=VERTEX_POINT('',#79550) ;
#20176=VERTEX_POINT('',#79606) ;
#20177=VERTEX_POINT('',#79613) ;
#20178=VERTEX_POINT('',#79727) ;
#20179=VERTEX_POINT('',#79729) ;
#20180=VERTEX_POINT('',#79733) ;
#20181=VERTEX_POINT('',#79737) ;
#20182=VERTEX_POINT('',#79750) ;
#20183=VERTEX_POINT('',#79759) ;
#20184=VERTEX_POINT('',#79760) ;
#20185=VERTEX_POINT('',#79762) ;
#20186=VERTEX_POINT('',#79771) ;
#20187=VERTEX_POINT('',#79782) ;
#20188=VERTEX_POINT('',#79793) ;
#20189=VERTEX_POINT('',#79802) ;
#20190=VERTEX_POINT('',#79804) ;
#20191=VERTEX_POINT('',#79806) ;
#20192=VERTEX_POINT('',#79808) ;
#20193=VERTEX_POINT('',#79815) ;
#20194=VERTEX_POINT('',#79824) ;
#20195=VERTEX_POINT('',#79833) ;
#20196=VERTEX_POINT('',#79842) ;
#20197=VERTEX_POINT('',#79849) ;
#20198=VERTEX_POINT('',#79858) ;
#20199=VERTEX_POINT('',#79865) ;
#20200=VERTEX_POINT('',#79867) ;
#20201=VERTEX_POINT('',#79869) ;
#20202=VERTEX_POINT('',#79873) ;
#20203=VERTEX_POINT('',#79875) ;
#20204=VERTEX_POINT('',#79900) ;
#20205=VERTEX_POINT('',#79904) ;
#20206=VERTEX_POINT('',#79968) ;
#20207=VERTEX_POINT('',#80059) ;
#20208=VERTEX_POINT('',#80149) ;
#20209=VERTEX_POINT('',#80150) ;
#20210=VERTEX_POINT('',#80222) ;
#20211=VERTEX_POINT('',#80264) ;
#20212=VERTEX_POINT('',#80265) ;
#20213=VERTEX_POINT('',#80332) ;
#20214=VERTEX_POINT('',#80336) ;
#20215=VERTEX_POINT('',#80340) ;
#20216=VERTEX_POINT('',#80385) ;
#20217=VERTEX_POINT('',#80458) ;
#20218=VERTEX_POINT('',#80573) ;
#20219=VERTEX_POINT('',#80667) ;
#20220=VERTEX_POINT('',#80728) ;
#20221=VERTEX_POINT('',#80840) ;
#20222=VERTEX_POINT('',#80842) ;
#20223=VERTEX_POINT('',#80860) ;
#20224=VERTEX_POINT('',#80869) ;
#20225=VERTEX_POINT('',#80873) ;
#20226=VERTEX_POINT('',#80877) ;
#20227=VERTEX_POINT('',#80890) ;
#20228=VERTEX_POINT('',#80908) ;
#20229=VERTEX_POINT('',#80926) ;
#20230=VERTEX_POINT('',#80972) ;
#20231=VERTEX_POINT('',#80981) ;
#20232=VERTEX_POINT('',#81024) ;
#20233=VERTEX_POINT('',#81025) ;
#20234=VERTEX_POINT('',#81048) ;
#20235=VERTEX_POINT('',#81072) ;
#20236=VERTEX_POINT('',#81089) ;
#20237=VERTEX_POINT('',#81093) ;
#20238=VERTEX_POINT('',#81094) ;
#20239=VERTEX_POINT('',#81161) ;
#20240=VERTEX_POINT('',#81205) ;
#20241=VERTEX_POINT('',#81283) ;
#20242=VERTEX_POINT('',#81336) ;
#20243=VERTEX_POINT('',#81518) ;
#20244=VERTEX_POINT('',#81519) ;
#20245=VERTEX_POINT('',#81521) ;
#20246=VERTEX_POINT('',#81523) ;
#20247=VERTEX_POINT('',#81527) ;
#20248=VERTEX_POINT('',#81529) ;
#20249=VERTEX_POINT('',#81536) ;
#20250=VERTEX_POINT('',#81538) ;
#20251=VERTEX_POINT('',#81542) ;
#20252=VERTEX_POINT('',#81547) ;
#20253=VERTEX_POINT('',#81548) ;
#20254=VERTEX_POINT('',#81550) ;
#20255=VERTEX_POINT('',#81552) ;
#20256=VERTEX_POINT('',#81556) ;
#20257=VERTEX_POINT('',#81558) ;
#20258=VERTEX_POINT('',#81562) ;
#20259=VERTEX_POINT('',#81564) ;
#20260=VERTEX_POINT('',#81571) ;
#20261=VERTEX_POINT('',#81573) ;
#20262=VERTEX_POINT('',#81577) ;
#20263=VERTEX_POINT('',#81582) ;
#20264=VERTEX_POINT('',#81583) ;
#20265=VERTEX_POINT('',#81585) ;
#20266=VERTEX_POINT('',#81587) ;
#20267=VERTEX_POINT('',#81591) ;
#20268=VERTEX_POINT('',#81593) ;
#20269=VERTEX_POINT('',#81600) ;
#20270=VERTEX_POINT('',#81602) ;
#20271=VERTEX_POINT('',#81606) ;
#20272=VERTEX_POINT('',#81611) ;
#20273=VERTEX_POINT('',#81612) ;
#20274=VERTEX_POINT('',#81685) ;
#20275=VERTEX_POINT('',#81770) ;
#20276=VERTEX_POINT('',#81792) ;
#20277=VERTEX_POINT('',#81794) ;
#20278=VERTEX_POINT('',#81837) ;
#20279=VERTEX_POINT('',#81846) ;
#20280=VERTEX_POINT('',#81917) ;
#20281=VERTEX_POINT('',#81928) ;
#20282=VERTEX_POINT('',#82019) ;
#20283=VERTEX_POINT('',#82030) ;
#20284=VERTEX_POINT('',#82121) ;
#20285=VERTEX_POINT('',#82132) ;
#20286=VERTEX_POINT('',#82193) ;
#20287=VERTEX_POINT('',#82202) ;
#20288=VERTEX_POINT('',#82251) ;
#20289=VERTEX_POINT('',#82253) ;
#20290=VERTEX_POINT('',#82255) ;
#20291=VERTEX_POINT('',#82259) ;
#20292=VERTEX_POINT('',#82261) ;
#20293=VERTEX_POINT('',#82265) ;
#20294=VERTEX_POINT('',#82267) ;
#20295=VERTEX_POINT('',#82303) ;
#20296=VERTEX_POINT('',#82305) ;
#20297=VERTEX_POINT('',#82358) ;
#20298=VERTEX_POINT('',#82426) ;
#20299=VERTEX_POINT('',#82555) ;
#20300=VERTEX_POINT('',#82556) ;
#20301=VERTEX_POINT('',#82558) ;
#20302=VERTEX_POINT('',#82560) ;
#20303=VERTEX_POINT('',#82562) ;
#20304=VERTEX_POINT('',#82564) ;
#20305=VERTEX_POINT('',#82566) ;
#20306=VERTEX_POINT('',#82568) ;
#20307=VERTEX_POINT('',#82570) ;
#20308=VERTEX_POINT('',#82572) ;
#20309=VERTEX_POINT('',#82575) ;
#20310=VERTEX_POINT('',#82577) ;
#20311=VERTEX_POINT('',#82579) ;
#20312=VERTEX_POINT('',#82581) ;
#20313=VERTEX_POINT('',#82583) ;
#20314=VERTEX_POINT('',#82585) ;
#20315=VERTEX_POINT('',#82587) ;
#20316=VERTEX_POINT('',#82589) ;
#20317=VERTEX_POINT('',#82591) ;
#20318=VERTEX_POINT('',#82593) ;
#20319=VERTEX_POINT('',#82595) ;
#20320=VERTEX_POINT('',#82597) ;
#20321=VERTEX_POINT('',#82599) ;
#20322=VERTEX_POINT('',#82601) ;
#20323=VERTEX_POINT('',#82603) ;
#20324=VERTEX_POINT('',#82605) ;
#20325=VERTEX_POINT('',#82607) ;
#20326=VERTEX_POINT('',#82609) ;
#20327=VERTEX_POINT('',#82611) ;
#20328=VERTEX_POINT('',#82613) ;
#20329=VERTEX_POINT('',#82615) ;
#20330=VERTEX_POINT('',#82617) ;
#20331=VERTEX_POINT('',#82619) ;
#20332=VERTEX_POINT('',#82621) ;
#20333=VERTEX_POINT('',#82623) ;
#20334=VERTEX_POINT('',#82625) ;
#20335=VERTEX_POINT('',#82627) ;
#20336=VERTEX_POINT('',#82629) ;
#20337=VERTEX_POINT('',#82631) ;
#20338=VERTEX_POINT('',#82633) ;
#20339=VERTEX_POINT('',#82635) ;
#20340=VERTEX_POINT('',#82637) ;
#20341=VERTEX_POINT('',#82639) ;
#20342=VERTEX_POINT('',#82641) ;
#20343=VERTEX_POINT('',#82643) ;
#20344=VERTEX_POINT('',#82645) ;
#20345=VERTEX_POINT('',#82647) ;
#20346=VERTEX_POINT('',#82649) ;
#20347=VERTEX_POINT('',#82652) ;
#20348=VERTEX_POINT('',#82653) ;
#20349=VERTEX_POINT('',#82655) ;
#20350=VERTEX_POINT('',#82658) ;
#20351=VERTEX_POINT('',#82659) ;
#20352=VERTEX_POINT('',#82661) ;
#20353=VERTEX_POINT('',#82664) ;
#20354=VERTEX_POINT('',#82665) ;
#20355=VERTEX_POINT('',#82667) ;
#20356=VERTEX_POINT('',#82669) ;
#20357=VERTEX_POINT('',#82671) ;
#20358=VERTEX_POINT('',#82673) ;
#20359=VERTEX_POINT('',#82675) ;
#20360=VERTEX_POINT('',#82677) ;
#20361=VERTEX_POINT('',#82679) ;
#20362=VERTEX_POINT('',#82681) ;
#20363=VERTEX_POINT('',#82683) ;
#20364=VERTEX_POINT('',#82685) ;
#20365=VERTEX_POINT('',#82687) ;
#20366=VERTEX_POINT('',#82689) ;
#20367=VERTEX_POINT('',#82692) ;
#20368=VERTEX_POINT('',#82693) ;
#20369=VERTEX_POINT('',#82695) ;
#20370=VERTEX_POINT('',#82697) ;
#20371=VERTEX_POINT('',#82699) ;
#20372=VERTEX_POINT('',#82701) ;
#20373=VERTEX_POINT('',#82703) ;
#20374=VERTEX_POINT('',#82705) ;
#20375=VERTEX_POINT('',#82707) ;
#20376=VERTEX_POINT('',#82709) ;
#20377=VERTEX_POINT('',#82711) ;
#20378=VERTEX_POINT('',#82713) ;
#20379=VERTEX_POINT('',#82715) ;
#20380=VERTEX_POINT('',#82717) ;
#20381=VERTEX_POINT('',#82719) ;
#20382=VERTEX_POINT('',#82721) ;
#20383=VERTEX_POINT('',#82724) ;
#20384=VERTEX_POINT('',#82725) ;
#20385=VERTEX_POINT('',#82727) ;
#20386=VERTEX_POINT('',#82729) ;
#20387=VERTEX_POINT('',#82731) ;
#20388=VERTEX_POINT('',#82733) ;
#20389=VERTEX_POINT('',#82735) ;
#20390=VERTEX_POINT('',#82737) ;
#20391=VERTEX_POINT('',#82739) ;
#20392=VERTEX_POINT('',#82741) ;
#20393=VERTEX_POINT('',#82743) ;
#20394=VERTEX_POINT('',#82745) ;
#20395=VERTEX_POINT('',#82747) ;
#20396=VERTEX_POINT('',#82749) ;
#20397=VERTEX_POINT('',#82752) ;
#20398=VERTEX_POINT('',#82753) ;
#20399=VERTEX_POINT('',#82755) ;
#20400=VERTEX_POINT('',#82757) ;
#20401=VERTEX_POINT('',#82759) ;
#20402=VERTEX_POINT('',#82761) ;
#20403=VERTEX_POINT('',#82763) ;
#20404=VERTEX_POINT('',#82765) ;
#20405=VERTEX_POINT('',#82767) ;
#20406=VERTEX_POINT('',#82769) ;
#20407=VERTEX_POINT('',#82771) ;
#20408=VERTEX_POINT('',#82773) ;
#20409=VERTEX_POINT('',#82775) ;
#20410=VERTEX_POINT('',#82777) ;
#20411=VERTEX_POINT('',#82780) ;
#20412=VERTEX_POINT('',#82781) ;
#20413=VERTEX_POINT('',#82783) ;
#20414=VERTEX_POINT('',#82785) ;
#20415=VERTEX_POINT('',#82787) ;
#20416=VERTEX_POINT('',#82789) ;
#20417=VERTEX_POINT('',#82791) ;
#20418=VERTEX_POINT('',#82793) ;
#20419=VERTEX_POINT('',#82795) ;
#20420=VERTEX_POINT('',#82797) ;
#20421=VERTEX_POINT('',#82799) ;
#20422=VERTEX_POINT('',#82801) ;
#20423=VERTEX_POINT('',#82803) ;
#20424=VERTEX_POINT('',#82805) ;
#20425=VERTEX_POINT('',#82808) ;
#20426=VERTEX_POINT('',#82810) ;
#20427=VERTEX_POINT('',#82811) ;
#20428=VERTEX_POINT('',#82813) ;
#20429=VERTEX_POINT('',#82815) ;
#20430=VERTEX_POINT('',#82817) ;
#20431=VERTEX_POINT('',#82819) ;
#20432=VERTEX_POINT('',#82821) ;
#20433=VERTEX_POINT('',#82823) ;
#20434=VERTEX_POINT('',#82825) ;
#20435=VERTEX_POINT('',#82827) ;
#20436=VERTEX_POINT('',#82829) ;
#20437=VERTEX_POINT('',#82831) ;
#20438=VERTEX_POINT('',#82833) ;
#20439=VERTEX_POINT('',#82835) ;
#20440=VERTEX_POINT('',#82837) ;
#20441=VERTEX_POINT('',#82840) ;
#20442=VERTEX_POINT('',#82842) ;
#20443=VERTEX_POINT('',#82844) ;
#20444=VERTEX_POINT('',#82845) ;
#20445=VERTEX_POINT('',#82847) ;
#20446=VERTEX_POINT('',#82849) ;
#20447=VERTEX_POINT('',#82851) ;
#20448=VERTEX_POINT('',#82853) ;
#20449=VERTEX_POINT('',#82855) ;
#20450=VERTEX_POINT('',#82857) ;
#20451=VERTEX_POINT('',#82859) ;
#20452=VERTEX_POINT('',#82861) ;
#20453=VERTEX_POINT('',#82863) ;
#20454=VERTEX_POINT('',#82865) ;
#20455=VERTEX_POINT('',#82867) ;
#20456=VERTEX_POINT('',#82869) ;
#20457=VERTEX_POINT('',#82872) ;
#20458=VERTEX_POINT('',#82874) ;
#20459=VERTEX_POINT('',#82876) ;
#20460=VERTEX_POINT('',#82877) ;
#20461=VERTEX_POINT('',#82879) ;
#20462=VERTEX_POINT('',#82881) ;
#20463=VERTEX_POINT('',#82883) ;
#20464=VERTEX_POINT('',#82885) ;
#20465=VERTEX_POINT('',#82887) ;
#20466=VERTEX_POINT('',#82889) ;
#20467=VERTEX_POINT('',#82892) ;
#20468=VERTEX_POINT('',#82893) ;
#20469=VERTEX_POINT('',#82895) ;
#20470=VERTEX_POINT('',#82897) ;
#20471=VERTEX_POINT('',#82899) ;
#20472=VERTEX_POINT('',#82901) ;
#20473=VERTEX_POINT('',#82903) ;
#20474=VERTEX_POINT('',#82905) ;
#20475=VERTEX_POINT('',#82907) ;
#20476=VERTEX_POINT('',#82909) ;
#20477=VERTEX_POINT('',#82911) ;
#20478=VERTEX_POINT('',#82913) ;
#20479=VERTEX_POINT('',#82915) ;
#20480=VERTEX_POINT('',#82917) ;
#20481=VERTEX_POINT('',#82920) ;
#20482=VERTEX_POINT('',#82921) ;
#20483=VERTEX_POINT('',#82923) ;
#20484=VERTEX_POINT('',#82925) ;
#20485=VERTEX_POINT('',#82942) ;
#20486=VERTEX_POINT('',#83012) ;
#20487=VERTEX_POINT('',#83013) ;
#20488=VERTEX_POINT('',#83015) ;
#20489=VERTEX_POINT('',#83020) ;
#20490=VERTEX_POINT('',#83023) ;
#20491=VERTEX_POINT('',#83027) ;
#20492=VERTEX_POINT('',#83031) ;
#20493=VERTEX_POINT('',#83035) ;
#20494=VERTEX_POINT('',#83039) ;
#20495=VERTEX_POINT('',#83040) ;
#20496=VERTEX_POINT('',#83042) ;
#20497=VERTEX_POINT('',#83044) ;
#20498=VERTEX_POINT('',#83046) ;
#20499=VERTEX_POINT('',#83048) ;
#20500=VERTEX_POINT('',#83050) ;
#20501=VERTEX_POINT('',#83052) ;
#20502=VERTEX_POINT('',#83054) ;
#20503=VERTEX_POINT('',#83056) ;
#20504=VERTEX_POINT('',#83058) ;
#20505=VERTEX_POINT('',#83060) ;
#20506=VERTEX_POINT('',#83062) ;
#20507=VERTEX_POINT('',#83064) ;
#20508=VERTEX_POINT('',#83066) ;
#20509=VERTEX_POINT('',#83068) ;
#20510=VERTEX_POINT('',#83070) ;
#20511=VERTEX_POINT('',#83072) ;
#20512=VERTEX_POINT('',#83074) ;
#20513=VERTEX_POINT('',#83076) ;
#20514=VERTEX_POINT('',#83078) ;
#20515=VERTEX_POINT('',#83080) ;
#20516=VERTEX_POINT('',#83082) ;
#20517=VERTEX_POINT('',#83084) ;
#20518=VERTEX_POINT('',#83086) ;
#20519=VERTEX_POINT('',#83088) ;
#20520=VERTEX_POINT('',#83090) ;
#20521=VERTEX_POINT('',#83092) ;
#20522=VERTEX_POINT('',#83094) ;
#20523=VERTEX_POINT('',#83096) ;
#20524=VERTEX_POINT('',#83098) ;
#20525=VERTEX_POINT('',#83100) ;
#20526=VERTEX_POINT('',#83102) ;
#20527=VERTEX_POINT('',#83104) ;
#20528=VERTEX_POINT('',#83106) ;
#20529=VERTEX_POINT('',#83108) ;
#20530=VERTEX_POINT('',#83110) ;
#20531=VERTEX_POINT('',#83112) ;
#20532=VERTEX_POINT('',#83114) ;
#20533=VERTEX_POINT('',#83116) ;
#20534=VERTEX_POINT('',#83118) ;
#20535=VERTEX_POINT('',#83120) ;
#20536=VERTEX_POINT('',#83122) ;
#20537=VERTEX_POINT('',#83124) ;
#20538=VERTEX_POINT('',#83126) ;
#20539=VERTEX_POINT('',#83128) ;
#20540=VERTEX_POINT('',#83130) ;
#20541=VERTEX_POINT('',#83132) ;
#20542=VERTEX_POINT('',#83134) ;
#20543=VERTEX_POINT('',#83136) ;
#20544=VERTEX_POINT('',#83138) ;
#20545=VERTEX_POINT('',#83145) ;
#20546=VERTEX_POINT('',#83147) ;
#20547=VERTEX_POINT('',#83154) ;
#20548=VERTEX_POINT('',#83156) ;
#20549=VERTEX_POINT('',#83158) ;
#20550=VERTEX_POINT('',#83160) ;
#20551=VERTEX_POINT('',#83163) ;
#20552=VERTEX_POINT('',#83165) ;
#20553=VERTEX_POINT('',#83166) ;
#20554=VERTEX_POINT('',#83168) ;
#20555=VERTEX_POINT('',#83170) ;
#20556=VERTEX_POINT('',#83172) ;
#20557=VERTEX_POINT('',#83174) ;
#20558=VERTEX_POINT('',#83176) ;
#20559=VERTEX_POINT('',#83178) ;
#20560=VERTEX_POINT('',#83180) ;
#20561=VERTEX_POINT('',#83182) ;
#20562=VERTEX_POINT('',#83184) ;
#20563=VERTEX_POINT('',#83186) ;
#20564=VERTEX_POINT('',#83188) ;
#20565=VERTEX_POINT('',#83190) ;
#20566=VERTEX_POINT('',#83193) ;
#20567=VERTEX_POINT('',#83195) ;
#20568=VERTEX_POINT('',#83197) ;
#20569=VERTEX_POINT('',#83198) ;
#20570=VERTEX_POINT('',#83200) ;
#20571=VERTEX_POINT('',#83202) ;
#20572=VERTEX_POINT('',#83204) ;
#20573=VERTEX_POINT('',#83206) ;
#20574=VERTEX_POINT('',#83208) ;
#20575=VERTEX_POINT('',#83210) ;
#20576=VERTEX_POINT('',#83212) ;
#20577=VERTEX_POINT('',#83214) ;
#20578=VERTEX_POINT('',#83216) ;
#20579=VERTEX_POINT('',#83218) ;
#20580=VERTEX_POINT('',#83220) ;
#20581=VERTEX_POINT('',#83222) ;
#20582=VERTEX_POINT('',#83224) ;
#20583=VERTEX_POINT('',#83226) ;
#20584=VERTEX_POINT('',#83229) ;
#20585=VERTEX_POINT('',#83231) ;
#20586=VERTEX_POINT('',#83232) ;
#20587=VERTEX_POINT('',#83234) ;
#20588=VERTEX_POINT('',#83236) ;
#20589=VERTEX_POINT('',#83238) ;
#20590=VERTEX_POINT('',#83240) ;
#20591=VERTEX_POINT('',#83242) ;
#20592=VERTEX_POINT('',#83244) ;
#20593=VERTEX_POINT('',#83246) ;
#20594=VERTEX_POINT('',#83248) ;
#20595=VERTEX_POINT('',#83250) ;
#20596=VERTEX_POINT('',#83252) ;
#20597=VERTEX_POINT('',#83254) ;
#20598=VERTEX_POINT('',#83256) ;
#20599=VERTEX_POINT('',#83259) ;
#20600=VERTEX_POINT('',#83260) ;
#20601=VERTEX_POINT('',#83262) ;
#20602=VERTEX_POINT('',#83264) ;
#20603=VERTEX_POINT('',#83266) ;
#20604=VERTEX_POINT('',#83268) ;
#20605=VERTEX_POINT('',#83270) ;
#20606=VERTEX_POINT('',#83272) ;
#20607=VERTEX_POINT('',#83275) ;
#20608=VERTEX_POINT('',#83276) ;
#20609=VERTEX_POINT('',#83278) ;
#20610=VERTEX_POINT('',#83280) ;
#20611=VERTEX_POINT('',#83282) ;
#20612=VERTEX_POINT('',#83289) ;
#20613=VERTEX_POINT('',#83291) ;
#20614=VERTEX_POINT('',#83293) ;
#20615=VERTEX_POINT('',#83295) ;
#20616=VERTEX_POINT('',#83297) ;
#20617=VERTEX_POINT('',#83299) ;
#20618=VERTEX_POINT('',#83301) ;
#20619=VERTEX_POINT('',#83303) ;
#20620=VERTEX_POINT('',#83305) ;
#20621=VERTEX_POINT('',#83313) ;
#20622=VERTEX_POINT('',#83314) ;
#20623=VERTEX_POINT('',#83316) ;
#20624=VERTEX_POINT('',#83323) ;
#20625=VERTEX_POINT('',#83325) ;
#20626=VERTEX_POINT('',#83327) ;
#20627=VERTEX_POINT('',#83329) ;
#20628=VERTEX_POINT('',#83331) ;
#20629=VERTEX_POINT('',#83333) ;
#20630=VERTEX_POINT('',#83335) ;
#20631=VERTEX_POINT('',#83337) ;
#20632=VERTEX_POINT('',#83339) ;
#20633=VERTEX_POINT('',#83341) ;
#20634=VERTEX_POINT('',#83343) ;
#20635=VERTEX_POINT('',#83351) ;
#20636=VERTEX_POINT('',#83352) ;
#20637=VERTEX_POINT('',#83354) ;
#20638=VERTEX_POINT('',#83356) ;
#20639=VERTEX_POINT('',#83358) ;
#20640=VERTEX_POINT('',#83360) ;
#20641=VERTEX_POINT('',#83362) ;
#20642=VERTEX_POINT('',#83364) ;
#20643=VERTEX_POINT('',#83366) ;
#20644=VERTEX_POINT('',#83368) ;
#20645=VERTEX_POINT('',#83370) ;
#20646=VERTEX_POINT('',#83372) ;
#20647=VERTEX_POINT('',#83374) ;
#20648=VERTEX_POINT('',#83376) ;
#20649=VERTEX_POINT('',#83379) ;
#20650=VERTEX_POINT('',#83380) ;
#20651=VERTEX_POINT('',#83382) ;
#20652=VERTEX_POINT('',#83384) ;
#20653=VERTEX_POINT('',#83386) ;
#20654=VERTEX_POINT('',#83388) ;
#20655=VERTEX_POINT('',#83390) ;
#20656=VERTEX_POINT('',#83392) ;
#20657=VERTEX_POINT('',#83394) ;
#20658=VERTEX_POINT('',#83396) ;
#20659=VERTEX_POINT('',#83398) ;
#20660=VERTEX_POINT('',#83400) ;
#20661=VERTEX_POINT('',#83402) ;
#20662=VERTEX_POINT('',#83404) ;
#20663=VERTEX_POINT('',#83407) ;
#20664=VERTEX_POINT('',#83427) ;
#20665=VERTEX_POINT('',#83428) ;
#20666=VERTEX_POINT('',#83431) ;
#20667=VERTEX_POINT('',#83435) ;
#20668=VERTEX_POINT('',#83436) ;
#20669=VERTEX_POINT('',#83441) ;
#20670=VERTEX_POINT('',#83442) ;
#20671=VERTEX_POINT('',#83447) ;
#20672=VERTEX_POINT('',#83448) ;
#20673=VERTEX_POINT('',#83453) ;
#20674=VERTEX_POINT('',#83454) ;
#20675=VERTEX_POINT('',#83459) ;
#20676=VERTEX_POINT('',#83460) ;
#20677=VERTEX_POINT('',#83465) ;
#20678=VERTEX_POINT('',#83466) ;
#20679=VERTEX_POINT('',#83471) ;
#20680=VERTEX_POINT('',#83472) ;
#20681=VERTEX_POINT('',#83477) ;
#20682=VERTEX_POINT('',#83478) ;
#20683=VERTEX_POINT('',#83483) ;
#20684=VERTEX_POINT('',#83484) ;
#20685=VERTEX_POINT('',#83489) ;
#20686=VERTEX_POINT('',#83490) ;
#20687=VERTEX_POINT('',#83495) ;
#20688=VERTEX_POINT('',#83496) ;
#20689=VERTEX_POINT('',#83501) ;
#20690=VERTEX_POINT('',#83506) ;
#20691=VERTEX_POINT('',#83508) ;
#20692=VERTEX_POINT('',#83510) ;
#20693=VERTEX_POINT('',#83512) ;
#20694=VERTEX_POINT('',#83514) ;
#20695=VERTEX_POINT('',#83518) ;
#20696=VERTEX_POINT('',#83522) ;
#20697=VERTEX_POINT('',#83526) ;
#20698=VERTEX_POINT('',#83530) ;
#20699=VERTEX_POINT('',#83534) ;
#20700=VERTEX_POINT('',#83538) ;
#20701=VERTEX_POINT('',#83542) ;
#20702=VERTEX_POINT('',#83546) ;
#20703=VERTEX_POINT('',#83550) ;
#20704=VERTEX_POINT('',#83554) ;
#20705=VERTEX_POINT('',#83556) ;
#20706=VERTEX_POINT('',#83558) ;
#20707=VERTEX_POINT('',#83560) ;
#20708=VERTEX_POINT('',#83564) ;
#20709=VERTEX_POINT('',#83568) ;
#20710=VERTEX_POINT('',#83661) ;
#20711=VERTEX_POINT('',#83667) ;
#20712=VERTEX_POINT('',#83688) ;
#20713=VERTEX_POINT('',#83692) ;
#20714=VERTEX_POINT('',#83695) ;
#20715=VERTEX_POINT('',#83696) ;
#20716=VERTEX_POINT('',#83701) ;
#20717=VERTEX_POINT('',#83705) ;
#20718=VERTEX_POINT('',#83707) ;
#20719=VERTEX_POINT('',#83709) ;
#20720=VERTEX_POINT('',#83713) ;
#20721=VERTEX_POINT('',#83715) ;
#20722=VERTEX_POINT('',#83719) ;
#20723=VERTEX_POINT('',#83720) ;
#20724=VERTEX_POINT('',#83722) ;
#20725=VERTEX_POINT('',#83724) ;
#20726=VERTEX_POINT('',#83726) ;
#20727=VERTEX_POINT('',#83728) ;
#20728=VERTEX_POINT('',#83732) ;
#20729=VERTEX_POINT('',#83736) ;
#20730=VERTEX_POINT('',#83737) ;
#20731=VERTEX_POINT('',#83744) ;
#20732=VERTEX_POINT('',#83746) ;
#20733=VERTEX_POINT('',#83754) ;
#20734=VERTEX_POINT('',#83756) ;
#20735=VERTEX_POINT('',#83758) ;
#20736=VERTEX_POINT('',#83762) ;
#20737=VERTEX_POINT('',#83764) ;
#20738=VERTEX_POINT('',#83768) ;
#20739=VERTEX_POINT('',#83769) ;
#20740=VERTEX_POINT('',#83771) ;
#20741=VERTEX_POINT('',#83773) ;
#20742=VERTEX_POINT('',#83775) ;
#20743=VERTEX_POINT('',#83777) ;
#20744=VERTEX_POINT('',#83781) ;
#20745=VERTEX_POINT('',#83785) ;
#20746=VERTEX_POINT('',#83786) ;
#20747=VERTEX_POINT('',#83792) ;
#20748=VERTEX_POINT('',#83794) ;
#20749=VERTEX_POINT('',#83803) ;
#20750=VERTEX_POINT('',#83805) ;
#20751=VERTEX_POINT('',#83809) ;
#20752=VERTEX_POINT('',#83813) ;
#20753=VERTEX_POINT('',#83817) ;
#20754=VERTEX_POINT('',#83821) ;
#20755=VERTEX_POINT('',#83825) ;
#20756=VERTEX_POINT('',#83827) ;
#20757=VERTEX_POINT('',#83829) ;
#20758=VERTEX_POINT('',#83831) ;
#20759=VERTEX_POINT('',#83833) ;
#20760=VERTEX_POINT('',#83845) ;
#20761=VERTEX_POINT('',#83856) ;
#20762=VERTEX_POINT('',#83858) ;
#20763=VERTEX_POINT('',#83860) ;
#20764=VERTEX_POINT('',#83872) ;
#20765=VERTEX_POINT('',#83883) ;
#20766=VERTEX_POINT('',#83885) ;
#20767=VERTEX_POINT('',#83887) ;
#20768=VERTEX_POINT('',#83889) ;
#20769=VERTEX_POINT('',#83895) ;
#20770=VERTEX_POINT('',#83897) ;
#20771=VERTEX_POINT('',#83917) ;
#20772=VERTEX_POINT('',#83936) ;
#20773=VERTEX_POINT('',#83939) ;
#20774=VERTEX_POINT('',#83941) ;
#20775=VERTEX_POINT('',#83961) ;
#20776=VERTEX_POINT('',#83980) ;
#20777=VERTEX_POINT('',#83982) ;
#20778=VERTEX_POINT('',#83984) ;
#20779=VERTEX_POINT('',#83986) ;
#20780=VERTEX_POINT('',#83991) ;
#20781=VERTEX_POINT('',#83993) ;
#20782=VERTEX_POINT('',#84037) ;
#20783=VERTEX_POINT('',#84060) ;
#20784=VERTEX_POINT('',#84082) ;
#20785=VERTEX_POINT('',#84120) ;
#20786=VERTEX_POINT('',#84122) ;
#20787=VERTEX_POINT('',#84126) ;
#20788=VERTEX_POINT('',#84130) ;
#20789=VERTEX_POINT('',#84134) ;
#20790=VERTEX_POINT('',#84157) ;
#20791=VERTEX_POINT('',#84159) ;
#20792=VERTEX_POINT('',#84163) ;
#20793=VERTEX_POINT('',#84167) ;
#20794=VERTEX_POINT('',#84171) ;
#20795=VERTEX_POINT('',#84172) ;
#20796=VERTEX_POINT('',#84180) ;
#20797=VERTEX_POINT('',#84182) ;
#20798=VERTEX_POINT('',#84186) ;
#20799=VERTEX_POINT('',#84187) ;
#20800=VERTEX_POINT('',#84196) ;
#20801=VERTEX_POINT('',#84197) ;
#20802=VERTEX_POINT('',#84205) ;
#20803=VERTEX_POINT('',#84206) ;
#20804=VERTEX_POINT('',#84214) ;
#20805=VERTEX_POINT('',#84218) ;
#20806=VERTEX_POINT('',#84222) ;
#20807=VERTEX_POINT('',#84228) ;
#20808=VERTEX_POINT('',#84232) ;
#20809=VERTEX_POINT('',#84234) ;
#20810=VERTEX_POINT('',#84240) ;
#20811=VERTEX_POINT('',#84241) ;
#20812=VERTEX_POINT('',#84246) ;
#20813=VERTEX_POINT('',#84247) ;
#20814=VERTEX_POINT('',#84274) ;
#20815=VERTEX_POINT('',#84299) ;
#20816=VERTEX_POINT('',#84300) ;
#20817=VERTEX_POINT('',#84305) ;
#20818=VERTEX_POINT('',#84306) ;
#20819=VERTEX_POINT('',#84314) ;
#20820=VERTEX_POINT('',#84320) ;
#20821=VERTEX_POINT('',#84322) ;
#20822=VERTEX_POINT('',#84326) ;
#20823=VERTEX_POINT('',#84330) ;
#20824=VERTEX_POINT('',#84334) ;
#20825=VERTEX_POINT('',#84338) ;
#20826=VERTEX_POINT('',#84344) ;
#20827=VERTEX_POINT('',#84348) ;
#20828=VERTEX_POINT('',#84350) ;
#20829=VERTEX_POINT('',#84354) ;
#20830=VERTEX_POINT('',#84358) ;
#20831=VERTEX_POINT('',#84362) ;
#20832=VERTEX_POINT('',#84366) ;
#20833=VERTEX_POINT('',#84370) ;
#20834=VERTEX_POINT('',#84374) ;
#20835=VERTEX_POINT('',#84378) ;
#20836=VERTEX_POINT('',#84382) ;
#20837=VERTEX_POINT('',#84386) ;
#20838=VERTEX_POINT('',#84390) ;
#20839=VERTEX_POINT('',#84394) ;
#20840=VERTEX_POINT('',#84396) ;
#20841=VERTEX_POINT('',#84400) ;
#20842=VERTEX_POINT('',#84404) ;
#20843=VERTEX_POINT('',#84408) ;
#20844=VERTEX_POINT('',#84412) ;
#20845=VERTEX_POINT('',#84416) ;
#20846=VERTEX_POINT('',#84420) ;
#20847=VERTEX_POINT('',#84424) ;
#20848=VERTEX_POINT('',#84428) ;
#20849=VERTEX_POINT('',#84432) ;
#20850=VERTEX_POINT('',#84434) ;
#20851=VERTEX_POINT('',#84438) ;
#20852=VERTEX_POINT('',#84442) ;
#20853=VERTEX_POINT('',#84446) ;
#20854=VERTEX_POINT('',#84450) ;
#20855=VERTEX_POINT('',#84458) ;
#20856=VERTEX_POINT('',#84460) ;
#20857=VERTEX_POINT('',#84464) ;
#20858=VERTEX_POINT('',#84468) ;
#20859=VERTEX_POINT('',#84472) ;
#20860=VERTEX_POINT('',#84476) ;
#20861=VERTEX_POINT('',#84480) ;
#20862=VERTEX_POINT('',#84484) ;
#20863=VERTEX_POINT('',#84488) ;
#20864=VERTEX_POINT('',#84492) ;
#20865=VERTEX_POINT('',#84494) ;
#20866=VERTEX_POINT('',#84498) ;
#20867=VERTEX_POINT('',#84499) ;
#20868=VERTEX_POINT('',#84504) ;
#20869=VERTEX_POINT('',#84508) ;
#20870=VERTEX_POINT('',#84512) ;
#20871=VERTEX_POINT('',#84516) ;
#20872=VERTEX_POINT('',#84520) ;
#20873=VERTEX_POINT('',#84524) ;
#20874=VERTEX_POINT('',#84528) ;
#20875=VERTEX_POINT('',#84532) ;
#20876=VERTEX_POINT('',#84538) ;
#20877=VERTEX_POINT('',#84542) ;
#20878=VERTEX_POINT('',#84543) ;
#20879=VERTEX_POINT('',#84570) ;
#20880=VERTEX_POINT('',#84571) ;
#20881=VERTEX_POINT('',#84598) ;
#20882=VERTEX_POINT('',#84602) ;
#20883=VERTEX_POINT('',#84606) ;
#20884=VERTEX_POINT('',#84608) ;
#20885=VERTEX_POINT('',#84612) ;
#20886=VERTEX_POINT('',#84616) ;
#20887=VERTEX_POINT('',#84618) ;
#20888=VERTEX_POINT('',#84622) ;
#20889=VERTEX_POINT('',#84626) ;
#20890=VERTEX_POINT('',#84630) ;
#20891=VERTEX_POINT('',#84634) ;
#20892=VERTEX_POINT('',#84640) ;
#20893=VERTEX_POINT('',#84642) ;
#20894=VERTEX_POINT('',#84646) ;
#20895=VERTEX_POINT('',#84652) ;
#20896=VERTEX_POINT('',#84654) ;
#20897=VERTEX_POINT('',#84658) ;
#20898=VERTEX_POINT('',#84662) ;
#20899=VERTEX_POINT('',#84666) ;
#20900=VERTEX_POINT('',#84670) ;
#20901=VERTEX_POINT('',#84674) ;
#20902=VERTEX_POINT('',#84678) ;
#20903=VERTEX_POINT('',#84682) ;
#20904=VERTEX_POINT('',#84686) ;
#20905=VERTEX_POINT('',#84690) ;
#20906=VERTEX_POINT('',#84692) ;
#20907=VERTEX_POINT('',#84696) ;
#20908=VERTEX_POINT('',#84700) ;
#20909=VERTEX_POINT('',#84702) ;
#20910=VERTEX_POINT('',#84706) ;
#20911=VERTEX_POINT('',#84710) ;
#20912=VERTEX_POINT('',#84714) ;
#20913=VERTEX_POINT('',#84718) ;
#20914=VERTEX_POINT('',#84724) ;
#20915=VERTEX_POINT('',#84726) ;
#20916=VERTEX_POINT('',#84730) ;
#20917=VERTEX_POINT('',#84736) ;
#20918=VERTEX_POINT('',#84738) ;
#20919=VERTEX_POINT('',#84742) ;
#20920=VERTEX_POINT('',#84746) ;
#20921=VERTEX_POINT('',#84750) ;
#20922=VERTEX_POINT('',#84754) ;
#20923=VERTEX_POINT('',#84758) ;
#20924=VERTEX_POINT('',#84762) ;
#20925=VERTEX_POINT('',#84766) ;
#20926=VERTEX_POINT('',#84770) ;
#20927=VERTEX_POINT('',#84776) ;
#20928=VERTEX_POINT('',#84781) ;
#20929=VERTEX_POINT('',#84790) ;
#20930=VERTEX_POINT('',#84795) ;
#20931=VERTEX_POINT('',#84799) ;
#20932=VERTEX_POINT('',#84803) ;
#20933=VERTEX_POINT('',#84807) ;
#20934=VERTEX_POINT('',#84811) ;
#20935=VERTEX_POINT('',#84815) ;
#20936=VERTEX_POINT('',#84819) ;
#20937=VERTEX_POINT('',#84823) ;
#20938=VERTEX_POINT('',#84829) ;
#20939=VERTEX_POINT('',#84833) ;
#20940=VERTEX_POINT('',#84837) ;
#20941=VERTEX_POINT('',#84841) ;
#20942=VERTEX_POINT('',#84845) ;
#20943=VERTEX_POINT('',#84849) ;
#20944=VERTEX_POINT('',#84853) ;
#20945=VERTEX_POINT('',#84857) ;
#20946=VERTEX_POINT('',#84865) ;
#20947=VERTEX_POINT('',#84867) ;
#20948=VERTEX_POINT('',#84871) ;
#20949=VERTEX_POINT('',#84873) ;
#20950=VERTEX_POINT('',#84875) ;
#20951=VERTEX_POINT('',#84879) ;
#20952=VERTEX_POINT('',#84886) ;
#20953=VERTEX_POINT('',#84890) ;
#20954=VERTEX_POINT('',#84900) ;
#20955=VERTEX_POINT('',#84915) ;
#20956=VERTEX_POINT('',#84917) ;
#20957=VERTEX_POINT('',#84921) ;
#20958=VERTEX_POINT('',#84923) ;
#20959=VERTEX_POINT('',#84928) ;
#20960=VERTEX_POINT('',#84930) ;
#20961=VERTEX_POINT('',#84948) ;
#20962=VERTEX_POINT('',#84954) ;
#20963=VERTEX_POINT('',#84962) ;
#20964=VERTEX_POINT('',#84966) ;
#20965=VERTEX_POINT('',#84988) ;
#20966=VERTEX_POINT('',#84990) ;
#20967=VERTEX_POINT('',#84994) ;
#20968=VERTEX_POINT('',#84996) ;
#20969=VERTEX_POINT('',#85001) ;
#20970=VERTEX_POINT('',#85003) ;
#20971=VERTEX_POINT('',#85018) ;
#20972=VERTEX_POINT('',#85028) ;
#20973=VERTEX_POINT('',#85033) ;
#20974=VERTEX_POINT('',#85040) ;
#20975=VERTEX_POINT('',#85061) ;
#20976=VERTEX_POINT('',#85063) ;
#20977=VERTEX_POINT('',#85067) ;
#20978=VERTEX_POINT('',#85069) ;
#20979=VERTEX_POINT('',#85081) ;
#20980=VERTEX_POINT('',#85085) ;
#20981=VERTEX_POINT('',#85089) ;
#20982=VERTEX_POINT('',#85105) ;
#20983=VERTEX_POINT('',#85109) ;
#20984=VERTEX_POINT('',#85113) ;
#20985=VERTEX_POINT('',#85117) ;
#20986=VERTEX_POINT('',#85121) ;
#20987=VERTEX_POINT('',#85125) ;
#20988=VERTEX_POINT('',#85129) ;
#20989=VERTEX_POINT('',#85133) ;
#20990=VERTEX_POINT('',#85137) ;
#20991=VERTEX_POINT('',#85141) ;
#20992=VERTEX_POINT('',#85145) ;
#20993=VERTEX_POINT('',#85149) ;
#20994=VERTEX_POINT('',#85153) ;
#20995=VERTEX_POINT('',#85157) ;
#20996=VERTEX_POINT('',#85161) ;
#20997=VERTEX_POINT('',#85165) ;
#20998=VERTEX_POINT('',#85169) ;
#20999=VERTEX_POINT('',#85173) ;
#21000=VERTEX_POINT('',#85177) ;
#21001=VERTEX_POINT('',#85181) ;
#21002=VERTEX_POINT('',#85185) ;
#21003=VERTEX_POINT('',#85189) ;
#21004=VERTEX_POINT('',#85193) ;
#21005=VERTEX_POINT('',#85199) ;
#21006=VERTEX_POINT('',#85200) ;
#21007=VERTEX_POINT('',#85210) ;
#21008=VERTEX_POINT('',#85211) ;
#21009=VERTEX_POINT('',#85219) ;
#21010=VERTEX_POINT('',#85223) ;
#21011=VERTEX_POINT('',#85225) ;
#21012=VERTEX_POINT('',#85229) ;
#21013=VERTEX_POINT('',#85233) ;
#21014=VERTEX_POINT('',#85237) ;
#21015=VERTEX_POINT('',#85241) ;
#21016=VERTEX_POINT('',#85245) ;
#21017=VERTEX_POINT('',#85249) ;
#21018=VERTEX_POINT('',#85253) ;
#21019=VERTEX_POINT('',#85257) ;
#21020=VERTEX_POINT('',#85261) ;
#21021=VERTEX_POINT('',#85265) ;
#21022=VERTEX_POINT('',#85269) ;
#21023=VERTEX_POINT('',#85273) ;
#21024=VERTEX_POINT('',#85277) ;
#21025=VERTEX_POINT('',#85281) ;
#21026=VERTEX_POINT('',#85285) ;
#21027=VERTEX_POINT('',#85289) ;
#21028=VERTEX_POINT('',#85293) ;
#21029=VERTEX_POINT('',#85297) ;
#21030=VERTEX_POINT('',#85301) ;
#21031=VERTEX_POINT('',#85305) ;
#21032=VERTEX_POINT('',#85309) ;
#21033=VERTEX_POINT('',#85317) ;
#21034=VERTEX_POINT('',#85318) ;
#21035=VERTEX_POINT('',#85320) ;
#21036=VERTEX_POINT('',#85322) ;
#21037=VERTEX_POINT('',#85326) ;
#21038=VERTEX_POINT('',#85333) ;
#21039=VERTEX_POINT('',#85337) ;
#21040=VERTEX_POINT('',#85341) ;
#21041=VERTEX_POINT('',#85343) ;
#21042=VERTEX_POINT('',#85345) ;
#21043=VERTEX_POINT('',#85349) ;
#21044=VERTEX_POINT('',#85353) ;
#21045=VERTEX_POINT('',#85362) ;
#21046=VERTEX_POINT('',#85364) ;
#21047=VERTEX_POINT('',#85368) ;
#21048=VERTEX_POINT('',#85369) ;
#21049=VERTEX_POINT('',#85376) ;
#21050=VERTEX_POINT('',#85377) ;
#21051=VERTEX_POINT('',#85384) ;
#21052=VERTEX_POINT('',#85385) ;
#21053=VERTEX_POINT('',#85392) ;
#21054=VERTEX_POINT('',#85393) ;
#21055=VERTEX_POINT('',#85400) ;
#21056=VERTEX_POINT('',#85402) ;
#21057=VERTEX_POINT('',#85432) ;
#21058=VERTEX_POINT('',#85434) ;
#21059=VERTEX_POINT('',#85438) ;
#21060=VERTEX_POINT('',#85440) ;
#21061=VERTEX_POINT('',#85449) ;
#21062=VERTEX_POINT('',#85451) ;
#21063=VERTEX_POINT('',#85460) ;
#21064=VERTEX_POINT('',#85492) ;
#21065=VERTEX_POINT('',#85493) ;
#21066=VERTEX_POINT('',#85495) ;
#21067=VERTEX_POINT('',#85497) ;
#21068=VERTEX_POINT('',#85506) ;
#21069=VERTEX_POINT('',#85510) ;
#21070=VERTEX_POINT('',#85511) ;
#21071=VERTEX_POINT('',#85513) ;
#21072=VERTEX_POINT('',#85515) ;
#21073=VERTEX_POINT('',#85545) ;
#21074=VERTEX_POINT('',#85546) ;
#21075=VERTEX_POINT('',#85548) ;
#21076=VERTEX_POINT('',#85550) ;
#21077=VERTEX_POINT('',#85560) ;
#21078=VERTEX_POINT('',#85564) ;
#21079=VERTEX_POINT('',#85568) ;
#21080=VERTEX_POINT('',#85570) ;
#21081=VERTEX_POINT('',#85572) ;
#21082=VERTEX_POINT('',#85576) ;
#21083=VERTEX_POINT('',#85580) ;
#21084=VERTEX_POINT('',#85589) ;
#21085=VERTEX_POINT('',#85590) ;
#21086=VERTEX_POINT('',#85595) ;
#21087=VERTEX_POINT('',#85596) ;
#21088=VERTEX_POINT('',#85601) ;
#21089=VERTEX_POINT('',#85602) ;
#21090=VERTEX_POINT('',#85607) ;
#21091=VERTEX_POINT('',#85608) ;
#21092=VERTEX_POINT('',#85649) ;
#21093=VERTEX_POINT('',#85651) ;
#21094=VERTEX_POINT('',#85655) ;
#21095=VERTEX_POINT('',#85656) ;
#21096=VERTEX_POINT('',#85661) ;
#21097=VERTEX_POINT('',#85663) ;
#21098=VERTEX_POINT('',#85667) ;
#21099=VERTEX_POINT('',#85668) ;
#21100=VERTEX_POINT('',#85673) ;
#21101=VERTEX_POINT('',#85675) ;
#21102=VERTEX_POINT('',#85679) ;
#21103=VERTEX_POINT('',#85680) ;
#21104=VERTEX_POINT('',#85685) ;
#21105=VERTEX_POINT('',#85687) ;
#21106=VERTEX_POINT('',#85693) ;
#21107=VERTEX_POINT('',#85694) ;
#21108=VERTEX_POINT('',#85729) ;
#21109=VERTEX_POINT('',#85733) ;
#21110=VERTEX_POINT('',#85735) ;
#21111=VERTEX_POINT('',#85741) ;
#21112=VERTEX_POINT('',#85742) ;
#21113=VERTEX_POINT('',#85744) ;
#21114=VERTEX_POINT('',#85746) ;
#21115=VERTEX_POINT('',#85756) ;
#21116=VERTEX_POINT('',#85760) ;
#21117=VERTEX_POINT('',#85762) ;
#21118=VERTEX_POINT('',#85764) ;
#21119=VERTEX_POINT('',#85768) ;
#21120=VERTEX_POINT('',#85772) ;
#21121=VERTEX_POINT('',#85776) ;
#21122=VERTEX_POINT('',#85808) ;
#21123=VERTEX_POINT('',#85810) ;
#21124=VERTEX_POINT('',#85816) ;
#21125=VERTEX_POINT('',#85818) ;
#21126=VERTEX_POINT('',#85873) ;
#21127=VERTEX_POINT('',#85877) ;
#21128=VERTEX_POINT('',#85881) ;
#21129=VERTEX_POINT('',#85887) ;
#21130=VERTEX_POINT('',#85891) ;
#21131=VERTEX_POINT('',#85894) ;
#21132=VERTEX_POINT('',#85895) ;
#21133=VERTEX_POINT('',#85900) ;
#21134=VERTEX_POINT('',#85904) ;
#21135=VERTEX_POINT('',#85906) ;
#21136=VERTEX_POINT('',#85910) ;
#21137=VERTEX_POINT('',#85912) ;
#21138=VERTEX_POINT('',#85914) ;
#21139=VERTEX_POINT('',#85918) ;
#21140=VERTEX_POINT('',#85920) ;
#21141=VERTEX_POINT('',#85924) ;
#21142=VERTEX_POINT('',#85928) ;
#21143=VERTEX_POINT('',#85931) ;
#21144=VERTEX_POINT('',#85935) ;
#21145=VERTEX_POINT('',#85939) ;
#21146=VERTEX_POINT('',#85941) ;
#21147=VERTEX_POINT('',#85943) ;
#21148=VERTEX_POINT('',#85947) ;
#21149=VERTEX_POINT('',#85949) ;
#21150=VERTEX_POINT('',#85953) ;
#21151=VERTEX_POINT('',#85957) ;
#21152=VERTEX_POINT('',#86010) ;
#21153=VERTEX_POINT('',#86038) ;
#21154=VERTEX_POINT('',#86039) ;
#21155=VERTEX_POINT('',#86042) ;
#21156=VERTEX_POINT('',#86071) ;
#21157=VERTEX_POINT('',#86074) ;
#21158=VERTEX_POINT('',#86076) ;
#21159=VERTEX_POINT('',#86104) ;
#21160=VERTEX_POINT('',#86105) ;
#21161=VERTEX_POINT('',#86110) ;
#21162=VERTEX_POINT('',#86172) ;
#21163=VERTEX_POINT('',#86179) ;
#21164=VERTEX_POINT('',#86241) ;
#21165=VERTEX_POINT('',#86248) ;
#21166=VERTEX_POINT('',#86252) ;
#21167=VERTEX_POINT('',#86260) ;
#21168=VERTEX_POINT('',#86268) ;
#21169=VERTEX_POINT('',#86276) ;
#24828=EDGE_CURVE('',#20162,#20163,#998,.T.) ;
#24829=EDGE_CURVE('',#20163,#20164,#999,.T.) ;
#24830=EDGE_CURVE('',#20164,#20165,#1000,.T.) ;
#24831=EDGE_CURVE('',#20162,#20165,#1001,.T.) ;
#24832=EDGE_CURVE('',#20166,#20167,#1002,.T.) ;
#24833=EDGE_CURVE('',#20167,#20168,#1003,.T.) ;
#24834=EDGE_CURVE('',#20168,#20169,#1004,.T.) ;
#24835=EDGE_CURVE('',#20169,#20166,#1005,.T.) ;
#24836=EDGE_CURVE('',#20163,#20170,#1006,.T.) ;
#24837=EDGE_CURVE('',#20170,#20171,#1007,.T.) ;
#24838=EDGE_CURVE('',#20171,#20164,#1008,.T.) ;
#24839=EDGE_CURVE('',#20170,#20172,#3323,.T.) ;
#24840=EDGE_CURVE('',#20172,#20173,#171,.T.) ;
#24841=EDGE_CURVE('',#20173,#20171,#3324,.T.) ;
#24842=EDGE_CURVE('',#20174,#20173,#3325,.T.) ;
#24843=EDGE_CURVE('',#20172,#20175,#3326,.T.) ;
#24844=EDGE_CURVE('',#20175,#20174,#172,.T.) ;
#24845=EDGE_CURVE('',#20167,#20174,#3327,.T.) ;
#24846=EDGE_CURVE('',#20175,#20168,#3328,.T.) ;
#24847=EDGE_CURVE('',#20176,#20166,#1009,.T.) ;
#24848=EDGE_CURVE('',#20169,#20177,#1010,.T.) ;
#24849=EDGE_CURVE('',#20177,#20176,#1011,.T.) ;
#24850=EDGE_CURVE('',#20165,#20176,#1012,.T.) ;
#24851=EDGE_CURVE('',#20177,#20162,#1013,.T.) ;
#24852=EDGE_CURVE('',#20178,#20173,#3329,.T.) ;
#24853=EDGE_CURVE('',#20179,#20178,#3330,.T.) ;
#24854=EDGE_CURVE('',#20179,#20171,#3331,.T.) ;
#24855=EDGE_CURVE('',#20180,#20174,#3332,.T.) ;
#24856=EDGE_CURVE('',#20178,#20180,#3333,.T.) ;
#24857=EDGE_CURVE('',#20181,#20167,#3334,.T.) ;
#24858=EDGE_CURVE('',#20180,#20181,#3335,.T.) ;
#24859=EDGE_CURVE('',#20182,#20166,#3336,.T.) ;
#24860=EDGE_CURVE('',#20181,#20182,#1014,.T.) ;
#24861=EDGE_CURVE('',#20183,#20184,#3337,.T.) ;
#24862=EDGE_CURVE('',#20185,#20183,#1015,.T.) ;
#24863=EDGE_CURVE('',#20186,#20185,#1016,.T.) ;
#24864=EDGE_CURVE('',#20187,#20186,#1017,.T.) ;
#24865=EDGE_CURVE('',#20188,#20187,#1018,.T.) ;
#24866=EDGE_CURVE('',#20189,#20188,#3338,.T.) ;
#24867=EDGE_CURVE('',#20190,#20189,#3339,.T.) ;
#24868=EDGE_CURVE('',#20191,#20190,#3340,.T.) ;
#24869=EDGE_CURVE('',#20192,#20191,#1019,.T.) ;
#24870=EDGE_CURVE('',#20193,#20192,#1020,.T.) ;
#24871=EDGE_CURVE('',#20194,#20193,#1021,.T.) ;
#24872=EDGE_CURVE('',#20195,#20194,#1022,.T.) ;
#24873=EDGE_CURVE('',#20196,#20195,#1023,.T.) ;
#24874=EDGE_CURVE('',#20197,#20196,#1024,.T.) ;
#24875=EDGE_CURVE('',#20198,#20197,#1025,.T.) ;
#24876=EDGE_CURVE('',#20199,#20198,#3341,.T.) ;
#24877=EDGE_CURVE('',#20200,#20199,#3342,.T.) ;
#24878=EDGE_CURVE('',#20201,#20200,#3343,.T.) ;
#24879=EDGE_CURVE('',#20184,#20201,#3344,.T.) ;
#24880=EDGE_CURVE('',#20190,#20202,#173,.T.) ;
#24881=EDGE_CURVE('',#20202,#20203,#3345,.T.) ;
#24882=EDGE_CURVE('',#20191,#20203,#1026,.T.) ;
#24883=EDGE_CURVE('',#20189,#20204,#174,.T.) ;
#24884=EDGE_CURVE('',#20204,#20202,#3346,.T.) ;
#24885=EDGE_CURVE('',#20188,#20205,#1027,.T.) ;
#24886=EDGE_CURVE('',#20205,#20204,#3347,.T.) ;
#24887=EDGE_CURVE('',#20187,#20206,#1028,.T.) ;
#24888=EDGE_CURVE('',#20206,#20205,#1029,.T.) ;
#24889=EDGE_CURVE('',#20186,#20207,#1030,.T.) ;
#24890=EDGE_CURVE('',#20207,#20206,#1031,.T.) ;
#24891=EDGE_CURVE('',#20208,#20209,#1032,.T.) ;
#24892=EDGE_CURVE('',#20209,#20198,#17504,.T.) ;
#24893=EDGE_CURVE('',#20197,#20208,#1033,.T.) ;
#24894=EDGE_CURVE('',#20185,#20210,#1034,.T.) ;
#24895=EDGE_CURVE('',#20210,#20207,#1035,.T.) ;
#24896=EDGE_CURVE('',#20211,#20212,#3348,.T.) ;
#24897=EDGE_CURVE('',#20212,#20183,#17505,.T.) ;
#24898=EDGE_CURVE('',#20184,#20211,#175,.T.) ;
#24899=EDGE_CURVE('',#20212,#20210,#1036,.T.) ;
#24900=EDGE_CURVE('',#20201,#20213,#176,.T.) ;
#24901=EDGE_CURVE('',#20213,#20211,#3349,.T.) ;
#24902=EDGE_CURVE('',#20214,#20213,#3350,.T.) ;
#24903=EDGE_CURVE('',#20200,#20214,#177,.T.) ;
#24904=EDGE_CURVE('',#20215,#20214,#3351,.T.) ;
#24905=EDGE_CURVE('',#20199,#20215,#178,.T.) ;
#24906=EDGE_CURVE('',#20209,#20215,#3352,.T.) ;
#24907=EDGE_CURVE('',#20216,#20208,#1037,.T.) ;
#24908=EDGE_CURVE('',#20196,#20216,#1038,.T.) ;
#24909=EDGE_CURVE('',#20217,#20216,#1039,.T.) ;
#24910=EDGE_CURVE('',#20195,#20217,#1040,.T.) ;
#24911=EDGE_CURVE('',#20218,#20217,#1041,.T.) ;
#24912=EDGE_CURVE('',#20194,#20218,#1042,.T.) ;
#24913=EDGE_CURVE('',#20219,#20218,#1043,.T.) ;
#24914=EDGE_CURVE('',#20193,#20219,#1044,.T.) ;
#24915=EDGE_CURVE('',#20220,#20219,#1045,.T.) ;
#24916=EDGE_CURVE('',#20192,#20220,#1046,.T.) ;
#24917=EDGE_CURVE('',#20203,#20220,#1047,.T.) ;
#24918=EDGE_CURVE('',#20221,#20220,#3353,.T.) ;
#24919=EDGE_CURVE('',#20222,#20221,#1048,.T.) ;
#24920=EDGE_CURVE('',#20222,#20219,#3354,.T.) ;
#24921=EDGE_CURVE('',#20223,#20203,#3355,.T.) ;
#24922=EDGE_CURVE('',#20221,#20223,#1049,.T.) ;
#24923=EDGE_CURVE('',#20224,#20202,#3356,.T.) ;
#24924=EDGE_CURVE('',#20223,#20224,#3357,.T.) ;
#24925=EDGE_CURVE('',#20225,#20204,#3358,.T.) ;
#24926=EDGE_CURVE('',#20224,#20225,#3359,.T.) ;
#24927=EDGE_CURVE('',#20226,#20205,#3360,.T.) ;
#24928=EDGE_CURVE('',#20225,#20226,#3361,.T.) ;
#24929=EDGE_CURVE('',#20227,#20206,#3362,.T.) ;
#24930=EDGE_CURVE('',#20226,#20227,#1050,.T.) ;
#24931=EDGE_CURVE('',#20228,#20207,#3363,.T.) ;
#24932=EDGE_CURVE('',#20227,#20228,#1051,.T.) ;
#24933=EDGE_CURVE('',#20229,#20210,#3364,.T.) ;
#24934=EDGE_CURVE('',#20228,#20229,#1052,.T.) ;
#24935=EDGE_CURVE('',#20230,#20212,#3365,.T.) ;
#24936=EDGE_CURVE('',#20229,#20230,#1053,.T.) ;
#24937=EDGE_CURVE('',#20231,#20211,#3366,.T.) ;
#24938=EDGE_CURVE('',#20230,#20231,#3367,.T.) ;
#24939=EDGE_CURVE('',#20232,#20233,#1054,.T.) ;
#24940=EDGE_CURVE('',#20233,#20182,#1055,.T.) ;
#24941=EDGE_CURVE('',#20182,#20234,#1056,.T.) ;
#24942=EDGE_CURVE('',#20232,#20234,#1057,.T.) ;
#24943=EDGE_CURVE('',#20181,#20235,#1058,.T.) ;
#24944=EDGE_CURVE('',#20235,#20236,#3368,.T.) ;
#24945=EDGE_CURVE('',#20236,#20180,#179,.T.) ;
#24946=EDGE_CURVE('',#20237,#20238,#3369,.T.) ;
#24947=EDGE_CURVE('',#20238,#20179,#1059,.T.) ;
#24948=EDGE_CURVE('',#20178,#20237,#180,.T.) ;
#24949=EDGE_CURVE('',#20239,#20179,#1060,.T.) ;
#24950=EDGE_CURVE('',#20238,#20240,#1061,.T.) ;
#24951=EDGE_CURVE('',#20240,#20239,#1062,.T.) ;
#24952=EDGE_CURVE('',#20236,#20237,#3370,.T.) ;
#24953=EDGE_CURVE('',#20241,#20239,#1063,.T.) ;
#24954=EDGE_CURVE('',#20240,#20242,#1064,.T.) ;
#24955=EDGE_CURVE('',#20242,#20241,#1065,.T.) ;
#24956=EDGE_CURVE('',#20234,#20241,#1066,.T.) ;
#24957=EDGE_CURVE('',#20242,#20232,#1067,.T.) ;
#24958=EDGE_CURVE('',#20233,#20235,#1068,.T.) ;
#24959=EDGE_CURVE('',#20243,#20244,#3371,.T.) ;
#24960=EDGE_CURVE('',#20244,#20245,#181,.T.) ;
#24961=EDGE_CURVE('',#20245,#20246,#3372,.T.) ;
#24962=EDGE_CURVE('',#20243,#20246,#182,.T.) ;
#24963=EDGE_CURVE('',#20247,#20245,#3373,.T.) ;
#24964=EDGE_CURVE('',#20244,#20248,#3374,.T.) ;
#24965=EDGE_CURVE('',#20248,#20247,#183,.T.) ;
#24966=EDGE_CURVE('',#20246,#20247,#3375,.T.) ;
#24967=EDGE_CURVE('',#20248,#20243,#3376,.T.) ;
#24968=EDGE_CURVE('',#20249,#20246,#3377,.T.) ;
#24969=EDGE_CURVE('',#20250,#20249,#3378,.T.) ;
#24970=EDGE_CURVE('',#20250,#20247,#3379,.T.) ;
#24971=EDGE_CURVE('',#20251,#20245,#3380,.T.) ;
#24972=EDGE_CURVE('',#20249,#20251,#3381,.T.) ;
#24973=EDGE_CURVE('',#20252,#20253,#3382,.T.) ;
#24974=EDGE_CURVE('',#20253,#20254,#184,.T.) ;
#24975=EDGE_CURVE('',#20254,#20255,#3383,.T.) ;
#24976=EDGE_CURVE('',#20252,#20255,#185,.T.) ;
#24977=EDGE_CURVE('',#20256,#20254,#3384,.T.) ;
#24978=EDGE_CURVE('',#20253,#20257,#3385,.T.) ;
#24979=EDGE_CURVE('',#20257,#20256,#186,.T.) ;
#24980=EDGE_CURVE('',#20258,#20256,#3386,.T.) ;
#24981=EDGE_CURVE('',#20257,#20259,#3387,.T.) ;
#24982=EDGE_CURVE('',#20259,#20258,#187,.T.) ;
#24983=EDGE_CURVE('',#20255,#20258,#3388,.T.) ;
#24984=EDGE_CURVE('',#20259,#20252,#3389,.T.) ;
#24985=EDGE_CURVE('',#20260,#20255,#3390,.T.) ;
#24986=EDGE_CURVE('',#20261,#20260,#3391,.T.) ;
#24987=EDGE_CURVE('',#20261,#20258,#3392,.T.) ;
#24988=EDGE_CURVE('',#20262,#20254,#3393,.T.) ;
#24989=EDGE_CURVE('',#20260,#20262,#3394,.T.) ;
#24990=EDGE_CURVE('',#20263,#20264,#3395,.T.) ;
#24991=EDGE_CURVE('',#20264,#20265,#188,.T.) ;
#24992=EDGE_CURVE('',#20265,#20266,#3396,.T.) ;
#24993=EDGE_CURVE('',#20263,#20266,#189,.T.) ;
#24994=EDGE_CURVE('',#20267,#20265,#3397,.T.) ;
#24995=EDGE_CURVE('',#20264,#20268,#3398,.T.) ;
#24996=EDGE_CURVE('',#20268,#20267,#190,.T.) ;
#24997=EDGE_CURVE('',#20266,#20267,#3399,.T.) ;
#24998=EDGE_CURVE('',#20268,#20263,#3400,.T.) ;
#24999=EDGE_CURVE('',#20269,#20266,#3401,.T.) ;
#25000=EDGE_CURVE('',#20270,#20269,#3402,.T.) ;
#25001=EDGE_CURVE('',#20270,#20267,#3403,.T.) ;
#25002=EDGE_CURVE('',#20271,#20265,#3404,.T.) ;
#25003=EDGE_CURVE('',#20269,#20271,#3405,.T.) ;
#25004=EDGE_CURVE('',#20272,#20273,#3406,.T.) ;
#25005=EDGE_CURVE('',#20273,#20223,#1069,.T.) ;
#25006=EDGE_CURVE('',#20272,#20224,#191,.T.) ;
#25007=EDGE_CURVE('',#20273,#20274,#1070,.T.) ;
#25008=EDGE_CURVE('',#20274,#20221,#1071,.T.) ;
#25009=EDGE_CURVE('',#20274,#20275,#1072,.T.) ;
#25010=EDGE_CURVE('',#20275,#20222,#1073,.T.) ;
#25011=EDGE_CURVE('',#20226,#20276,#17506,.T.) ;
#25012=EDGE_CURVE('',#20276,#20277,#3407,.T.) ;
#25013=EDGE_CURVE('',#20277,#20225,#192,.T.) ;
#25014=EDGE_CURVE('',#20275,#20278,#1074,.T.) ;
#25015=EDGE_CURVE('',#20278,#20279,#1075,.T.) ;
#25016=EDGE_CURVE('',#20279,#20222,#1076,.T.) ;
#25017=EDGE_CURVE('',#20278,#20280,#1077,.T.) ;
#25018=EDGE_CURVE('',#20280,#20281,#1078,.T.) ;
#25019=EDGE_CURVE('',#20281,#20279,#1079,.T.) ;
#25020=EDGE_CURVE('',#20280,#20282,#1080,.T.) ;
#25021=EDGE_CURVE('',#20282,#20283,#1081,.T.) ;
#25022=EDGE_CURVE('',#20283,#20281,#1082,.T.) ;
#25023=EDGE_CURVE('',#20282,#20284,#1083,.T.) ;
#25024=EDGE_CURVE('',#20284,#20285,#1084,.T.) ;
#25025=EDGE_CURVE('',#20285,#20283,#1085,.T.) ;
#25026=EDGE_CURVE('',#20284,#20286,#1086,.T.) ;
#25027=EDGE_CURVE('',#20286,#20287,#1087,.T.) ;
#25028=EDGE_CURVE('',#20287,#20285,#1088,.T.) ;
#25029=EDGE_CURVE('',#20231,#20288,#3408,.T.) ;
#25030=EDGE_CURVE('',#20288,#20289,#193,.T.) ;
#25031=EDGE_CURVE('',#20289,#20290,#3409,.T.) ;
#25032=EDGE_CURVE('',#20290,#20231,#194,.T.) ;
#25033=EDGE_CURVE('',#20286,#20291,#3410,.T.) ;
#25034=EDGE_CURVE('',#20291,#20292,#195,.T.) ;
#25035=EDGE_CURVE('',#20292,#20287,#3411,.T.) ;
#25036=EDGE_CURVE('',#20291,#20293,#3412,.T.) ;
#25037=EDGE_CURVE('',#20293,#20294,#196,.T.) ;
#25038=EDGE_CURVE('',#20294,#20292,#3413,.T.) ;
#25039=EDGE_CURVE('',#20288,#20294,#3414,.T.) ;
#25040=EDGE_CURVE('',#20293,#20289,#3415,.T.) ;
#25041=EDGE_CURVE('',#20230,#20295,#17507,.T.) ;
#25042=EDGE_CURVE('',#20295,#20296,#1089,.T.) ;
#25043=EDGE_CURVE('',#20296,#20229,#1090,.T.) ;
#25044=EDGE_CURVE('',#20290,#20295,#3416,.T.) ;
#25045=EDGE_CURVE('',#20296,#20297,#1091,.T.) ;
#25046=EDGE_CURVE('',#20297,#20228,#1092,.T.) ;
#25047=EDGE_CURVE('',#20297,#20298,#1093,.T.) ;
#25048=EDGE_CURVE('',#20298,#20227,#1094,.T.) ;
#25049=EDGE_CURVE('',#20298,#20276,#1095,.T.) ;
#25050=EDGE_CURVE('',#20277,#20272,#3417,.T.) ;
#25051=EDGE_CURVE('',#20279,#20218,#3418,.T.) ;
#25052=EDGE_CURVE('',#20281,#20217,#3419,.T.) ;
#25053=EDGE_CURVE('',#20283,#20216,#3420,.T.) ;
#25054=EDGE_CURVE('',#20285,#20208,#3421,.T.) ;
#25055=EDGE_CURVE('',#20287,#20209,#3422,.T.) ;
#25056=EDGE_CURVE('',#20292,#20215,#3423,.T.) ;
#25057=EDGE_CURVE('',#20294,#20214,#3424,.T.) ;
#25058=EDGE_CURVE('',#20288,#20213,#3425,.T.) ;
#25059=EDGE_CURVE('',#20299,#20300,#3426,.T.) ;
#25060=EDGE_CURVE('',#20301,#20299,#3427,.T.) ;
#25061=EDGE_CURVE('',#20302,#20301,#3428,.T.) ;
#25062=EDGE_CURVE('',#20303,#20302,#197,.T.) ;
#25063=EDGE_CURVE('',#20304,#20303,#3429,.T.) ;
#25064=EDGE_CURVE('',#20305,#20304,#198,.T.) ;
#25065=EDGE_CURVE('',#20306,#20305,#3430,.T.) ;
#25066=EDGE_CURVE('',#20307,#20306,#3431,.T.) ;
#25067=EDGE_CURVE('',#20308,#20307,#17508,.T.) ;
#25068=EDGE_CURVE('',#20307,#20308,#17509,.T.) ;
#25069=EDGE_CURVE('',#20309,#20307,#3432,.T.) ;
#25070=EDGE_CURVE('',#20310,#20309,#3433,.T.) ;
#25071=EDGE_CURVE('',#20311,#20310,#199,.T.) ;
#25072=EDGE_CURVE('',#20312,#20311,#3434,.T.) ;
#25073=EDGE_CURVE('',#20313,#20312,#200,.T.) ;
#25074=EDGE_CURVE('',#20314,#20313,#3435,.T.) ;
#25075=EDGE_CURVE('',#20315,#20314,#3436,.T.) ;
#25076=EDGE_CURVE('',#20316,#20315,#3437,.T.) ;
#25077=EDGE_CURVE('',#20317,#20316,#17510,.T.) ;
#25078=EDGE_CURVE('',#20318,#20317,#3438,.T.) ;
#25079=EDGE_CURVE('',#20319,#20318,#17511,.T.) ;
#25080=EDGE_CURVE('',#20320,#20319,#3439,.T.) ;
#25081=EDGE_CURVE('',#20321,#20320,#17512,.T.) ;
#25082=EDGE_CURVE('',#20322,#20321,#3440,.T.) ;
#25083=EDGE_CURVE('',#20323,#20322,#17513,.T.) ;
#25084=EDGE_CURVE('',#20324,#20323,#3441,.T.) ;
#25085=EDGE_CURVE('',#20325,#20324,#17514,.T.) ;
#25086=EDGE_CURVE('',#20326,#20325,#3442,.T.) ;
#25087=EDGE_CURVE('',#20327,#20326,#17515,.T.) ;
#25088=EDGE_CURVE('',#20328,#20327,#3443,.T.) ;
#25089=EDGE_CURVE('',#20329,#20328,#17516,.T.) ;
#25090=EDGE_CURVE('',#20330,#20329,#3444,.T.) ;
#25091=EDGE_CURVE('',#20331,#20330,#17517,.T.) ;
#25092=EDGE_CURVE('',#20332,#20331,#3445,.T.) ;
#25093=EDGE_CURVE('',#20333,#20332,#17518,.T.) ;
#25094=EDGE_CURVE('',#20334,#20333,#3446,.T.) ;
#25095=EDGE_CURVE('',#20335,#20334,#17519,.T.) ;
#25096=EDGE_CURVE('',#20336,#20335,#3447,.T.) ;
#25097=EDGE_CURVE('',#20337,#20336,#17520,.T.) ;
#25098=EDGE_CURVE('',#20338,#20337,#3448,.T.) ;
#25099=EDGE_CURVE('',#20339,#20338,#17521,.T.) ;
#25100=EDGE_CURVE('',#20340,#20339,#17522,.T.) ;
#25101=EDGE_CURVE('',#20341,#20340,#3449,.T.) ;
#25102=EDGE_CURVE('',#20342,#20341,#17523,.T.) ;
#25103=EDGE_CURVE('',#20343,#20342,#17524,.T.) ;
#25104=EDGE_CURVE('',#20344,#20343,#3450,.T.) ;
#25105=EDGE_CURVE('',#20345,#20344,#17525,.T.) ;
#25106=EDGE_CURVE('',#20346,#20345,#3451,.T.) ;
#25107=EDGE_CURVE('',#20300,#20346,#17526,.T.) ;
#25108=EDGE_CURVE('',#20347,#20348,#3452,.T.) ;
#25109=EDGE_CURVE('',#20349,#20347,#3453,.T.) ;
#25110=EDGE_CURVE('',#20348,#20349,#3454,.T.) ;
#25111=EDGE_CURVE('',#20350,#20351,#3455,.T.) ;
#25112=EDGE_CURVE('',#20352,#20350,#3456,.T.) ;
#25113=EDGE_CURVE('',#20351,#20352,#3457,.T.) ;
#25114=EDGE_CURVE('',#20353,#20354,#17527,.T.) ;
#25115=EDGE_CURVE('',#20355,#20353,#3458,.T.) ;
#25116=EDGE_CURVE('',#20356,#20355,#17528,.T.) ;
#25117=EDGE_CURVE('',#20357,#20356,#3459,.T.) ;
#25118=EDGE_CURVE('',#20358,#20357,#17529,.T.) ;
#25119=EDGE_CURVE('',#20359,#20358,#3460,.T.) ;
#25120=EDGE_CURVE('',#20360,#20359,#3461,.T.) ;
#25121=EDGE_CURVE('',#20361,#20360,#17530,.T.) ;
#25122=EDGE_CURVE('',#20362,#20361,#3462,.T.) ;
#25123=EDGE_CURVE('',#20363,#20362,#17531,.T.) ;
#25124=EDGE_CURVE('',#20364,#20363,#3463,.T.) ;
#25125=EDGE_CURVE('',#20365,#20364,#3464,.T.) ;
#25126=EDGE_CURVE('',#20366,#20365,#17532,.T.) ;
#25127=EDGE_CURVE('',#20354,#20366,#3465,.T.) ;
#25128=EDGE_CURVE('',#20367,#20368,#3466,.T.) ;
#25129=EDGE_CURVE('',#20369,#20368,#3467,.T.) ;
#25130=EDGE_CURVE('',#20370,#20369,#3468,.T.) ;
#25131=EDGE_CURVE('',#20371,#20370,#3469,.T.) ;
#25132=EDGE_CURVE('',#20371,#20372,#3470,.T.) ;
#25133=EDGE_CURVE('',#20373,#20372,#17533,.T.) ;
#25134=EDGE_CURVE('',#20374,#20373,#3471,.T.) ;
#25135=EDGE_CURVE('',#20375,#20374,#17534,.T.) ;
#25136=EDGE_CURVE('',#20376,#20375,#3472,.T.) ;
#25137=EDGE_CURVE('',#20377,#20376,#17535,.T.) ;
#25138=EDGE_CURVE('',#20378,#20377,#3473,.T.) ;
#25139=EDGE_CURVE('',#20379,#20378,#17536,.T.) ;
#25140=EDGE_CURVE('',#20380,#20379,#3474,.T.) ;
#25141=EDGE_CURVE('',#20381,#20380,#17537,.T.) ;
#25142=EDGE_CURVE('',#20382,#20381,#3475,.T.) ;
#25143=EDGE_CURVE('',#20367,#20382,#17538,.T.) ;
#25144=EDGE_CURVE('',#20383,#20384,#17539,.T.) ;
#25145=EDGE_CURVE('',#20385,#20383,#3476,.T.) ;
#25146=EDGE_CURVE('',#20386,#20385,#3477,.T.) ;
#25147=EDGE_CURVE('',#20387,#20386,#17540,.T.) ;
#25148=EDGE_CURVE('',#20388,#20387,#3478,.T.) ;
#25149=EDGE_CURVE('',#20389,#20388,#17541,.T.) ;
#25150=EDGE_CURVE('',#20390,#20389,#3479,.T.) ;
#25151=EDGE_CURVE('',#20391,#20390,#3480,.T.) ;
#25152=EDGE_CURVE('',#20392,#20391,#17542,.T.) ;
#25153=EDGE_CURVE('',#20393,#20392,#3481,.T.) ;
#25154=EDGE_CURVE('',#20394,#20393,#17543,.T.) ;
#25155=EDGE_CURVE('',#20395,#20394,#3482,.T.) ;
#25156=EDGE_CURVE('',#20396,#20395,#17544,.T.) ;
#25157=EDGE_CURVE('',#20384,#20396,#3483,.T.) ;
#25158=EDGE_CURVE('',#20397,#20398,#17545,.T.) ;
#25159=EDGE_CURVE('',#20399,#20397,#3484,.T.) ;
#25160=EDGE_CURVE('',#20400,#20399,#3485,.T.) ;
#25161=EDGE_CURVE('',#20401,#20400,#17546,.T.) ;
#25162=EDGE_CURVE('',#20402,#20401,#3486,.T.) ;
#25163=EDGE_CURVE('',#20403,#20402,#17547,.T.) ;
#25164=EDGE_CURVE('',#20404,#20403,#3487,.T.) ;
#25165=EDGE_CURVE('',#20405,#20404,#3488,.T.) ;
#25166=EDGE_CURVE('',#20406,#20405,#17548,.T.) ;
#25167=EDGE_CURVE('',#20407,#20406,#3489,.T.) ;
#25168=EDGE_CURVE('',#20408,#20407,#17549,.T.) ;
#25169=EDGE_CURVE('',#20409,#20408,#3490,.T.) ;
#25170=EDGE_CURVE('',#20410,#20409,#17550,.T.) ;
#25171=EDGE_CURVE('',#20398,#20410,#3491,.T.) ;
#25172=EDGE_CURVE('',#20411,#20412,#3492,.T.) ;
#25173=EDGE_CURVE('',#20413,#20412,#3493,.T.) ;
#25174=EDGE_CURVE('',#20414,#20413,#3494,.T.) ;
#25175=EDGE_CURVE('',#20415,#20414,#3495,.T.) ;
#25176=EDGE_CURVE('',#20415,#20416,#3496,.T.) ;
#25177=EDGE_CURVE('',#20417,#20416,#3497,.T.) ;
#25178=EDGE_CURVE('',#20418,#20417,#17551,.T.) ;
#25179=EDGE_CURVE('',#20419,#20418,#3498,.T.) ;
#25180=EDGE_CURVE('',#20420,#20419,#17552,.T.) ;
#25181=EDGE_CURVE('',#20421,#20420,#3499,.T.) ;
#25182=EDGE_CURVE('',#20422,#20421,#17553,.T.) ;
#25183=EDGE_CURVE('',#20423,#20422,#3500,.T.) ;
#25184=EDGE_CURVE('',#20424,#20423,#17554,.T.) ;
#25185=EDGE_CURVE('',#20411,#20424,#3501,.T.) ;
#25186=EDGE_CURVE('',#20425,#20425,#17555,.T.) ;
#25187=EDGE_CURVE('',#20426,#20427,#3502,.T.) ;
#25188=EDGE_CURVE('',#20428,#20427,#17556,.T.) ;
#25189=EDGE_CURVE('',#20429,#20428,#3503,.T.) ;
#25190=EDGE_CURVE('',#20430,#20429,#17557,.T.) ;
#25191=EDGE_CURVE('',#20431,#20430,#3504,.T.) ;
#25192=EDGE_CURVE('',#20432,#20431,#17558,.T.) ;
#25193=EDGE_CURVE('',#20433,#20432,#3505,.T.) ;
#25194=EDGE_CURVE('',#20434,#20433,#17559,.T.) ;
#25195=EDGE_CURVE('',#20435,#20434,#3506,.T.) ;
#25196=EDGE_CURVE('',#20436,#20435,#17560,.T.) ;
#25197=EDGE_CURVE('',#20437,#20436,#3507,.T.) ;
#25198=EDGE_CURVE('',#20437,#20438,#3508,.T.) ;
#25199=EDGE_CURVE('',#20439,#20438,#3509,.T.) ;
#25200=EDGE_CURVE('',#20440,#20439,#3510,.T.) ;
#25201=EDGE_CURVE('',#20426,#20440,#3511,.T.) ;
#25202=EDGE_CURVE('',#20441,#20441,#17561,.T.) ;
#25203=EDGE_CURVE('',#20442,#20442,#17562,.T.) ;
#25204=EDGE_CURVE('',#20443,#20444,#3512,.T.) ;
#25205=EDGE_CURVE('',#20443,#20445,#3513,.T.) ;
#25206=EDGE_CURVE('',#20446,#20445,#3514,.T.) ;
#25207=EDGE_CURVE('',#20447,#20446,#17563,.T.) ;
#25208=EDGE_CURVE('',#20448,#20447,#3515,.T.) ;
#25209=EDGE_CURVE('',#20449,#20448,#17564,.T.) ;
#25210=EDGE_CURVE('',#20450,#20449,#3516,.T.) ;
#25211=EDGE_CURVE('',#20451,#20450,#17565,.T.) ;
#25212=EDGE_CURVE('',#20452,#20451,#3517,.T.) ;
#25213=EDGE_CURVE('',#20453,#20452,#17566,.T.) ;
#25214=EDGE_CURVE('',#20454,#20453,#3518,.T.) ;
#25215=EDGE_CURVE('',#20454,#20455,#3519,.T.) ;
#25216=EDGE_CURVE('',#20456,#20455,#3520,.T.) ;
#25217=EDGE_CURVE('',#20444,#20456,#3521,.T.) ;
#25218=EDGE_CURVE('',#20457,#20457,#17567,.T.) ;
#25219=EDGE_CURVE('',#20458,#20458,#17568,.T.) ;
#25220=EDGE_CURVE('',#20459,#20460,#17569,.T.) ;
#25221=EDGE_CURVE('',#20461,#20459,#3522,.T.) ;
#25222=EDGE_CURVE('',#20462,#20461,#17570,.T.) ;
#25223=EDGE_CURVE('',#20463,#20462,#3523,.T.) ;
#25224=EDGE_CURVE('',#20464,#20463,#17571,.T.) ;
#25225=EDGE_CURVE('',#20465,#20464,#3524,.T.) ;
#25226=EDGE_CURVE('',#20466,#20465,#17572,.T.) ;
#25227=EDGE_CURVE('',#20460,#20466,#3525,.T.) ;
#25228=EDGE_CURVE('',#20467,#20468,#17573,.T.) ;
#25229=EDGE_CURVE('',#20469,#20467,#3526,.T.) ;
#25230=EDGE_CURVE('',#20470,#20469,#17574,.T.) ;
#25231=EDGE_CURVE('',#20471,#20470,#3527,.T.) ;
#25232=EDGE_CURVE('',#20472,#20471,#17575,.T.) ;
#25233=EDGE_CURVE('',#20473,#20472,#3528,.T.) ;
#25234=EDGE_CURVE('',#20474,#20473,#3529,.T.) ;
#25235=EDGE_CURVE('',#20475,#20474,#17576,.T.) ;
#25236=EDGE_CURVE('',#20476,#20475,#3530,.T.) ;
#25237=EDGE_CURVE('',#20477,#20476,#17577,.T.) ;
#25238=EDGE_CURVE('',#20478,#20477,#3531,.T.) ;
#25239=EDGE_CURVE('',#20479,#20478,#3532,.T.) ;
#25240=EDGE_CURVE('',#20480,#20479,#17578,.T.) ;
#25241=EDGE_CURVE('',#20468,#20480,#3533,.T.) ;
#25242=EDGE_CURVE('',#20481,#20482,#3534,.T.) ;
#25243=EDGE_CURVE('',#20483,#20481,#3535,.T.) ;
#25244=EDGE_CURVE('',#20484,#20483,#3536,.T.) ;
#25245=EDGE_CURVE('',#20482,#20484,#3537,.T.) ;
#25246=EDGE_CURVE('',#20348,#20249,#201,.T.) ;
#25247=EDGE_CURVE('',#20251,#20347,#202,.T.) ;
#25248=EDGE_CURVE('',#20349,#20250,#203,.T.) ;
#25249=EDGE_CURVE('',#20251,#20250,#3538,.T.) ;
#25250=EDGE_CURVE('',#20482,#20260,#204,.T.) ;
#25251=EDGE_CURVE('',#20262,#20481,#205,.T.) ;
#25252=EDGE_CURVE('',#20484,#20261,#206,.T.) ;
#25253=EDGE_CURVE('',#20485,#20261,#3539,.T.) ;
#25254=EDGE_CURVE('',#20483,#20485,#207,.T.) ;
#25255=EDGE_CURVE('',#20262,#20485,#3540,.T.) ;
#25256=EDGE_CURVE('',#20485,#20256,#3541,.T.) ;
#25257=EDGE_CURVE('',#20351,#20269,#208,.T.) ;
#25258=EDGE_CURVE('',#20271,#20350,#209,.T.) ;
#25259=EDGE_CURVE('',#20352,#20270,#210,.T.) ;
#25260=EDGE_CURVE('',#20271,#20270,#3542,.T.) ;
#25261=EDGE_CURVE('',#20239,#20164,#3543,.T.) ;
#25262=EDGE_CURVE('',#20241,#20165,#3544,.T.) ;
#25263=EDGE_CURVE('',#20234,#20176,#3545,.T.) ;
#25264=EDGE_CURVE('',#20486,#20487,#17579,.T.) ;
#25265=EDGE_CURVE('',#20487,#20488,#17580,.T.) ;
#25266=EDGE_CURVE('',#20488,#20488,#17581,.T.) ;
#25267=EDGE_CURVE('',#20487,#20486,#17582,.T.) ;
#25268=EDGE_CURVE('',#20489,#20489,#17583,.T.) ;
#25269=EDGE_CURVE('',#20486,#20490,#3546,.T.) ;
#25270=EDGE_CURVE('',#20490,#20490,#17584,.T.) ;
#25271=EDGE_CURVE('',#20491,#20491,#17585,.T.) ;
#25272=EDGE_CURVE('',#20491,#20489,#17586,.T.) ;
#25273=EDGE_CURVE('',#20492,#20492,#17587,.T.) ;
#25274=EDGE_CURVE('',#20492,#20491,#3547,.T.) ;
#25275=EDGE_CURVE('',#20493,#20493,#17588,.T.) ;
#25276=EDGE_CURVE('',#20493,#20492,#17589,.T.) ;
#25277=EDGE_CURVE('',#20494,#20495,#3548,.T.) ;
#25278=EDGE_CURVE('',#20496,#20494,#17590,.T.) ;
#25279=EDGE_CURVE('',#20497,#20496,#3549,.T.) ;
#25280=EDGE_CURVE('',#20498,#20497,#3550,.T.) ;
#25281=EDGE_CURVE('',#20498,#20499,#3551,.T.) ;
#25282=EDGE_CURVE('',#20499,#20500,#3552,.T.) ;
#25283=EDGE_CURVE('',#20501,#20500,#3553,.T.) ;
#25284=EDGE_CURVE('',#20502,#20501,#17591,.T.) ;
#25285=EDGE_CURVE('',#20503,#20502,#3554,.T.) ;
#25286=EDGE_CURVE('',#20504,#20503,#17592,.T.) ;
#25287=EDGE_CURVE('',#20505,#20504,#3555,.T.) ;
#25288=EDGE_CURVE('',#20506,#20505,#17593,.T.) ;
#25289=EDGE_CURVE('',#20507,#20506,#3556,.T.) ;
#25290=EDGE_CURVE('',#20508,#20507,#3557,.T.) ;
#25291=EDGE_CURVE('',#20508,#20509,#211,.T.) ;
#25292=EDGE_CURVE('',#20510,#20509,#3558,.F.) ;
#25293=EDGE_CURVE('',#20510,#20511,#212,.T.) ;
#25294=EDGE_CURVE('',#20512,#20511,#3559,.F.) ;
#25295=EDGE_CURVE('',#20513,#20512,#3560,.T.) ;
#25296=EDGE_CURVE('',#20514,#20513,#3561,.T.) ;
#25297=EDGE_CURVE('',#20514,#20515,#213,.T.) ;
#25298=EDGE_CURVE('',#20516,#20515,#3562,.F.) ;
#25299=EDGE_CURVE('',#20516,#20517,#214,.T.) ;
#25300=EDGE_CURVE('',#20518,#20517,#3563,.T.) ;
#25301=EDGE_CURVE('',#20519,#20518,#3564,.T.) ;
#25302=EDGE_CURVE('',#20520,#20519,#17594,.T.) ;
#25303=EDGE_CURVE('',#20521,#20520,#3565,.T.) ;
#25304=EDGE_CURVE('',#20522,#20521,#17595,.T.) ;
#25305=EDGE_CURVE('',#20523,#20522,#3566,.T.) ;
#25306=EDGE_CURVE('',#20524,#20523,#17596,.T.) ;
#25307=EDGE_CURVE('',#20525,#20524,#17597,.T.) ;
#25308=EDGE_CURVE('',#20526,#20525,#3567,.T.) ;
#25309=EDGE_CURVE('',#20527,#20526,#17598,.T.) ;
#25310=EDGE_CURVE('',#20528,#20527,#17599,.T.) ;
#25311=EDGE_CURVE('',#20529,#20528,#3568,.T.) ;
#25312=EDGE_CURVE('',#20530,#20529,#17600,.T.) ;
#25313=EDGE_CURVE('',#20531,#20530,#3569,.T.) ;
#25314=EDGE_CURVE('',#20532,#20531,#17601,.T.) ;
#25315=EDGE_CURVE('',#20533,#20532,#3570,.T.) ;
#25316=EDGE_CURVE('',#20534,#20533,#17602,.T.) ;
#25317=EDGE_CURVE('',#20535,#20534,#3571,.T.) ;
#25318=EDGE_CURVE('',#20536,#20535,#17603,.T.) ;
#25319=EDGE_CURVE('',#20537,#20536,#3572,.T.) ;
#25320=EDGE_CURVE('',#20538,#20537,#17604,.T.) ;
#25321=EDGE_CURVE('',#20539,#20538,#3573,.T.) ;
#25322=EDGE_CURVE('',#20540,#20539,#17605,.T.) ;
#25323=EDGE_CURVE('',#20541,#20540,#3574,.T.) ;
#25324=EDGE_CURVE('',#20542,#20541,#17606,.T.) ;
#25325=EDGE_CURVE('',#20543,#20542,#3575,.T.) ;
#25326=EDGE_CURVE('',#20544,#20543,#1096,.T.) ;
#25327=EDGE_CURVE('',#20544,#20545,#3576,.T.) ;
#25328=EDGE_CURVE('',#20546,#20545,#1097,.T.) ;
#25329=EDGE_CURVE('',#20547,#20546,#3577,.T.) ;
#25330=EDGE_CURVE('',#20548,#20547,#17607,.T.) ;
#25331=EDGE_CURVE('',#20549,#20548,#3578,.T.) ;
#25332=EDGE_CURVE('',#20550,#20549,#17608,.T.) ;
#25333=EDGE_CURVE('',#20495,#20550,#3579,.T.) ;
#25334=EDGE_CURVE('',#20551,#20551,#17609,.T.) ;
#25335=EDGE_CURVE('',#20552,#20553,#3580,.T.) ;
#25336=EDGE_CURVE('',#20554,#20552,#3581,.T.) ;
#25337=EDGE_CURVE('',#20555,#20554,#17610,.T.) ;
#25338=EDGE_CURVE('',#20556,#20555,#3582,.T.) ;
#25339=EDGE_CURVE('',#20557,#20556,#17611,.T.) ;
#25340=EDGE_CURVE('',#20558,#20557,#3583,.T.) ;
#25341=EDGE_CURVE('',#20559,#20558,#3584,.T.) ;
#25342=EDGE_CURVE('',#20560,#20559,#17612,.T.) ;
#25343=EDGE_CURVE('',#20561,#20560,#3585,.T.) ;
#25344=EDGE_CURVE('',#20562,#20561,#17613,.T.) ;
#25345=EDGE_CURVE('',#20563,#20562,#3586,.T.) ;
#25346=EDGE_CURVE('',#20564,#20563,#17614,.T.) ;
#25347=EDGE_CURVE('',#20565,#20564,#3587,.T.) ;
#25348=EDGE_CURVE('',#20553,#20565,#17615,.T.) ;
#25349=EDGE_CURVE('',#20566,#20566,#17616,.T.) ;
#25350=EDGE_CURVE('',#20567,#20567,#17617,.T.) ;
#25351=EDGE_CURVE('',#20568,#20569,#3588,.T.) ;
#25352=EDGE_CURVE('',#20570,#20568,#3589,.T.) ;
#25353=EDGE_CURVE('',#20571,#20570,#17618,.T.) ;
#25354=EDGE_CURVE('',#20572,#20571,#3590,.T.) ;
#25355=EDGE_CURVE('',#20573,#20572,#17619,.T.) ;
#25356=EDGE_CURVE('',#20574,#20573,#3591,.T.) ;
#25357=EDGE_CURVE('',#20575,#20574,#17620,.T.) ;
#25358=EDGE_CURVE('',#20576,#20575,#3592,.T.) ;
#25359=EDGE_CURVE('',#20577,#20576,#17621,.T.) ;
#25360=EDGE_CURVE('',#20578,#20577,#3593,.T.) ;
#25361=EDGE_CURVE('',#20579,#20578,#17622,.T.) ;
#25362=EDGE_CURVE('',#20580,#20579,#3594,.T.) ;
#25363=EDGE_CURVE('',#20581,#20580,#17623,.T.) ;
#25364=EDGE_CURVE('',#20582,#20581,#3595,.T.) ;
#25365=EDGE_CURVE('',#20583,#20582,#3596,.T.) ;
#25366=EDGE_CURVE('',#20583,#20569,#3597,.T.) ;
#25367=EDGE_CURVE('',#20584,#20584,#17624,.T.) ;
#25368=EDGE_CURVE('',#20585,#20586,#3598,.T.) ;
#25369=EDGE_CURVE('',#20587,#20586,#17625,.T.) ;
#25370=EDGE_CURVE('',#20588,#20587,#3599,.T.) ;
#25371=EDGE_CURVE('',#20589,#20588,#17626,.T.) ;
#25372=EDGE_CURVE('',#20589,#20590,#3600,.T.) ;
#25373=EDGE_CURVE('',#20591,#20590,#17627,.T.) ;
#25374=EDGE_CURVE('',#20592,#20591,#3601,.T.) ;
#25375=EDGE_CURVE('',#20593,#20592,#17628,.T.) ;
#25376=EDGE_CURVE('',#20593,#20594,#3602,.T.) ;
#25377=EDGE_CURVE('',#20595,#20594,#17629,.T.) ;
#25378=EDGE_CURVE('',#20595,#20596,#3603,.T.) ;
#25379=EDGE_CURVE('',#20596,#20597,#3604,.T.) ;
#25380=EDGE_CURVE('',#20597,#20598,#3605,.T.) ;
#25381=EDGE_CURVE('',#20585,#20598,#17630,.T.) ;
#25382=EDGE_CURVE('',#20599,#20600,#17631,.T.) ;
#25383=EDGE_CURVE('',#20601,#20599,#3606,.T.) ;
#25384=EDGE_CURVE('',#20602,#20601,#17632,.T.) ;
#25385=EDGE_CURVE('',#20603,#20602,#3607,.T.) ;
#25386=EDGE_CURVE('',#20604,#20603,#17633,.T.) ;
#25387=EDGE_CURVE('',#20605,#20604,#3608,.T.) ;
#25388=EDGE_CURVE('',#20606,#20605,#17634,.T.) ;
#25389=EDGE_CURVE('',#20600,#20606,#3609,.T.) ;
#25390=EDGE_CURVE('',#20607,#20608,#3610,.T.) ;
#25391=EDGE_CURVE('',#20608,#20609,#3611,.T.) ;
#25392=EDGE_CURVE('',#20609,#20610,#3612,.T.) ;
#25393=EDGE_CURVE('',#20611,#20610,#1098,.T.) ;
#25394=EDGE_CURVE('',#20612,#20611,#3613,.T.) ;
#25395=EDGE_CURVE('',#20613,#20612,#17635,.T.) ;
#25396=EDGE_CURVE('',#20614,#20613,#3614,.T.) ;
#25397=EDGE_CURVE('',#20615,#20614,#17636,.T.) ;
#25398=EDGE_CURVE('',#20616,#20615,#3615,.T.) ;
#25399=EDGE_CURVE('',#20617,#20616,#17637,.T.) ;
#25400=EDGE_CURVE('',#20618,#20617,#3616,.T.) ;
#25401=EDGE_CURVE('',#20619,#20618,#17638,.T.) ;
#25402=EDGE_CURVE('',#20620,#20619,#3617,.T.) ;
#25403=EDGE_CURVE('',#20607,#20620,#1099,.T.) ;
#25404=EDGE_CURVE('',#20621,#20622,#3618,.T.) ;
#25405=EDGE_CURVE('',#20623,#20622,#1100,.T.) ;
#25406=EDGE_CURVE('',#20624,#20623,#3619,.T.) ;
#25407=EDGE_CURVE('',#20625,#20624,#3620,.T.) ;
#25408=EDGE_CURVE('',#20626,#20625,#17639,.T.) ;
#25409=EDGE_CURVE('',#20627,#20626,#3621,.T.) ;
#25410=EDGE_CURVE('',#20628,#20627,#17640,.T.) ;
#25411=EDGE_CURVE('',#20629,#20628,#3622,.T.) ;
#25412=EDGE_CURVE('',#20630,#20629,#17641,.T.) ;
#25413=EDGE_CURVE('',#20631,#20630,#3623,.T.) ;
#25414=EDGE_CURVE('',#20632,#20631,#17642,.T.) ;
#25415=EDGE_CURVE('',#20633,#20632,#3624,.T.) ;
#25416=EDGE_CURVE('',#20634,#20633,#3625,.T.) ;
#25417=EDGE_CURVE('',#20621,#20634,#1101,.T.) ;
#25418=EDGE_CURVE('',#20635,#20636,#17643,.T.) ;
#25419=EDGE_CURVE('',#20637,#20635,#3626,.T.) ;
#25420=EDGE_CURVE('',#20638,#20637,#17644,.T.) ;
#25421=EDGE_CURVE('',#20639,#20638,#3627,.T.) ;
#25422=EDGE_CURVE('',#20640,#20639,#17645,.T.) ;
#25423=EDGE_CURVE('',#20641,#20640,#3628,.T.) ;
#25424=EDGE_CURVE('',#20642,#20641,#17646,.T.) ;
#25425=EDGE_CURVE('',#20643,#20642,#3629,.T.) ;
#25426=EDGE_CURVE('',#20644,#20643,#3630,.T.) ;
#25427=EDGE_CURVE('',#20645,#20644,#17647,.T.) ;
#25428=EDGE_CURVE('',#20646,#20645,#3631,.T.) ;
#25429=EDGE_CURVE('',#20647,#20646,#17648,.T.) ;
#25430=EDGE_CURVE('',#20648,#20647,#3632,.T.) ;
#25431=EDGE_CURVE('',#20636,#20648,#3633,.T.) ;
#25432=EDGE_CURVE('',#20649,#20650,#17649,.T.) ;
#25433=EDGE_CURVE('',#20651,#20649,#3634,.T.) ;
#25434=EDGE_CURVE('',#20652,#20651,#17650,.T.) ;
#25435=EDGE_CURVE('',#20653,#20652,#3635,.T.) ;
#25436=EDGE_CURVE('',#20654,#20653,#17651,.T.) ;
#25437=EDGE_CURVE('',#20655,#20654,#3636,.T.) ;
#25438=EDGE_CURVE('',#20656,#20655,#17652,.T.) ;
#25439=EDGE_CURVE('',#20657,#20656,#3637,.T.) ;
#25440=EDGE_CURVE('',#20658,#20657,#3638,.T.) ;
#25441=EDGE_CURVE('',#20659,#20658,#17653,.T.) ;
#25442=EDGE_CURVE('',#20660,#20659,#3639,.T.) ;
#25443=EDGE_CURVE('',#20661,#20660,#17654,.T.) ;
#25444=EDGE_CURVE('',#20662,#20661,#3640,.T.) ;
#25445=EDGE_CURVE('',#20650,#20662,#3641,.T.) ;
#25446=EDGE_CURVE('',#20663,#20663,#1102,.T.) ;
#25447=EDGE_CURVE('',#20664,#20665,#17655,.T.) ;
#25448=EDGE_CURVE('',#20495,#20665,#17656,.T.) ;
#25449=EDGE_CURVE('',#20495,#20666,#17657,.T.) ;
#25450=EDGE_CURVE('',#20666,#20664,#17658,.T.) ;
#25451=EDGE_CURVE('',#20667,#20668,#17659,.T.) ;
#25452=EDGE_CURVE('',#20668,#20665,#3642,.T.) ;
#25453=EDGE_CURVE('',#20664,#20667,#3643,.T.) ;
#25454=EDGE_CURVE('',#20669,#20670,#17660,.T.) ;
#25455=EDGE_CURVE('',#20670,#20668,#17661,.T.) ;
#25456=EDGE_CURVE('',#20667,#20669,#17662,.T.) ;
#25457=EDGE_CURVE('',#20671,#20672,#17663,.T.) ;
#25458=EDGE_CURVE('',#20672,#20670,#3644,.T.) ;
#25459=EDGE_CURVE('',#20669,#20671,#3645,.T.) ;
#25460=EDGE_CURVE('',#20673,#20674,#17664,.T.) ;
#25461=EDGE_CURVE('',#20674,#20672,#17665,.T.) ;
#25462=EDGE_CURVE('',#20671,#20673,#17666,.T.) ;
#25463=EDGE_CURVE('',#20675,#20676,#17667,.T.) ;
#25464=EDGE_CURVE('',#20676,#20674,#3646,.T.) ;
#25465=EDGE_CURVE('',#20673,#20675,#3647,.T.) ;
#25466=EDGE_CURVE('',#20677,#20678,#17668,.T.) ;
#25467=EDGE_CURVE('',#20678,#20676,#17669,.T.) ;
#25468=EDGE_CURVE('',#20675,#20677,#17670,.T.) ;
#25469=EDGE_CURVE('',#20679,#20680,#17671,.T.) ;
#25470=EDGE_CURVE('',#20680,#20678,#3648,.T.) ;
#25471=EDGE_CURVE('',#20677,#20679,#3649,.T.) ;
#25472=EDGE_CURVE('',#20681,#20682,#17672,.T.) ;
#25473=EDGE_CURVE('',#20682,#20680,#17673,.T.) ;
#25474=EDGE_CURVE('',#20679,#20681,#17674,.T.) ;
#25475=EDGE_CURVE('',#20683,#20684,#17675,.T.) ;
#25476=EDGE_CURVE('',#20684,#20682,#3650,.T.) ;
#25477=EDGE_CURVE('',#20681,#20683,#3651,.T.) ;
#25478=EDGE_CURVE('',#20685,#20686,#17676,.T.) ;
#25479=EDGE_CURVE('',#20686,#20684,#17677,.T.) ;
#25480=EDGE_CURVE('',#20683,#20685,#17678,.T.) ;
#25481=EDGE_CURVE('',#20687,#20688,#17679,.T.) ;
#25482=EDGE_CURVE('',#20688,#20686,#3652,.T.) ;
#25483=EDGE_CURVE('',#20685,#20687,#3653,.T.) ;
#25484=EDGE_CURVE('',#20687,#20689,#17680,.T.) ;
#25485=EDGE_CURVE('',#20689,#20518,#17681,.T.) ;
#25486=EDGE_CURVE('',#20688,#20518,#17682,.T.) ;
#25487=EDGE_CURVE('',#20690,#20685,#3654,.T.) ;
#25488=EDGE_CURVE('',#20691,#20690,#3655,.T.) ;
#25489=EDGE_CURVE('',#20692,#20691,#17683,.T.) ;
#25490=EDGE_CURVE('',#20693,#20692,#3656,.T.) ;
#25491=EDGE_CURVE('',#20694,#20693,#3657,.T.) ;
#25492=EDGE_CURVE('',#20689,#20694,#3658,.T.) ;
#25493=EDGE_CURVE('',#20683,#20695,#3659,.T.) ;
#25494=EDGE_CURVE('',#20690,#20695,#17684,.T.) ;
#25495=EDGE_CURVE('',#20696,#20681,#3660,.T.) ;
#25496=EDGE_CURVE('',#20695,#20696,#3661,.T.) ;
#25497=EDGE_CURVE('',#20679,#20697,#3662,.T.) ;
#25498=EDGE_CURVE('',#20696,#20697,#17685,.T.) ;
#25499=EDGE_CURVE('',#20677,#20698,#3663,.T.) ;
#25500=EDGE_CURVE('',#20697,#20698,#3664,.T.) ;
#25501=EDGE_CURVE('',#20675,#20699,#3665,.T.) ;
#25502=EDGE_CURVE('',#20698,#20699,#17686,.T.) ;
#25503=EDGE_CURVE('',#20700,#20673,#3666,.T.) ;
#25504=EDGE_CURVE('',#20699,#20700,#3667,.T.) ;
#25505=EDGE_CURVE('',#20671,#20701,#3668,.T.) ;
#25506=EDGE_CURVE('',#20700,#20701,#17687,.T.) ;
#25507=EDGE_CURVE('',#20702,#20669,#3669,.T.) ;
#25508=EDGE_CURVE('',#20701,#20702,#3670,.T.) ;
#25509=EDGE_CURVE('',#20667,#20703,#3671,.T.) ;
#25510=EDGE_CURVE('',#20702,#20703,#17688,.T.) ;
#25511=EDGE_CURVE('',#20704,#20666,#3672,.T.) ;
#25512=EDGE_CURVE('',#20705,#20704,#3673,.T.) ;
#25513=EDGE_CURVE('',#20706,#20705,#3674,.T.) ;
#25514=EDGE_CURVE('',#20707,#20706,#17689,.T.) ;
#25515=EDGE_CURVE('',#20703,#20707,#3675,.T.) ;
#25516=EDGE_CURVE('',#20551,#20708,#17690,.T.) ;
#25517=EDGE_CURVE('',#20708,#20708,#17691,.T.) ;
#25518=EDGE_CURVE('',#20708,#20709,#3676,.T.) ;
#25519=EDGE_CURVE('',#20709,#20709,#17692,.T.) ;
#25520=EDGE_CURVE('',#20663,#20710,#1103,.T.) ;
#25521=EDGE_CURVE('',#20710,#20711,#1104,.T.) ;
#25522=EDGE_CURVE('',#20711,#20710,#3677,.T.) ;
#25523=EDGE_CURVE('',#20711,#20712,#17693,.T.) ;
#25524=EDGE_CURVE('',#20712,#20712,#17694,.T.) ;
#25525=EDGE_CURVE('',#20713,#20713,#17695,.T.) ;
#25526=EDGE_CURVE('',#20714,#20715,#17696,.T.) ;
#25527=EDGE_CURVE('',#20715,#20713,#17697,.T.) ;
#25528=EDGE_CURVE('',#20715,#20714,#17698,.T.) ;
#25529=EDGE_CURVE('',#20714,#20716,#3678,.T.) ;
#25530=EDGE_CURVE('',#20716,#20716,#17699,.T.) ;
#25531=EDGE_CURVE('',#20717,#20717,#17700,.T.) ;
#25532=EDGE_CURVE('',#20717,#20718,#17701,.T.) ;
#25533=EDGE_CURVE('',#20718,#20719,#17702,.T.) ;
#25534=EDGE_CURVE('',#20719,#20718,#17703,.T.) ;
#25535=EDGE_CURVE('',#20719,#20720,#3679,.T.) ;
#25536=EDGE_CURVE('',#20721,#20720,#17704,.T.) ;
#25537=EDGE_CURVE('',#20720,#20721,#17705,.T.) ;
#25538=EDGE_CURVE('',#20722,#20723,#3680,.T.) ;
#25539=EDGE_CURVE('',#20724,#20722,#3681,.T.) ;
#25540=EDGE_CURVE('',#20725,#20724,#215,.T.) ;
#25541=EDGE_CURVE('',#20725,#20726,#3682,.T.) ;
#25542=EDGE_CURVE('',#20727,#20726,#216,.T.) ;
#25543=EDGE_CURVE('',#20723,#20727,#3683,.T.) ;
#25544=EDGE_CURVE('',#20728,#20728,#17706,.T.) ;
#25545=EDGE_CURVE('',#20728,#20721,#17707,.T.) ;
#25546=EDGE_CURVE('',#20729,#20730,#1105,.T.) ;
#25547=EDGE_CURVE('',#20730,#20516,#3684,.T.) ;
#25548=EDGE_CURVE('',#20515,#20731,#3685,.T.) ;
#25549=EDGE_CURVE('',#20731,#20732,#1106,.T.) ;
#25550=EDGE_CURVE('',#20729,#20732,#3686,.T.) ;
#25551=EDGE_CURVE('',#20733,#20733,#17708,.T.) ;
#25552=EDGE_CURVE('',#20733,#20734,#17709,.T.) ;
#25553=EDGE_CURVE('',#20734,#20735,#17710,.T.) ;
#25554=EDGE_CURVE('',#20735,#20734,#17711,.T.) ;
#25555=EDGE_CURVE('',#20735,#20736,#3687,.T.) ;
#25556=EDGE_CURVE('',#20737,#20736,#17712,.T.) ;
#25557=EDGE_CURVE('',#20736,#20737,#17713,.T.) ;
#25558=EDGE_CURVE('',#20738,#20739,#3688,.T.) ;
#25559=EDGE_CURVE('',#20740,#20738,#3689,.T.) ;
#25560=EDGE_CURVE('',#20741,#20740,#217,.T.) ;
#25561=EDGE_CURVE('',#20741,#20742,#3690,.T.) ;
#25562=EDGE_CURVE('',#20743,#20742,#218,.T.) ;
#25563=EDGE_CURVE('',#20739,#20743,#3691,.T.) ;
#25564=EDGE_CURVE('',#20744,#20744,#17714,.T.) ;
#25565=EDGE_CURVE('',#20744,#20737,#17715,.T.) ;
#25566=EDGE_CURVE('',#20745,#20746,#1107,.T.) ;
#25567=EDGE_CURVE('',#20747,#20746,#3692,.T.) ;
#25568=EDGE_CURVE('',#20747,#20748,#1108,.T.) ;
#25569=EDGE_CURVE('',#20748,#20510,#3693,.T.) ;
#25570=EDGE_CURVE('',#20509,#20745,#3694,.T.) ;
#25571=EDGE_CURVE('',#20701,#20749,#17716,.T.) ;
#25572=EDGE_CURVE('',#20749,#20750,#17717,.T.) ;
#25573=EDGE_CURVE('',#20750,#20700,#17718,.T.) ;
#25574=EDGE_CURVE('',#20751,#20699,#17719,.T.) ;
#25575=EDGE_CURVE('',#20750,#20751,#3695,.T.) ;
#25576=EDGE_CURVE('',#20752,#20698,#17720,.T.) ;
#25577=EDGE_CURVE('',#20751,#20752,#17721,.T.) ;
#25578=EDGE_CURVE('',#20753,#20697,#17722,.T.) ;
#25579=EDGE_CURVE('',#20752,#20753,#3696,.T.) ;
#25580=EDGE_CURVE('',#20754,#20696,#17723,.T.) ;
#25581=EDGE_CURVE('',#20753,#20754,#17724,.T.) ;
#25582=EDGE_CURVE('',#20755,#20749,#3697,.T.) ;
#25583=EDGE_CURVE('',#20756,#20755,#17725,.T.) ;
#25584=EDGE_CURVE('',#20757,#20756,#3698,.T.) ;
#25585=EDGE_CURVE('',#20758,#20757,#3699,.T.) ;
#25586=EDGE_CURVE('',#20759,#20758,#3700,.T.) ;
#25587=EDGE_CURVE('',#20742,#20759,#1109,.T.) ;
#25588=EDGE_CURVE('',#20760,#20741,#1110,.T.) ;
#25589=EDGE_CURVE('',#20761,#20760,#3701,.T.) ;
#25590=EDGE_CURVE('',#20762,#20761,#3702,.T.) ;
#25591=EDGE_CURVE('',#20763,#20762,#3703,.T.) ;
#25592=EDGE_CURVE('',#20726,#20763,#1111,.T.) ;
#25593=EDGE_CURVE('',#20764,#20725,#1112,.T.) ;
#25594=EDGE_CURVE('',#20765,#20764,#3704,.T.) ;
#25595=EDGE_CURVE('',#20766,#20765,#3705,.T.) ;
#25596=EDGE_CURVE('',#20767,#20766,#3706,.T.) ;
#25597=EDGE_CURVE('',#20768,#20767,#17726,.T.) ;
#25598=EDGE_CURVE('',#20754,#20768,#3707,.T.) ;
#25599=EDGE_CURVE('',#20755,#20702,#17727,.T.) ;
#25600=EDGE_CURVE('',#20769,#20688,#3708,.T.) ;
#25601=EDGE_CURVE('',#20770,#20769,#219,.T.) ;
#25602=EDGE_CURVE('',#20770,#20729,#1113,.T.) ;
#25603=EDGE_CURVE('',#20732,#20771,#1114,.T.) ;
#25604=EDGE_CURVE('',#20772,#20771,#220,.T.) ;
#25605=EDGE_CURVE('',#20513,#20772,#3709,.T.) ;
#25606=EDGE_CURVE('',#20512,#20773,#3710,.T.) ;
#25607=EDGE_CURVE('',#20774,#20773,#221,.T.) ;
#25608=EDGE_CURVE('',#20774,#20747,#1115,.T.) ;
#25609=EDGE_CURVE('',#20746,#20775,#1116,.T.) ;
#25610=EDGE_CURVE('',#20776,#20775,#222,.T.) ;
#25611=EDGE_CURVE('',#20777,#20776,#3711,.T.) ;
#25612=EDGE_CURVE('',#20778,#20777,#223,.T.) ;
#25613=EDGE_CURVE('',#20779,#20778,#1117,.T.) ;
#25614=EDGE_CURVE('',#20780,#20779,#3712,.T.) ;
#25615=EDGE_CURVE('',#20781,#20780,#1118,.T.) ;
#25616=EDGE_CURVE('',#20665,#20781,#3713,.T.) ;
#25617=EDGE_CURVE('',#20768,#20695,#17728,.T.) ;
#25618=EDGE_CURVE('',#20508,#20776,#1119,.T.) ;
#25619=EDGE_CURVE('',#20507,#20777,#17729,.T.) ;
#25620=EDGE_CURVE('',#20782,#20778,#17730,.T.) ;
#25621=EDGE_CURVE('',#20507,#20782,#224,.T.) ;
#25622=EDGE_CURVE('',#20783,#20779,#17731,.T.) ;
#25623=EDGE_CURVE('',#20782,#20783,#1120,.T.) ;
#25624=EDGE_CURVE('',#20784,#20780,#17732,.T.) ;
#25625=EDGE_CURVE('',#20783,#20784,#3714,.T.) ;
#25626=EDGE_CURVE('',#20494,#20781,#17733,.T.) ;
#25627=EDGE_CURVE('',#20784,#20494,#1121,.T.) ;
#25628=EDGE_CURVE('',#20550,#20704,#17734,.T.) ;
#25629=EDGE_CURVE('',#20785,#20784,#17735,.T.) ;
#25630=EDGE_CURVE('',#20785,#20786,#17736,.T.) ;
#25631=EDGE_CURVE('',#20786,#20496,#17737,.T.) ;
#25632=EDGE_CURVE('',#20787,#20783,#17738,.T.) ;
#25633=EDGE_CURVE('',#20787,#20785,#3715,.T.) ;
#25634=EDGE_CURVE('',#20788,#20782,#17739,.T.) ;
#25635=EDGE_CURVE('',#20788,#20787,#17740,.T.) ;
#25636=EDGE_CURVE('',#20789,#20506,#17741,.T.) ;
#25637=EDGE_CURVE('',#20789,#20788,#3716,.T.) ;
#25638=EDGE_CURVE('',#20769,#20517,#1122,.T.) ;
#25639=EDGE_CURVE('',#20770,#20730,#1123,.T.) ;
#25640=EDGE_CURVE('',#20399,#20790,#17742,.F.) ;
#25641=EDGE_CURVE('',#20791,#20399,#17743,.F.) ;
#25642=EDGE_CURVE('',#20790,#20791,#17744,.F.) ;
#25643=EDGE_CURVE('',#20397,#20792,#17745,.T.) ;
#25644=EDGE_CURVE('',#20792,#20791,#3717,.T.) ;
#25645=EDGE_CURVE('',#20398,#20793,#17746,.T.) ;
#25646=EDGE_CURVE('',#20792,#20793,#17747,.T.) ;
#25647=EDGE_CURVE('',#20794,#20795,#17748,.T.) ;
#25648=EDGE_CURVE('',#20795,#20624,#17749,.T.) ;
#25649=EDGE_CURVE('',#20624,#20794,#17750,.T.) ;
#25650=EDGE_CURVE('',#20794,#20790,#3718,.T.) ;
#25651=EDGE_CURVE('',#20791,#20795,#3719,.T.) ;
#25652=EDGE_CURVE('',#20796,#20402,#17751,.T.) ;
#25653=EDGE_CURVE('',#20797,#20796,#17752,.F.) ;
#25654=EDGE_CURVE('',#20403,#20797,#17753,.T.) ;
#25655=EDGE_CURVE('',#20798,#20799,#17754,.F.) ;
#25656=EDGE_CURVE('',#20401,#20798,#17755,.T.) ;
#25657=EDGE_CURVE('',#20799,#20400,#17756,.T.) ;
#25658=EDGE_CURVE('',#20798,#20796,#3720,.T.) ;
#25659=EDGE_CURVE('',#20790,#20799,#3721,.T.) ;
#25660=EDGE_CURVE('',#20800,#20801,#17757,.T.) ;
#25661=EDGE_CURVE('',#20801,#20623,#17758,.T.) ;
#25662=EDGE_CURVE('',#20622,#20800,#17759,.T.) ;
#25663=EDGE_CURVE('',#20799,#20801,#3722,.T.) ;
#25664=EDGE_CURVE('',#20800,#20798,#3723,.T.) ;
#25665=EDGE_CURVE('',#20802,#20803,#17760,.T.) ;
#25666=EDGE_CURVE('',#20803,#20797,#3724,.T.) ;
#25667=EDGE_CURVE('',#20796,#20802,#3725,.T.) ;
#25668=EDGE_CURVE('',#20634,#20803,#17761,.T.) ;
#25669=EDGE_CURVE('',#20802,#20621,#17762,.T.) ;
#25670=EDGE_CURVE('',#20804,#20404,#17763,.T.) ;
#25671=EDGE_CURVE('',#20797,#20804,#3726,.T.) ;
#25672=EDGE_CURVE('',#20804,#20805,#17764,.T.) ;
#25673=EDGE_CURVE('',#20805,#20404,#17765,.T.) ;
#25674=EDGE_CURVE('',#20795,#20806,#3727,.T.) ;
#25675=EDGE_CURVE('',#20806,#20625,#17766,.T.) ;
#25676=EDGE_CURVE('',#20806,#20792,#3728,.T.) ;
#25677=EDGE_CURVE('',#20805,#20807,#3729,.T.) ;
#25678=EDGE_CURVE('',#20807,#20405,#17767,.T.) ;
#25679=EDGE_CURVE('',#20804,#20808,#3730,.T.) ;
#25680=EDGE_CURVE('',#20809,#20808,#17768,.T.) ;
#25681=EDGE_CURVE('',#20809,#20805,#3731,.T.) ;
#25682=EDGE_CURVE('',#20808,#20803,#3732,.T.) ;
#25683=EDGE_CURVE('',#20810,#20811,#17769,.T.) ;
#25684=EDGE_CURVE('',#20811,#20611,#17770,.T.) ;
#25685=EDGE_CURVE('',#20610,#20810,#17771,.T.) ;
#25686=EDGE_CURVE('',#20812,#20813,#17772,.T.) ;
#25687=EDGE_CURVE('',#20813,#20811,#3733,.T.) ;
#25688=EDGE_CURVE('',#20810,#20812,#3734,.T.) ;
#25689=EDGE_CURVE('',#20812,#20454,#225,.T.) ;
#25690=EDGE_CURVE('',#20454,#20813,#226,.T.) ;
#25691=EDGE_CURVE('',#20812,#20814,#3735,.T.) ;
#25692=EDGE_CURVE('',#20455,#20814,#227,.F.) ;
#25693=EDGE_CURVE('',#20609,#20814,#3736,.T.) ;
#25694=EDGE_CURVE('',#20815,#20816,#17773,.T.) ;
#25695=EDGE_CURVE('',#20816,#20445,#228,.T.) ;
#25696=EDGE_CURVE('',#20445,#20815,#229,.T.) ;
#25697=EDGE_CURVE('',#20817,#20818,#17774,.T.) ;
#25698=EDGE_CURVE('',#20818,#20816,#3737,.T.) ;
#25699=EDGE_CURVE('',#20815,#20817,#3738,.T.) ;
#25700=EDGE_CURVE('',#20620,#20818,#17775,.T.) ;
#25701=EDGE_CURVE('',#20817,#20607,#17776,.T.) ;
#25702=EDGE_CURVE('',#20819,#20815,#3739,.T.) ;
#25703=EDGE_CURVE('',#20819,#20608,#3740,.T.) ;
#25704=EDGE_CURVE('',#20443,#20819,#230,.T.) ;
#25705=EDGE_CURVE('',#20820,#20501,#17777,.T.) ;
#25706=EDGE_CURVE('',#20500,#20821,#17778,.F.) ;
#25707=EDGE_CURVE('',#20821,#20820,#3741,.T.) ;
#25708=EDGE_CURVE('',#20822,#20502,#17779,.T.) ;
#25709=EDGE_CURVE('',#20820,#20822,#17780,.T.) ;
#25710=EDGE_CURVE('',#20823,#20503,#17781,.T.) ;
#25711=EDGE_CURVE('',#20822,#20823,#3742,.T.) ;
#25712=EDGE_CURVE('',#20824,#20504,#17782,.T.) ;
#25713=EDGE_CURVE('',#20823,#20824,#17783,.T.) ;
#25714=EDGE_CURVE('',#20825,#20505,#17784,.T.) ;
#25715=EDGE_CURVE('',#20824,#20825,#3743,.T.) ;
#25716=EDGE_CURVE('',#20825,#20789,#17785,.T.) ;
#25717=EDGE_CURVE('',#20497,#20826,#17786,.T.) ;
#25718=EDGE_CURVE('',#20786,#20826,#3744,.T.) ;
#25719=EDGE_CURVE('',#20827,#20786,#3745,.T.) ;
#25720=EDGE_CURVE('',#20828,#20827,#3746,.T.) ;
#25721=EDGE_CURVE('',#20828,#20826,#3747,.T.) ;
#25722=EDGE_CURVE('',#20785,#20829,#3748,.T.) ;
#25723=EDGE_CURVE('',#20829,#20827,#17787,.F.) ;
#25724=EDGE_CURVE('',#20830,#20787,#3749,.T.) ;
#25725=EDGE_CURVE('',#20829,#20830,#3750,.T.) ;
#25726=EDGE_CURVE('',#20788,#20831,#3751,.T.) ;
#25727=EDGE_CURVE('',#20831,#20830,#17788,.F.) ;
#25728=EDGE_CURVE('',#20832,#20789,#3752,.T.) ;
#25729=EDGE_CURVE('',#20831,#20832,#3753,.T.) ;
#25730=EDGE_CURVE('',#20825,#20833,#3754,.T.) ;
#25731=EDGE_CURVE('',#20833,#20832,#17789,.F.) ;
#25732=EDGE_CURVE('',#20834,#20824,#3755,.T.) ;
#25733=EDGE_CURVE('',#20833,#20834,#3756,.T.) ;
#25734=EDGE_CURVE('',#20823,#20835,#3757,.T.) ;
#25735=EDGE_CURVE('',#20835,#20834,#17790,.F.) ;
#25736=EDGE_CURVE('',#20836,#20822,#3758,.T.) ;
#25737=EDGE_CURVE('',#20835,#20836,#3759,.T.) ;
#25738=EDGE_CURVE('',#20820,#20837,#3760,.T.) ;
#25739=EDGE_CURVE('',#20837,#20836,#17791,.F.) ;
#25740=EDGE_CURVE('',#20821,#20838,#3761,.T.) ;
#25741=EDGE_CURVE('',#20837,#20838,#3762,.T.) ;
#25742=EDGE_CURVE('',#20553,#20839,#17792,.T.) ;
#25743=EDGE_CURVE('',#20839,#20840,#3763,.T.) ;
#25744=EDGE_CURVE('',#20840,#20552,#17793,.T.) ;
#25745=EDGE_CURVE('',#20565,#20841,#17794,.T.) ;
#25746=EDGE_CURVE('',#20841,#20839,#17795,.T.) ;
#25747=EDGE_CURVE('',#20564,#20842,#17796,.T.) ;
#25748=EDGE_CURVE('',#20842,#20841,#3764,.T.) ;
#25749=EDGE_CURVE('',#20563,#20843,#17797,.T.) ;
#25750=EDGE_CURVE('',#20843,#20842,#17798,.T.) ;
#25751=EDGE_CURVE('',#20562,#20844,#17799,.T.) ;
#25752=EDGE_CURVE('',#20844,#20843,#3765,.T.) ;
#25753=EDGE_CURVE('',#20561,#20845,#17800,.T.) ;
#25754=EDGE_CURVE('',#20845,#20844,#17801,.T.) ;
#25755=EDGE_CURVE('',#20560,#20846,#17802,.T.) ;
#25756=EDGE_CURVE('',#20846,#20845,#3766,.T.) ;
#25757=EDGE_CURVE('',#20559,#20847,#17803,.T.) ;
#25758=EDGE_CURVE('',#20847,#20846,#17804,.T.) ;
#25759=EDGE_CURVE('',#20558,#20848,#17805,.T.) ;
#25760=EDGE_CURVE('',#20848,#20847,#3767,.T.) ;
#25761=EDGE_CURVE('',#20557,#20849,#17806,.T.) ;
#25762=EDGE_CURVE('',#20849,#20850,#3768,.T.) ;
#25763=EDGE_CURVE('',#20850,#20558,#17807,.T.) ;
#25764=EDGE_CURVE('',#20556,#20851,#17808,.T.) ;
#25765=EDGE_CURVE('',#20851,#20849,#17809,.T.) ;
#25766=EDGE_CURVE('',#20555,#20852,#17810,.T.) ;
#25767=EDGE_CURVE('',#20852,#20851,#3769,.T.) ;
#25768=EDGE_CURVE('',#20554,#20853,#17811,.T.) ;
#25769=EDGE_CURVE('',#20853,#20852,#17812,.T.) ;
#25770=EDGE_CURVE('',#20552,#20854,#17813,.T.) ;
#25771=EDGE_CURVE('',#20854,#20853,#3770,.T.) ;
#25772=EDGE_CURVE('',#20850,#20848,#17814,.T.) ;
#25773=EDGE_CURVE('',#20840,#20854,#17815,.T.) ;
#25774=EDGE_CURVE('',#20843,#20855,#3771,.T.) ;
#25775=EDGE_CURVE('',#20855,#20856,#17816,.F.) ;
#25776=EDGE_CURVE('',#20856,#20842,#3772,.T.) ;
#25777=EDGE_CURVE('',#20857,#20844,#3773,.T.) ;
#25778=EDGE_CURVE('',#20855,#20857,#3774,.T.) ;
#25779=EDGE_CURVE('',#20845,#20858,#3775,.T.) ;
#25780=EDGE_CURVE('',#20858,#20857,#17817,.F.) ;
#25781=EDGE_CURVE('',#20859,#20846,#3776,.T.) ;
#25782=EDGE_CURVE('',#20858,#20859,#3777,.T.) ;
#25783=EDGE_CURVE('',#20847,#20860,#3778,.T.) ;
#25784=EDGE_CURVE('',#20860,#20859,#17818,.F.) ;
#25785=EDGE_CURVE('',#20861,#20848,#3779,.T.) ;
#25786=EDGE_CURVE('',#20860,#20861,#3780,.T.) ;
#25787=EDGE_CURVE('',#20850,#20862,#3781,.T.) ;
#25788=EDGE_CURVE('',#20862,#20861,#17819,.F.) ;
#25789=EDGE_CURVE('',#20863,#20849,#3782,.T.) ;
#25790=EDGE_CURVE('',#20862,#20863,#3783,.T.) ;
#25791=EDGE_CURVE('',#20864,#20580,#17820,.T.) ;
#25792=EDGE_CURVE('',#20865,#20864,#17821,.F.) ;
#25793=EDGE_CURVE('',#20581,#20865,#17822,.T.) ;
#25794=EDGE_CURVE('',#20866,#20867,#17823,.F.) ;
#25795=EDGE_CURVE('',#20571,#20866,#17824,.T.) ;
#25796=EDGE_CURVE('',#20867,#20570,#17825,.T.) ;
#25797=EDGE_CURVE('',#20868,#20572,#17826,.T.) ;
#25798=EDGE_CURVE('',#20866,#20868,#3784,.T.) ;
#25799=EDGE_CURVE('',#20869,#20573,#17827,.T.) ;
#25800=EDGE_CURVE('',#20868,#20869,#17828,.T.) ;
#25801=EDGE_CURVE('',#20870,#20574,#17829,.T.) ;
#25802=EDGE_CURVE('',#20869,#20870,#3785,.T.) ;
#25803=EDGE_CURVE('',#20871,#20575,#17830,.T.) ;
#25804=EDGE_CURVE('',#20870,#20871,#17831,.T.) ;
#25805=EDGE_CURVE('',#20872,#20576,#17832,.T.) ;
#25806=EDGE_CURVE('',#20871,#20872,#3786,.T.) ;
#25807=EDGE_CURVE('',#20873,#20577,#17833,.T.) ;
#25808=EDGE_CURVE('',#20872,#20873,#17834,.T.) ;
#25809=EDGE_CURVE('',#20874,#20578,#17835,.T.) ;
#25810=EDGE_CURVE('',#20873,#20874,#3787,.T.) ;
#25811=EDGE_CURVE('',#20875,#20579,#17836,.T.) ;
#25812=EDGE_CURVE('',#20874,#20875,#17837,.T.) ;
#25813=EDGE_CURVE('',#20875,#20864,#3788,.T.) ;
#25814=EDGE_CURVE('',#20568,#20876,#17838,.F.) ;
#25815=EDGE_CURVE('',#20876,#20867,#3789,.T.) ;
#25816=EDGE_CURVE('',#20877,#20878,#17839,.T.) ;
#25817=EDGE_CURVE('',#20878,#20866,#3790,.T.) ;
#25818=EDGE_CURVE('',#20867,#20877,#3791,.T.) ;
#25819=EDGE_CURVE('',#20877,#20411,#231,.T.) ;
#25820=EDGE_CURVE('',#20411,#20878,#232,.T.) ;
#25821=EDGE_CURVE('',#20879,#20880,#17840,.T.) ;
#25822=EDGE_CURVE('',#20880,#20865,#3792,.T.) ;
#25823=EDGE_CURVE('',#20864,#20879,#3793,.T.) ;
#25824=EDGE_CURVE('',#20879,#20416,#233,.T.) ;
#25825=EDGE_CURVE('',#20416,#20880,#234,.T.) ;
#25826=EDGE_CURVE('',#20582,#20881,#17841,.T.) ;
#25827=EDGE_CURVE('',#20865,#20881,#3794,.T.) ;
#25828=EDGE_CURVE('',#20876,#20882,#3795,.T.) ;
#25829=EDGE_CURVE('',#20877,#20882,#3796,.T.) ;
#25830=EDGE_CURVE('',#20650,#20883,#17842,.T.) ;
#25831=EDGE_CURVE('',#20883,#20884,#17843,.T.) ;
#25832=EDGE_CURVE('',#20884,#20649,#17844,.T.) ;
#25833=EDGE_CURVE('',#20662,#20885,#17845,.T.) ;
#25834=EDGE_CURVE('',#20885,#20883,#3797,.T.) ;
#25835=EDGE_CURVE('',#20661,#20886,#17846,.T.) ;
#25836=EDGE_CURVE('',#20886,#20887,#3798,.T.) ;
#25837=EDGE_CURVE('',#20887,#20662,#17847,.T.) ;
#25838=EDGE_CURVE('',#20660,#20888,#17848,.T.) ;
#25839=EDGE_CURVE('',#20888,#20886,#17849,.T.) ;
#25840=EDGE_CURVE('',#20659,#20889,#17850,.T.) ;
#25841=EDGE_CURVE('',#20889,#20888,#3799,.T.) ;
#25842=EDGE_CURVE('',#20658,#20890,#17851,.T.) ;
#25843=EDGE_CURVE('',#20890,#20889,#17852,.T.) ;
#25844=EDGE_CURVE('',#20657,#20891,#17853,.T.) ;
#25845=EDGE_CURVE('',#20891,#20890,#3800,.T.) ;
#25846=EDGE_CURVE('',#20887,#20885,#17854,.T.) ;
#25847=EDGE_CURVE('',#20656,#20892,#17855,.T.) ;
#25848=EDGE_CURVE('',#20892,#20893,#3801,.T.) ;
#25849=EDGE_CURVE('',#20893,#20657,#17856,.T.) ;
#25850=EDGE_CURVE('',#20655,#20894,#17857,.T.) ;
#25851=EDGE_CURVE('',#20892,#20894,#17858,.T.) ;
#25852=EDGE_CURVE('',#20893,#20891,#17859,.T.) ;
#25853=EDGE_CURVE('',#20895,#20885,#3802,.T.) ;
#25854=EDGE_CURVE('',#20896,#20895,#3803,.T.) ;
#25855=EDGE_CURVE('',#20883,#20896,#3804,.T.) ;
#25856=EDGE_CURVE('',#20887,#20897,#3805,.T.) ;
#25857=EDGE_CURVE('',#20897,#20895,#17860,.F.) ;
#25858=EDGE_CURVE('',#20898,#20886,#3806,.T.) ;
#25859=EDGE_CURVE('',#20897,#20898,#3807,.T.) ;
#25860=EDGE_CURVE('',#20888,#20899,#3808,.T.) ;
#25861=EDGE_CURVE('',#20899,#20898,#17861,.F.) ;
#25862=EDGE_CURVE('',#20900,#20889,#3809,.T.) ;
#25863=EDGE_CURVE('',#20899,#20900,#3810,.T.) ;
#25864=EDGE_CURVE('',#20890,#20901,#3811,.T.) ;
#25865=EDGE_CURVE('',#20901,#20900,#17862,.F.) ;
#25866=EDGE_CURVE('',#20902,#20891,#3812,.T.) ;
#25867=EDGE_CURVE('',#20901,#20902,#3813,.T.) ;
#25868=EDGE_CURVE('',#20893,#20903,#3814,.T.) ;
#25869=EDGE_CURVE('',#20903,#20902,#17863,.F.) ;
#25870=EDGE_CURVE('',#20904,#20892,#3815,.T.) ;
#25871=EDGE_CURVE('',#20903,#20904,#3816,.T.) ;
#25872=EDGE_CURVE('',#20636,#20905,#17864,.T.) ;
#25873=EDGE_CURVE('',#20905,#20906,#17865,.T.) ;
#25874=EDGE_CURVE('',#20906,#20635,#17866,.T.) ;
#25875=EDGE_CURVE('',#20648,#20907,#17867,.T.) ;
#25876=EDGE_CURVE('',#20907,#20905,#3817,.T.) ;
#25877=EDGE_CURVE('',#20647,#20908,#17868,.T.) ;
#25878=EDGE_CURVE('',#20908,#20909,#3818,.T.) ;
#25879=EDGE_CURVE('',#20909,#20648,#17869,.T.) ;
#25880=EDGE_CURVE('',#20646,#20910,#17870,.T.) ;
#25881=EDGE_CURVE('',#20910,#20908,#17871,.T.) ;
#25882=EDGE_CURVE('',#20645,#20911,#17872,.T.) ;
#25883=EDGE_CURVE('',#20911,#20910,#3819,.T.) ;
#25884=EDGE_CURVE('',#20644,#20912,#17873,.T.) ;
#25885=EDGE_CURVE('',#20912,#20911,#17874,.T.) ;
#25886=EDGE_CURVE('',#20643,#20913,#17875,.T.) ;
#25887=EDGE_CURVE('',#20913,#20912,#3820,.T.) ;
#25888=EDGE_CURVE('',#20909,#20907,#17876,.T.) ;
#25889=EDGE_CURVE('',#20642,#20914,#17877,.T.) ;
#25890=EDGE_CURVE('',#20914,#20915,#3821,.T.) ;
#25891=EDGE_CURVE('',#20915,#20643,#17878,.T.) ;
#25892=EDGE_CURVE('',#20641,#20916,#17879,.T.) ;
#25893=EDGE_CURVE('',#20914,#20916,#17880,.T.) ;
#25894=EDGE_CURVE('',#20915,#20913,#17881,.T.) ;
#25895=EDGE_CURVE('',#20917,#20907,#3822,.T.) ;
#25896=EDGE_CURVE('',#20918,#20917,#3823,.T.) ;
#25897=EDGE_CURVE('',#20905,#20918,#3824,.T.) ;
#25898=EDGE_CURVE('',#20909,#20919,#3825,.T.) ;
#25899=EDGE_CURVE('',#20919,#20917,#17882,.F.) ;
#25900=EDGE_CURVE('',#20920,#20908,#3826,.T.) ;
#25901=EDGE_CURVE('',#20919,#20920,#3827,.T.) ;
#25902=EDGE_CURVE('',#20910,#20921,#3828,.T.) ;
#25903=EDGE_CURVE('',#20921,#20920,#17883,.F.) ;
#25904=EDGE_CURVE('',#20922,#20911,#3829,.T.) ;
#25905=EDGE_CURVE('',#20921,#20922,#3830,.T.) ;
#25906=EDGE_CURVE('',#20912,#20923,#3831,.T.) ;
#25907=EDGE_CURVE('',#20923,#20922,#17884,.F.) ;
#25908=EDGE_CURVE('',#20924,#20913,#3832,.T.) ;
#25909=EDGE_CURVE('',#20923,#20924,#3833,.T.) ;
#25910=EDGE_CURVE('',#20915,#20925,#3834,.T.) ;
#25911=EDGE_CURVE('',#20925,#20924,#17885,.F.) ;
#25912=EDGE_CURVE('',#20926,#20914,#3835,.T.) ;
#25913=EDGE_CURVE('',#20925,#20926,#3836,.T.) ;
#25914=EDGE_CURVE('',#20633,#20808,#17886,.T.) ;
#25915=EDGE_CURVE('',#20632,#20927,#17887,.T.) ;
#25916=EDGE_CURVE('',#20927,#20809,#3837,.T.) ;
#25917=EDGE_CURVE('',#20809,#20633,#17888,.T.) ;
#25918=EDGE_CURVE('',#20631,#20928,#17889,.T.) ;
#25919=EDGE_CURVE('',#20927,#20928,#17890,.T.) ;
#25920=EDGE_CURVE('',#20807,#20927,#3838,.T.) ;
#25921=EDGE_CURVE('',#20801,#20794,#3839,.T.) ;
#25922=EDGE_CURVE('',#20806,#20929,#17891,.T.) ;
#25923=EDGE_CURVE('',#20929,#20626,#17892,.T.) ;
#25924=EDGE_CURVE('',#20811,#20930,#3840,.T.) ;
#25925=EDGE_CURVE('',#20930,#20612,#17893,.T.) ;
#25926=EDGE_CURVE('',#20931,#20613,#17894,.T.) ;
#25927=EDGE_CURVE('',#20930,#20931,#17895,.T.) ;
#25928=EDGE_CURVE('',#20932,#20614,#17896,.T.) ;
#25929=EDGE_CURVE('',#20931,#20932,#3841,.T.) ;
#25930=EDGE_CURVE('',#20933,#20615,#17897,.T.) ;
#25931=EDGE_CURVE('',#20932,#20933,#17898,.T.) ;
#25932=EDGE_CURVE('',#20934,#20616,#17899,.T.) ;
#25933=EDGE_CURVE('',#20933,#20934,#3842,.T.) ;
#25934=EDGE_CURVE('',#20935,#20617,#17900,.T.) ;
#25935=EDGE_CURVE('',#20934,#20935,#17901,.T.) ;
#25936=EDGE_CURVE('',#20936,#20618,#17902,.T.) ;
#25937=EDGE_CURVE('',#20935,#20936,#3843,.T.) ;
#25938=EDGE_CURVE('',#20937,#20619,#17903,.T.) ;
#25939=EDGE_CURVE('',#20936,#20937,#17904,.T.) ;
#25940=EDGE_CURVE('',#20937,#20818,#3844,.T.) ;
#25941=EDGE_CURVE('',#20938,#20937,#3845,.T.) ;
#25942=EDGE_CURVE('',#20816,#20938,#3846,.T.) ;
#25943=EDGE_CURVE('',#20936,#20939,#3847,.T.) ;
#25944=EDGE_CURVE('',#20939,#20938,#17905,.F.) ;
#25945=EDGE_CURVE('',#20940,#20935,#3848,.T.) ;
#25946=EDGE_CURVE('',#20939,#20940,#3849,.T.) ;
#25947=EDGE_CURVE('',#20934,#20941,#3850,.T.) ;
#25948=EDGE_CURVE('',#20941,#20940,#17906,.F.) ;
#25949=EDGE_CURVE('',#20942,#20933,#3851,.T.) ;
#25950=EDGE_CURVE('',#20941,#20942,#3852,.T.) ;
#25951=EDGE_CURVE('',#20932,#20943,#3853,.T.) ;
#25952=EDGE_CURVE('',#20943,#20942,#17907,.F.) ;
#25953=EDGE_CURVE('',#20944,#20931,#3854,.T.) ;
#25954=EDGE_CURVE('',#20943,#20944,#3855,.T.) ;
#25955=EDGE_CURVE('',#20930,#20945,#3856,.T.) ;
#25956=EDGE_CURVE('',#20945,#20944,#17908,.F.) ;
#25957=EDGE_CURVE('',#20945,#20813,#3857,.T.) ;
#25958=EDGE_CURVE('',#20793,#20929,#3858,.T.) ;
#25959=EDGE_CURVE('',#20946,#20629,#17909,.T.) ;
#25960=EDGE_CURVE('',#20946,#20947,#17910,.T.) ;
#25961=EDGE_CURVE('',#20947,#20630,#17911,.T.) ;
#25962=EDGE_CURVE('',#20948,#20946,#3859,.T.) ;
#25963=EDGE_CURVE('',#20949,#20948,#3860,.T.) ;
#25964=EDGE_CURVE('',#20950,#20949,#3861,.T.) ;
#25965=EDGE_CURVE('',#20946,#20950,#3862,.T.) ;
#25966=EDGE_CURVE('',#20951,#20807,#17912,.F.) ;
#25967=EDGE_CURVE('',#20406,#20951,#17913,.T.) ;
#25968=EDGE_CURVE('',#20928,#20951,#3863,.T.) ;
#25969=EDGE_CURVE('',#20949,#20409,#17914,.T.) ;
#25970=EDGE_CURVE('',#20952,#20949,#17915,.F.) ;
#25971=EDGE_CURVE('',#20410,#20952,#17916,.T.) ;
#25972=EDGE_CURVE('',#20953,#20407,#17917,.T.) ;
#25973=EDGE_CURVE('',#20950,#20953,#17918,.F.) ;
#25974=EDGE_CURVE('',#20408,#20950,#17919,.T.) ;
#25975=EDGE_CURVE('',#20951,#20953,#3864,.T.) ;
#25976=EDGE_CURVE('',#20953,#20947,#3865,.T.) ;
#25977=EDGE_CURVE('',#20948,#20954,#17920,.F.) ;
#25978=EDGE_CURVE('',#20628,#20948,#17921,.T.) ;
#25979=EDGE_CURVE('',#20954,#20627,#17922,.T.) ;
#25980=EDGE_CURVE('',#20929,#20954,#3866,.T.) ;
#25981=EDGE_CURVE('',#20954,#20952,#3867,.T.) ;
#25982=EDGE_CURVE('',#20952,#20793,#3868,.T.) ;
#25983=EDGE_CURVE('',#20947,#20928,#3869,.T.) ;
#25984=EDGE_CURVE('',#20955,#20652,#17923,.T.) ;
#25985=EDGE_CURVE('',#20651,#20956,#17924,.T.) ;
#25986=EDGE_CURVE('',#20955,#20956,#17925,.T.) ;
#25987=EDGE_CURVE('',#20957,#20653,#17926,.T.) ;
#25988=EDGE_CURVE('',#20957,#20958,#17927,.T.) ;
#25989=EDGE_CURVE('',#20958,#20654,#17928,.T.) ;
#25990=EDGE_CURVE('',#20955,#20957,#3870,.T.) ;
#25991=EDGE_CURVE('',#20959,#20955,#3871,.T.) ;
#25992=EDGE_CURVE('',#20960,#20959,#3872,.T.) ;
#25993=EDGE_CURVE('',#20957,#20960,#3873,.T.) ;
#25994=EDGE_CURVE('',#20361,#20899,#17929,.T.) ;
#25995=EDGE_CURVE('',#20898,#20360,#17930,.T.) ;
#25996=EDGE_CURVE('',#20900,#20362,#17931,.T.) ;
#25997=EDGE_CURVE('',#20363,#20901,#17932,.T.) ;
#25998=EDGE_CURVE('',#20359,#20897,#17933,.F.) ;
#25999=EDGE_CURVE('',#20895,#20359,#17934,.F.) ;
#26000=EDGE_CURVE('',#20364,#20903,#17935,.F.) ;
#26001=EDGE_CURVE('',#20902,#20364,#17936,.F.) ;
#26002=EDGE_CURVE('',#20961,#20357,#17937,.T.) ;
#26003=EDGE_CURVE('',#20896,#20961,#17938,.F.) ;
#26004=EDGE_CURVE('',#20358,#20896,#17939,.T.) ;
#26005=EDGE_CURVE('',#20904,#20365,#17940,.T.) ;
#26006=EDGE_CURVE('',#20962,#20904,#17941,.F.) ;
#26007=EDGE_CURVE('',#20366,#20962,#17942,.T.) ;
#26008=EDGE_CURVE('',#20894,#20962,#3874,.T.) ;
#26009=EDGE_CURVE('',#20959,#20355,#17943,.T.) ;
#26010=EDGE_CURVE('',#20963,#20959,#17944,.F.) ;
#26011=EDGE_CURVE('',#20356,#20963,#17945,.T.) ;
#26012=EDGE_CURVE('',#20964,#20354,#17946,.T.) ;
#26013=EDGE_CURVE('',#20960,#20964,#17947,.F.) ;
#26014=EDGE_CURVE('',#20353,#20960,#17948,.T.) ;
#26015=EDGE_CURVE('',#20962,#20964,#3875,.T.) ;
#26016=EDGE_CURVE('',#20964,#20958,#3876,.T.) ;
#26017=EDGE_CURVE('',#20956,#20963,#3877,.T.) ;
#26018=EDGE_CURVE('',#20963,#20961,#3878,.T.) ;
#26019=EDGE_CURVE('',#20961,#20884,#3879,.T.) ;
#26020=EDGE_CURVE('',#20958,#20894,#3880,.T.) ;
#26021=EDGE_CURVE('',#20965,#20638,#17949,.T.) ;
#26022=EDGE_CURVE('',#20637,#20966,#17950,.T.) ;
#26023=EDGE_CURVE('',#20965,#20966,#17951,.T.) ;
#26024=EDGE_CURVE('',#20967,#20639,#17952,.T.) ;
#26025=EDGE_CURVE('',#20967,#20968,#17953,.T.) ;
#26026=EDGE_CURVE('',#20968,#20640,#17954,.T.) ;
#26027=EDGE_CURVE('',#20965,#20967,#3881,.T.) ;
#26028=EDGE_CURVE('',#20969,#20965,#3882,.T.) ;
#26029=EDGE_CURVE('',#20970,#20969,#3883,.T.) ;
#26030=EDGE_CURVE('',#20967,#20970,#3884,.T.) ;
#26031=EDGE_CURVE('',#20920,#20474,#17955,.T.) ;
#26032=EDGE_CURVE('',#20475,#20921,#17956,.T.) ;
#26033=EDGE_CURVE('',#20473,#20919,#17957,.F.) ;
#26034=EDGE_CURVE('',#20917,#20473,#17958,.F.) ;
#26035=EDGE_CURVE('',#20922,#20476,#17959,.T.) ;
#26036=EDGE_CURVE('',#20477,#20923,#17960,.T.) ;
#26037=EDGE_CURVE('',#20971,#20471,#17961,.T.) ;
#26038=EDGE_CURVE('',#20918,#20971,#17962,.F.) ;
#26039=EDGE_CURVE('',#20472,#20918,#17963,.T.) ;
#26040=EDGE_CURVE('',#20478,#20925,#17964,.F.) ;
#26041=EDGE_CURVE('',#20924,#20478,#17965,.F.) ;
#26042=EDGE_CURVE('',#20969,#20469,#17966,.T.) ;
#26043=EDGE_CURVE('',#20972,#20969,#17967,.F.) ;
#26044=EDGE_CURVE('',#20470,#20972,#17968,.T.) ;
#26045=EDGE_CURVE('',#20926,#20479,#17969,.T.) ;
#26046=EDGE_CURVE('',#20973,#20926,#17970,.F.) ;
#26047=EDGE_CURVE('',#20480,#20973,#17971,.T.) ;
#26048=EDGE_CURVE('',#20916,#20973,#3885,.T.) ;
#26049=EDGE_CURVE('',#20974,#20468,#17972,.T.) ;
#26050=EDGE_CURVE('',#20970,#20974,#17973,.F.) ;
#26051=EDGE_CURVE('',#20467,#20970,#17974,.T.) ;
#26052=EDGE_CURVE('',#20973,#20974,#3886,.T.) ;
#26053=EDGE_CURVE('',#20974,#20968,#3887,.T.) ;
#26054=EDGE_CURVE('',#20966,#20972,#3888,.T.) ;
#26055=EDGE_CURVE('',#20972,#20971,#3889,.T.) ;
#26056=EDGE_CURVE('',#20971,#20906,#3890,.T.) ;
#26057=EDGE_CURVE('',#20968,#20916,#3891,.T.) ;
#26058=EDGE_CURVE('',#20975,#20322,#17975,.T.) ;
#26059=EDGE_CURVE('',#20976,#20975,#17976,.F.) ;
#26060=EDGE_CURVE('',#20323,#20976,#17977,.T.) ;
#26061=EDGE_CURVE('',#20977,#20320,#17978,.T.) ;
#26062=EDGE_CURVE('',#20978,#20977,#17979,.F.) ;
#26063=EDGE_CURVE('',#20321,#20978,#17980,.T.) ;
#26064=EDGE_CURVE('',#20756,#20703,#17981,.T.) ;
#26065=EDGE_CURVE('',#20707,#20757,#17982,.T.) ;
#26066=EDGE_CURVE('',#20706,#20315,#17983,.T.) ;
#26067=EDGE_CURVE('',#20315,#20757,#17984,.T.) ;
#26068=EDGE_CURVE('',#20705,#20316,#17985,.T.) ;
#26069=EDGE_CURVE('',#20979,#20317,#17986,.T.) ;
#26070=EDGE_CURVE('',#20705,#20979,#17987,.T.) ;
#26071=EDGE_CURVE('',#20980,#20318,#17988,.T.) ;
#26072=EDGE_CURVE('',#20979,#20980,#3892,.T.) ;
#26073=EDGE_CURVE('',#20981,#20319,#17989,.T.) ;
#26074=EDGE_CURVE('',#20980,#20981,#17990,.T.) ;
#26075=EDGE_CURVE('',#20981,#20977,#3893,.T.) ;
#26076=EDGE_CURVE('',#20767,#20690,#17991,.T.) ;
#26077=EDGE_CURVE('',#20766,#20691,#17992,.T.) ;
#26078=EDGE_CURVE('',#20299,#20692,#17993,.T.) ;
#26079=EDGE_CURVE('',#20766,#20299,#17994,.T.) ;
#26080=EDGE_CURVE('',#20300,#20693,#17995,.T.) ;
#26081=EDGE_CURVE('',#20346,#20982,#17996,.T.) ;
#26082=EDGE_CURVE('',#20982,#20693,#17997,.T.) ;
#26083=EDGE_CURVE('',#20345,#20983,#17998,.T.) ;
#26084=EDGE_CURVE('',#20983,#20982,#3894,.T.) ;
#26085=EDGE_CURVE('',#20344,#20984,#17999,.T.) ;
#26086=EDGE_CURVE('',#20984,#20983,#18000,.T.) ;
#26087=EDGE_CURVE('',#20343,#20985,#18001,.T.) ;
#26088=EDGE_CURVE('',#20985,#20984,#3895,.T.) ;
#26089=EDGE_CURVE('',#20342,#20986,#18002,.T.) ;
#26090=EDGE_CURVE('',#20986,#20985,#18003,.T.) ;
#26091=EDGE_CURVE('',#20341,#20987,#18004,.T.) ;
#26092=EDGE_CURVE('',#20987,#20986,#18005,.T.) ;
#26093=EDGE_CURVE('',#20340,#20988,#18006,.T.) ;
#26094=EDGE_CURVE('',#20988,#20987,#3896,.T.) ;
#26095=EDGE_CURVE('',#20339,#20989,#18007,.T.) ;
#26096=EDGE_CURVE('',#20989,#20988,#18008,.T.) ;
#26097=EDGE_CURVE('',#20338,#20990,#18009,.T.) ;
#26098=EDGE_CURVE('',#20990,#20989,#18010,.T.) ;
#26099=EDGE_CURVE('',#20337,#20991,#18011,.T.) ;
#26100=EDGE_CURVE('',#20991,#20990,#3897,.T.) ;
#26101=EDGE_CURVE('',#20336,#20992,#18012,.T.) ;
#26102=EDGE_CURVE('',#20992,#20991,#18013,.T.) ;
#26103=EDGE_CURVE('',#20335,#20993,#18014,.T.) ;
#26104=EDGE_CURVE('',#20993,#20992,#3898,.T.) ;
#26105=EDGE_CURVE('',#20334,#20994,#18015,.T.) ;
#26106=EDGE_CURVE('',#20994,#20993,#18016,.T.) ;
#26107=EDGE_CURVE('',#20333,#20995,#18017,.T.) ;
#26108=EDGE_CURVE('',#20995,#20994,#3899,.T.) ;
#26109=EDGE_CURVE('',#20332,#20996,#18018,.T.) ;
#26110=EDGE_CURVE('',#20996,#20995,#18019,.T.) ;
#26111=EDGE_CURVE('',#20331,#20997,#18020,.T.) ;
#26112=EDGE_CURVE('',#20997,#20996,#3900,.T.) ;
#26113=EDGE_CURVE('',#20330,#20998,#18021,.T.) ;
#26114=EDGE_CURVE('',#20998,#20997,#18022,.T.) ;
#26115=EDGE_CURVE('',#20329,#20999,#18023,.T.) ;
#26116=EDGE_CURVE('',#20999,#20998,#3901,.T.) ;
#26117=EDGE_CURVE('',#20328,#21000,#18024,.T.) ;
#26118=EDGE_CURVE('',#21000,#20999,#18025,.T.) ;
#26119=EDGE_CURVE('',#20327,#21001,#18026,.T.) ;
#26120=EDGE_CURVE('',#21001,#21000,#3902,.T.) ;
#26121=EDGE_CURVE('',#20326,#21002,#18027,.T.) ;
#26122=EDGE_CURVE('',#21002,#21001,#18028,.T.) ;
#26123=EDGE_CURVE('',#20325,#21003,#18029,.T.) ;
#26124=EDGE_CURVE('',#21003,#21002,#3903,.T.) ;
#26125=EDGE_CURVE('',#20324,#21004,#18030,.T.) ;
#26126=EDGE_CURVE('',#21004,#21003,#18031,.T.) ;
#26127=EDGE_CURVE('',#20976,#21004,#3904,.T.) ;
#26128=EDGE_CURVE('',#21005,#21006,#18032,.T.) ;
#26129=EDGE_CURVE('',#21006,#20546,#18033,.T.) ;
#26130=EDGE_CURVE('',#20545,#21005,#18034,.T.) ;
#26131=EDGE_CURVE('',#20977,#21006,#3905,.T.) ;
#26132=EDGE_CURVE('',#21005,#20978,#3906,.T.) ;
#26133=EDGE_CURVE('',#20978,#20975,#3907,.T.) ;
#26134=EDGE_CURVE('',#21007,#21008,#18035,.T.) ;
#26135=EDGE_CURVE('',#21008,#20976,#3908,.T.) ;
#26136=EDGE_CURVE('',#20975,#21007,#3909,.T.) ;
#26137=EDGE_CURVE('',#20543,#21008,#18036,.T.) ;
#26138=EDGE_CURVE('',#21007,#20544,#18037,.T.) ;
#26139=EDGE_CURVE('',#21009,#20765,#235,.T.) ;
#26140=EDGE_CURVE('',#20301,#21009,#236,.T.) ;
#26141=EDGE_CURVE('',#21010,#20983,#3910,.T.) ;
#26142=EDGE_CURVE('',#21011,#21010,#3911,.T.) ;
#26143=EDGE_CURVE('',#20982,#21011,#3912,.T.) ;
#26144=EDGE_CURVE('',#20984,#21012,#3913,.T.) ;
#26145=EDGE_CURVE('',#21010,#21012,#18038,.T.) ;
#26146=EDGE_CURVE('',#21013,#20985,#3914,.T.) ;
#26147=EDGE_CURVE('',#21012,#21013,#3915,.T.) ;
#26148=EDGE_CURVE('',#20986,#21014,#3916,.T.) ;
#26149=EDGE_CURVE('',#21013,#21014,#18039,.T.) ;
#26150=EDGE_CURVE('',#21015,#20987,#3917,.T.) ;
#26151=EDGE_CURVE('',#21014,#21015,#18040,.T.) ;
#26152=EDGE_CURVE('',#21016,#20988,#3918,.T.) ;
#26153=EDGE_CURVE('',#21015,#21016,#3919,.T.) ;
#26154=EDGE_CURVE('',#21017,#20989,#3920,.T.) ;
#26155=EDGE_CURVE('',#21016,#21017,#18041,.T.) ;
#26156=EDGE_CURVE('',#20990,#21018,#3921,.T.) ;
#26157=EDGE_CURVE('',#21017,#21018,#18042,.T.) ;
#26158=EDGE_CURVE('',#21019,#20991,#3922,.T.) ;
#26159=EDGE_CURVE('',#21018,#21019,#3923,.T.) ;
#26160=EDGE_CURVE('',#20992,#21020,#3924,.T.) ;
#26161=EDGE_CURVE('',#21019,#21020,#18043,.T.) ;
#26162=EDGE_CURVE('',#21021,#20993,#3925,.T.) ;
#26163=EDGE_CURVE('',#21020,#21021,#3926,.T.) ;
#26164=EDGE_CURVE('',#20994,#21022,#3927,.T.) ;
#26165=EDGE_CURVE('',#21021,#21022,#18044,.T.) ;
#26166=EDGE_CURVE('',#21023,#20995,#3928,.T.) ;
#26167=EDGE_CURVE('',#21022,#21023,#3929,.T.) ;
#26168=EDGE_CURVE('',#21024,#20996,#3930,.T.) ;
#26169=EDGE_CURVE('',#21023,#21024,#18045,.T.) ;
#26170=EDGE_CURVE('',#21025,#20997,#3931,.T.) ;
#26171=EDGE_CURVE('',#21024,#21025,#3932,.T.) ;
#26172=EDGE_CURVE('',#20998,#21026,#3933,.T.) ;
#26173=EDGE_CURVE('',#21025,#21026,#18046,.T.) ;
#26174=EDGE_CURVE('',#21027,#20999,#3934,.T.) ;
#26175=EDGE_CURVE('',#21026,#21027,#3935,.T.) ;
#26176=EDGE_CURVE('',#21000,#21028,#3936,.T.) ;
#26177=EDGE_CURVE('',#21027,#21028,#18047,.T.) ;
#26178=EDGE_CURVE('',#21029,#21001,#3937,.T.) ;
#26179=EDGE_CURVE('',#21028,#21029,#3938,.T.) ;
#26180=EDGE_CURVE('',#21002,#21030,#3939,.T.) ;
#26181=EDGE_CURVE('',#21029,#21030,#18048,.T.) ;
#26182=EDGE_CURVE('',#21031,#21003,#3940,.T.) ;
#26183=EDGE_CURVE('',#21030,#21031,#3941,.T.) ;
#26184=EDGE_CURVE('',#21004,#21032,#3942,.T.) ;
#26185=EDGE_CURVE('',#21031,#21032,#18049,.T.) ;
#26186=EDGE_CURVE('',#21032,#21008,#3943,.T.) ;
#26187=EDGE_CURVE('',#21032,#20542,#18050,.T.) ;
#26188=EDGE_CURVE('',#21033,#21034,#18051,.T.) ;
#26189=EDGE_CURVE('',#21034,#21035,#3944,.T.) ;
#26190=EDGE_CURVE('',#21035,#21036,#18052,.T.) ;
#26191=EDGE_CURVE('',#21036,#21033,#3945,.T.) ;
#26192=EDGE_CURVE('',#20369,#21037,#18053,.T.) ;
#26193=EDGE_CURVE('',#21037,#21036,#18054,.T.) ;
#26194=EDGE_CURVE('',#21035,#20369,#18055,.T.) ;
#26195=EDGE_CURVE('',#20368,#21037,#237,.F.) ;
#26196=EDGE_CURVE('',#21035,#21038,#3946,.T.) ;
#26197=EDGE_CURVE('',#20370,#21038,#18056,.T.) ;
#26198=EDGE_CURVE('',#21039,#21034,#3947,.T.) ;
#26199=EDGE_CURVE('',#21038,#21039,#3948,.T.) ;
#26200=EDGE_CURVE('',#21033,#21040,#3949,.T.) ;
#26201=EDGE_CURVE('',#21040,#21041,#3950,.T.) ;
#26202=EDGE_CURVE('',#21041,#21042,#3951,.T.) ;
#26203=EDGE_CURVE('',#21039,#21042,#18057,.T.) ;
#26204=EDGE_CURVE('',#21042,#21043,#3952,.T.) ;
#26205=EDGE_CURVE('',#21043,#21038,#18058,.T.) ;
#26206=EDGE_CURVE('',#21044,#20370,#18059,.T.) ;
#26207=EDGE_CURVE('',#21043,#21044,#18060,.T.) ;
#26208=EDGE_CURVE('',#20371,#21044,#238,.T.) ;
#26209=EDGE_CURVE('',#21041,#20596,#3953,.T.) ;
#26210=EDGE_CURVE('',#21044,#20596,#3954,.T.) ;
#26211=EDGE_CURVE('',#21045,#20382,#18061,.T.) ;
#26212=EDGE_CURVE('',#21046,#21045,#18062,.F.) ;
#26213=EDGE_CURVE('',#20367,#21046,#18063,.T.) ;
#26214=EDGE_CURVE('',#21047,#21048,#18064,.F.) ;
#26215=EDGE_CURVE('',#20381,#21047,#18065,.T.) ;
#26216=EDGE_CURVE('',#21048,#20380,#18066,.T.) ;
#26217=EDGE_CURVE('',#21047,#21045,#3955,.T.) ;
#26218=EDGE_CURVE('',#21049,#21050,#18067,.F.) ;
#26219=EDGE_CURVE('',#20379,#21049,#18068,.T.) ;
#26220=EDGE_CURVE('',#21050,#20378,#18069,.T.) ;
#26221=EDGE_CURVE('',#21049,#21048,#3956,.T.) ;
#26222=EDGE_CURVE('',#21051,#21052,#18070,.F.) ;
#26223=EDGE_CURVE('',#20377,#21051,#18071,.T.) ;
#26224=EDGE_CURVE('',#21052,#20376,#18072,.T.) ;
#26225=EDGE_CURVE('',#21051,#21050,#3957,.T.) ;
#26226=EDGE_CURVE('',#21053,#21054,#18073,.F.) ;
#26227=EDGE_CURVE('',#20375,#21053,#18074,.T.) ;
#26228=EDGE_CURVE('',#21054,#20374,#18075,.T.) ;
#26229=EDGE_CURVE('',#21053,#21052,#3958,.T.) ;
#26230=EDGE_CURVE('',#21055,#20372,#18076,.T.) ;
#26231=EDGE_CURVE('',#21056,#21055,#18077,.F.) ;
#26232=EDGE_CURVE('',#20373,#21056,#18078,.T.) ;
#26233=EDGE_CURVE('',#21044,#21055,#3959,.T.) ;
#26234=EDGE_CURVE('',#20594,#21056,#3960,.T.) ;
#26235=EDGE_CURVE('',#21055,#20595,#3961,.T.) ;
#26236=EDGE_CURVE('',#21056,#21054,#3962,.T.) ;
#26237=EDGE_CURVE('',#20592,#21053,#3963,.T.) ;
#26238=EDGE_CURVE('',#21054,#20593,#3964,.T.) ;
#26239=EDGE_CURVE('',#20590,#21051,#3965,.T.) ;
#26240=EDGE_CURVE('',#21052,#20591,#3966,.T.) ;
#26241=EDGE_CURVE('',#20588,#21049,#3967,.T.) ;
#26242=EDGE_CURVE('',#21050,#20589,#3968,.T.) ;
#26243=EDGE_CURVE('',#20586,#21047,#3969,.T.) ;
#26244=EDGE_CURVE('',#21048,#20587,#3970,.T.) ;
#26245=EDGE_CURVE('',#20598,#21046,#3971,.T.) ;
#26246=EDGE_CURVE('',#21045,#20585,#3972,.T.) ;
#26247=EDGE_CURVE('',#21046,#21037,#3973,.T.) ;
#26248=EDGE_CURVE('',#20390,#21057,#18079,.F.) ;
#26249=EDGE_CURVE('',#21058,#20390,#18080,.F.) ;
#26250=EDGE_CURVE('',#21057,#21058,#18081,.F.) ;
#26251=EDGE_CURVE('',#21059,#20391,#18082,.T.) ;
#26252=EDGE_CURVE('',#21060,#21059,#18083,.F.) ;
#26253=EDGE_CURVE('',#20392,#21060,#18084,.T.) ;
#26254=EDGE_CURVE('',#21057,#21059,#3974,.T.) ;
#26255=EDGE_CURVE('',#20841,#21060,#3975,.T.) ;
#26256=EDGE_CURVE('',#21059,#20839,#3976,.T.) ;
#26257=EDGE_CURVE('',#21061,#20388,#18085,.T.) ;
#26258=EDGE_CURVE('',#21062,#21061,#18086,.F.) ;
#26259=EDGE_CURVE('',#20389,#21062,#18087,.T.) ;
#26260=EDGE_CURVE('',#20856,#20393,#18088,.T.) ;
#26261=EDGE_CURVE('',#20394,#20855,#18089,.T.) ;
#26262=EDGE_CURVE('',#21060,#20856,#3977,.T.) ;
#26263=EDGE_CURVE('',#21063,#20863,#18090,.F.) ;
#26264=EDGE_CURVE('',#20387,#21063,#18091,.T.) ;
#26265=EDGE_CURVE('',#20863,#20386,#18092,.T.) ;
#26266=EDGE_CURVE('',#21063,#21061,#3978,.T.) ;
#26267=EDGE_CURVE('',#20857,#20395,#18093,.T.) ;
#26268=EDGE_CURVE('',#20396,#20858,#18094,.T.) ;
#26269=EDGE_CURVE('',#20385,#20862,#18095,.F.) ;
#26270=EDGE_CURVE('',#20861,#20385,#18096,.F.) ;
#26271=EDGE_CURVE('',#20859,#20384,#18097,.T.) ;
#26272=EDGE_CURVE('',#20383,#20860,#18098,.T.) ;
#26273=EDGE_CURVE('',#20851,#21063,#3979,.T.) ;
#26274=EDGE_CURVE('',#20853,#21062,#3980,.T.) ;
#26275=EDGE_CURVE('',#21061,#20852,#3981,.T.) ;
#26276=EDGE_CURVE('',#21062,#21058,#3982,.T.) ;
#26277=EDGE_CURVE('',#20840,#21057,#3983,.T.) ;
#26278=EDGE_CURVE('',#21058,#20854,#3984,.T.) ;
#26279=EDGE_CURVE('',#21064,#21065,#18099,.T.) ;
#26280=EDGE_CURVE('',#21065,#21066,#3985,.T.) ;
#26281=EDGE_CURVE('',#21066,#21067,#18100,.T.) ;
#26282=EDGE_CURVE('',#21067,#21064,#3986,.T.) ;
#26283=EDGE_CURVE('',#20819,#20444,#18101,.T.) ;
#26284=EDGE_CURVE('',#20444,#21067,#18102,.T.) ;
#26285=EDGE_CURVE('',#21066,#20819,#18103,.T.) ;
#26286=EDGE_CURVE('',#21068,#21065,#3987,.T.) ;
#26287=EDGE_CURVE('',#21068,#20608,#3988,.T.) ;
#26288=EDGE_CURVE('',#21069,#21070,#18104,.T.) ;
#26289=EDGE_CURVE('',#21070,#21071,#3989,.T.) ;
#26290=EDGE_CURVE('',#21071,#21072,#18105,.T.) ;
#26291=EDGE_CURVE('',#21072,#21069,#3990,.T.) ;
#26292=EDGE_CURVE('',#20456,#20814,#18106,.T.) ;
#26293=EDGE_CURVE('',#20814,#21072,#18107,.T.) ;
#26294=EDGE_CURVE('',#21071,#20456,#18108,.T.) ;
#26295=EDGE_CURVE('',#21071,#21067,#3991,.T.) ;
#26296=EDGE_CURVE('',#21064,#21070,#3992,.T.) ;
#26297=EDGE_CURVE('',#20453,#20945,#18109,.T.) ;
#26298=EDGE_CURVE('',#20944,#20452,#18110,.T.) ;
#26299=EDGE_CURVE('',#20451,#20943,#18111,.T.) ;
#26300=EDGE_CURVE('',#20942,#20450,#18112,.T.) ;
#26301=EDGE_CURVE('',#20449,#20941,#18113,.T.) ;
#26302=EDGE_CURVE('',#20940,#20448,#18114,.T.) ;
#26303=EDGE_CURVE('',#20447,#20939,#18115,.T.) ;
#26304=EDGE_CURVE('',#20938,#20446,#18116,.T.) ;
#26305=EDGE_CURVE('',#21073,#21074,#18117,.T.) ;
#26306=EDGE_CURVE('',#21074,#21075,#3993,.T.) ;
#26307=EDGE_CURVE('',#21075,#21076,#18118,.T.) ;
#26308=EDGE_CURVE('',#21076,#21073,#3994,.T.) ;
#26309=EDGE_CURVE('',#20413,#20882,#18119,.T.) ;
#26310=EDGE_CURVE('',#20882,#21076,#18120,.T.) ;
#26311=EDGE_CURVE('',#21075,#20413,#18121,.T.) ;
#26312=EDGE_CURVE('',#20412,#20882,#239,.F.) ;
#26313=EDGE_CURVE('',#21075,#21077,#3995,.T.) ;
#26314=EDGE_CURVE('',#20414,#21077,#18122,.T.) ;
#26315=EDGE_CURVE('',#21078,#21074,#3996,.T.) ;
#26316=EDGE_CURVE('',#21077,#21078,#3997,.T.) ;
#26317=EDGE_CURVE('',#21073,#21079,#3998,.T.) ;
#26318=EDGE_CURVE('',#21079,#21080,#3999,.T.) ;
#26319=EDGE_CURVE('',#21080,#21081,#4000,.T.) ;
#26320=EDGE_CURVE('',#21078,#21081,#18123,.T.) ;
#26321=EDGE_CURVE('',#21081,#21082,#4001,.T.) ;
#26322=EDGE_CURVE('',#21082,#21077,#18124,.T.) ;
#26323=EDGE_CURVE('',#21083,#20414,#18125,.T.) ;
#26324=EDGE_CURVE('',#21082,#21083,#18126,.T.) ;
#26325=EDGE_CURVE('',#20415,#21083,#240,.T.) ;
#26326=EDGE_CURVE('',#21080,#20583,#4002,.T.) ;
#26327=EDGE_CURVE('',#21083,#20881,#4003,.T.) ;
#26328=EDGE_CURVE('',#21084,#21085,#18127,.F.) ;
#26329=EDGE_CURVE('',#20418,#21084,#18128,.T.) ;
#26330=EDGE_CURVE('',#21085,#20417,#18129,.T.) ;
#26331=EDGE_CURVE('',#21086,#21087,#18130,.F.) ;
#26332=EDGE_CURVE('',#20420,#21086,#18131,.T.) ;
#26333=EDGE_CURVE('',#21087,#20419,#18132,.T.) ;
#26334=EDGE_CURVE('',#21088,#21089,#18133,.F.) ;
#26335=EDGE_CURVE('',#20422,#21088,#18134,.T.) ;
#26336=EDGE_CURVE('',#21089,#20421,#18135,.T.) ;
#26337=EDGE_CURVE('',#21090,#21091,#18136,.F.) ;
#26338=EDGE_CURVE('',#20424,#21090,#18137,.T.) ;
#26339=EDGE_CURVE('',#21091,#20423,#18138,.T.) ;
#26340=EDGE_CURVE('',#21090,#20878,#4004,.T.) ;
#26341=EDGE_CURVE('',#21088,#21091,#4005,.T.) ;
#26342=EDGE_CURVE('',#20868,#21090,#4006,.T.) ;
#26343=EDGE_CURVE('',#21091,#20869,#4007,.T.) ;
#26344=EDGE_CURVE('',#21086,#21089,#4008,.T.) ;
#26345=EDGE_CURVE('',#20870,#21088,#4009,.T.) ;
#26346=EDGE_CURVE('',#21089,#20871,#4010,.T.) ;
#26347=EDGE_CURVE('',#21084,#21087,#4011,.T.) ;
#26348=EDGE_CURVE('',#20872,#21086,#4012,.T.) ;
#26349=EDGE_CURVE('',#21087,#20873,#4013,.T.) ;
#26350=EDGE_CURVE('',#20879,#21085,#4014,.T.) ;
#26351=EDGE_CURVE('',#20874,#21084,#4015,.T.) ;
#26352=EDGE_CURVE('',#21085,#20875,#4016,.T.) ;
#26353=EDGE_CURVE('',#21083,#20880,#4017,.T.) ;
#26354=EDGE_CURVE('',#20884,#20956,#4018,.T.) ;
#26355=EDGE_CURVE('',#20906,#20966,#4019,.T.) ;
#26356=EDGE_CURVE('',#21092,#20463,#18139,.T.) ;
#26357=EDGE_CURVE('',#21093,#21092,#18140,.F.) ;
#26358=EDGE_CURVE('',#20464,#21093,#18141,.T.) ;
#26359=EDGE_CURVE('',#21094,#21095,#18142,.F.) ;
#26360=EDGE_CURVE('',#20604,#21094,#18143,.T.) ;
#26361=EDGE_CURVE('',#21095,#20603,#18144,.T.) ;
#26362=EDGE_CURVE('',#21096,#20461,#18145,.T.) ;
#26363=EDGE_CURVE('',#21097,#21096,#18146,.F.) ;
#26364=EDGE_CURVE('',#20462,#21097,#18147,.T.) ;
#26365=EDGE_CURVE('',#21098,#21099,#18148,.F.) ;
#26366=EDGE_CURVE('',#20466,#21098,#18149,.T.) ;
#26367=EDGE_CURVE('',#21099,#20465,#18150,.T.) ;
#26368=EDGE_CURVE('',#21100,#20601,#18151,.T.) ;
#26369=EDGE_CURVE('',#21101,#21100,#18152,.F.) ;
#26370=EDGE_CURVE('',#20602,#21101,#18153,.T.) ;
#26371=EDGE_CURVE('',#21102,#21103,#18154,.F.) ;
#26372=EDGE_CURVE('',#20606,#21102,#18155,.T.) ;
#26373=EDGE_CURVE('',#21103,#20605,#18156,.T.) ;
#26374=EDGE_CURVE('',#21104,#20460,#18157,.T.) ;
#26375=EDGE_CURVE('',#21105,#21104,#18158,.F.) ;
#26376=EDGE_CURVE('',#20459,#21105,#18159,.T.) ;
#26377=EDGE_CURVE('',#21098,#21104,#4020,.T.) ;
#26378=EDGE_CURVE('',#21106,#21107,#18160,.F.) ;
#26379=EDGE_CURVE('',#20599,#21106,#18161,.T.) ;
#26380=EDGE_CURVE('',#21107,#20600,#18162,.T.) ;
#26381=EDGE_CURVE('',#21106,#21100,#4021,.T.) ;
#26382=EDGE_CURVE('',#21102,#21107,#4022,.T.) ;
#26383=EDGE_CURVE('',#21104,#21106,#4023,.T.) ;
#26384=EDGE_CURVE('',#21107,#21105,#4024,.T.) ;
#26385=EDGE_CURVE('',#21105,#21096,#4025,.T.) ;
#26386=EDGE_CURVE('',#21094,#21103,#4026,.T.) ;
#26387=EDGE_CURVE('',#21096,#21102,#4027,.T.) ;
#26388=EDGE_CURVE('',#21103,#21097,#4028,.T.) ;
#26389=EDGE_CURVE('',#21099,#21101,#4029,.T.) ;
#26390=EDGE_CURVE('',#21100,#21098,#4030,.T.) ;
#26391=EDGE_CURVE('',#21101,#21095,#4031,.T.) ;
#26392=EDGE_CURVE('',#21093,#21099,#4032,.T.) ;
#26393=EDGE_CURVE('',#21097,#21092,#4033,.T.) ;
#26394=EDGE_CURVE('',#21092,#21094,#4034,.T.) ;
#26395=EDGE_CURVE('',#21095,#21093,#4035,.T.) ;
#26396=EDGE_CURVE('',#20566,#21108,#18163,.T.) ;
#26397=EDGE_CURVE('',#21108,#21108,#18164,.T.) ;
#26398=EDGE_CURVE('',#21108,#21109,#4036,.T.) ;
#26399=EDGE_CURVE('',#21110,#21109,#18165,.T.) ;
#26400=EDGE_CURVE('',#21109,#21110,#18166,.T.) ;
#26401=EDGE_CURVE('',#20425,#21110,#18167,.T.) ;
#26402=EDGE_CURVE('',#21111,#21112,#18168,.T.) ;
#26403=EDGE_CURVE('',#21112,#21113,#4037,.T.) ;
#26404=EDGE_CURVE('',#21113,#21114,#18169,.T.) ;
#26405=EDGE_CURVE('',#21114,#21111,#4038,.T.) ;
#26406=EDGE_CURVE('',#20828,#20440,#18170,.T.) ;
#26407=EDGE_CURVE('',#20440,#21114,#18171,.T.) ;
#26408=EDGE_CURVE('',#21113,#20828,#18172,.T.) ;
#26409=EDGE_CURVE('',#20426,#20828,#241,.T.) ;
#26410=EDGE_CURVE('',#21115,#21112,#4039,.T.) ;
#26411=EDGE_CURVE('',#21115,#20498,#4040,.T.) ;
#26412=EDGE_CURVE('',#21111,#21116,#4041,.T.) ;
#26413=EDGE_CURVE('',#21117,#21116,#18173,.T.) ;
#26414=EDGE_CURVE('',#21117,#21118,#4042,.T.) ;
#26415=EDGE_CURVE('',#21118,#21115,#4043,.T.) ;
#26416=EDGE_CURVE('',#21119,#21114,#4044,.T.) ;
#26417=EDGE_CURVE('',#21116,#21119,#4045,.T.) ;
#26418=EDGE_CURVE('',#21119,#21120,#18174,.T.) ;
#26419=EDGE_CURVE('',#21120,#21117,#4046,.T.) ;
#26420=EDGE_CURVE('',#20439,#21121,#18175,.T.) ;
#26421=EDGE_CURVE('',#21121,#21120,#18176,.T.) ;
#26422=EDGE_CURVE('',#21119,#20439,#18177,.T.) ;
#26423=EDGE_CURVE('',#20438,#21121,#242,.F.) ;
#26424=EDGE_CURVE('',#20436,#20837,#18178,.T.) ;
#26425=EDGE_CURVE('',#20836,#20435,#18179,.T.) ;
#26426=EDGE_CURVE('',#20838,#20437,#243,.T.) ;
#26427=EDGE_CURVE('',#20434,#20835,#18180,.T.) ;
#26428=EDGE_CURVE('',#20834,#20433,#18181,.T.) ;
#26429=EDGE_CURVE('',#20432,#20833,#18182,.T.) ;
#26430=EDGE_CURVE('',#20832,#20431,#18183,.T.) ;
#26431=EDGE_CURVE('',#20430,#20831,#18184,.T.) ;
#26432=EDGE_CURVE('',#20830,#20429,#18185,.T.) ;
#26433=EDGE_CURVE('',#20428,#20829,#18186,.T.) ;
#26434=EDGE_CURVE('',#20827,#20427,#18187,.T.) ;
#26435=EDGE_CURVE('',#20838,#21121,#4047,.T.) ;
#26436=EDGE_CURVE('',#20308,#21122,#18188,.T.) ;
#26437=EDGE_CURVE('',#21122,#21123,#18189,.T.) ;
#26438=EDGE_CURVE('',#21123,#21122,#18190,.T.) ;
#26439=EDGE_CURVE('',#20567,#21123,#4048,.T.) ;
#26440=EDGE_CURVE('',#20458,#21124,#18191,.T.) ;
#26441=EDGE_CURVE('',#21124,#21125,#18192,.T.) ;
#26442=EDGE_CURVE('',#21125,#21124,#18193,.T.) ;
#26443=EDGE_CURVE('',#20584,#21125,#4049,.T.) ;
#26444=EDGE_CURVE('',#20694,#20519,#18194,.T.) ;
#26445=EDGE_CURVE('',#21011,#20520,#18195,.T.) ;
#26446=EDGE_CURVE('',#20694,#21011,#18196,.T.) ;
#26447=EDGE_CURVE('',#21010,#20521,#18197,.T.) ;
#26448=EDGE_CURVE('',#21012,#20522,#18198,.T.) ;
#26449=EDGE_CURVE('',#21013,#20523,#18199,.T.) ;
#26450=EDGE_CURVE('',#21014,#20524,#18200,.T.) ;
#26451=EDGE_CURVE('',#21015,#20525,#18201,.T.) ;
#26452=EDGE_CURVE('',#21016,#20526,#18202,.T.) ;
#26453=EDGE_CURVE('',#21017,#20527,#18203,.T.) ;
#26454=EDGE_CURVE('',#21018,#20528,#18204,.T.) ;
#26455=EDGE_CURVE('',#21019,#20529,#18205,.T.) ;
#26456=EDGE_CURVE('',#21020,#20530,#18206,.T.) ;
#26457=EDGE_CURVE('',#21021,#20531,#18207,.T.) ;
#26458=EDGE_CURVE('',#21022,#20532,#18208,.T.) ;
#26459=EDGE_CURVE('',#21023,#20533,#18209,.T.) ;
#26460=EDGE_CURVE('',#21024,#20534,#18210,.T.) ;
#26461=EDGE_CURVE('',#21025,#20535,#18211,.T.) ;
#26462=EDGE_CURVE('',#21026,#20536,#18212,.T.) ;
#26463=EDGE_CURVE('',#21027,#20537,#18213,.T.) ;
#26464=EDGE_CURVE('',#21028,#20538,#18214,.T.) ;
#26465=EDGE_CURVE('',#21029,#20539,#18215,.T.) ;
#26466=EDGE_CURVE('',#21030,#20540,#18216,.T.) ;
#26467=EDGE_CURVE('',#21031,#20541,#18217,.T.) ;
#26468=EDGE_CURVE('',#20549,#21126,#18218,.T.) ;
#26469=EDGE_CURVE('',#21126,#20704,#18219,.T.) ;
#26470=EDGE_CURVE('',#20548,#21127,#18220,.T.) ;
#26471=EDGE_CURVE('',#21127,#21126,#4050,.T.) ;
#26472=EDGE_CURVE('',#20547,#21128,#18221,.T.) ;
#26473=EDGE_CURVE('',#21128,#21127,#18222,.T.) ;
#26474=EDGE_CURVE('',#21006,#21128,#4051,.T.) ;
#26475=EDGE_CURVE('',#20716,#21129,#18223,.T.) ;
#26476=EDGE_CURVE('',#21129,#21129,#18224,.T.) ;
#26477=EDGE_CURVE('',#21130,#21130,#18225,.T.) ;
#26478=EDGE_CURVE('',#21131,#21132,#18226,.T.) ;
#26479=EDGE_CURVE('',#21132,#21130,#18227,.T.) ;
#26480=EDGE_CURVE('',#21132,#21131,#18228,.T.) ;
#26481=EDGE_CURVE('',#21133,#21133,#18229,.T.) ;
#26482=EDGE_CURVE('',#21133,#21131,#4052,.T.) ;
#26483=EDGE_CURVE('',#21133,#21134,#18230,.T.) ;
#26484=EDGE_CURVE('',#21134,#21135,#18231,.T.) ;
#26485=EDGE_CURVE('',#21135,#21134,#18232,.T.) ;
#26486=EDGE_CURVE('',#21136,#21136,#18233,.T.) ;
#26487=EDGE_CURVE('',#21136,#21137,#18234,.T.) ;
#26488=EDGE_CURVE('',#21137,#21138,#18235,.T.) ;
#26489=EDGE_CURVE('',#21138,#21137,#18236,.T.) ;
#26490=EDGE_CURVE('',#21136,#21139,#4053,.T.) ;
#26491=EDGE_CURVE('',#21140,#21139,#18237,.T.) ;
#26492=EDGE_CURVE('',#21139,#21140,#18238,.T.) ;
#26493=EDGE_CURVE('',#21140,#21141,#18239,.T.) ;
#26494=EDGE_CURVE('',#21141,#21141,#18240,.T.) ;
#26495=EDGE_CURVE('',#21142,#21142,#18241,.T.) ;
#26496=EDGE_CURVE('',#21143,#21143,#18242,.T.) ;
#26497=EDGE_CURVE('',#21143,#21142,#18243,.T.) ;
#26498=EDGE_CURVE('',#21144,#21144,#18244,.F.) ;
#26499=EDGE_CURVE('',#21144,#21143,#4054,.T.) ;
#26500=EDGE_CURVE('',#21145,#21145,#18245,.T.) ;
#26501=EDGE_CURVE('',#21145,#21146,#18246,.T.) ;
#26502=EDGE_CURVE('',#21146,#21147,#18247,.T.) ;
#26503=EDGE_CURVE('',#21147,#21146,#18248,.T.) ;
#26504=EDGE_CURVE('',#21145,#21148,#4055,.T.) ;
#26505=EDGE_CURVE('',#21149,#21148,#18249,.T.) ;
#26506=EDGE_CURVE('',#21148,#21149,#18250,.T.) ;
#26507=EDGE_CURVE('',#20490,#21150,#18251,.T.) ;
#26508=EDGE_CURVE('',#21150,#21150,#18252,.T.) ;
#26509=EDGE_CURVE('',#21151,#21151,#18253,.T.) ;
#26510=EDGE_CURVE('',#21149,#21151,#18254,.T.) ;
#26511=EDGE_CURVE('',#21135,#20441,#18255,.T.) ;
#26512=EDGE_CURVE('',#21138,#20457,#18256,.T.) ;
#26513=EDGE_CURVE('',#21147,#20442,#18257,.T.) ;
#26514=EDGE_CURVE('',#20980,#21127,#4056,.T.) ;
#26515=EDGE_CURVE('',#21128,#20981,#4057,.T.) ;
#26516=EDGE_CURVE('',#21126,#20979,#4058,.T.) ;
#26517=EDGE_CURVE('',#20758,#20314,#244,.T.) ;
#26518=EDGE_CURVE('',#20314,#21152,#245,.T.) ;
#26519=EDGE_CURVE('',#21152,#20758,#18258,.T.) ;
#26520=EDGE_CURVE('',#21153,#21154,#246,.T.) ;
#26521=EDGE_CURVE('',#21154,#20309,#247,.T.) ;
#26522=EDGE_CURVE('',#20309,#21155,#248,.T.) ;
#26523=EDGE_CURVE('',#21155,#20761,#249,.T.) ;
#26524=EDGE_CURVE('',#20761,#21153,#18259,.T.) ;
#26525=EDGE_CURVE('',#20762,#21156,#250,.T.) ;
#26526=EDGE_CURVE('',#21156,#20306,#251,.T.) ;
#26527=EDGE_CURVE('',#20306,#21157,#252,.T.) ;
#26528=EDGE_CURVE('',#21157,#21158,#253,.T.) ;
#26529=EDGE_CURVE('',#21158,#20762,#18260,.T.) ;
#26530=EDGE_CURVE('',#21159,#21160,#254,.T.) ;
#26531=EDGE_CURVE('',#21160,#20301,#255,.T.) ;
#26532=EDGE_CURVE('',#20765,#21159,#18261,.T.) ;
#26533=EDGE_CURVE('',#21159,#21161,#4059,.T.) ;
#26534=EDGE_CURVE('',#21161,#20302,#18262,.T.) ;
#26535=EDGE_CURVE('',#20722,#20303,#18263,.T.) ;
#26536=EDGE_CURVE('',#21161,#20722,#256,.T.) ;
#26537=EDGE_CURVE('',#20723,#20304,#18264,.T.) ;
#26538=EDGE_CURVE('',#21162,#20305,#18265,.T.) ;
#26539=EDGE_CURVE('',#20723,#21162,#257,.T.) ;
#26540=EDGE_CURVE('',#21162,#21158,#4060,.T.) ;
#26541=EDGE_CURVE('',#21153,#21163,#4061,.T.) ;
#26542=EDGE_CURVE('',#21163,#20310,#18266,.T.) ;
#26543=EDGE_CURVE('',#20738,#20311,#18267,.T.) ;
#26544=EDGE_CURVE('',#21163,#20738,#258,.T.) ;
#26545=EDGE_CURVE('',#20739,#20312,#18268,.T.) ;
#26546=EDGE_CURVE('',#21164,#20313,#18269,.T.) ;
#26547=EDGE_CURVE('',#20739,#21164,#259,.T.) ;
#26548=EDGE_CURVE('',#21164,#21152,#4062,.T.) ;
#26549=EDGE_CURVE('',#20743,#21165,#18270,.T.) ;
#26550=EDGE_CURVE('',#21165,#21164,#4063,.T.) ;
#26551=EDGE_CURVE('',#21163,#21166,#4064,.T.) ;
#26552=EDGE_CURVE('',#21166,#20740,#18271,.T.) ;
#26553=EDGE_CURVE('',#21166,#21153,#4065,.T.) ;
#26554=EDGE_CURVE('',#21166,#20760,#260,.T.) ;
#26555=EDGE_CURVE('',#21158,#21167,#4066,.T.) ;
#26556=EDGE_CURVE('',#20763,#21167,#261,.T.) ;
#26557=EDGE_CURVE('',#21167,#21162,#4067,.T.) ;
#26558=EDGE_CURVE('',#20727,#21167,#18272,.T.) ;
#26559=EDGE_CURVE('',#21161,#21168,#4068,.T.) ;
#26560=EDGE_CURVE('',#21168,#20724,#18273,.T.) ;
#26561=EDGE_CURVE('',#21168,#21159,#4069,.T.) ;
#26562=EDGE_CURVE('',#21168,#20764,#262,.T.) ;
#26563=EDGE_CURVE('',#21169,#20609,#4070,.T.) ;
#26564=EDGE_CURVE('',#21069,#21169,#4071,.T.) ;
#26565=EDGE_CURVE('',#21169,#21068,#4072,.T.) ;
#26566=EDGE_CURVE('',#20499,#21121,#4073,.T.) ;
#26567=EDGE_CURVE('',#21118,#20499,#4074,.T.) ;
#26568=EDGE_CURVE('',#20597,#21037,#4075,.T.) ;
#26569=EDGE_CURVE('',#21040,#20597,#4076,.T.) ;
#26570=EDGE_CURVE('',#21079,#20569,#4077,.T.) ;
#26571=EDGE_CURVE('',#20745,#20775,#1124,.T.) ;
#26572=EDGE_CURVE('',#20731,#20771,#1125,.T.) ;
#26573=EDGE_CURVE('',#20772,#20514,#4078,.T.) ;
#26574=EDGE_CURVE('',#20511,#20773,#4079,.T.) ;
#26575=EDGE_CURVE('',#20774,#20748,#1126,.T.) ;
#26576=EDGE_CURVE('',#20759,#21165,#263,.T.) ;
#26577=EDGE_CURVE('',#21152,#21165,#4080,.T.) ;
#33100=ORIENTED_EDGE('',*,*,#24828,.T.) ;
#33101=ORIENTED_EDGE('',*,*,#24829,.T.) ;
#33102=ORIENTED_EDGE('',*,*,#24830,.T.) ;
#33103=ORIENTED_EDGE('',*,*,#24831,.F.) ;
#33104=ORIENTED_EDGE('',*,*,#24832,.T.) ;
#33105=ORIENTED_EDGE('',*,*,#24833,.T.) ;
#33106=ORIENTED_EDGE('',*,*,#24834,.T.) ;
#33107=ORIENTED_EDGE('',*,*,#24835,.T.) ;
#33108=ORIENTED_EDGE('',*,*,#24836,.T.) ;
#33109=ORIENTED_EDGE('',*,*,#24837,.T.) ;
#33110=ORIENTED_EDGE('',*,*,#24838,.T.) ;
#33111=ORIENTED_EDGE('',*,*,#24829,.F.) ;
#33112=ORIENTED_EDGE('',*,*,#24839,.T.) ;
#33113=ORIENTED_EDGE('',*,*,#24840,.T.) ;
#33114=ORIENTED_EDGE('',*,*,#24841,.T.) ;
#33115=ORIENTED_EDGE('',*,*,#24837,.F.) ;
#33116=ORIENTED_EDGE('',*,*,#24842,.T.) ;
#33117=ORIENTED_EDGE('',*,*,#24840,.F.) ;
#33118=ORIENTED_EDGE('',*,*,#24843,.T.) ;
#33119=ORIENTED_EDGE('',*,*,#24844,.T.) ;
#33120=ORIENTED_EDGE('',*,*,#24833,.F.) ;
#33121=ORIENTED_EDGE('',*,*,#24845,.T.) ;
#33122=ORIENTED_EDGE('',*,*,#24844,.F.) ;
#33123=ORIENTED_EDGE('',*,*,#24846,.T.) ;
#33124=ORIENTED_EDGE('',*,*,#24847,.T.) ;
#33125=ORIENTED_EDGE('',*,*,#24835,.F.) ;
#33126=ORIENTED_EDGE('',*,*,#24848,.T.) ;
#33127=ORIENTED_EDGE('',*,*,#24849,.T.) ;
#33128=ORIENTED_EDGE('',*,*,#24850,.T.) ;
#33129=ORIENTED_EDGE('',*,*,#24849,.F.) ;
#33130=ORIENTED_EDGE('',*,*,#24851,.T.) ;
#33131=ORIENTED_EDGE('',*,*,#24831,.T.) ;
#33132=ORIENTED_EDGE('',*,*,#24841,.F.) ;
#33133=ORIENTED_EDGE('',*,*,#24852,.F.) ;
#33134=ORIENTED_EDGE('',*,*,#24853,.F.) ;
#33135=ORIENTED_EDGE('',*,*,#24854,.T.) ;
#33136=ORIENTED_EDGE('',*,*,#24842,.F.) ;
#33137=ORIENTED_EDGE('',*,*,#24855,.F.) ;
#33138=ORIENTED_EDGE('',*,*,#24856,.F.) ;
#33139=ORIENTED_EDGE('',*,*,#24852,.T.) ;
#33140=ORIENTED_EDGE('',*,*,#24845,.F.) ;
#33141=ORIENTED_EDGE('',*,*,#24857,.F.) ;
#33142=ORIENTED_EDGE('',*,*,#24858,.F.) ;
#33143=ORIENTED_EDGE('',*,*,#24855,.T.) ;
#33144=ORIENTED_EDGE('',*,*,#24832,.F.) ;
#33145=ORIENTED_EDGE('',*,*,#24859,.F.) ;
#33146=ORIENTED_EDGE('',*,*,#24860,.F.) ;
#33147=ORIENTED_EDGE('',*,*,#24857,.T.) ;
#33148=ORIENTED_EDGE('',*,*,#24861,.F.) ;
#33149=ORIENTED_EDGE('',*,*,#24862,.F.) ;
#33150=ORIENTED_EDGE('',*,*,#24863,.F.) ;
#33151=ORIENTED_EDGE('',*,*,#24864,.F.) ;
#33152=ORIENTED_EDGE('',*,*,#24865,.F.) ;
#33153=ORIENTED_EDGE('',*,*,#24866,.F.) ;
#33154=ORIENTED_EDGE('',*,*,#24867,.F.) ;
#33155=ORIENTED_EDGE('',*,*,#24868,.F.) ;
#33156=ORIENTED_EDGE('',*,*,#24869,.F.) ;
#33157=ORIENTED_EDGE('',*,*,#24870,.F.) ;
#33158=ORIENTED_EDGE('',*,*,#24871,.F.) ;
#33159=ORIENTED_EDGE('',*,*,#24872,.F.) ;
#33160=ORIENTED_EDGE('',*,*,#24873,.F.) ;
#33161=ORIENTED_EDGE('',*,*,#24874,.F.) ;
#33162=ORIENTED_EDGE('',*,*,#24875,.F.) ;
#33163=ORIENTED_EDGE('',*,*,#24876,.F.) ;
#33164=ORIENTED_EDGE('',*,*,#24877,.F.) ;
#33165=ORIENTED_EDGE('',*,*,#24878,.F.) ;
#33166=ORIENTED_EDGE('',*,*,#24879,.F.) ;
#33167=ORIENTED_EDGE('',*,*,#24834,.F.) ;
#33168=ORIENTED_EDGE('',*,*,#24846,.F.) ;
#33169=ORIENTED_EDGE('',*,*,#24843,.F.) ;
#33170=ORIENTED_EDGE('',*,*,#24839,.F.) ;
#33171=ORIENTED_EDGE('',*,*,#24836,.F.) ;
#33172=ORIENTED_EDGE('',*,*,#24828,.F.) ;
#33173=ORIENTED_EDGE('',*,*,#24851,.F.) ;
#33174=ORIENTED_EDGE('',*,*,#24848,.F.) ;
#33175=ORIENTED_EDGE('',*,*,#24868,.T.) ;
#33176=ORIENTED_EDGE('',*,*,#24880,.T.) ;
#33177=ORIENTED_EDGE('',*,*,#24881,.T.) ;
#33178=ORIENTED_EDGE('',*,*,#24882,.F.) ;
#33179=ORIENTED_EDGE('',*,*,#24867,.T.) ;
#33180=ORIENTED_EDGE('',*,*,#24883,.T.) ;
#33181=ORIENTED_EDGE('',*,*,#24884,.T.) ;
#33182=ORIENTED_EDGE('',*,*,#24880,.F.) ;
#33183=ORIENTED_EDGE('',*,*,#24866,.T.) ;
#33184=ORIENTED_EDGE('',*,*,#24885,.T.) ;
#33185=ORIENTED_EDGE('',*,*,#24886,.T.) ;
#33186=ORIENTED_EDGE('',*,*,#24883,.F.) ;
#33187=ORIENTED_EDGE('',*,*,#24865,.T.) ;
#33188=ORIENTED_EDGE('',*,*,#24887,.T.) ;
#33189=ORIENTED_EDGE('',*,*,#24888,.T.) ;
#33190=ORIENTED_EDGE('',*,*,#24885,.F.) ;
#33191=ORIENTED_EDGE('',*,*,#24864,.T.) ;
#33192=ORIENTED_EDGE('',*,*,#24889,.T.) ;
#33193=ORIENTED_EDGE('',*,*,#24890,.T.) ;
#33194=ORIENTED_EDGE('',*,*,#24887,.F.) ;
#33195=ORIENTED_EDGE('',*,*,#24891,.T.) ;
#33196=ORIENTED_EDGE('',*,*,#24892,.T.) ;
#33197=ORIENTED_EDGE('',*,*,#24875,.T.) ;
#33198=ORIENTED_EDGE('',*,*,#24893,.T.) ;
#33199=ORIENTED_EDGE('',*,*,#24863,.T.) ;
#33200=ORIENTED_EDGE('',*,*,#24894,.T.) ;
#33201=ORIENTED_EDGE('',*,*,#24895,.T.) ;
#33202=ORIENTED_EDGE('',*,*,#24889,.F.) ;
#33203=ORIENTED_EDGE('',*,*,#24896,.T.) ;
#33204=ORIENTED_EDGE('',*,*,#24897,.T.) ;
#33205=ORIENTED_EDGE('',*,*,#24861,.T.) ;
#33206=ORIENTED_EDGE('',*,*,#24898,.T.) ;
#33207=ORIENTED_EDGE('',*,*,#24862,.T.) ;
#33208=ORIENTED_EDGE('',*,*,#24897,.F.) ;
#33209=ORIENTED_EDGE('',*,*,#24899,.T.) ;
#33210=ORIENTED_EDGE('',*,*,#24894,.F.) ;
#33211=ORIENTED_EDGE('',*,*,#24879,.T.) ;
#33212=ORIENTED_EDGE('',*,*,#24900,.T.) ;
#33213=ORIENTED_EDGE('',*,*,#24901,.T.) ;
#33214=ORIENTED_EDGE('',*,*,#24898,.F.) ;
#33215=ORIENTED_EDGE('',*,*,#24902,.T.) ;
#33216=ORIENTED_EDGE('',*,*,#24900,.F.) ;
#33217=ORIENTED_EDGE('',*,*,#24878,.T.) ;
#33218=ORIENTED_EDGE('',*,*,#24903,.T.) ;
#33219=ORIENTED_EDGE('',*,*,#24904,.T.) ;
#33220=ORIENTED_EDGE('',*,*,#24903,.F.) ;
#33221=ORIENTED_EDGE('',*,*,#24877,.T.) ;
#33222=ORIENTED_EDGE('',*,*,#24905,.T.) ;
#33223=ORIENTED_EDGE('',*,*,#24892,.F.) ;
#33224=ORIENTED_EDGE('',*,*,#24906,.T.) ;
#33225=ORIENTED_EDGE('',*,*,#24905,.F.) ;
#33226=ORIENTED_EDGE('',*,*,#24876,.T.) ;
#33227=ORIENTED_EDGE('',*,*,#24907,.T.) ;
#33228=ORIENTED_EDGE('',*,*,#24893,.F.) ;
#33229=ORIENTED_EDGE('',*,*,#24874,.T.) ;
#33230=ORIENTED_EDGE('',*,*,#24908,.T.) ;
#33231=ORIENTED_EDGE('',*,*,#24909,.T.) ;
#33232=ORIENTED_EDGE('',*,*,#24908,.F.) ;
#33233=ORIENTED_EDGE('',*,*,#24873,.T.) ;
#33234=ORIENTED_EDGE('',*,*,#24910,.T.) ;
#33235=ORIENTED_EDGE('',*,*,#24911,.T.) ;
#33236=ORIENTED_EDGE('',*,*,#24910,.F.) ;
#33237=ORIENTED_EDGE('',*,*,#24872,.T.) ;
#33238=ORIENTED_EDGE('',*,*,#24912,.T.) ;
#33239=ORIENTED_EDGE('',*,*,#24913,.T.) ;
#33240=ORIENTED_EDGE('',*,*,#24912,.F.) ;
#33241=ORIENTED_EDGE('',*,*,#24871,.T.) ;
#33242=ORIENTED_EDGE('',*,*,#24914,.T.) ;
#33243=ORIENTED_EDGE('',*,*,#24915,.T.) ;
#33244=ORIENTED_EDGE('',*,*,#24914,.F.) ;
#33245=ORIENTED_EDGE('',*,*,#24870,.T.) ;
#33246=ORIENTED_EDGE('',*,*,#24916,.T.) ;
#33247=ORIENTED_EDGE('',*,*,#24917,.T.) ;
#33248=ORIENTED_EDGE('',*,*,#24916,.F.) ;
#33249=ORIENTED_EDGE('',*,*,#24869,.T.) ;
#33250=ORIENTED_EDGE('',*,*,#24882,.T.) ;
#33251=ORIENTED_EDGE('',*,*,#24915,.F.) ;
#33252=ORIENTED_EDGE('',*,*,#24918,.F.) ;
#33253=ORIENTED_EDGE('',*,*,#24919,.F.) ;
#33254=ORIENTED_EDGE('',*,*,#24920,.T.) ;
#33255=ORIENTED_EDGE('',*,*,#24917,.F.) ;
#33256=ORIENTED_EDGE('',*,*,#24921,.F.) ;
#33257=ORIENTED_EDGE('',*,*,#24922,.F.) ;
#33258=ORIENTED_EDGE('',*,*,#24918,.T.) ;
#33259=ORIENTED_EDGE('',*,*,#24881,.F.) ;
#33260=ORIENTED_EDGE('',*,*,#24923,.F.) ;
#33261=ORIENTED_EDGE('',*,*,#24924,.F.) ;
#33262=ORIENTED_EDGE('',*,*,#24921,.T.) ;
#33263=ORIENTED_EDGE('',*,*,#24884,.F.) ;
#33264=ORIENTED_EDGE('',*,*,#24925,.F.) ;
#33265=ORIENTED_EDGE('',*,*,#24926,.F.) ;
#33266=ORIENTED_EDGE('',*,*,#24923,.T.) ;
#33267=ORIENTED_EDGE('',*,*,#24886,.F.) ;
#33268=ORIENTED_EDGE('',*,*,#24927,.F.) ;
#33269=ORIENTED_EDGE('',*,*,#24928,.F.) ;
#33270=ORIENTED_EDGE('',*,*,#24925,.T.) ;
#33271=ORIENTED_EDGE('',*,*,#24888,.F.) ;
#33272=ORIENTED_EDGE('',*,*,#24929,.F.) ;
#33273=ORIENTED_EDGE('',*,*,#24930,.F.) ;
#33274=ORIENTED_EDGE('',*,*,#24927,.T.) ;
#33275=ORIENTED_EDGE('',*,*,#24890,.F.) ;
#33276=ORIENTED_EDGE('',*,*,#24931,.F.) ;
#33277=ORIENTED_EDGE('',*,*,#24932,.F.) ;
#33278=ORIENTED_EDGE('',*,*,#24929,.T.) ;
#33279=ORIENTED_EDGE('',*,*,#24895,.F.) ;
#33280=ORIENTED_EDGE('',*,*,#24933,.F.) ;
#33281=ORIENTED_EDGE('',*,*,#24934,.F.) ;
#33282=ORIENTED_EDGE('',*,*,#24931,.T.) ;
#33283=ORIENTED_EDGE('',*,*,#24899,.F.) ;
#33284=ORIENTED_EDGE('',*,*,#24935,.F.) ;
#33285=ORIENTED_EDGE('',*,*,#24936,.F.) ;
#33286=ORIENTED_EDGE('',*,*,#24933,.T.) ;
#33287=ORIENTED_EDGE('',*,*,#24896,.F.) ;
#33288=ORIENTED_EDGE('',*,*,#24937,.F.) ;
#33289=ORIENTED_EDGE('',*,*,#24938,.F.) ;
#33290=ORIENTED_EDGE('',*,*,#24935,.T.) ;
#33291=ORIENTED_EDGE('',*,*,#24939,.T.) ;
#33292=ORIENTED_EDGE('',*,*,#24940,.T.) ;
#33293=ORIENTED_EDGE('',*,*,#24941,.T.) ;
#33294=ORIENTED_EDGE('',*,*,#24942,.F.) ;
#33295=ORIENTED_EDGE('',*,*,#24943,.T.) ;
#33296=ORIENTED_EDGE('',*,*,#24944,.T.) ;
#33297=ORIENTED_EDGE('',*,*,#24945,.T.) ;
#33298=ORIENTED_EDGE('',*,*,#24858,.T.) ;
#33299=ORIENTED_EDGE('',*,*,#24946,.T.) ;
#33300=ORIENTED_EDGE('',*,*,#24947,.T.) ;
#33301=ORIENTED_EDGE('',*,*,#24853,.T.) ;
#33302=ORIENTED_EDGE('',*,*,#24948,.T.) ;
#33303=ORIENTED_EDGE('',*,*,#24949,.T.) ;
#33304=ORIENTED_EDGE('',*,*,#24947,.F.) ;
#33305=ORIENTED_EDGE('',*,*,#24950,.T.) ;
#33306=ORIENTED_EDGE('',*,*,#24951,.T.) ;
#33307=ORIENTED_EDGE('',*,*,#24952,.T.) ;
#33308=ORIENTED_EDGE('',*,*,#24948,.F.) ;
#33309=ORIENTED_EDGE('',*,*,#24856,.T.) ;
#33310=ORIENTED_EDGE('',*,*,#24945,.F.) ;
#33311=ORIENTED_EDGE('',*,*,#24953,.T.) ;
#33312=ORIENTED_EDGE('',*,*,#24951,.F.) ;
#33313=ORIENTED_EDGE('',*,*,#24954,.T.) ;
#33314=ORIENTED_EDGE('',*,*,#24955,.T.) ;
#33315=ORIENTED_EDGE('',*,*,#24956,.T.) ;
#33316=ORIENTED_EDGE('',*,*,#24955,.F.) ;
#33317=ORIENTED_EDGE('',*,*,#24957,.T.) ;
#33318=ORIENTED_EDGE('',*,*,#24942,.T.) ;
#33319=ORIENTED_EDGE('',*,*,#24958,.T.) ;
#33320=ORIENTED_EDGE('',*,*,#24943,.F.) ;
#33321=ORIENTED_EDGE('',*,*,#24860,.T.) ;
#33322=ORIENTED_EDGE('',*,*,#24940,.F.) ;
#33323=ORIENTED_EDGE('',*,*,#24946,.F.) ;
#33324=ORIENTED_EDGE('',*,*,#24952,.F.) ;
#33325=ORIENTED_EDGE('',*,*,#24944,.F.) ;
#33326=ORIENTED_EDGE('',*,*,#24958,.F.) ;
#33327=ORIENTED_EDGE('',*,*,#24939,.F.) ;
#33328=ORIENTED_EDGE('',*,*,#24957,.F.) ;
#33329=ORIENTED_EDGE('',*,*,#24954,.F.) ;
#33330=ORIENTED_EDGE('',*,*,#24950,.F.) ;
#33331=ORIENTED_EDGE('',*,*,#24959,.T.) ;
#33332=ORIENTED_EDGE('',*,*,#24960,.T.) ;
#33333=ORIENTED_EDGE('',*,*,#24961,.T.) ;
#33334=ORIENTED_EDGE('',*,*,#24962,.F.) ;
#33335=ORIENTED_EDGE('',*,*,#24963,.T.) ;
#33336=ORIENTED_EDGE('',*,*,#24960,.F.) ;
#33337=ORIENTED_EDGE('',*,*,#24964,.T.) ;
#33338=ORIENTED_EDGE('',*,*,#24965,.T.) ;
#33339=ORIENTED_EDGE('',*,*,#24966,.T.) ;
#33340=ORIENTED_EDGE('',*,*,#24965,.F.) ;
#33341=ORIENTED_EDGE('',*,*,#24967,.T.) ;
#33342=ORIENTED_EDGE('',*,*,#24962,.T.) ;
#33343=ORIENTED_EDGE('',*,*,#24966,.F.) ;
#33344=ORIENTED_EDGE('',*,*,#24968,.F.) ;
#33345=ORIENTED_EDGE('',*,*,#24969,.F.) ;
#33346=ORIENTED_EDGE('',*,*,#24970,.T.) ;
#33347=ORIENTED_EDGE('',*,*,#24961,.F.) ;
#33348=ORIENTED_EDGE('',*,*,#24971,.F.) ;
#33349=ORIENTED_EDGE('',*,*,#24972,.F.) ;
#33350=ORIENTED_EDGE('',*,*,#24968,.T.) ;
#33351=ORIENTED_EDGE('',*,*,#24959,.F.) ;
#33352=ORIENTED_EDGE('',*,*,#24967,.F.) ;
#33353=ORIENTED_EDGE('',*,*,#24964,.F.) ;
#33354=ORIENTED_EDGE('',*,*,#24973,.T.) ;
#33355=ORIENTED_EDGE('',*,*,#24974,.T.) ;
#33356=ORIENTED_EDGE('',*,*,#24975,.T.) ;
#33357=ORIENTED_EDGE('',*,*,#24976,.F.) ;
#33358=ORIENTED_EDGE('',*,*,#24977,.T.) ;
#33359=ORIENTED_EDGE('',*,*,#24974,.F.) ;
#33360=ORIENTED_EDGE('',*,*,#24978,.T.) ;
#33361=ORIENTED_EDGE('',*,*,#24979,.T.) ;
#33362=ORIENTED_EDGE('',*,*,#24980,.T.) ;
#33363=ORIENTED_EDGE('',*,*,#24979,.F.) ;
#33364=ORIENTED_EDGE('',*,*,#24981,.T.) ;
#33365=ORIENTED_EDGE('',*,*,#24982,.T.) ;
#33366=ORIENTED_EDGE('',*,*,#24983,.T.) ;
#33367=ORIENTED_EDGE('',*,*,#24982,.F.) ;
#33368=ORIENTED_EDGE('',*,*,#24984,.T.) ;
#33369=ORIENTED_EDGE('',*,*,#24976,.T.) ;
#33370=ORIENTED_EDGE('',*,*,#24983,.F.) ;
#33371=ORIENTED_EDGE('',*,*,#24985,.F.) ;
#33372=ORIENTED_EDGE('',*,*,#24986,.F.) ;
#33373=ORIENTED_EDGE('',*,*,#24987,.T.) ;
#33374=ORIENTED_EDGE('',*,*,#24975,.F.) ;
#33375=ORIENTED_EDGE('',*,*,#24988,.F.) ;
#33376=ORIENTED_EDGE('',*,*,#24989,.F.) ;
#33377=ORIENTED_EDGE('',*,*,#24985,.T.) ;
#33378=ORIENTED_EDGE('',*,*,#24973,.F.) ;
#33379=ORIENTED_EDGE('',*,*,#24984,.F.) ;
#33380=ORIENTED_EDGE('',*,*,#24981,.F.) ;
#33381=ORIENTED_EDGE('',*,*,#24978,.F.) ;
#33382=ORIENTED_EDGE('',*,*,#24990,.T.) ;
#33383=ORIENTED_EDGE('',*,*,#24991,.T.) ;
#33384=ORIENTED_EDGE('',*,*,#24992,.T.) ;
#33385=ORIENTED_EDGE('',*,*,#24993,.F.) ;
#33386=ORIENTED_EDGE('',*,*,#24994,.T.) ;
#33387=ORIENTED_EDGE('',*,*,#24991,.F.) ;
#33388=ORIENTED_EDGE('',*,*,#24995,.T.) ;
#33389=ORIENTED_EDGE('',*,*,#24996,.T.) ;
#33390=ORIENTED_EDGE('',*,*,#24997,.T.) ;
#33391=ORIENTED_EDGE('',*,*,#24996,.F.) ;
#33392=ORIENTED_EDGE('',*,*,#24998,.T.) ;
#33393=ORIENTED_EDGE('',*,*,#24993,.T.) ;
#33394=ORIENTED_EDGE('',*,*,#24997,.F.) ;
#33395=ORIENTED_EDGE('',*,*,#24999,.F.) ;
#33396=ORIENTED_EDGE('',*,*,#25000,.F.) ;
#33397=ORIENTED_EDGE('',*,*,#25001,.T.) ;
#33398=ORIENTED_EDGE('',*,*,#24992,.F.) ;
#33399=ORIENTED_EDGE('',*,*,#25002,.F.) ;
#33400=ORIENTED_EDGE('',*,*,#25003,.F.) ;
#33401=ORIENTED_EDGE('',*,*,#24999,.T.) ;
#33402=ORIENTED_EDGE('',*,*,#24990,.F.) ;
#33403=ORIENTED_EDGE('',*,*,#24998,.F.) ;
#33404=ORIENTED_EDGE('',*,*,#24995,.F.) ;
#33405=ORIENTED_EDGE('',*,*,#25004,.T.) ;
#33406=ORIENTED_EDGE('',*,*,#25005,.T.) ;
#33407=ORIENTED_EDGE('',*,*,#24924,.T.) ;
#33408=ORIENTED_EDGE('',*,*,#25006,.F.) ;
#33409=ORIENTED_EDGE('',*,*,#25007,.T.) ;
#33410=ORIENTED_EDGE('',*,*,#25008,.T.) ;
#33411=ORIENTED_EDGE('',*,*,#24922,.T.) ;
#33412=ORIENTED_EDGE('',*,*,#25005,.F.) ;
#33413=ORIENTED_EDGE('',*,*,#25009,.T.) ;
#33414=ORIENTED_EDGE('',*,*,#25010,.T.) ;
#33415=ORIENTED_EDGE('',*,*,#24919,.T.) ;
#33416=ORIENTED_EDGE('',*,*,#25008,.F.) ;
#33417=ORIENTED_EDGE('',*,*,#24928,.T.) ;
#33418=ORIENTED_EDGE('',*,*,#25011,.T.) ;
#33419=ORIENTED_EDGE('',*,*,#25012,.T.) ;
#33420=ORIENTED_EDGE('',*,*,#25013,.T.) ;
#33421=ORIENTED_EDGE('',*,*,#25014,.T.) ;
#33422=ORIENTED_EDGE('',*,*,#25015,.T.) ;
#33423=ORIENTED_EDGE('',*,*,#25016,.T.) ;
#33424=ORIENTED_EDGE('',*,*,#25010,.F.) ;
#33425=ORIENTED_EDGE('',*,*,#25017,.T.) ;
#33426=ORIENTED_EDGE('',*,*,#25018,.T.) ;
#33427=ORIENTED_EDGE('',*,*,#25019,.T.) ;
#33428=ORIENTED_EDGE('',*,*,#25015,.F.) ;
#33429=ORIENTED_EDGE('',*,*,#25020,.T.) ;
#33430=ORIENTED_EDGE('',*,*,#25021,.T.) ;
#33431=ORIENTED_EDGE('',*,*,#25022,.T.) ;
#33432=ORIENTED_EDGE('',*,*,#25018,.F.) ;
#33433=ORIENTED_EDGE('',*,*,#25023,.T.) ;
#33434=ORIENTED_EDGE('',*,*,#25024,.T.) ;
#33435=ORIENTED_EDGE('',*,*,#25025,.T.) ;
#33436=ORIENTED_EDGE('',*,*,#25021,.F.) ;
#33437=ORIENTED_EDGE('',*,*,#25026,.T.) ;
#33438=ORIENTED_EDGE('',*,*,#25027,.T.) ;
#33439=ORIENTED_EDGE('',*,*,#25028,.T.) ;
#33440=ORIENTED_EDGE('',*,*,#25024,.F.) ;
#33441=ORIENTED_EDGE('',*,*,#25029,.T.) ;
#33442=ORIENTED_EDGE('',*,*,#25030,.T.) ;
#33443=ORIENTED_EDGE('',*,*,#25031,.T.) ;
#33444=ORIENTED_EDGE('',*,*,#25032,.T.) ;
#33445=ORIENTED_EDGE('',*,*,#25033,.T.) ;
#33446=ORIENTED_EDGE('',*,*,#25034,.T.) ;
#33447=ORIENTED_EDGE('',*,*,#25035,.T.) ;
#33448=ORIENTED_EDGE('',*,*,#25027,.F.) ;
#33449=ORIENTED_EDGE('',*,*,#25036,.T.) ;
#33450=ORIENTED_EDGE('',*,*,#25037,.T.) ;
#33451=ORIENTED_EDGE('',*,*,#25038,.T.) ;
#33452=ORIENTED_EDGE('',*,*,#25034,.F.) ;
#33453=ORIENTED_EDGE('',*,*,#25039,.T.) ;
#33454=ORIENTED_EDGE('',*,*,#25037,.F.) ;
#33455=ORIENTED_EDGE('',*,*,#25040,.T.) ;
#33456=ORIENTED_EDGE('',*,*,#25030,.F.) ;
#33457=ORIENTED_EDGE('',*,*,#24936,.T.) ;
#33458=ORIENTED_EDGE('',*,*,#25041,.T.) ;
#33459=ORIENTED_EDGE('',*,*,#25042,.T.) ;
#33460=ORIENTED_EDGE('',*,*,#25043,.T.) ;
#33461=ORIENTED_EDGE('',*,*,#25044,.T.) ;
#33462=ORIENTED_EDGE('',*,*,#25041,.F.) ;
#33463=ORIENTED_EDGE('',*,*,#24938,.T.) ;
#33464=ORIENTED_EDGE('',*,*,#25032,.F.) ;
#33465=ORIENTED_EDGE('',*,*,#24934,.T.) ;
#33466=ORIENTED_EDGE('',*,*,#25043,.F.) ;
#33467=ORIENTED_EDGE('',*,*,#25045,.T.) ;
#33468=ORIENTED_EDGE('',*,*,#25046,.T.) ;
#33469=ORIENTED_EDGE('',*,*,#24932,.T.) ;
#33470=ORIENTED_EDGE('',*,*,#25046,.F.) ;
#33471=ORIENTED_EDGE('',*,*,#25047,.T.) ;
#33472=ORIENTED_EDGE('',*,*,#25048,.T.) ;
#33473=ORIENTED_EDGE('',*,*,#25011,.F.) ;
#33474=ORIENTED_EDGE('',*,*,#24930,.T.) ;
#33475=ORIENTED_EDGE('',*,*,#25048,.F.) ;
#33476=ORIENTED_EDGE('',*,*,#25049,.T.) ;
#33477=ORIENTED_EDGE('',*,*,#24926,.T.) ;
#33478=ORIENTED_EDGE('',*,*,#25013,.F.) ;
#33479=ORIENTED_EDGE('',*,*,#25050,.T.) ;
#33480=ORIENTED_EDGE('',*,*,#25006,.T.) ;
#33481=ORIENTED_EDGE('',*,*,#24911,.F.) ;
#33482=ORIENTED_EDGE('',*,*,#25051,.F.) ;
#33483=ORIENTED_EDGE('',*,*,#25019,.F.) ;
#33484=ORIENTED_EDGE('',*,*,#25052,.T.) ;
#33485=ORIENTED_EDGE('',*,*,#24909,.F.) ;
#33486=ORIENTED_EDGE('',*,*,#25052,.F.) ;
#33487=ORIENTED_EDGE('',*,*,#25022,.F.) ;
#33488=ORIENTED_EDGE('',*,*,#25053,.T.) ;
#33489=ORIENTED_EDGE('',*,*,#24907,.F.) ;
#33490=ORIENTED_EDGE('',*,*,#25053,.F.) ;
#33491=ORIENTED_EDGE('',*,*,#25025,.F.) ;
#33492=ORIENTED_EDGE('',*,*,#25054,.T.) ;
#33493=ORIENTED_EDGE('',*,*,#24891,.F.) ;
#33494=ORIENTED_EDGE('',*,*,#25054,.F.) ;
#33495=ORIENTED_EDGE('',*,*,#25028,.F.) ;
#33496=ORIENTED_EDGE('',*,*,#25055,.T.) ;
#33497=ORIENTED_EDGE('',*,*,#24906,.F.) ;
#33498=ORIENTED_EDGE('',*,*,#25055,.F.) ;
#33499=ORIENTED_EDGE('',*,*,#25035,.F.) ;
#33500=ORIENTED_EDGE('',*,*,#25056,.T.) ;
#33501=ORIENTED_EDGE('',*,*,#24904,.F.) ;
#33502=ORIENTED_EDGE('',*,*,#25056,.F.) ;
#33503=ORIENTED_EDGE('',*,*,#25038,.F.) ;
#33504=ORIENTED_EDGE('',*,*,#25057,.T.) ;
#33505=ORIENTED_EDGE('',*,*,#24902,.F.) ;
#33506=ORIENTED_EDGE('',*,*,#25057,.F.) ;
#33507=ORIENTED_EDGE('',*,*,#25039,.F.) ;
#33508=ORIENTED_EDGE('',*,*,#25058,.T.) ;
#33509=ORIENTED_EDGE('',*,*,#24901,.F.) ;
#33510=ORIENTED_EDGE('',*,*,#25058,.F.) ;
#33511=ORIENTED_EDGE('',*,*,#25029,.F.) ;
#33512=ORIENTED_EDGE('',*,*,#24937,.T.) ;
#33513=ORIENTED_EDGE('',*,*,#25059,.F.) ;
#33514=ORIENTED_EDGE('',*,*,#25060,.F.) ;
#33515=ORIENTED_EDGE('',*,*,#25061,.F.) ;
#33516=ORIENTED_EDGE('',*,*,#25062,.F.) ;
#33517=ORIENTED_EDGE('',*,*,#25063,.F.) ;
#33518=ORIENTED_EDGE('',*,*,#25064,.F.) ;
#33519=ORIENTED_EDGE('',*,*,#25065,.F.) ;
#33520=ORIENTED_EDGE('',*,*,#25066,.F.) ;
#33521=ORIENTED_EDGE('',*,*,#25067,.F.) ;
#33522=ORIENTED_EDGE('',*,*,#25068,.F.) ;
#33523=ORIENTED_EDGE('',*,*,#25069,.F.) ;
#33524=ORIENTED_EDGE('',*,*,#25070,.F.) ;
#33525=ORIENTED_EDGE('',*,*,#25071,.F.) ;
#33526=ORIENTED_EDGE('',*,*,#25072,.F.) ;
#33527=ORIENTED_EDGE('',*,*,#25073,.F.) ;
#33528=ORIENTED_EDGE('',*,*,#25074,.F.) ;
#33529=ORIENTED_EDGE('',*,*,#25075,.F.) ;
#33530=ORIENTED_EDGE('',*,*,#25076,.F.) ;
#33531=ORIENTED_EDGE('',*,*,#25077,.F.) ;
#33532=ORIENTED_EDGE('',*,*,#25078,.F.) ;
#33533=ORIENTED_EDGE('',*,*,#25079,.F.) ;
#33534=ORIENTED_EDGE('',*,*,#25080,.F.) ;
#33535=ORIENTED_EDGE('',*,*,#25081,.F.) ;
#33536=ORIENTED_EDGE('',*,*,#25082,.F.) ;
#33537=ORIENTED_EDGE('',*,*,#25083,.F.) ;
#33538=ORIENTED_EDGE('',*,*,#25084,.F.) ;
#33539=ORIENTED_EDGE('',*,*,#25085,.F.) ;
#33540=ORIENTED_EDGE('',*,*,#25086,.F.) ;
#33541=ORIENTED_EDGE('',*,*,#25087,.F.) ;
#33542=ORIENTED_EDGE('',*,*,#25088,.F.) ;
#33543=ORIENTED_EDGE('',*,*,#25089,.F.) ;
#33544=ORIENTED_EDGE('',*,*,#25090,.F.) ;
#33545=ORIENTED_EDGE('',*,*,#25091,.F.) ;
#33546=ORIENTED_EDGE('',*,*,#25092,.F.) ;
#33547=ORIENTED_EDGE('',*,*,#25093,.F.) ;
#33548=ORIENTED_EDGE('',*,*,#25094,.F.) ;
#33549=ORIENTED_EDGE('',*,*,#25095,.F.) ;
#33550=ORIENTED_EDGE('',*,*,#25096,.F.) ;
#33551=ORIENTED_EDGE('',*,*,#25097,.F.) ;
#33552=ORIENTED_EDGE('',*,*,#25098,.F.) ;
#33553=ORIENTED_EDGE('',*,*,#25099,.F.) ;
#33554=ORIENTED_EDGE('',*,*,#25100,.F.) ;
#33555=ORIENTED_EDGE('',*,*,#25101,.F.) ;
#33556=ORIENTED_EDGE('',*,*,#25102,.F.) ;
#33557=ORIENTED_EDGE('',*,*,#25103,.F.) ;
#33558=ORIENTED_EDGE('',*,*,#25104,.F.) ;
#33559=ORIENTED_EDGE('',*,*,#25105,.F.) ;
#33560=ORIENTED_EDGE('',*,*,#25106,.F.) ;
#33561=ORIENTED_EDGE('',*,*,#25107,.F.) ;
#33562=ORIENTED_EDGE('',*,*,#25108,.F.) ;
#33563=ORIENTED_EDGE('',*,*,#25109,.F.) ;
#33564=ORIENTED_EDGE('',*,*,#25110,.F.) ;
#33565=ORIENTED_EDGE('',*,*,#25111,.F.) ;
#33566=ORIENTED_EDGE('',*,*,#25112,.F.) ;
#33567=ORIENTED_EDGE('',*,*,#25113,.F.) ;
#33568=ORIENTED_EDGE('',*,*,#25114,.F.) ;
#33569=ORIENTED_EDGE('',*,*,#25115,.F.) ;
#33570=ORIENTED_EDGE('',*,*,#25116,.F.) ;
#33571=ORIENTED_EDGE('',*,*,#25117,.F.) ;
#33572=ORIENTED_EDGE('',*,*,#25118,.F.) ;
#33573=ORIENTED_EDGE('',*,*,#25119,.F.) ;
#33574=ORIENTED_EDGE('',*,*,#25120,.F.) ;
#33575=ORIENTED_EDGE('',*,*,#25121,.F.) ;
#33576=ORIENTED_EDGE('',*,*,#25122,.F.) ;
#33577=ORIENTED_EDGE('',*,*,#25123,.F.) ;
#33578=ORIENTED_EDGE('',*,*,#25124,.F.) ;
#33579=ORIENTED_EDGE('',*,*,#25125,.F.) ;
#33580=ORIENTED_EDGE('',*,*,#25126,.F.) ;
#33581=ORIENTED_EDGE('',*,*,#25127,.F.) ;
#33582=ORIENTED_EDGE('',*,*,#25128,.T.) ;
#33583=ORIENTED_EDGE('',*,*,#25129,.F.) ;
#33584=ORIENTED_EDGE('',*,*,#25130,.F.) ;
#33585=ORIENTED_EDGE('',*,*,#25131,.F.) ;
#33586=ORIENTED_EDGE('',*,*,#25132,.T.) ;
#33587=ORIENTED_EDGE('',*,*,#25133,.F.) ;
#33588=ORIENTED_EDGE('',*,*,#25134,.F.) ;
#33589=ORIENTED_EDGE('',*,*,#25135,.F.) ;
#33590=ORIENTED_EDGE('',*,*,#25136,.F.) ;
#33591=ORIENTED_EDGE('',*,*,#25137,.F.) ;
#33592=ORIENTED_EDGE('',*,*,#25138,.F.) ;
#33593=ORIENTED_EDGE('',*,*,#25139,.F.) ;
#33594=ORIENTED_EDGE('',*,*,#25140,.F.) ;
#33595=ORIENTED_EDGE('',*,*,#25141,.F.) ;
#33596=ORIENTED_EDGE('',*,*,#25142,.F.) ;
#33597=ORIENTED_EDGE('',*,*,#25143,.F.) ;
#33598=ORIENTED_EDGE('',*,*,#25144,.F.) ;
#33599=ORIENTED_EDGE('',*,*,#25145,.F.) ;
#33600=ORIENTED_EDGE('',*,*,#25146,.F.) ;
#33601=ORIENTED_EDGE('',*,*,#25147,.F.) ;
#33602=ORIENTED_EDGE('',*,*,#25148,.F.) ;
#33603=ORIENTED_EDGE('',*,*,#25149,.F.) ;
#33604=ORIENTED_EDGE('',*,*,#25150,.F.) ;
#33605=ORIENTED_EDGE('',*,*,#25151,.F.) ;
#33606=ORIENTED_EDGE('',*,*,#25152,.F.) ;
#33607=ORIENTED_EDGE('',*,*,#25153,.F.) ;
#33608=ORIENTED_EDGE('',*,*,#25154,.F.) ;
#33609=ORIENTED_EDGE('',*,*,#25155,.F.) ;
#33610=ORIENTED_EDGE('',*,*,#25156,.F.) ;
#33611=ORIENTED_EDGE('',*,*,#25157,.F.) ;
#33612=ORIENTED_EDGE('',*,*,#25158,.F.) ;
#33613=ORIENTED_EDGE('',*,*,#25159,.F.) ;
#33614=ORIENTED_EDGE('',*,*,#25160,.F.) ;
#33615=ORIENTED_EDGE('',*,*,#25161,.F.) ;
#33616=ORIENTED_EDGE('',*,*,#25162,.F.) ;
#33617=ORIENTED_EDGE('',*,*,#25163,.F.) ;
#33618=ORIENTED_EDGE('',*,*,#25164,.F.) ;
#33619=ORIENTED_EDGE('',*,*,#25165,.F.) ;
#33620=ORIENTED_EDGE('',*,*,#25166,.F.) ;
#33621=ORIENTED_EDGE('',*,*,#25167,.F.) ;
#33622=ORIENTED_EDGE('',*,*,#25168,.F.) ;
#33623=ORIENTED_EDGE('',*,*,#25169,.F.) ;
#33624=ORIENTED_EDGE('',*,*,#25170,.F.) ;
#33625=ORIENTED_EDGE('',*,*,#25171,.F.) ;
#33626=ORIENTED_EDGE('',*,*,#25172,.T.) ;
#33627=ORIENTED_EDGE('',*,*,#25173,.F.) ;
#33628=ORIENTED_EDGE('',*,*,#25174,.F.) ;
#33629=ORIENTED_EDGE('',*,*,#25175,.F.) ;
#33630=ORIENTED_EDGE('',*,*,#25176,.T.) ;
#33631=ORIENTED_EDGE('',*,*,#25177,.F.) ;
#33632=ORIENTED_EDGE('',*,*,#25178,.F.) ;
#33633=ORIENTED_EDGE('',*,*,#25179,.F.) ;
#33634=ORIENTED_EDGE('',*,*,#25180,.F.) ;
#33635=ORIENTED_EDGE('',*,*,#25181,.F.) ;
#33636=ORIENTED_EDGE('',*,*,#25182,.F.) ;
#33637=ORIENTED_EDGE('',*,*,#25183,.F.) ;
#33638=ORIENTED_EDGE('',*,*,#25184,.F.) ;
#33639=ORIENTED_EDGE('',*,*,#25185,.F.) ;
#33640=ORIENTED_EDGE('',*,*,#25186,.F.) ;
#33641=ORIENTED_EDGE('',*,*,#25187,.T.) ;
#33642=ORIENTED_EDGE('',*,*,#25188,.F.) ;
#33643=ORIENTED_EDGE('',*,*,#25189,.F.) ;
#33644=ORIENTED_EDGE('',*,*,#25190,.F.) ;
#33645=ORIENTED_EDGE('',*,*,#25191,.F.) ;
#33646=ORIENTED_EDGE('',*,*,#25192,.F.) ;
#33647=ORIENTED_EDGE('',*,*,#25193,.F.) ;
#33648=ORIENTED_EDGE('',*,*,#25194,.F.) ;
#33649=ORIENTED_EDGE('',*,*,#25195,.F.) ;
#33650=ORIENTED_EDGE('',*,*,#25196,.F.) ;
#33651=ORIENTED_EDGE('',*,*,#25197,.F.) ;
#33652=ORIENTED_EDGE('',*,*,#25198,.T.) ;
#33653=ORIENTED_EDGE('',*,*,#25199,.F.) ;
#33654=ORIENTED_EDGE('',*,*,#25200,.F.) ;
#33655=ORIENTED_EDGE('',*,*,#25201,.F.) ;
#33656=ORIENTED_EDGE('',*,*,#25202,.F.) ;
#33657=ORIENTED_EDGE('',*,*,#25203,.F.) ;
#33658=ORIENTED_EDGE('',*,*,#25204,.F.) ;
#33659=ORIENTED_EDGE('',*,*,#25205,.T.) ;
#33660=ORIENTED_EDGE('',*,*,#25206,.F.) ;
#33661=ORIENTED_EDGE('',*,*,#25207,.F.) ;
#33662=ORIENTED_EDGE('',*,*,#25208,.F.) ;
#33663=ORIENTED_EDGE('',*,*,#25209,.F.) ;
#33664=ORIENTED_EDGE('',*,*,#25210,.F.) ;
#33665=ORIENTED_EDGE('',*,*,#25211,.F.) ;
#33666=ORIENTED_EDGE('',*,*,#25212,.F.) ;
#33667=ORIENTED_EDGE('',*,*,#25213,.F.) ;
#33668=ORIENTED_EDGE('',*,*,#25214,.F.) ;
#33669=ORIENTED_EDGE('',*,*,#25215,.T.) ;
#33670=ORIENTED_EDGE('',*,*,#25216,.F.) ;
#33671=ORIENTED_EDGE('',*,*,#25217,.F.) ;
#33672=ORIENTED_EDGE('',*,*,#25218,.F.) ;
#33673=ORIENTED_EDGE('',*,*,#25219,.F.) ;
#33674=ORIENTED_EDGE('',*,*,#25220,.F.) ;
#33675=ORIENTED_EDGE('',*,*,#25221,.F.) ;
#33676=ORIENTED_EDGE('',*,*,#25222,.F.) ;
#33677=ORIENTED_EDGE('',*,*,#25223,.F.) ;
#33678=ORIENTED_EDGE('',*,*,#25224,.F.) ;
#33679=ORIENTED_EDGE('',*,*,#25225,.F.) ;
#33680=ORIENTED_EDGE('',*,*,#25226,.F.) ;
#33681=ORIENTED_EDGE('',*,*,#25227,.F.) ;
#33682=ORIENTED_EDGE('',*,*,#25228,.F.) ;
#33683=ORIENTED_EDGE('',*,*,#25229,.F.) ;
#33684=ORIENTED_EDGE('',*,*,#25230,.F.) ;
#33685=ORIENTED_EDGE('',*,*,#25231,.F.) ;
#33686=ORIENTED_EDGE('',*,*,#25232,.F.) ;
#33687=ORIENTED_EDGE('',*,*,#25233,.F.) ;
#33688=ORIENTED_EDGE('',*,*,#25234,.F.) ;
#33689=ORIENTED_EDGE('',*,*,#25235,.F.) ;
#33690=ORIENTED_EDGE('',*,*,#25236,.F.) ;
#33691=ORIENTED_EDGE('',*,*,#25237,.F.) ;
#33692=ORIENTED_EDGE('',*,*,#25238,.F.) ;
#33693=ORIENTED_EDGE('',*,*,#25239,.F.) ;
#33694=ORIENTED_EDGE('',*,*,#25240,.F.) ;
#33695=ORIENTED_EDGE('',*,*,#25241,.F.) ;
#33696=ORIENTED_EDGE('',*,*,#25242,.F.) ;
#33697=ORIENTED_EDGE('',*,*,#25243,.F.) ;
#33698=ORIENTED_EDGE('',*,*,#25244,.F.) ;
#33699=ORIENTED_EDGE('',*,*,#25245,.F.) ;
#33700=ORIENTED_EDGE('',*,*,#25042,.F.) ;
#33701=ORIENTED_EDGE('',*,*,#25044,.F.) ;
#33702=ORIENTED_EDGE('',*,*,#25031,.F.) ;
#33703=ORIENTED_EDGE('',*,*,#25040,.F.) ;
#33704=ORIENTED_EDGE('',*,*,#25036,.F.) ;
#33705=ORIENTED_EDGE('',*,*,#25033,.F.) ;
#33706=ORIENTED_EDGE('',*,*,#25026,.F.) ;
#33707=ORIENTED_EDGE('',*,*,#25023,.F.) ;
#33708=ORIENTED_EDGE('',*,*,#25020,.F.) ;
#33709=ORIENTED_EDGE('',*,*,#25017,.F.) ;
#33710=ORIENTED_EDGE('',*,*,#25014,.F.) ;
#33711=ORIENTED_EDGE('',*,*,#25009,.F.) ;
#33712=ORIENTED_EDGE('',*,*,#25007,.F.) ;
#33713=ORIENTED_EDGE('',*,*,#25004,.F.) ;
#33714=ORIENTED_EDGE('',*,*,#25050,.F.) ;
#33715=ORIENTED_EDGE('',*,*,#25012,.F.) ;
#33716=ORIENTED_EDGE('',*,*,#25049,.F.) ;
#33717=ORIENTED_EDGE('',*,*,#25047,.F.) ;
#33718=ORIENTED_EDGE('',*,*,#25045,.F.) ;
#33719=ORIENTED_EDGE('',*,*,#25108,.T.) ;
#33720=ORIENTED_EDGE('',*,*,#25246,.T.) ;
#33721=ORIENTED_EDGE('',*,*,#24972,.T.) ;
#33722=ORIENTED_EDGE('',*,*,#25247,.T.) ;
#33723=ORIENTED_EDGE('',*,*,#25110,.T.) ;
#33724=ORIENTED_EDGE('',*,*,#25248,.T.) ;
#33725=ORIENTED_EDGE('',*,*,#24969,.T.) ;
#33726=ORIENTED_EDGE('',*,*,#25246,.F.) ;
#33727=ORIENTED_EDGE('',*,*,#25249,.T.) ;
#33728=ORIENTED_EDGE('',*,*,#25248,.F.) ;
#33729=ORIENTED_EDGE('',*,*,#25109,.T.) ;
#33730=ORIENTED_EDGE('',*,*,#25247,.F.) ;
#33731=ORIENTED_EDGE('',*,*,#24963,.F.) ;
#33732=ORIENTED_EDGE('',*,*,#24970,.F.) ;
#33733=ORIENTED_EDGE('',*,*,#25249,.F.) ;
#33734=ORIENTED_EDGE('',*,*,#24971,.T.) ;
#33735=ORIENTED_EDGE('',*,*,#25242,.T.) ;
#33736=ORIENTED_EDGE('',*,*,#25250,.T.) ;
#33737=ORIENTED_EDGE('',*,*,#24989,.T.) ;
#33738=ORIENTED_EDGE('',*,*,#25251,.T.) ;
#33739=ORIENTED_EDGE('',*,*,#25245,.T.) ;
#33740=ORIENTED_EDGE('',*,*,#25252,.T.) ;
#33741=ORIENTED_EDGE('',*,*,#24986,.T.) ;
#33742=ORIENTED_EDGE('',*,*,#25250,.F.) ;
#33743=ORIENTED_EDGE('',*,*,#25253,.T.) ;
#33744=ORIENTED_EDGE('',*,*,#25252,.F.) ;
#33745=ORIENTED_EDGE('',*,*,#25244,.T.) ;
#33746=ORIENTED_EDGE('',*,*,#25254,.T.) ;
#33747=ORIENTED_EDGE('',*,*,#25243,.T.) ;
#33748=ORIENTED_EDGE('',*,*,#25251,.F.) ;
#33749=ORIENTED_EDGE('',*,*,#25255,.T.) ;
#33750=ORIENTED_EDGE('',*,*,#25254,.F.) ;
#33751=ORIENTED_EDGE('',*,*,#24977,.F.) ;
#33752=ORIENTED_EDGE('',*,*,#25256,.F.) ;
#33753=ORIENTED_EDGE('',*,*,#25255,.F.) ;
#33754=ORIENTED_EDGE('',*,*,#24988,.T.) ;
#33755=ORIENTED_EDGE('',*,*,#25111,.T.) ;
#33756=ORIENTED_EDGE('',*,*,#25257,.T.) ;
#33757=ORIENTED_EDGE('',*,*,#25003,.T.) ;
#33758=ORIENTED_EDGE('',*,*,#25258,.T.) ;
#33759=ORIENTED_EDGE('',*,*,#25000,.T.) ;
#33760=ORIENTED_EDGE('',*,*,#25257,.F.) ;
#33761=ORIENTED_EDGE('',*,*,#25113,.T.) ;
#33762=ORIENTED_EDGE('',*,*,#25259,.T.) ;
#33763=ORIENTED_EDGE('',*,*,#25112,.T.) ;
#33764=ORIENTED_EDGE('',*,*,#25258,.F.) ;
#33765=ORIENTED_EDGE('',*,*,#25260,.T.) ;
#33766=ORIENTED_EDGE('',*,*,#25259,.F.) ;
#33767=ORIENTED_EDGE('',*,*,#24994,.F.) ;
#33768=ORIENTED_EDGE('',*,*,#25001,.F.) ;
#33769=ORIENTED_EDGE('',*,*,#25260,.F.) ;
#33770=ORIENTED_EDGE('',*,*,#25002,.T.) ;
#33771=ORIENTED_EDGE('',*,*,#24980,.F.) ;
#33772=ORIENTED_EDGE('',*,*,#24987,.F.) ;
#33773=ORIENTED_EDGE('',*,*,#25253,.F.) ;
#33774=ORIENTED_EDGE('',*,*,#25256,.T.) ;
#33775=ORIENTED_EDGE('',*,*,#24838,.F.) ;
#33776=ORIENTED_EDGE('',*,*,#24854,.F.) ;
#33777=ORIENTED_EDGE('',*,*,#24949,.F.) ;
#33778=ORIENTED_EDGE('',*,*,#25261,.T.) ;
#33779=ORIENTED_EDGE('',*,*,#24830,.F.) ;
#33780=ORIENTED_EDGE('',*,*,#25261,.F.) ;
#33781=ORIENTED_EDGE('',*,*,#24953,.F.) ;
#33782=ORIENTED_EDGE('',*,*,#25262,.T.) ;
#33783=ORIENTED_EDGE('',*,*,#24850,.F.) ;
#33784=ORIENTED_EDGE('',*,*,#25262,.F.) ;
#33785=ORIENTED_EDGE('',*,*,#24956,.F.) ;
#33786=ORIENTED_EDGE('',*,*,#25263,.T.) ;
#33787=ORIENTED_EDGE('',*,*,#24847,.F.) ;
#33788=ORIENTED_EDGE('',*,*,#25263,.F.) ;
#33789=ORIENTED_EDGE('',*,*,#24941,.F.) ;
#33790=ORIENTED_EDGE('',*,*,#24859,.T.) ;
#33791=ORIENTED_EDGE('',*,*,#24913,.F.) ;
#33792=ORIENTED_EDGE('',*,*,#24920,.F.) ;
#33793=ORIENTED_EDGE('',*,*,#25016,.F.) ;
#33794=ORIENTED_EDGE('',*,*,#25051,.T.) ;
#33795=ORIENTED_EDGE('',*,*,#25264,.T.) ;
#33796=ORIENTED_EDGE('',*,*,#25265,.T.) ;
#33797=ORIENTED_EDGE('',*,*,#25266,.T.) ;
#33798=ORIENTED_EDGE('',*,*,#25265,.F.) ;
#33799=ORIENTED_EDGE('',*,*,#25267,.T.) ;
#33800=ORIENTED_EDGE('',*,*,#25268,.F.) ;
#33801=ORIENTED_EDGE('',*,*,#25266,.F.) ;
#33802=ORIENTED_EDGE('',*,*,#25264,.F.) ;
#33803=ORIENTED_EDGE('',*,*,#25269,.T.) ;
#33804=ORIENTED_EDGE('',*,*,#25270,.F.) ;
#33805=ORIENTED_EDGE('',*,*,#25269,.F.) ;
#33806=ORIENTED_EDGE('',*,*,#25267,.F.) ;
#33807=ORIENTED_EDGE('',*,*,#25271,.T.) ;
#33808=ORIENTED_EDGE('',*,*,#25272,.T.) ;
#33809=ORIENTED_EDGE('',*,*,#25268,.T.) ;
#33810=ORIENTED_EDGE('',*,*,#25272,.F.) ;
#33811=ORIENTED_EDGE('',*,*,#25273,.F.) ;
#33812=ORIENTED_EDGE('',*,*,#25274,.T.) ;
#33813=ORIENTED_EDGE('',*,*,#25271,.F.) ;
#33814=ORIENTED_EDGE('',*,*,#25274,.F.) ;
#33815=ORIENTED_EDGE('',*,*,#25275,.T.) ;
#33816=ORIENTED_EDGE('',*,*,#25276,.T.) ;
#33817=ORIENTED_EDGE('',*,*,#25273,.T.) ;
#33818=ORIENTED_EDGE('',*,*,#25276,.F.) ;
#33819=ORIENTED_EDGE('',*,*,#25277,.F.) ;
#33820=ORIENTED_EDGE('',*,*,#25278,.F.) ;
#33821=ORIENTED_EDGE('',*,*,#25279,.F.) ;
#33822=ORIENTED_EDGE('',*,*,#25280,.F.) ;
#33823=ORIENTED_EDGE('',*,*,#25281,.T.) ;
#33824=ORIENTED_EDGE('',*,*,#25282,.T.) ;
#33825=ORIENTED_EDGE('',*,*,#25283,.F.) ;
#33826=ORIENTED_EDGE('',*,*,#25284,.F.) ;
#33827=ORIENTED_EDGE('',*,*,#25285,.F.) ;
#33828=ORIENTED_EDGE('',*,*,#25286,.F.) ;
#33829=ORIENTED_EDGE('',*,*,#25287,.F.) ;
#33830=ORIENTED_EDGE('',*,*,#25288,.F.) ;
#33831=ORIENTED_EDGE('',*,*,#25289,.F.) ;
#33832=ORIENTED_EDGE('',*,*,#25290,.F.) ;
#33833=ORIENTED_EDGE('',*,*,#25291,.T.) ;
#33834=ORIENTED_EDGE('',*,*,#25292,.F.) ;
#33835=ORIENTED_EDGE('',*,*,#25293,.T.) ;
#33836=ORIENTED_EDGE('',*,*,#25294,.F.) ;
#33837=ORIENTED_EDGE('',*,*,#25295,.F.) ;
#33838=ORIENTED_EDGE('',*,*,#25296,.F.) ;
#33839=ORIENTED_EDGE('',*,*,#25297,.T.) ;
#33840=ORIENTED_EDGE('',*,*,#25298,.F.) ;
#33841=ORIENTED_EDGE('',*,*,#25299,.T.) ;
#33842=ORIENTED_EDGE('',*,*,#25300,.F.) ;
#33843=ORIENTED_EDGE('',*,*,#25301,.F.) ;
#33844=ORIENTED_EDGE('',*,*,#25302,.F.) ;
#33845=ORIENTED_EDGE('',*,*,#25303,.F.) ;
#33846=ORIENTED_EDGE('',*,*,#25304,.F.) ;
#33847=ORIENTED_EDGE('',*,*,#25305,.F.) ;
#33848=ORIENTED_EDGE('',*,*,#25306,.F.) ;
#33849=ORIENTED_EDGE('',*,*,#25307,.F.) ;
#33850=ORIENTED_EDGE('',*,*,#25308,.F.) ;
#33851=ORIENTED_EDGE('',*,*,#25309,.F.) ;
#33852=ORIENTED_EDGE('',*,*,#25310,.F.) ;
#33853=ORIENTED_EDGE('',*,*,#25311,.F.) ;
#33854=ORIENTED_EDGE('',*,*,#25312,.F.) ;
#33855=ORIENTED_EDGE('',*,*,#25313,.F.) ;
#33856=ORIENTED_EDGE('',*,*,#25314,.F.) ;
#33857=ORIENTED_EDGE('',*,*,#25315,.F.) ;
#33858=ORIENTED_EDGE('',*,*,#25316,.F.) ;
#33859=ORIENTED_EDGE('',*,*,#25317,.F.) ;
#33860=ORIENTED_EDGE('',*,*,#25318,.F.) ;
#33861=ORIENTED_EDGE('',*,*,#25319,.F.) ;
#33862=ORIENTED_EDGE('',*,*,#25320,.F.) ;
#33863=ORIENTED_EDGE('',*,*,#25321,.F.) ;
#33864=ORIENTED_EDGE('',*,*,#25322,.F.) ;
#33865=ORIENTED_EDGE('',*,*,#25323,.F.) ;
#33866=ORIENTED_EDGE('',*,*,#25324,.F.) ;
#33867=ORIENTED_EDGE('',*,*,#25325,.F.) ;
#33868=ORIENTED_EDGE('',*,*,#25326,.F.) ;
#33869=ORIENTED_EDGE('',*,*,#25327,.T.) ;
#33870=ORIENTED_EDGE('',*,*,#25328,.F.) ;
#33871=ORIENTED_EDGE('',*,*,#25329,.F.) ;
#33872=ORIENTED_EDGE('',*,*,#25330,.F.) ;
#33873=ORIENTED_EDGE('',*,*,#25331,.F.) ;
#33874=ORIENTED_EDGE('',*,*,#25332,.F.) ;
#33875=ORIENTED_EDGE('',*,*,#25333,.F.) ;
#33876=ORIENTED_EDGE('',*,*,#25334,.F.) ;
#33877=ORIENTED_EDGE('',*,*,#25335,.F.) ;
#33878=ORIENTED_EDGE('',*,*,#25336,.F.) ;
#33879=ORIENTED_EDGE('',*,*,#25337,.F.) ;
#33880=ORIENTED_EDGE('',*,*,#25338,.F.) ;
#33881=ORIENTED_EDGE('',*,*,#25339,.F.) ;
#33882=ORIENTED_EDGE('',*,*,#25340,.F.) ;
#33883=ORIENTED_EDGE('',*,*,#25341,.F.) ;
#33884=ORIENTED_EDGE('',*,*,#25342,.F.) ;
#33885=ORIENTED_EDGE('',*,*,#25343,.F.) ;
#33886=ORIENTED_EDGE('',*,*,#25344,.F.) ;
#33887=ORIENTED_EDGE('',*,*,#25345,.F.) ;
#33888=ORIENTED_EDGE('',*,*,#25346,.F.) ;
#33889=ORIENTED_EDGE('',*,*,#25347,.F.) ;
#33890=ORIENTED_EDGE('',*,*,#25348,.F.) ;
#33891=ORIENTED_EDGE('',*,*,#25349,.F.) ;
#33892=ORIENTED_EDGE('',*,*,#25350,.T.) ;
#33893=ORIENTED_EDGE('',*,*,#25351,.F.) ;
#33894=ORIENTED_EDGE('',*,*,#25352,.F.) ;
#33895=ORIENTED_EDGE('',*,*,#25353,.F.) ;
#33896=ORIENTED_EDGE('',*,*,#25354,.F.) ;
#33897=ORIENTED_EDGE('',*,*,#25355,.F.) ;
#33898=ORIENTED_EDGE('',*,*,#25356,.F.) ;
#33899=ORIENTED_EDGE('',*,*,#25357,.F.) ;
#33900=ORIENTED_EDGE('',*,*,#25358,.F.) ;
#33901=ORIENTED_EDGE('',*,*,#25359,.F.) ;
#33902=ORIENTED_EDGE('',*,*,#25360,.F.) ;
#33903=ORIENTED_EDGE('',*,*,#25361,.F.) ;
#33904=ORIENTED_EDGE('',*,*,#25362,.F.) ;
#33905=ORIENTED_EDGE('',*,*,#25363,.F.) ;
#33906=ORIENTED_EDGE('',*,*,#25364,.F.) ;
#33907=ORIENTED_EDGE('',*,*,#25365,.F.) ;
#33908=ORIENTED_EDGE('',*,*,#25366,.T.) ;
#33909=ORIENTED_EDGE('',*,*,#25367,.T.) ;
#33910=ORIENTED_EDGE('',*,*,#25368,.T.) ;
#33911=ORIENTED_EDGE('',*,*,#25369,.F.) ;
#33912=ORIENTED_EDGE('',*,*,#25370,.F.) ;
#33913=ORIENTED_EDGE('',*,*,#25371,.F.) ;
#33914=ORIENTED_EDGE('',*,*,#25372,.T.) ;
#33915=ORIENTED_EDGE('',*,*,#25373,.F.) ;
#33916=ORIENTED_EDGE('',*,*,#25374,.F.) ;
#33917=ORIENTED_EDGE('',*,*,#25375,.F.) ;
#33918=ORIENTED_EDGE('',*,*,#25376,.T.) ;
#33919=ORIENTED_EDGE('',*,*,#25377,.F.) ;
#33920=ORIENTED_EDGE('',*,*,#25378,.T.) ;
#33921=ORIENTED_EDGE('',*,*,#25379,.T.) ;
#33922=ORIENTED_EDGE('',*,*,#25380,.T.) ;
#33923=ORIENTED_EDGE('',*,*,#25381,.F.) ;
#33924=ORIENTED_EDGE('',*,*,#25382,.F.) ;
#33925=ORIENTED_EDGE('',*,*,#25383,.F.) ;
#33926=ORIENTED_EDGE('',*,*,#25384,.F.) ;
#33927=ORIENTED_EDGE('',*,*,#25385,.F.) ;
#33928=ORIENTED_EDGE('',*,*,#25386,.F.) ;
#33929=ORIENTED_EDGE('',*,*,#25387,.F.) ;
#33930=ORIENTED_EDGE('',*,*,#25388,.F.) ;
#33931=ORIENTED_EDGE('',*,*,#25389,.F.) ;
#33932=ORIENTED_EDGE('',*,*,#25390,.T.) ;
#33933=ORIENTED_EDGE('',*,*,#25391,.T.) ;
#33934=ORIENTED_EDGE('',*,*,#25392,.T.) ;
#33935=ORIENTED_EDGE('',*,*,#25393,.F.) ;
#33936=ORIENTED_EDGE('',*,*,#25394,.F.) ;
#33937=ORIENTED_EDGE('',*,*,#25395,.F.) ;
#33938=ORIENTED_EDGE('',*,*,#25396,.F.) ;
#33939=ORIENTED_EDGE('',*,*,#25397,.F.) ;
#33940=ORIENTED_EDGE('',*,*,#25398,.F.) ;
#33941=ORIENTED_EDGE('',*,*,#25399,.F.) ;
#33942=ORIENTED_EDGE('',*,*,#25400,.F.) ;
#33943=ORIENTED_EDGE('',*,*,#25401,.F.) ;
#33944=ORIENTED_EDGE('',*,*,#25402,.F.) ;
#33945=ORIENTED_EDGE('',*,*,#25403,.F.) ;
#33946=ORIENTED_EDGE('',*,*,#25404,.T.) ;
#33947=ORIENTED_EDGE('',*,*,#25405,.F.) ;
#33948=ORIENTED_EDGE('',*,*,#25406,.F.) ;
#33949=ORIENTED_EDGE('',*,*,#25407,.F.) ;
#33950=ORIENTED_EDGE('',*,*,#25408,.F.) ;
#33951=ORIENTED_EDGE('',*,*,#25409,.F.) ;
#33952=ORIENTED_EDGE('',*,*,#25410,.F.) ;
#33953=ORIENTED_EDGE('',*,*,#25411,.F.) ;
#33954=ORIENTED_EDGE('',*,*,#25412,.F.) ;
#33955=ORIENTED_EDGE('',*,*,#25413,.F.) ;
#33956=ORIENTED_EDGE('',*,*,#25414,.F.) ;
#33957=ORIENTED_EDGE('',*,*,#25415,.F.) ;
#33958=ORIENTED_EDGE('',*,*,#25416,.F.) ;
#33959=ORIENTED_EDGE('',*,*,#25417,.F.) ;
#33960=ORIENTED_EDGE('',*,*,#25418,.F.) ;
#33961=ORIENTED_EDGE('',*,*,#25419,.F.) ;
#33962=ORIENTED_EDGE('',*,*,#25420,.F.) ;
#33963=ORIENTED_EDGE('',*,*,#25421,.F.) ;
#33964=ORIENTED_EDGE('',*,*,#25422,.F.) ;
#33965=ORIENTED_EDGE('',*,*,#25423,.F.) ;
#33966=ORIENTED_EDGE('',*,*,#25424,.F.) ;
#33967=ORIENTED_EDGE('',*,*,#25425,.F.) ;
#33968=ORIENTED_EDGE('',*,*,#25426,.F.) ;
#33969=ORIENTED_EDGE('',*,*,#25427,.F.) ;
#33970=ORIENTED_EDGE('',*,*,#25428,.F.) ;
#33971=ORIENTED_EDGE('',*,*,#25429,.F.) ;
#33972=ORIENTED_EDGE('',*,*,#25430,.F.) ;
#33973=ORIENTED_EDGE('',*,*,#25431,.F.) ;
#33974=ORIENTED_EDGE('',*,*,#25432,.F.) ;
#33975=ORIENTED_EDGE('',*,*,#25433,.F.) ;
#33976=ORIENTED_EDGE('',*,*,#25434,.F.) ;
#33977=ORIENTED_EDGE('',*,*,#25435,.F.) ;
#33978=ORIENTED_EDGE('',*,*,#25436,.F.) ;
#33979=ORIENTED_EDGE('',*,*,#25437,.F.) ;
#33980=ORIENTED_EDGE('',*,*,#25438,.F.) ;
#33981=ORIENTED_EDGE('',*,*,#25439,.F.) ;
#33982=ORIENTED_EDGE('',*,*,#25440,.F.) ;
#33983=ORIENTED_EDGE('',*,*,#25441,.F.) ;
#33984=ORIENTED_EDGE('',*,*,#25442,.F.) ;
#33985=ORIENTED_EDGE('',*,*,#25443,.F.) ;
#33986=ORIENTED_EDGE('',*,*,#25444,.F.) ;
#33987=ORIENTED_EDGE('',*,*,#25445,.F.) ;
#33988=ORIENTED_EDGE('',*,*,#25446,.F.) ;
#33989=ORIENTED_EDGE('',*,*,#25275,.F.) ;
#33990=ORIENTED_EDGE('',*,*,#25447,.T.) ;
#33991=ORIENTED_EDGE('',*,*,#25448,.F.) ;
#33992=ORIENTED_EDGE('',*,*,#25449,.T.) ;
#33993=ORIENTED_EDGE('',*,*,#25450,.T.) ;
#33994=ORIENTED_EDGE('',*,*,#25451,.T.) ;
#33995=ORIENTED_EDGE('',*,*,#25452,.T.) ;
#33996=ORIENTED_EDGE('',*,*,#25447,.F.) ;
#33997=ORIENTED_EDGE('',*,*,#25453,.T.) ;
#33998=ORIENTED_EDGE('',*,*,#25454,.T.) ;
#33999=ORIENTED_EDGE('',*,*,#25455,.T.) ;
#34000=ORIENTED_EDGE('',*,*,#25451,.F.) ;
#34001=ORIENTED_EDGE('',*,*,#25456,.T.) ;
#34002=ORIENTED_EDGE('',*,*,#25457,.T.) ;
#34003=ORIENTED_EDGE('',*,*,#25458,.T.) ;
#34004=ORIENTED_EDGE('',*,*,#25454,.F.) ;
#34005=ORIENTED_EDGE('',*,*,#25459,.T.) ;
#34006=ORIENTED_EDGE('',*,*,#25460,.T.) ;
#34007=ORIENTED_EDGE('',*,*,#25461,.T.) ;
#34008=ORIENTED_EDGE('',*,*,#25457,.F.) ;
#34009=ORIENTED_EDGE('',*,*,#25462,.T.) ;
#34010=ORIENTED_EDGE('',*,*,#25463,.T.) ;
#34011=ORIENTED_EDGE('',*,*,#25464,.T.) ;
#34012=ORIENTED_EDGE('',*,*,#25460,.F.) ;
#34013=ORIENTED_EDGE('',*,*,#25465,.T.) ;
#34014=ORIENTED_EDGE('',*,*,#25466,.T.) ;
#34015=ORIENTED_EDGE('',*,*,#25467,.T.) ;
#34016=ORIENTED_EDGE('',*,*,#25463,.F.) ;
#34017=ORIENTED_EDGE('',*,*,#25468,.T.) ;
#34018=ORIENTED_EDGE('',*,*,#25469,.T.) ;
#34019=ORIENTED_EDGE('',*,*,#25470,.T.) ;
#34020=ORIENTED_EDGE('',*,*,#25466,.F.) ;
#34021=ORIENTED_EDGE('',*,*,#25471,.T.) ;
#34022=ORIENTED_EDGE('',*,*,#25472,.T.) ;
#34023=ORIENTED_EDGE('',*,*,#25473,.T.) ;
#34024=ORIENTED_EDGE('',*,*,#25469,.F.) ;
#34025=ORIENTED_EDGE('',*,*,#25474,.T.) ;
#34026=ORIENTED_EDGE('',*,*,#25475,.T.) ;
#34027=ORIENTED_EDGE('',*,*,#25476,.T.) ;
#34028=ORIENTED_EDGE('',*,*,#25472,.F.) ;
#34029=ORIENTED_EDGE('',*,*,#25477,.T.) ;
#34030=ORIENTED_EDGE('',*,*,#25478,.T.) ;
#34031=ORIENTED_EDGE('',*,*,#25479,.T.) ;
#34032=ORIENTED_EDGE('',*,*,#25475,.F.) ;
#34033=ORIENTED_EDGE('',*,*,#25480,.T.) ;
#34034=ORIENTED_EDGE('',*,*,#25481,.T.) ;
#34035=ORIENTED_EDGE('',*,*,#25482,.T.) ;
#34036=ORIENTED_EDGE('',*,*,#25478,.F.) ;
#34037=ORIENTED_EDGE('',*,*,#25483,.T.) ;
#34038=ORIENTED_EDGE('',*,*,#25481,.F.) ;
#34039=ORIENTED_EDGE('',*,*,#25484,.T.) ;
#34040=ORIENTED_EDGE('',*,*,#25485,.T.) ;
#34041=ORIENTED_EDGE('',*,*,#25486,.F.) ;
#34042=ORIENTED_EDGE('',*,*,#25484,.F.) ;
#34043=ORIENTED_EDGE('',*,*,#25483,.F.) ;
#34044=ORIENTED_EDGE('',*,*,#25487,.F.) ;
#34045=ORIENTED_EDGE('',*,*,#25488,.F.) ;
#34046=ORIENTED_EDGE('',*,*,#25489,.F.) ;
#34047=ORIENTED_EDGE('',*,*,#25490,.F.) ;
#34048=ORIENTED_EDGE('',*,*,#25491,.F.) ;
#34049=ORIENTED_EDGE('',*,*,#25492,.F.) ;
#34050=ORIENTED_EDGE('',*,*,#25480,.F.) ;
#34051=ORIENTED_EDGE('',*,*,#25493,.T.) ;
#34052=ORIENTED_EDGE('',*,*,#25494,.F.) ;
#34053=ORIENTED_EDGE('',*,*,#25487,.T.) ;
#34054=ORIENTED_EDGE('',*,*,#25477,.F.) ;
#34055=ORIENTED_EDGE('',*,*,#25495,.F.) ;
#34056=ORIENTED_EDGE('',*,*,#25496,.F.) ;
#34057=ORIENTED_EDGE('',*,*,#25493,.F.) ;
#34058=ORIENTED_EDGE('',*,*,#25474,.F.) ;
#34059=ORIENTED_EDGE('',*,*,#25497,.T.) ;
#34060=ORIENTED_EDGE('',*,*,#25498,.F.) ;
#34061=ORIENTED_EDGE('',*,*,#25495,.T.) ;
#34062=ORIENTED_EDGE('',*,*,#25471,.F.) ;
#34063=ORIENTED_EDGE('',*,*,#25499,.T.) ;
#34064=ORIENTED_EDGE('',*,*,#25500,.F.) ;
#34065=ORIENTED_EDGE('',*,*,#25497,.F.) ;
#34066=ORIENTED_EDGE('',*,*,#25468,.F.) ;
#34067=ORIENTED_EDGE('',*,*,#25501,.T.) ;
#34068=ORIENTED_EDGE('',*,*,#25502,.F.) ;
#34069=ORIENTED_EDGE('',*,*,#25499,.F.) ;
#34070=ORIENTED_EDGE('',*,*,#25465,.F.) ;
#34071=ORIENTED_EDGE('',*,*,#25503,.F.) ;
#34072=ORIENTED_EDGE('',*,*,#25504,.F.) ;
#34073=ORIENTED_EDGE('',*,*,#25501,.F.) ;
#34074=ORIENTED_EDGE('',*,*,#25462,.F.) ;
#34075=ORIENTED_EDGE('',*,*,#25505,.T.) ;
#34076=ORIENTED_EDGE('',*,*,#25506,.F.) ;
#34077=ORIENTED_EDGE('',*,*,#25503,.T.) ;
#34078=ORIENTED_EDGE('',*,*,#25459,.F.) ;
#34079=ORIENTED_EDGE('',*,*,#25507,.F.) ;
#34080=ORIENTED_EDGE('',*,*,#25508,.F.) ;
#34081=ORIENTED_EDGE('',*,*,#25505,.F.) ;
#34082=ORIENTED_EDGE('',*,*,#25456,.F.) ;
#34083=ORIENTED_EDGE('',*,*,#25509,.T.) ;
#34084=ORIENTED_EDGE('',*,*,#25510,.F.) ;
#34085=ORIENTED_EDGE('',*,*,#25507,.T.) ;
#34086=ORIENTED_EDGE('',*,*,#25453,.F.) ;
#34087=ORIENTED_EDGE('',*,*,#25450,.F.) ;
#34088=ORIENTED_EDGE('',*,*,#25511,.F.) ;
#34089=ORIENTED_EDGE('',*,*,#25512,.F.) ;
#34090=ORIENTED_EDGE('',*,*,#25513,.F.) ;
#34091=ORIENTED_EDGE('',*,*,#25514,.F.) ;
#34092=ORIENTED_EDGE('',*,*,#25515,.F.) ;
#34093=ORIENTED_EDGE('',*,*,#25509,.F.) ;
#34094=ORIENTED_EDGE('',*,*,#25334,.T.) ;
#34095=ORIENTED_EDGE('',*,*,#25516,.T.) ;
#34096=ORIENTED_EDGE('',*,*,#25517,.T.) ;
#34097=ORIENTED_EDGE('',*,*,#25516,.F.) ;
#34098=ORIENTED_EDGE('',*,*,#25517,.F.) ;
#34099=ORIENTED_EDGE('',*,*,#25518,.T.) ;
#34100=ORIENTED_EDGE('',*,*,#25519,.T.) ;
#34101=ORIENTED_EDGE('',*,*,#25518,.F.) ;
#34102=ORIENTED_EDGE('',*,*,#25520,.T.) ;
#34103=ORIENTED_EDGE('',*,*,#25521,.T.) ;
#34104=ORIENTED_EDGE('',*,*,#25522,.T.) ;
#34105=ORIENTED_EDGE('',*,*,#25520,.F.) ;
#34106=ORIENTED_EDGE('',*,*,#25446,.T.) ;
#34107=ORIENTED_EDGE('',*,*,#25521,.F.) ;
#34108=ORIENTED_EDGE('',*,*,#25522,.F.) ;
#34109=ORIENTED_EDGE('',*,*,#25523,.T.) ;
#34110=ORIENTED_EDGE('',*,*,#25524,.T.) ;
#34111=ORIENTED_EDGE('',*,*,#25523,.F.) ;
#34112=ORIENTED_EDGE('',*,*,#25524,.F.) ;
#34113=ORIENTED_EDGE('',*,*,#25525,.F.) ;
#34114=ORIENTED_EDGE('',*,*,#25526,.T.) ;
#34115=ORIENTED_EDGE('',*,*,#25527,.T.) ;
#34116=ORIENTED_EDGE('',*,*,#25525,.T.) ;
#34117=ORIENTED_EDGE('',*,*,#25527,.F.) ;
#34118=ORIENTED_EDGE('',*,*,#25528,.T.) ;
#34119=ORIENTED_EDGE('',*,*,#25526,.F.) ;
#34120=ORIENTED_EDGE('',*,*,#25529,.T.) ;
#34121=ORIENTED_EDGE('',*,*,#25530,.F.) ;
#34122=ORIENTED_EDGE('',*,*,#25529,.F.) ;
#34123=ORIENTED_EDGE('',*,*,#25528,.F.) ;
#34124=ORIENTED_EDGE('',*,*,#25531,.T.) ;
#34125=ORIENTED_EDGE('',*,*,#25532,.T.) ;
#34126=ORIENTED_EDGE('',*,*,#25533,.T.) ;
#34127=ORIENTED_EDGE('',*,*,#25534,.T.) ;
#34128=ORIENTED_EDGE('',*,*,#25532,.F.) ;
#34129=ORIENTED_EDGE('',*,*,#25534,.F.) ;
#34130=ORIENTED_EDGE('',*,*,#25535,.T.) ;
#34131=ORIENTED_EDGE('',*,*,#25536,.F.) ;
#34132=ORIENTED_EDGE('',*,*,#25537,.F.) ;
#34133=ORIENTED_EDGE('',*,*,#25535,.F.) ;
#34134=ORIENTED_EDGE('',*,*,#25533,.F.) ;
#34135=ORIENTED_EDGE('',*,*,#25538,.F.) ;
#34136=ORIENTED_EDGE('',*,*,#25539,.F.) ;
#34137=ORIENTED_EDGE('',*,*,#25540,.F.) ;
#34138=ORIENTED_EDGE('',*,*,#25541,.T.) ;
#34139=ORIENTED_EDGE('',*,*,#25542,.F.) ;
#34140=ORIENTED_EDGE('',*,*,#25543,.F.) ;
#34141=ORIENTED_EDGE('',*,*,#25531,.F.) ;
#34142=ORIENTED_EDGE('',*,*,#25544,.T.) ;
#34143=ORIENTED_EDGE('',*,*,#25545,.T.) ;
#34144=ORIENTED_EDGE('',*,*,#25536,.T.) ;
#34145=ORIENTED_EDGE('',*,*,#25537,.T.) ;
#34146=ORIENTED_EDGE('',*,*,#25545,.F.) ;
#34147=ORIENTED_EDGE('',*,*,#25546,.T.) ;
#34148=ORIENTED_EDGE('',*,*,#25547,.T.) ;
#34149=ORIENTED_EDGE('',*,*,#25298,.T.) ;
#34150=ORIENTED_EDGE('',*,*,#25548,.T.) ;
#34151=ORIENTED_EDGE('',*,*,#25549,.T.) ;
#34152=ORIENTED_EDGE('',*,*,#25550,.F.) ;
#34153=ORIENTED_EDGE('',*,*,#25544,.F.) ;
#34154=ORIENTED_EDGE('',*,*,#25551,.T.) ;
#34155=ORIENTED_EDGE('',*,*,#25552,.T.) ;
#34156=ORIENTED_EDGE('',*,*,#25553,.T.) ;
#34157=ORIENTED_EDGE('',*,*,#25554,.T.) ;
#34158=ORIENTED_EDGE('',*,*,#25552,.F.) ;
#34159=ORIENTED_EDGE('',*,*,#25554,.F.) ;
#34160=ORIENTED_EDGE('',*,*,#25555,.T.) ;
#34161=ORIENTED_EDGE('',*,*,#25556,.F.) ;
#34162=ORIENTED_EDGE('',*,*,#25557,.F.) ;
#34163=ORIENTED_EDGE('',*,*,#25555,.F.) ;
#34164=ORIENTED_EDGE('',*,*,#25553,.F.) ;
#34165=ORIENTED_EDGE('',*,*,#25558,.F.) ;
#34166=ORIENTED_EDGE('',*,*,#25559,.F.) ;
#34167=ORIENTED_EDGE('',*,*,#25560,.F.) ;
#34168=ORIENTED_EDGE('',*,*,#25561,.T.) ;
#34169=ORIENTED_EDGE('',*,*,#25562,.F.) ;
#34170=ORIENTED_EDGE('',*,*,#25563,.F.) ;
#34171=ORIENTED_EDGE('',*,*,#25551,.F.) ;
#34172=ORIENTED_EDGE('',*,*,#25564,.T.) ;
#34173=ORIENTED_EDGE('',*,*,#25565,.T.) ;
#34174=ORIENTED_EDGE('',*,*,#25556,.T.) ;
#34175=ORIENTED_EDGE('',*,*,#25557,.T.) ;
#34176=ORIENTED_EDGE('',*,*,#25565,.F.) ;
#34177=ORIENTED_EDGE('',*,*,#25566,.T.) ;
#34178=ORIENTED_EDGE('',*,*,#25567,.F.) ;
#34179=ORIENTED_EDGE('',*,*,#25568,.T.) ;
#34180=ORIENTED_EDGE('',*,*,#25569,.T.) ;
#34181=ORIENTED_EDGE('',*,*,#25292,.T.) ;
#34182=ORIENTED_EDGE('',*,*,#25570,.T.) ;
#34183=ORIENTED_EDGE('',*,*,#25564,.F.) ;
#34184=ORIENTED_EDGE('',*,*,#25571,.T.) ;
#34185=ORIENTED_EDGE('',*,*,#25572,.T.) ;
#34186=ORIENTED_EDGE('',*,*,#25573,.T.) ;
#34187=ORIENTED_EDGE('',*,*,#25506,.T.) ;
#34188=ORIENTED_EDGE('',*,*,#25574,.T.) ;
#34189=ORIENTED_EDGE('',*,*,#25504,.T.) ;
#34190=ORIENTED_EDGE('',*,*,#25573,.F.) ;
#34191=ORIENTED_EDGE('',*,*,#25575,.T.) ;
#34192=ORIENTED_EDGE('',*,*,#25576,.T.) ;
#34193=ORIENTED_EDGE('',*,*,#25502,.T.) ;
#34194=ORIENTED_EDGE('',*,*,#25574,.F.) ;
#34195=ORIENTED_EDGE('',*,*,#25577,.T.) ;
#34196=ORIENTED_EDGE('',*,*,#25578,.T.) ;
#34197=ORIENTED_EDGE('',*,*,#25500,.T.) ;
#34198=ORIENTED_EDGE('',*,*,#25576,.F.) ;
#34199=ORIENTED_EDGE('',*,*,#25579,.T.) ;
#34200=ORIENTED_EDGE('',*,*,#25580,.T.) ;
#34201=ORIENTED_EDGE('',*,*,#25498,.T.) ;
#34202=ORIENTED_EDGE('',*,*,#25578,.F.) ;
#34203=ORIENTED_EDGE('',*,*,#25581,.T.) ;
#34204=ORIENTED_EDGE('',*,*,#25581,.F.) ;
#34205=ORIENTED_EDGE('',*,*,#25579,.F.) ;
#34206=ORIENTED_EDGE('',*,*,#25577,.F.) ;
#34207=ORIENTED_EDGE('',*,*,#25575,.F.) ;
#34208=ORIENTED_EDGE('',*,*,#25572,.F.) ;
#34209=ORIENTED_EDGE('',*,*,#25582,.F.) ;
#34210=ORIENTED_EDGE('',*,*,#25583,.F.) ;
#34211=ORIENTED_EDGE('',*,*,#25584,.F.) ;
#34212=ORIENTED_EDGE('',*,*,#25585,.F.) ;
#34213=ORIENTED_EDGE('',*,*,#25586,.F.) ;
#34214=ORIENTED_EDGE('',*,*,#25587,.F.) ;
#34215=ORIENTED_EDGE('',*,*,#25561,.F.) ;
#34216=ORIENTED_EDGE('',*,*,#25588,.F.) ;
#34217=ORIENTED_EDGE('',*,*,#25589,.F.) ;
#34218=ORIENTED_EDGE('',*,*,#25590,.F.) ;
#34219=ORIENTED_EDGE('',*,*,#25591,.F.) ;
#34220=ORIENTED_EDGE('',*,*,#25592,.F.) ;
#34221=ORIENTED_EDGE('',*,*,#25541,.F.) ;
#34222=ORIENTED_EDGE('',*,*,#25593,.F.) ;
#34223=ORIENTED_EDGE('',*,*,#25594,.F.) ;
#34224=ORIENTED_EDGE('',*,*,#25595,.F.) ;
#34225=ORIENTED_EDGE('',*,*,#25596,.F.) ;
#34226=ORIENTED_EDGE('',*,*,#25597,.F.) ;
#34227=ORIENTED_EDGE('',*,*,#25598,.F.) ;
#34228=ORIENTED_EDGE('',*,*,#25571,.F.) ;
#34229=ORIENTED_EDGE('',*,*,#25508,.T.) ;
#34230=ORIENTED_EDGE('',*,*,#25599,.F.) ;
#34231=ORIENTED_EDGE('',*,*,#25582,.T.) ;
#34232=ORIENTED_EDGE('',*,*,#25482,.F.) ;
#34233=ORIENTED_EDGE('',*,*,#25600,.F.) ;
#34234=ORIENTED_EDGE('',*,*,#25601,.F.) ;
#34235=ORIENTED_EDGE('',*,*,#25602,.T.) ;
#34236=ORIENTED_EDGE('',*,*,#25550,.T.) ;
#34237=ORIENTED_EDGE('',*,*,#25603,.T.) ;
#34238=ORIENTED_EDGE('',*,*,#25604,.F.) ;
#34239=ORIENTED_EDGE('',*,*,#25605,.F.) ;
#34240=ORIENTED_EDGE('',*,*,#25295,.T.) ;
#34241=ORIENTED_EDGE('',*,*,#25606,.T.) ;
#34242=ORIENTED_EDGE('',*,*,#25607,.F.) ;
#34243=ORIENTED_EDGE('',*,*,#25608,.T.) ;
#34244=ORIENTED_EDGE('',*,*,#25567,.T.) ;
#34245=ORIENTED_EDGE('',*,*,#25609,.T.) ;
#34246=ORIENTED_EDGE('',*,*,#25610,.F.) ;
#34247=ORIENTED_EDGE('',*,*,#25611,.F.) ;
#34248=ORIENTED_EDGE('',*,*,#25612,.F.) ;
#34249=ORIENTED_EDGE('',*,*,#25613,.F.) ;
#34250=ORIENTED_EDGE('',*,*,#25614,.F.) ;
#34251=ORIENTED_EDGE('',*,*,#25615,.F.) ;
#34252=ORIENTED_EDGE('',*,*,#25616,.F.) ;
#34253=ORIENTED_EDGE('',*,*,#25452,.F.) ;
#34254=ORIENTED_EDGE('',*,*,#25455,.F.) ;
#34255=ORIENTED_EDGE('',*,*,#25458,.F.) ;
#34256=ORIENTED_EDGE('',*,*,#25461,.F.) ;
#34257=ORIENTED_EDGE('',*,*,#25464,.F.) ;
#34258=ORIENTED_EDGE('',*,*,#25467,.F.) ;
#34259=ORIENTED_EDGE('',*,*,#25470,.F.) ;
#34260=ORIENTED_EDGE('',*,*,#25473,.F.) ;
#34261=ORIENTED_EDGE('',*,*,#25476,.F.) ;
#34262=ORIENTED_EDGE('',*,*,#25479,.F.) ;
#34263=ORIENTED_EDGE('',*,*,#25580,.F.) ;
#34264=ORIENTED_EDGE('',*,*,#25598,.T.) ;
#34265=ORIENTED_EDGE('',*,*,#25617,.T.) ;
#34266=ORIENTED_EDGE('',*,*,#25496,.T.) ;
#34267=ORIENTED_EDGE('',*,*,#25618,.F.) ;
#34268=ORIENTED_EDGE('',*,*,#25290,.T.) ;
#34269=ORIENTED_EDGE('',*,*,#25619,.T.) ;
#34270=ORIENTED_EDGE('',*,*,#25611,.T.) ;
#34271=ORIENTED_EDGE('',*,*,#25620,.T.) ;
#34272=ORIENTED_EDGE('',*,*,#25612,.T.) ;
#34273=ORIENTED_EDGE('',*,*,#25619,.F.) ;
#34274=ORIENTED_EDGE('',*,*,#25621,.T.) ;
#34275=ORIENTED_EDGE('',*,*,#25622,.T.) ;
#34276=ORIENTED_EDGE('',*,*,#25613,.T.) ;
#34277=ORIENTED_EDGE('',*,*,#25620,.F.) ;
#34278=ORIENTED_EDGE('',*,*,#25623,.T.) ;
#34279=ORIENTED_EDGE('',*,*,#25624,.T.) ;
#34280=ORIENTED_EDGE('',*,*,#25614,.T.) ;
#34281=ORIENTED_EDGE('',*,*,#25622,.F.) ;
#34282=ORIENTED_EDGE('',*,*,#25625,.T.) ;
#34283=ORIENTED_EDGE('',*,*,#25626,.T.) ;
#34284=ORIENTED_EDGE('',*,*,#25615,.T.) ;
#34285=ORIENTED_EDGE('',*,*,#25624,.F.) ;
#34286=ORIENTED_EDGE('',*,*,#25627,.T.) ;
#34287=ORIENTED_EDGE('',*,*,#25626,.F.) ;
#34288=ORIENTED_EDGE('',*,*,#25277,.T.) ;
#34289=ORIENTED_EDGE('',*,*,#25448,.T.) ;
#34290=ORIENTED_EDGE('',*,*,#25616,.T.) ;
#34291=ORIENTED_EDGE('',*,*,#25449,.F.) ;
#34292=ORIENTED_EDGE('',*,*,#25333,.T.) ;
#34293=ORIENTED_EDGE('',*,*,#25628,.T.) ;
#34294=ORIENTED_EDGE('',*,*,#25511,.T.) ;
#34295=ORIENTED_EDGE('',*,*,#25627,.F.) ;
#34296=ORIENTED_EDGE('',*,*,#25629,.F.) ;
#34297=ORIENTED_EDGE('',*,*,#25630,.T.) ;
#34298=ORIENTED_EDGE('',*,*,#25631,.T.) ;
#34299=ORIENTED_EDGE('',*,*,#25278,.T.) ;
#34300=ORIENTED_EDGE('',*,*,#25625,.F.) ;
#34301=ORIENTED_EDGE('',*,*,#25632,.F.) ;
#34302=ORIENTED_EDGE('',*,*,#25633,.T.) ;
#34303=ORIENTED_EDGE('',*,*,#25629,.T.) ;
#34304=ORIENTED_EDGE('',*,*,#25623,.F.) ;
#34305=ORIENTED_EDGE('',*,*,#25634,.F.) ;
#34306=ORIENTED_EDGE('',*,*,#25635,.T.) ;
#34307=ORIENTED_EDGE('',*,*,#25632,.T.) ;
#34308=ORIENTED_EDGE('',*,*,#25621,.F.) ;
#34309=ORIENTED_EDGE('',*,*,#25289,.T.) ;
#34310=ORIENTED_EDGE('',*,*,#25636,.F.) ;
#34311=ORIENTED_EDGE('',*,*,#25637,.T.) ;
#34312=ORIENTED_EDGE('',*,*,#25634,.T.) ;
#34313=ORIENTED_EDGE('',*,*,#25638,.F.) ;
#34314=ORIENTED_EDGE('',*,*,#25600,.T.) ;
#34315=ORIENTED_EDGE('',*,*,#25486,.T.) ;
#34316=ORIENTED_EDGE('',*,*,#25300,.T.) ;
#34317=ORIENTED_EDGE('',*,*,#25638,.T.) ;
#34318=ORIENTED_EDGE('',*,*,#25299,.F.) ;
#34319=ORIENTED_EDGE('',*,*,#25547,.F.) ;
#34320=ORIENTED_EDGE('',*,*,#25639,.F.) ;
#34321=ORIENTED_EDGE('',*,*,#25601,.T.) ;
#34322=ORIENTED_EDGE('',*,*,#25640,.F.) ;
#34323=ORIENTED_EDGE('',*,*,#25641,.F.) ;
#34324=ORIENTED_EDGE('',*,*,#25642,.F.) ;
#34325=ORIENTED_EDGE('',*,*,#25643,.T.) ;
#34326=ORIENTED_EDGE('',*,*,#25644,.T.) ;
#34327=ORIENTED_EDGE('',*,*,#25641,.T.) ;
#34328=ORIENTED_EDGE('',*,*,#25159,.T.) ;
#34329=ORIENTED_EDGE('',*,*,#25643,.F.) ;
#34330=ORIENTED_EDGE('',*,*,#25158,.T.) ;
#34331=ORIENTED_EDGE('',*,*,#25645,.T.) ;
#34332=ORIENTED_EDGE('',*,*,#25646,.F.) ;
#34333=ORIENTED_EDGE('',*,*,#25647,.T.) ;
#34334=ORIENTED_EDGE('',*,*,#25648,.T.) ;
#34335=ORIENTED_EDGE('',*,*,#25649,.T.) ;
#34336=ORIENTED_EDGE('',*,*,#25647,.F.) ;
#34337=ORIENTED_EDGE('',*,*,#25650,.T.) ;
#34338=ORIENTED_EDGE('',*,*,#25642,.T.) ;
#34339=ORIENTED_EDGE('',*,*,#25651,.T.) ;
#34340=ORIENTED_EDGE('',*,*,#25163,.T.) ;
#34341=ORIENTED_EDGE('',*,*,#25652,.F.) ;
#34342=ORIENTED_EDGE('',*,*,#25653,.F.) ;
#34343=ORIENTED_EDGE('',*,*,#25654,.F.) ;
#34344=ORIENTED_EDGE('',*,*,#25655,.F.) ;
#34345=ORIENTED_EDGE('',*,*,#25656,.F.) ;
#34346=ORIENTED_EDGE('',*,*,#25161,.T.) ;
#34347=ORIENTED_EDGE('',*,*,#25657,.F.) ;
#34348=ORIENTED_EDGE('',*,*,#25652,.T.) ;
#34349=ORIENTED_EDGE('',*,*,#25162,.T.) ;
#34350=ORIENTED_EDGE('',*,*,#25656,.T.) ;
#34351=ORIENTED_EDGE('',*,*,#25658,.T.) ;
#34352=ORIENTED_EDGE('',*,*,#25657,.T.) ;
#34353=ORIENTED_EDGE('',*,*,#25160,.T.) ;
#34354=ORIENTED_EDGE('',*,*,#25640,.T.) ;
#34355=ORIENTED_EDGE('',*,*,#25659,.T.) ;
#34356=ORIENTED_EDGE('',*,*,#25660,.T.) ;
#34357=ORIENTED_EDGE('',*,*,#25661,.T.) ;
#34358=ORIENTED_EDGE('',*,*,#25405,.T.) ;
#34359=ORIENTED_EDGE('',*,*,#25662,.T.) ;
#34360=ORIENTED_EDGE('',*,*,#25655,.T.) ;
#34361=ORIENTED_EDGE('',*,*,#25663,.T.) ;
#34362=ORIENTED_EDGE('',*,*,#25660,.F.) ;
#34363=ORIENTED_EDGE('',*,*,#25664,.T.) ;
#34364=ORIENTED_EDGE('',*,*,#25665,.T.) ;
#34365=ORIENTED_EDGE('',*,*,#25666,.T.) ;
#34366=ORIENTED_EDGE('',*,*,#25653,.T.) ;
#34367=ORIENTED_EDGE('',*,*,#25667,.T.) ;
#34368=ORIENTED_EDGE('',*,*,#25417,.T.) ;
#34369=ORIENTED_EDGE('',*,*,#25668,.T.) ;
#34370=ORIENTED_EDGE('',*,*,#25665,.F.) ;
#34371=ORIENTED_EDGE('',*,*,#25669,.T.) ;
#34372=ORIENTED_EDGE('',*,*,#25670,.T.) ;
#34373=ORIENTED_EDGE('',*,*,#25164,.T.) ;
#34374=ORIENTED_EDGE('',*,*,#25654,.T.) ;
#34375=ORIENTED_EDGE('',*,*,#25671,.T.) ;
#34376=ORIENTED_EDGE('',*,*,#25670,.F.) ;
#34377=ORIENTED_EDGE('',*,*,#25672,.T.) ;
#34378=ORIENTED_EDGE('',*,*,#25673,.T.) ;
#34379=ORIENTED_EDGE('',*,*,#25648,.F.) ;
#34380=ORIENTED_EDGE('',*,*,#25674,.T.) ;
#34381=ORIENTED_EDGE('',*,*,#25675,.T.) ;
#34382=ORIENTED_EDGE('',*,*,#25407,.T.) ;
#34383=ORIENTED_EDGE('',*,*,#25651,.F.) ;
#34384=ORIENTED_EDGE('',*,*,#25644,.F.) ;
#34385=ORIENTED_EDGE('',*,*,#25676,.F.) ;
#34386=ORIENTED_EDGE('',*,*,#25674,.F.) ;
#34387=ORIENTED_EDGE('',*,*,#25673,.F.) ;
#34388=ORIENTED_EDGE('',*,*,#25677,.T.) ;
#34389=ORIENTED_EDGE('',*,*,#25678,.T.) ;
#34390=ORIENTED_EDGE('',*,*,#25165,.T.) ;
#34391=ORIENTED_EDGE('',*,*,#25672,.F.) ;
#34392=ORIENTED_EDGE('',*,*,#25679,.T.) ;
#34393=ORIENTED_EDGE('',*,*,#25680,.F.) ;
#34394=ORIENTED_EDGE('',*,*,#25681,.T.) ;
#34395=ORIENTED_EDGE('',*,*,#25671,.F.) ;
#34396=ORIENTED_EDGE('',*,*,#25666,.F.) ;
#34397=ORIENTED_EDGE('',*,*,#25682,.F.) ;
#34398=ORIENTED_EDGE('',*,*,#25679,.F.) ;
#34399=ORIENTED_EDGE('',*,*,#25683,.T.) ;
#34400=ORIENTED_EDGE('',*,*,#25684,.T.) ;
#34401=ORIENTED_EDGE('',*,*,#25393,.T.) ;
#34402=ORIENTED_EDGE('',*,*,#25685,.T.) ;
#34403=ORIENTED_EDGE('',*,*,#25686,.T.) ;
#34404=ORIENTED_EDGE('',*,*,#25687,.T.) ;
#34405=ORIENTED_EDGE('',*,*,#25683,.F.) ;
#34406=ORIENTED_EDGE('',*,*,#25688,.T.) ;
#34407=ORIENTED_EDGE('',*,*,#25686,.F.) ;
#34408=ORIENTED_EDGE('',*,*,#25689,.T.) ;
#34409=ORIENTED_EDGE('',*,*,#25690,.T.) ;
#34410=ORIENTED_EDGE('',*,*,#25689,.F.) ;
#34411=ORIENTED_EDGE('',*,*,#25691,.T.) ;
#34412=ORIENTED_EDGE('',*,*,#25692,.F.) ;
#34413=ORIENTED_EDGE('',*,*,#25215,.F.) ;
#34414=ORIENTED_EDGE('',*,*,#25688,.F.) ;
#34415=ORIENTED_EDGE('',*,*,#25685,.F.) ;
#34416=ORIENTED_EDGE('',*,*,#25392,.F.) ;
#34417=ORIENTED_EDGE('',*,*,#25693,.T.) ;
#34418=ORIENTED_EDGE('',*,*,#25691,.F.) ;
#34419=ORIENTED_EDGE('',*,*,#25694,.T.) ;
#34420=ORIENTED_EDGE('',*,*,#25695,.T.) ;
#34421=ORIENTED_EDGE('',*,*,#25696,.T.) ;
#34422=ORIENTED_EDGE('',*,*,#25697,.T.) ;
#34423=ORIENTED_EDGE('',*,*,#25698,.T.) ;
#34424=ORIENTED_EDGE('',*,*,#25694,.F.) ;
#34425=ORIENTED_EDGE('',*,*,#25699,.T.) ;
#34426=ORIENTED_EDGE('',*,*,#25403,.T.) ;
#34427=ORIENTED_EDGE('',*,*,#25700,.T.) ;
#34428=ORIENTED_EDGE('',*,*,#25697,.F.) ;
#34429=ORIENTED_EDGE('',*,*,#25701,.T.) ;
#34430=ORIENTED_EDGE('',*,*,#25701,.F.) ;
#34431=ORIENTED_EDGE('',*,*,#25699,.F.) ;
#34432=ORIENTED_EDGE('',*,*,#25702,.F.) ;
#34433=ORIENTED_EDGE('',*,*,#25703,.T.) ;
#34434=ORIENTED_EDGE('',*,*,#25390,.F.) ;
#34435=ORIENTED_EDGE('',*,*,#25696,.F.) ;
#34436=ORIENTED_EDGE('',*,*,#25205,.F.) ;
#34437=ORIENTED_EDGE('',*,*,#25704,.T.) ;
#34438=ORIENTED_EDGE('',*,*,#25702,.T.) ;
#34439=ORIENTED_EDGE('',*,*,#25705,.T.) ;
#34440=ORIENTED_EDGE('',*,*,#25283,.T.) ;
#34441=ORIENTED_EDGE('',*,*,#25706,.T.) ;
#34442=ORIENTED_EDGE('',*,*,#25707,.T.) ;
#34443=ORIENTED_EDGE('',*,*,#25708,.T.) ;
#34444=ORIENTED_EDGE('',*,*,#25284,.T.) ;
#34445=ORIENTED_EDGE('',*,*,#25705,.F.) ;
#34446=ORIENTED_EDGE('',*,*,#25709,.T.) ;
#34447=ORIENTED_EDGE('',*,*,#25710,.T.) ;
#34448=ORIENTED_EDGE('',*,*,#25285,.T.) ;
#34449=ORIENTED_EDGE('',*,*,#25708,.F.) ;
#34450=ORIENTED_EDGE('',*,*,#25711,.T.) ;
#34451=ORIENTED_EDGE('',*,*,#25712,.T.) ;
#34452=ORIENTED_EDGE('',*,*,#25286,.T.) ;
#34453=ORIENTED_EDGE('',*,*,#25710,.F.) ;
#34454=ORIENTED_EDGE('',*,*,#25713,.T.) ;
#34455=ORIENTED_EDGE('',*,*,#25714,.T.) ;
#34456=ORIENTED_EDGE('',*,*,#25287,.T.) ;
#34457=ORIENTED_EDGE('',*,*,#25712,.F.) ;
#34458=ORIENTED_EDGE('',*,*,#25715,.T.) ;
#34459=ORIENTED_EDGE('',*,*,#25636,.T.) ;
#34460=ORIENTED_EDGE('',*,*,#25288,.T.) ;
#34461=ORIENTED_EDGE('',*,*,#25714,.F.) ;
#34462=ORIENTED_EDGE('',*,*,#25716,.T.) ;
#34463=ORIENTED_EDGE('',*,*,#25717,.F.) ;
#34464=ORIENTED_EDGE('',*,*,#25279,.T.) ;
#34465=ORIENTED_EDGE('',*,*,#25631,.F.) ;
#34466=ORIENTED_EDGE('',*,*,#25718,.T.) ;
#34467=ORIENTED_EDGE('',*,*,#25718,.F.) ;
#34468=ORIENTED_EDGE('',*,*,#25719,.F.) ;
#34469=ORIENTED_EDGE('',*,*,#25720,.F.) ;
#34470=ORIENTED_EDGE('',*,*,#25721,.T.) ;
#34471=ORIENTED_EDGE('',*,*,#25630,.F.) ;
#34472=ORIENTED_EDGE('',*,*,#25722,.T.) ;
#34473=ORIENTED_EDGE('',*,*,#25723,.T.) ;
#34474=ORIENTED_EDGE('',*,*,#25719,.T.) ;
#34475=ORIENTED_EDGE('',*,*,#25633,.F.) ;
#34476=ORIENTED_EDGE('',*,*,#25724,.F.) ;
#34477=ORIENTED_EDGE('',*,*,#25725,.F.) ;
#34478=ORIENTED_EDGE('',*,*,#25722,.F.) ;
#34479=ORIENTED_EDGE('',*,*,#25635,.F.) ;
#34480=ORIENTED_EDGE('',*,*,#25726,.T.) ;
#34481=ORIENTED_EDGE('',*,*,#25727,.T.) ;
#34482=ORIENTED_EDGE('',*,*,#25724,.T.) ;
#34483=ORIENTED_EDGE('',*,*,#25637,.F.) ;
#34484=ORIENTED_EDGE('',*,*,#25728,.F.) ;
#34485=ORIENTED_EDGE('',*,*,#25729,.F.) ;
#34486=ORIENTED_EDGE('',*,*,#25726,.F.) ;
#34487=ORIENTED_EDGE('',*,*,#25716,.F.) ;
#34488=ORIENTED_EDGE('',*,*,#25730,.T.) ;
#34489=ORIENTED_EDGE('',*,*,#25731,.T.) ;
#34490=ORIENTED_EDGE('',*,*,#25728,.T.) ;
#34491=ORIENTED_EDGE('',*,*,#25715,.F.) ;
#34492=ORIENTED_EDGE('',*,*,#25732,.F.) ;
#34493=ORIENTED_EDGE('',*,*,#25733,.F.) ;
#34494=ORIENTED_EDGE('',*,*,#25730,.F.) ;
#34495=ORIENTED_EDGE('',*,*,#25713,.F.) ;
#34496=ORIENTED_EDGE('',*,*,#25734,.T.) ;
#34497=ORIENTED_EDGE('',*,*,#25735,.T.) ;
#34498=ORIENTED_EDGE('',*,*,#25732,.T.) ;
#34499=ORIENTED_EDGE('',*,*,#25711,.F.) ;
#34500=ORIENTED_EDGE('',*,*,#25736,.F.) ;
#34501=ORIENTED_EDGE('',*,*,#25737,.F.) ;
#34502=ORIENTED_EDGE('',*,*,#25734,.F.) ;
#34503=ORIENTED_EDGE('',*,*,#25709,.F.) ;
#34504=ORIENTED_EDGE('',*,*,#25738,.T.) ;
#34505=ORIENTED_EDGE('',*,*,#25739,.T.) ;
#34506=ORIENTED_EDGE('',*,*,#25736,.T.) ;
#34507=ORIENTED_EDGE('',*,*,#25707,.F.) ;
#34508=ORIENTED_EDGE('',*,*,#25740,.T.) ;
#34509=ORIENTED_EDGE('',*,*,#25741,.F.) ;
#34510=ORIENTED_EDGE('',*,*,#25738,.F.) ;
#34511=ORIENTED_EDGE('',*,*,#25742,.T.) ;
#34512=ORIENTED_EDGE('',*,*,#25743,.T.) ;
#34513=ORIENTED_EDGE('',*,*,#25744,.T.) ;
#34514=ORIENTED_EDGE('',*,*,#25335,.T.) ;
#34515=ORIENTED_EDGE('',*,*,#25745,.T.) ;
#34516=ORIENTED_EDGE('',*,*,#25746,.T.) ;
#34517=ORIENTED_EDGE('',*,*,#25742,.F.) ;
#34518=ORIENTED_EDGE('',*,*,#25348,.T.) ;
#34519=ORIENTED_EDGE('',*,*,#25747,.T.) ;
#34520=ORIENTED_EDGE('',*,*,#25748,.T.) ;
#34521=ORIENTED_EDGE('',*,*,#25745,.F.) ;
#34522=ORIENTED_EDGE('',*,*,#25347,.T.) ;
#34523=ORIENTED_EDGE('',*,*,#25749,.T.) ;
#34524=ORIENTED_EDGE('',*,*,#25750,.T.) ;
#34525=ORIENTED_EDGE('',*,*,#25747,.F.) ;
#34526=ORIENTED_EDGE('',*,*,#25346,.T.) ;
#34527=ORIENTED_EDGE('',*,*,#25751,.T.) ;
#34528=ORIENTED_EDGE('',*,*,#25752,.T.) ;
#34529=ORIENTED_EDGE('',*,*,#25749,.F.) ;
#34530=ORIENTED_EDGE('',*,*,#25345,.T.) ;
#34531=ORIENTED_EDGE('',*,*,#25753,.T.) ;
#34532=ORIENTED_EDGE('',*,*,#25754,.T.) ;
#34533=ORIENTED_EDGE('',*,*,#25751,.F.) ;
#34534=ORIENTED_EDGE('',*,*,#25344,.T.) ;
#34535=ORIENTED_EDGE('',*,*,#25755,.T.) ;
#34536=ORIENTED_EDGE('',*,*,#25756,.T.) ;
#34537=ORIENTED_EDGE('',*,*,#25753,.F.) ;
#34538=ORIENTED_EDGE('',*,*,#25343,.T.) ;
#34539=ORIENTED_EDGE('',*,*,#25757,.T.) ;
#34540=ORIENTED_EDGE('',*,*,#25758,.T.) ;
#34541=ORIENTED_EDGE('',*,*,#25755,.F.) ;
#34542=ORIENTED_EDGE('',*,*,#25342,.T.) ;
#34543=ORIENTED_EDGE('',*,*,#25759,.T.) ;
#34544=ORIENTED_EDGE('',*,*,#25760,.T.) ;
#34545=ORIENTED_EDGE('',*,*,#25757,.F.) ;
#34546=ORIENTED_EDGE('',*,*,#25341,.T.) ;
#34547=ORIENTED_EDGE('',*,*,#25761,.T.) ;
#34548=ORIENTED_EDGE('',*,*,#25762,.T.) ;
#34549=ORIENTED_EDGE('',*,*,#25763,.T.) ;
#34550=ORIENTED_EDGE('',*,*,#25340,.T.) ;
#34551=ORIENTED_EDGE('',*,*,#25764,.T.) ;
#34552=ORIENTED_EDGE('',*,*,#25765,.T.) ;
#34553=ORIENTED_EDGE('',*,*,#25761,.F.) ;
#34554=ORIENTED_EDGE('',*,*,#25339,.T.) ;
#34555=ORIENTED_EDGE('',*,*,#25766,.T.) ;
#34556=ORIENTED_EDGE('',*,*,#25767,.T.) ;
#34557=ORIENTED_EDGE('',*,*,#25764,.F.) ;
#34558=ORIENTED_EDGE('',*,*,#25338,.T.) ;
#34559=ORIENTED_EDGE('',*,*,#25768,.T.) ;
#34560=ORIENTED_EDGE('',*,*,#25769,.T.) ;
#34561=ORIENTED_EDGE('',*,*,#25766,.F.) ;
#34562=ORIENTED_EDGE('',*,*,#25337,.T.) ;
#34563=ORIENTED_EDGE('',*,*,#25770,.T.) ;
#34564=ORIENTED_EDGE('',*,*,#25771,.T.) ;
#34565=ORIENTED_EDGE('',*,*,#25768,.F.) ;
#34566=ORIENTED_EDGE('',*,*,#25336,.T.) ;
#34567=ORIENTED_EDGE('',*,*,#25763,.F.) ;
#34568=ORIENTED_EDGE('',*,*,#25772,.T.) ;
#34569=ORIENTED_EDGE('',*,*,#25759,.F.) ;
#34570=ORIENTED_EDGE('',*,*,#25744,.F.) ;
#34571=ORIENTED_EDGE('',*,*,#25773,.T.) ;
#34572=ORIENTED_EDGE('',*,*,#25770,.F.) ;
#34573=ORIENTED_EDGE('',*,*,#25750,.F.) ;
#34574=ORIENTED_EDGE('',*,*,#25774,.T.) ;
#34575=ORIENTED_EDGE('',*,*,#25775,.T.) ;
#34576=ORIENTED_EDGE('',*,*,#25776,.T.) ;
#34577=ORIENTED_EDGE('',*,*,#25752,.F.) ;
#34578=ORIENTED_EDGE('',*,*,#25777,.F.) ;
#34579=ORIENTED_EDGE('',*,*,#25778,.F.) ;
#34580=ORIENTED_EDGE('',*,*,#25774,.F.) ;
#34581=ORIENTED_EDGE('',*,*,#25754,.F.) ;
#34582=ORIENTED_EDGE('',*,*,#25779,.T.) ;
#34583=ORIENTED_EDGE('',*,*,#25780,.T.) ;
#34584=ORIENTED_EDGE('',*,*,#25777,.T.) ;
#34585=ORIENTED_EDGE('',*,*,#25756,.F.) ;
#34586=ORIENTED_EDGE('',*,*,#25781,.F.) ;
#34587=ORIENTED_EDGE('',*,*,#25782,.F.) ;
#34588=ORIENTED_EDGE('',*,*,#25779,.F.) ;
#34589=ORIENTED_EDGE('',*,*,#25758,.F.) ;
#34590=ORIENTED_EDGE('',*,*,#25783,.T.) ;
#34591=ORIENTED_EDGE('',*,*,#25784,.T.) ;
#34592=ORIENTED_EDGE('',*,*,#25781,.T.) ;
#34593=ORIENTED_EDGE('',*,*,#25760,.F.) ;
#34594=ORIENTED_EDGE('',*,*,#25785,.F.) ;
#34595=ORIENTED_EDGE('',*,*,#25786,.F.) ;
#34596=ORIENTED_EDGE('',*,*,#25783,.F.) ;
#34597=ORIENTED_EDGE('',*,*,#25772,.F.) ;
#34598=ORIENTED_EDGE('',*,*,#25787,.T.) ;
#34599=ORIENTED_EDGE('',*,*,#25788,.T.) ;
#34600=ORIENTED_EDGE('',*,*,#25785,.T.) ;
#34601=ORIENTED_EDGE('',*,*,#25762,.F.) ;
#34602=ORIENTED_EDGE('',*,*,#25789,.F.) ;
#34603=ORIENTED_EDGE('',*,*,#25790,.F.) ;
#34604=ORIENTED_EDGE('',*,*,#25787,.F.) ;
#34605=ORIENTED_EDGE('',*,*,#25363,.T.) ;
#34606=ORIENTED_EDGE('',*,*,#25791,.F.) ;
#34607=ORIENTED_EDGE('',*,*,#25792,.F.) ;
#34608=ORIENTED_EDGE('',*,*,#25793,.F.) ;
#34609=ORIENTED_EDGE('',*,*,#25794,.F.) ;
#34610=ORIENTED_EDGE('',*,*,#25795,.F.) ;
#34611=ORIENTED_EDGE('',*,*,#25353,.T.) ;
#34612=ORIENTED_EDGE('',*,*,#25796,.F.) ;
#34613=ORIENTED_EDGE('',*,*,#25797,.T.) ;
#34614=ORIENTED_EDGE('',*,*,#25354,.T.) ;
#34615=ORIENTED_EDGE('',*,*,#25795,.T.) ;
#34616=ORIENTED_EDGE('',*,*,#25798,.T.) ;
#34617=ORIENTED_EDGE('',*,*,#25799,.T.) ;
#34618=ORIENTED_EDGE('',*,*,#25355,.T.) ;
#34619=ORIENTED_EDGE('',*,*,#25797,.F.) ;
#34620=ORIENTED_EDGE('',*,*,#25800,.T.) ;
#34621=ORIENTED_EDGE('',*,*,#25801,.T.) ;
#34622=ORIENTED_EDGE('',*,*,#25356,.T.) ;
#34623=ORIENTED_EDGE('',*,*,#25799,.F.) ;
#34624=ORIENTED_EDGE('',*,*,#25802,.T.) ;
#34625=ORIENTED_EDGE('',*,*,#25803,.T.) ;
#34626=ORIENTED_EDGE('',*,*,#25357,.T.) ;
#34627=ORIENTED_EDGE('',*,*,#25801,.F.) ;
#34628=ORIENTED_EDGE('',*,*,#25804,.T.) ;
#34629=ORIENTED_EDGE('',*,*,#25805,.T.) ;
#34630=ORIENTED_EDGE('',*,*,#25358,.T.) ;
#34631=ORIENTED_EDGE('',*,*,#25803,.F.) ;
#34632=ORIENTED_EDGE('',*,*,#25806,.T.) ;
#34633=ORIENTED_EDGE('',*,*,#25807,.T.) ;
#34634=ORIENTED_EDGE('',*,*,#25359,.T.) ;
#34635=ORIENTED_EDGE('',*,*,#25805,.F.) ;
#34636=ORIENTED_EDGE('',*,*,#25808,.T.) ;
#34637=ORIENTED_EDGE('',*,*,#25809,.T.) ;
#34638=ORIENTED_EDGE('',*,*,#25360,.T.) ;
#34639=ORIENTED_EDGE('',*,*,#25807,.F.) ;
#34640=ORIENTED_EDGE('',*,*,#25810,.T.) ;
#34641=ORIENTED_EDGE('',*,*,#25811,.T.) ;
#34642=ORIENTED_EDGE('',*,*,#25361,.T.) ;
#34643=ORIENTED_EDGE('',*,*,#25809,.F.) ;
#34644=ORIENTED_EDGE('',*,*,#25812,.T.) ;
#34645=ORIENTED_EDGE('',*,*,#25791,.T.) ;
#34646=ORIENTED_EDGE('',*,*,#25362,.T.) ;
#34647=ORIENTED_EDGE('',*,*,#25811,.F.) ;
#34648=ORIENTED_EDGE('',*,*,#25813,.T.) ;
#34649=ORIENTED_EDGE('',*,*,#25814,.T.) ;
#34650=ORIENTED_EDGE('',*,*,#25815,.T.) ;
#34651=ORIENTED_EDGE('',*,*,#25796,.T.) ;
#34652=ORIENTED_EDGE('',*,*,#25352,.T.) ;
#34653=ORIENTED_EDGE('',*,*,#25816,.T.) ;
#34654=ORIENTED_EDGE('',*,*,#25817,.T.) ;
#34655=ORIENTED_EDGE('',*,*,#25794,.T.) ;
#34656=ORIENTED_EDGE('',*,*,#25818,.T.) ;
#34657=ORIENTED_EDGE('',*,*,#25816,.F.) ;
#34658=ORIENTED_EDGE('',*,*,#25819,.T.) ;
#34659=ORIENTED_EDGE('',*,*,#25820,.T.) ;
#34660=ORIENTED_EDGE('',*,*,#25821,.T.) ;
#34661=ORIENTED_EDGE('',*,*,#25822,.T.) ;
#34662=ORIENTED_EDGE('',*,*,#25792,.T.) ;
#34663=ORIENTED_EDGE('',*,*,#25823,.T.) ;
#34664=ORIENTED_EDGE('',*,*,#25821,.F.) ;
#34665=ORIENTED_EDGE('',*,*,#25824,.T.) ;
#34666=ORIENTED_EDGE('',*,*,#25825,.T.) ;
#34667=ORIENTED_EDGE('',*,*,#25826,.F.) ;
#34668=ORIENTED_EDGE('',*,*,#25364,.T.) ;
#34669=ORIENTED_EDGE('',*,*,#25793,.T.) ;
#34670=ORIENTED_EDGE('',*,*,#25827,.T.) ;
#34671=ORIENTED_EDGE('',*,*,#25818,.F.) ;
#34672=ORIENTED_EDGE('',*,*,#25815,.F.) ;
#34673=ORIENTED_EDGE('',*,*,#25828,.T.) ;
#34674=ORIENTED_EDGE('',*,*,#25829,.F.) ;
#34675=ORIENTED_EDGE('',*,*,#25830,.T.) ;
#34676=ORIENTED_EDGE('',*,*,#25831,.T.) ;
#34677=ORIENTED_EDGE('',*,*,#25832,.T.) ;
#34678=ORIENTED_EDGE('',*,*,#25432,.T.) ;
#34679=ORIENTED_EDGE('',*,*,#25833,.T.) ;
#34680=ORIENTED_EDGE('',*,*,#25834,.T.) ;
#34681=ORIENTED_EDGE('',*,*,#25830,.F.) ;
#34682=ORIENTED_EDGE('',*,*,#25445,.T.) ;
#34683=ORIENTED_EDGE('',*,*,#25835,.T.) ;
#34684=ORIENTED_EDGE('',*,*,#25836,.T.) ;
#34685=ORIENTED_EDGE('',*,*,#25837,.T.) ;
#34686=ORIENTED_EDGE('',*,*,#25444,.T.) ;
#34687=ORIENTED_EDGE('',*,*,#25838,.T.) ;
#34688=ORIENTED_EDGE('',*,*,#25839,.T.) ;
#34689=ORIENTED_EDGE('',*,*,#25835,.F.) ;
#34690=ORIENTED_EDGE('',*,*,#25443,.T.) ;
#34691=ORIENTED_EDGE('',*,*,#25840,.T.) ;
#34692=ORIENTED_EDGE('',*,*,#25841,.T.) ;
#34693=ORIENTED_EDGE('',*,*,#25838,.F.) ;
#34694=ORIENTED_EDGE('',*,*,#25442,.T.) ;
#34695=ORIENTED_EDGE('',*,*,#25842,.T.) ;
#34696=ORIENTED_EDGE('',*,*,#25843,.T.) ;
#34697=ORIENTED_EDGE('',*,*,#25840,.F.) ;
#34698=ORIENTED_EDGE('',*,*,#25441,.T.) ;
#34699=ORIENTED_EDGE('',*,*,#25844,.T.) ;
#34700=ORIENTED_EDGE('',*,*,#25845,.T.) ;
#34701=ORIENTED_EDGE('',*,*,#25842,.F.) ;
#34702=ORIENTED_EDGE('',*,*,#25440,.T.) ;
#34703=ORIENTED_EDGE('',*,*,#25837,.F.) ;
#34704=ORIENTED_EDGE('',*,*,#25846,.T.) ;
#34705=ORIENTED_EDGE('',*,*,#25833,.F.) ;
#34706=ORIENTED_EDGE('',*,*,#25847,.T.) ;
#34707=ORIENTED_EDGE('',*,*,#25848,.T.) ;
#34708=ORIENTED_EDGE('',*,*,#25849,.T.) ;
#34709=ORIENTED_EDGE('',*,*,#25439,.T.) ;
#34710=ORIENTED_EDGE('',*,*,#25847,.F.) ;
#34711=ORIENTED_EDGE('',*,*,#25438,.T.) ;
#34712=ORIENTED_EDGE('',*,*,#25850,.T.) ;
#34713=ORIENTED_EDGE('',*,*,#25851,.F.) ;
#34714=ORIENTED_EDGE('',*,*,#25849,.F.) ;
#34715=ORIENTED_EDGE('',*,*,#25852,.T.) ;
#34716=ORIENTED_EDGE('',*,*,#25844,.F.) ;
#34717=ORIENTED_EDGE('',*,*,#25834,.F.) ;
#34718=ORIENTED_EDGE('',*,*,#25853,.F.) ;
#34719=ORIENTED_EDGE('',*,*,#25854,.F.) ;
#34720=ORIENTED_EDGE('',*,*,#25855,.F.) ;
#34721=ORIENTED_EDGE('',*,*,#25846,.F.) ;
#34722=ORIENTED_EDGE('',*,*,#25856,.T.) ;
#34723=ORIENTED_EDGE('',*,*,#25857,.T.) ;
#34724=ORIENTED_EDGE('',*,*,#25853,.T.) ;
#34725=ORIENTED_EDGE('',*,*,#25836,.F.) ;
#34726=ORIENTED_EDGE('',*,*,#25858,.F.) ;
#34727=ORIENTED_EDGE('',*,*,#25859,.F.) ;
#34728=ORIENTED_EDGE('',*,*,#25856,.F.) ;
#34729=ORIENTED_EDGE('',*,*,#25839,.F.) ;
#34730=ORIENTED_EDGE('',*,*,#25860,.T.) ;
#34731=ORIENTED_EDGE('',*,*,#25861,.T.) ;
#34732=ORIENTED_EDGE('',*,*,#25858,.T.) ;
#34733=ORIENTED_EDGE('',*,*,#25841,.F.) ;
#34734=ORIENTED_EDGE('',*,*,#25862,.F.) ;
#34735=ORIENTED_EDGE('',*,*,#25863,.F.) ;
#34736=ORIENTED_EDGE('',*,*,#25860,.F.) ;
#34737=ORIENTED_EDGE('',*,*,#25843,.F.) ;
#34738=ORIENTED_EDGE('',*,*,#25864,.T.) ;
#34739=ORIENTED_EDGE('',*,*,#25865,.T.) ;
#34740=ORIENTED_EDGE('',*,*,#25862,.T.) ;
#34741=ORIENTED_EDGE('',*,*,#25845,.F.) ;
#34742=ORIENTED_EDGE('',*,*,#25866,.F.) ;
#34743=ORIENTED_EDGE('',*,*,#25867,.F.) ;
#34744=ORIENTED_EDGE('',*,*,#25864,.F.) ;
#34745=ORIENTED_EDGE('',*,*,#25852,.F.) ;
#34746=ORIENTED_EDGE('',*,*,#25868,.T.) ;
#34747=ORIENTED_EDGE('',*,*,#25869,.T.) ;
#34748=ORIENTED_EDGE('',*,*,#25866,.T.) ;
#34749=ORIENTED_EDGE('',*,*,#25848,.F.) ;
#34750=ORIENTED_EDGE('',*,*,#25870,.F.) ;
#34751=ORIENTED_EDGE('',*,*,#25871,.F.) ;
#34752=ORIENTED_EDGE('',*,*,#25868,.F.) ;
#34753=ORIENTED_EDGE('',*,*,#25872,.T.) ;
#34754=ORIENTED_EDGE('',*,*,#25873,.T.) ;
#34755=ORIENTED_EDGE('',*,*,#25874,.T.) ;
#34756=ORIENTED_EDGE('',*,*,#25418,.T.) ;
#34757=ORIENTED_EDGE('',*,*,#25875,.T.) ;
#34758=ORIENTED_EDGE('',*,*,#25876,.T.) ;
#34759=ORIENTED_EDGE('',*,*,#25872,.F.) ;
#34760=ORIENTED_EDGE('',*,*,#25431,.T.) ;
#34761=ORIENTED_EDGE('',*,*,#25877,.T.) ;
#34762=ORIENTED_EDGE('',*,*,#25878,.T.) ;
#34763=ORIENTED_EDGE('',*,*,#25879,.T.) ;
#34764=ORIENTED_EDGE('',*,*,#25430,.T.) ;
#34765=ORIENTED_EDGE('',*,*,#25880,.T.) ;
#34766=ORIENTED_EDGE('',*,*,#25881,.T.) ;
#34767=ORIENTED_EDGE('',*,*,#25877,.F.) ;
#34768=ORIENTED_EDGE('',*,*,#25429,.T.) ;
#34769=ORIENTED_EDGE('',*,*,#25882,.T.) ;
#34770=ORIENTED_EDGE('',*,*,#25883,.T.) ;
#34771=ORIENTED_EDGE('',*,*,#25880,.F.) ;
#34772=ORIENTED_EDGE('',*,*,#25428,.T.) ;
#34773=ORIENTED_EDGE('',*,*,#25884,.T.) ;
#34774=ORIENTED_EDGE('',*,*,#25885,.T.) ;
#34775=ORIENTED_EDGE('',*,*,#25882,.F.) ;
#34776=ORIENTED_EDGE('',*,*,#25427,.T.) ;
#34777=ORIENTED_EDGE('',*,*,#25886,.T.) ;
#34778=ORIENTED_EDGE('',*,*,#25887,.T.) ;
#34779=ORIENTED_EDGE('',*,*,#25884,.F.) ;
#34780=ORIENTED_EDGE('',*,*,#25426,.T.) ;
#34781=ORIENTED_EDGE('',*,*,#25879,.F.) ;
#34782=ORIENTED_EDGE('',*,*,#25888,.T.) ;
#34783=ORIENTED_EDGE('',*,*,#25875,.F.) ;
#34784=ORIENTED_EDGE('',*,*,#25889,.T.) ;
#34785=ORIENTED_EDGE('',*,*,#25890,.T.) ;
#34786=ORIENTED_EDGE('',*,*,#25891,.T.) ;
#34787=ORIENTED_EDGE('',*,*,#25425,.T.) ;
#34788=ORIENTED_EDGE('',*,*,#25889,.F.) ;
#34789=ORIENTED_EDGE('',*,*,#25424,.T.) ;
#34790=ORIENTED_EDGE('',*,*,#25892,.T.) ;
#34791=ORIENTED_EDGE('',*,*,#25893,.F.) ;
#34792=ORIENTED_EDGE('',*,*,#25891,.F.) ;
#34793=ORIENTED_EDGE('',*,*,#25894,.T.) ;
#34794=ORIENTED_EDGE('',*,*,#25886,.F.) ;
#34795=ORIENTED_EDGE('',*,*,#25876,.F.) ;
#34796=ORIENTED_EDGE('',*,*,#25895,.F.) ;
#34797=ORIENTED_EDGE('',*,*,#25896,.F.) ;
#34798=ORIENTED_EDGE('',*,*,#25897,.F.) ;
#34799=ORIENTED_EDGE('',*,*,#25888,.F.) ;
#34800=ORIENTED_EDGE('',*,*,#25898,.T.) ;
#34801=ORIENTED_EDGE('',*,*,#25899,.T.) ;
#34802=ORIENTED_EDGE('',*,*,#25895,.T.) ;
#34803=ORIENTED_EDGE('',*,*,#25878,.F.) ;
#34804=ORIENTED_EDGE('',*,*,#25900,.F.) ;
#34805=ORIENTED_EDGE('',*,*,#25901,.F.) ;
#34806=ORIENTED_EDGE('',*,*,#25898,.F.) ;
#34807=ORIENTED_EDGE('',*,*,#25881,.F.) ;
#34808=ORIENTED_EDGE('',*,*,#25902,.T.) ;
#34809=ORIENTED_EDGE('',*,*,#25903,.T.) ;
#34810=ORIENTED_EDGE('',*,*,#25900,.T.) ;
#34811=ORIENTED_EDGE('',*,*,#25883,.F.) ;
#34812=ORIENTED_EDGE('',*,*,#25904,.F.) ;
#34813=ORIENTED_EDGE('',*,*,#25905,.F.) ;
#34814=ORIENTED_EDGE('',*,*,#25902,.F.) ;
#34815=ORIENTED_EDGE('',*,*,#25885,.F.) ;
#34816=ORIENTED_EDGE('',*,*,#25906,.T.) ;
#34817=ORIENTED_EDGE('',*,*,#25907,.T.) ;
#34818=ORIENTED_EDGE('',*,*,#25904,.T.) ;
#34819=ORIENTED_EDGE('',*,*,#25887,.F.) ;
#34820=ORIENTED_EDGE('',*,*,#25908,.F.) ;
#34821=ORIENTED_EDGE('',*,*,#25909,.F.) ;
#34822=ORIENTED_EDGE('',*,*,#25906,.F.) ;
#34823=ORIENTED_EDGE('',*,*,#25894,.F.) ;
#34824=ORIENTED_EDGE('',*,*,#25910,.T.) ;
#34825=ORIENTED_EDGE('',*,*,#25911,.T.) ;
#34826=ORIENTED_EDGE('',*,*,#25908,.T.) ;
#34827=ORIENTED_EDGE('',*,*,#25890,.F.) ;
#34828=ORIENTED_EDGE('',*,*,#25912,.F.) ;
#34829=ORIENTED_EDGE('',*,*,#25913,.F.) ;
#34830=ORIENTED_EDGE('',*,*,#25910,.F.) ;
#34831=ORIENTED_EDGE('',*,*,#25668,.F.) ;
#34832=ORIENTED_EDGE('',*,*,#25416,.T.) ;
#34833=ORIENTED_EDGE('',*,*,#25914,.T.) ;
#34834=ORIENTED_EDGE('',*,*,#25682,.T.) ;
#34835=ORIENTED_EDGE('',*,*,#25915,.T.) ;
#34836=ORIENTED_EDGE('',*,*,#25916,.T.) ;
#34837=ORIENTED_EDGE('',*,*,#25917,.T.) ;
#34838=ORIENTED_EDGE('',*,*,#25415,.T.) ;
#34839=ORIENTED_EDGE('',*,*,#25915,.F.) ;
#34840=ORIENTED_EDGE('',*,*,#25414,.T.) ;
#34841=ORIENTED_EDGE('',*,*,#25918,.T.) ;
#34842=ORIENTED_EDGE('',*,*,#25919,.F.) ;
#34843=ORIENTED_EDGE('',*,*,#25917,.F.) ;
#34844=ORIENTED_EDGE('',*,*,#25680,.T.) ;
#34845=ORIENTED_EDGE('',*,*,#25914,.F.) ;
#34846=ORIENTED_EDGE('',*,*,#25916,.F.) ;
#34847=ORIENTED_EDGE('',*,*,#25920,.F.) ;
#34848=ORIENTED_EDGE('',*,*,#25677,.F.) ;
#34849=ORIENTED_EDGE('',*,*,#25681,.F.) ;
#34850=ORIENTED_EDGE('',*,*,#25649,.F.) ;
#34851=ORIENTED_EDGE('',*,*,#25406,.T.) ;
#34852=ORIENTED_EDGE('',*,*,#25661,.F.) ;
#34853=ORIENTED_EDGE('',*,*,#25921,.T.) ;
#34854=ORIENTED_EDGE('',*,*,#25675,.F.) ;
#34855=ORIENTED_EDGE('',*,*,#25922,.T.) ;
#34856=ORIENTED_EDGE('',*,*,#25923,.T.) ;
#34857=ORIENTED_EDGE('',*,*,#25408,.T.) ;
#34858=ORIENTED_EDGE('',*,*,#25650,.F.) ;
#34859=ORIENTED_EDGE('',*,*,#25921,.F.) ;
#34860=ORIENTED_EDGE('',*,*,#25663,.F.) ;
#34861=ORIENTED_EDGE('',*,*,#25659,.F.) ;
#34862=ORIENTED_EDGE('',*,*,#25684,.F.) ;
#34863=ORIENTED_EDGE('',*,*,#25924,.T.) ;
#34864=ORIENTED_EDGE('',*,*,#25925,.T.) ;
#34865=ORIENTED_EDGE('',*,*,#25394,.T.) ;
#34866=ORIENTED_EDGE('',*,*,#25926,.T.) ;
#34867=ORIENTED_EDGE('',*,*,#25395,.T.) ;
#34868=ORIENTED_EDGE('',*,*,#25925,.F.) ;
#34869=ORIENTED_EDGE('',*,*,#25927,.T.) ;
#34870=ORIENTED_EDGE('',*,*,#25928,.T.) ;
#34871=ORIENTED_EDGE('',*,*,#25396,.T.) ;
#34872=ORIENTED_EDGE('',*,*,#25926,.F.) ;
#34873=ORIENTED_EDGE('',*,*,#25929,.T.) ;
#34874=ORIENTED_EDGE('',*,*,#25930,.T.) ;
#34875=ORIENTED_EDGE('',*,*,#25397,.T.) ;
#34876=ORIENTED_EDGE('',*,*,#25928,.F.) ;
#34877=ORIENTED_EDGE('',*,*,#25931,.T.) ;
#34878=ORIENTED_EDGE('',*,*,#25932,.T.) ;
#34879=ORIENTED_EDGE('',*,*,#25398,.T.) ;
#34880=ORIENTED_EDGE('',*,*,#25930,.F.) ;
#34881=ORIENTED_EDGE('',*,*,#25933,.T.) ;
#34882=ORIENTED_EDGE('',*,*,#25934,.T.) ;
#34883=ORIENTED_EDGE('',*,*,#25399,.T.) ;
#34884=ORIENTED_EDGE('',*,*,#25932,.F.) ;
#34885=ORIENTED_EDGE('',*,*,#25935,.T.) ;
#34886=ORIENTED_EDGE('',*,*,#25936,.T.) ;
#34887=ORIENTED_EDGE('',*,*,#25400,.T.) ;
#34888=ORIENTED_EDGE('',*,*,#25934,.F.) ;
#34889=ORIENTED_EDGE('',*,*,#25937,.T.) ;
#34890=ORIENTED_EDGE('',*,*,#25938,.T.) ;
#34891=ORIENTED_EDGE('',*,*,#25401,.T.) ;
#34892=ORIENTED_EDGE('',*,*,#25936,.F.) ;
#34893=ORIENTED_EDGE('',*,*,#25939,.T.) ;
#34894=ORIENTED_EDGE('',*,*,#25700,.F.) ;
#34895=ORIENTED_EDGE('',*,*,#25402,.T.) ;
#34896=ORIENTED_EDGE('',*,*,#25938,.F.) ;
#34897=ORIENTED_EDGE('',*,*,#25940,.T.) ;
#34898=ORIENTED_EDGE('',*,*,#25698,.F.) ;
#34899=ORIENTED_EDGE('',*,*,#25940,.F.) ;
#34900=ORIENTED_EDGE('',*,*,#25941,.F.) ;
#34901=ORIENTED_EDGE('',*,*,#25942,.F.) ;
#34902=ORIENTED_EDGE('',*,*,#25939,.F.) ;
#34903=ORIENTED_EDGE('',*,*,#25943,.T.) ;
#34904=ORIENTED_EDGE('',*,*,#25944,.T.) ;
#34905=ORIENTED_EDGE('',*,*,#25941,.T.) ;
#34906=ORIENTED_EDGE('',*,*,#25937,.F.) ;
#34907=ORIENTED_EDGE('',*,*,#25945,.F.) ;
#34908=ORIENTED_EDGE('',*,*,#25946,.F.) ;
#34909=ORIENTED_EDGE('',*,*,#25943,.F.) ;
#34910=ORIENTED_EDGE('',*,*,#25935,.F.) ;
#34911=ORIENTED_EDGE('',*,*,#25947,.T.) ;
#34912=ORIENTED_EDGE('',*,*,#25948,.T.) ;
#34913=ORIENTED_EDGE('',*,*,#25945,.T.) ;
#34914=ORIENTED_EDGE('',*,*,#25933,.F.) ;
#34915=ORIENTED_EDGE('',*,*,#25949,.F.) ;
#34916=ORIENTED_EDGE('',*,*,#25950,.F.) ;
#34917=ORIENTED_EDGE('',*,*,#25947,.F.) ;
#34918=ORIENTED_EDGE('',*,*,#25931,.F.) ;
#34919=ORIENTED_EDGE('',*,*,#25951,.T.) ;
#34920=ORIENTED_EDGE('',*,*,#25952,.T.) ;
#34921=ORIENTED_EDGE('',*,*,#25949,.T.) ;
#34922=ORIENTED_EDGE('',*,*,#25929,.F.) ;
#34923=ORIENTED_EDGE('',*,*,#25953,.F.) ;
#34924=ORIENTED_EDGE('',*,*,#25954,.F.) ;
#34925=ORIENTED_EDGE('',*,*,#25951,.F.) ;
#34926=ORIENTED_EDGE('',*,*,#25927,.F.) ;
#34927=ORIENTED_EDGE('',*,*,#25955,.T.) ;
#34928=ORIENTED_EDGE('',*,*,#25956,.T.) ;
#34929=ORIENTED_EDGE('',*,*,#25953,.T.) ;
#34930=ORIENTED_EDGE('',*,*,#25687,.F.) ;
#34931=ORIENTED_EDGE('',*,*,#25957,.F.) ;
#34932=ORIENTED_EDGE('',*,*,#25955,.F.) ;
#34933=ORIENTED_EDGE('',*,*,#25924,.F.) ;
#34934=ORIENTED_EDGE('',*,*,#25646,.T.) ;
#34935=ORIENTED_EDGE('',*,*,#25958,.T.) ;
#34936=ORIENTED_EDGE('',*,*,#25922,.F.) ;
#34937=ORIENTED_EDGE('',*,*,#25676,.T.) ;
#34938=ORIENTED_EDGE('',*,*,#25959,.F.) ;
#34939=ORIENTED_EDGE('',*,*,#25960,.T.) ;
#34940=ORIENTED_EDGE('',*,*,#25961,.T.) ;
#34941=ORIENTED_EDGE('',*,*,#25412,.T.) ;
#34942=ORIENTED_EDGE('',*,*,#25962,.F.) ;
#34943=ORIENTED_EDGE('',*,*,#25963,.F.) ;
#34944=ORIENTED_EDGE('',*,*,#25964,.F.) ;
#34945=ORIENTED_EDGE('',*,*,#25965,.F.) ;
#34946=ORIENTED_EDGE('',*,*,#25166,.T.) ;
#34947=ORIENTED_EDGE('',*,*,#25678,.F.) ;
#34948=ORIENTED_EDGE('',*,*,#25966,.F.) ;
#34949=ORIENTED_EDGE('',*,*,#25967,.F.) ;
#34950=ORIENTED_EDGE('',*,*,#25919,.T.) ;
#34951=ORIENTED_EDGE('',*,*,#25968,.T.) ;
#34952=ORIENTED_EDGE('',*,*,#25966,.T.) ;
#34953=ORIENTED_EDGE('',*,*,#25920,.T.) ;
#34954=ORIENTED_EDGE('',*,*,#25170,.T.) ;
#34955=ORIENTED_EDGE('',*,*,#25969,.F.) ;
#34956=ORIENTED_EDGE('',*,*,#25970,.F.) ;
#34957=ORIENTED_EDGE('',*,*,#25971,.F.) ;
#34958=ORIENTED_EDGE('',*,*,#25168,.T.) ;
#34959=ORIENTED_EDGE('',*,*,#25972,.F.) ;
#34960=ORIENTED_EDGE('',*,*,#25973,.F.) ;
#34961=ORIENTED_EDGE('',*,*,#25974,.F.) ;
#34962=ORIENTED_EDGE('',*,*,#25972,.T.) ;
#34963=ORIENTED_EDGE('',*,*,#25167,.T.) ;
#34964=ORIENTED_EDGE('',*,*,#25967,.T.) ;
#34965=ORIENTED_EDGE('',*,*,#25975,.T.) ;
#34966=ORIENTED_EDGE('',*,*,#25973,.T.) ;
#34967=ORIENTED_EDGE('',*,*,#25976,.T.) ;
#34968=ORIENTED_EDGE('',*,*,#25960,.F.) ;
#34969=ORIENTED_EDGE('',*,*,#25965,.T.) ;
#34970=ORIENTED_EDGE('',*,*,#25969,.T.) ;
#34971=ORIENTED_EDGE('',*,*,#25169,.T.) ;
#34972=ORIENTED_EDGE('',*,*,#25974,.T.) ;
#34973=ORIENTED_EDGE('',*,*,#25964,.T.) ;
#34974=ORIENTED_EDGE('',*,*,#25977,.F.) ;
#34975=ORIENTED_EDGE('',*,*,#25978,.F.) ;
#34976=ORIENTED_EDGE('',*,*,#25410,.T.) ;
#34977=ORIENTED_EDGE('',*,*,#25979,.F.) ;
#34978=ORIENTED_EDGE('',*,*,#25411,.T.) ;
#34979=ORIENTED_EDGE('',*,*,#25978,.T.) ;
#34980=ORIENTED_EDGE('',*,*,#25962,.T.) ;
#34981=ORIENTED_EDGE('',*,*,#25959,.T.) ;
#34982=ORIENTED_EDGE('',*,*,#25923,.F.) ;
#34983=ORIENTED_EDGE('',*,*,#25980,.T.) ;
#34984=ORIENTED_EDGE('',*,*,#25979,.T.) ;
#34985=ORIENTED_EDGE('',*,*,#25409,.T.) ;
#34986=ORIENTED_EDGE('',*,*,#25970,.T.) ;
#34987=ORIENTED_EDGE('',*,*,#25963,.T.) ;
#34988=ORIENTED_EDGE('',*,*,#25977,.T.) ;
#34989=ORIENTED_EDGE('',*,*,#25981,.T.) ;
#34990=ORIENTED_EDGE('',*,*,#25645,.F.) ;
#34991=ORIENTED_EDGE('',*,*,#25171,.T.) ;
#34992=ORIENTED_EDGE('',*,*,#25971,.T.) ;
#34993=ORIENTED_EDGE('',*,*,#25982,.T.) ;
#34994=ORIENTED_EDGE('',*,*,#25976,.F.) ;
#34995=ORIENTED_EDGE('',*,*,#25975,.F.) ;
#34996=ORIENTED_EDGE('',*,*,#25968,.F.) ;
#34997=ORIENTED_EDGE('',*,*,#25983,.F.) ;
#34998=ORIENTED_EDGE('',*,*,#25961,.F.) ;
#34999=ORIENTED_EDGE('',*,*,#25983,.T.) ;
#35000=ORIENTED_EDGE('',*,*,#25918,.F.) ;
#35001=ORIENTED_EDGE('',*,*,#25413,.T.) ;
#35002=ORIENTED_EDGE('',*,*,#25984,.T.) ;
#35003=ORIENTED_EDGE('',*,*,#25434,.T.) ;
#35004=ORIENTED_EDGE('',*,*,#25985,.T.) ;
#35005=ORIENTED_EDGE('',*,*,#25986,.F.) ;
#35006=ORIENTED_EDGE('',*,*,#25987,.F.) ;
#35007=ORIENTED_EDGE('',*,*,#25988,.T.) ;
#35008=ORIENTED_EDGE('',*,*,#25989,.T.) ;
#35009=ORIENTED_EDGE('',*,*,#25436,.T.) ;
#35010=ORIENTED_EDGE('',*,*,#25990,.F.) ;
#35011=ORIENTED_EDGE('',*,*,#25991,.F.) ;
#35012=ORIENTED_EDGE('',*,*,#25992,.F.) ;
#35013=ORIENTED_EDGE('',*,*,#25993,.F.) ;
#35014=ORIENTED_EDGE('',*,*,#25861,.F.) ;
#35015=ORIENTED_EDGE('',*,*,#25994,.F.) ;
#35016=ORIENTED_EDGE('',*,*,#25121,.T.) ;
#35017=ORIENTED_EDGE('',*,*,#25995,.F.) ;
#35018=ORIENTED_EDGE('',*,*,#25123,.T.) ;
#35019=ORIENTED_EDGE('',*,*,#25996,.F.) ;
#35020=ORIENTED_EDGE('',*,*,#25865,.F.) ;
#35021=ORIENTED_EDGE('',*,*,#25997,.F.) ;
#35022=ORIENTED_EDGE('',*,*,#25996,.T.) ;
#35023=ORIENTED_EDGE('',*,*,#25122,.T.) ;
#35024=ORIENTED_EDGE('',*,*,#25994,.T.) ;
#35025=ORIENTED_EDGE('',*,*,#25863,.T.) ;
#35026=ORIENTED_EDGE('',*,*,#25998,.F.) ;
#35027=ORIENTED_EDGE('',*,*,#25999,.F.) ;
#35028=ORIENTED_EDGE('',*,*,#25857,.F.) ;
#35029=ORIENTED_EDGE('',*,*,#26000,.F.) ;
#35030=ORIENTED_EDGE('',*,*,#26001,.F.) ;
#35031=ORIENTED_EDGE('',*,*,#25869,.F.) ;
#35032=ORIENTED_EDGE('',*,*,#26001,.T.) ;
#35033=ORIENTED_EDGE('',*,*,#25124,.T.) ;
#35034=ORIENTED_EDGE('',*,*,#25997,.T.) ;
#35035=ORIENTED_EDGE('',*,*,#25867,.T.) ;
#35036=ORIENTED_EDGE('',*,*,#25118,.T.) ;
#35037=ORIENTED_EDGE('',*,*,#26002,.F.) ;
#35038=ORIENTED_EDGE('',*,*,#26003,.F.) ;
#35039=ORIENTED_EDGE('',*,*,#26004,.F.) ;
#35040=ORIENTED_EDGE('',*,*,#25126,.T.) ;
#35041=ORIENTED_EDGE('',*,*,#26005,.F.) ;
#35042=ORIENTED_EDGE('',*,*,#26006,.F.) ;
#35043=ORIENTED_EDGE('',*,*,#26007,.F.) ;
#35044=ORIENTED_EDGE('',*,*,#26005,.T.) ;
#35045=ORIENTED_EDGE('',*,*,#25125,.T.) ;
#35046=ORIENTED_EDGE('',*,*,#26000,.T.) ;
#35047=ORIENTED_EDGE('',*,*,#25871,.T.) ;
#35048=ORIENTED_EDGE('',*,*,#25851,.T.) ;
#35049=ORIENTED_EDGE('',*,*,#26008,.T.) ;
#35050=ORIENTED_EDGE('',*,*,#26006,.T.) ;
#35051=ORIENTED_EDGE('',*,*,#25870,.T.) ;
#35052=ORIENTED_EDGE('',*,*,#25116,.T.) ;
#35053=ORIENTED_EDGE('',*,*,#26009,.F.) ;
#35054=ORIENTED_EDGE('',*,*,#26010,.F.) ;
#35055=ORIENTED_EDGE('',*,*,#26011,.F.) ;
#35056=ORIENTED_EDGE('',*,*,#25114,.T.) ;
#35057=ORIENTED_EDGE('',*,*,#26012,.F.) ;
#35058=ORIENTED_EDGE('',*,*,#26013,.F.) ;
#35059=ORIENTED_EDGE('',*,*,#26014,.F.) ;
#35060=ORIENTED_EDGE('',*,*,#26012,.T.) ;
#35061=ORIENTED_EDGE('',*,*,#25127,.T.) ;
#35062=ORIENTED_EDGE('',*,*,#26007,.T.) ;
#35063=ORIENTED_EDGE('',*,*,#26015,.T.) ;
#35064=ORIENTED_EDGE('',*,*,#26013,.T.) ;
#35065=ORIENTED_EDGE('',*,*,#26016,.T.) ;
#35066=ORIENTED_EDGE('',*,*,#25988,.F.) ;
#35067=ORIENTED_EDGE('',*,*,#25993,.T.) ;
#35068=ORIENTED_EDGE('',*,*,#26009,.T.) ;
#35069=ORIENTED_EDGE('',*,*,#25115,.T.) ;
#35070=ORIENTED_EDGE('',*,*,#26014,.T.) ;
#35071=ORIENTED_EDGE('',*,*,#25992,.T.) ;
#35072=ORIENTED_EDGE('',*,*,#25986,.T.) ;
#35073=ORIENTED_EDGE('',*,*,#26017,.T.) ;
#35074=ORIENTED_EDGE('',*,*,#26010,.T.) ;
#35075=ORIENTED_EDGE('',*,*,#25991,.T.) ;
#35076=ORIENTED_EDGE('',*,*,#26002,.T.) ;
#35077=ORIENTED_EDGE('',*,*,#25117,.T.) ;
#35078=ORIENTED_EDGE('',*,*,#26011,.T.) ;
#35079=ORIENTED_EDGE('',*,*,#26018,.T.) ;
#35080=ORIENTED_EDGE('',*,*,#26003,.T.) ;
#35081=ORIENTED_EDGE('',*,*,#26019,.T.) ;
#35082=ORIENTED_EDGE('',*,*,#25831,.F.) ;
#35083=ORIENTED_EDGE('',*,*,#25855,.T.) ;
#35084=ORIENTED_EDGE('',*,*,#25999,.T.) ;
#35085=ORIENTED_EDGE('',*,*,#25119,.T.) ;
#35086=ORIENTED_EDGE('',*,*,#26004,.T.) ;
#35087=ORIENTED_EDGE('',*,*,#25854,.T.) ;
#35088=ORIENTED_EDGE('',*,*,#25995,.T.) ;
#35089=ORIENTED_EDGE('',*,*,#25120,.T.) ;
#35090=ORIENTED_EDGE('',*,*,#25998,.T.) ;
#35091=ORIENTED_EDGE('',*,*,#25859,.T.) ;
#35092=ORIENTED_EDGE('',*,*,#25435,.T.) ;
#35093=ORIENTED_EDGE('',*,*,#25984,.F.) ;
#35094=ORIENTED_EDGE('',*,*,#25990,.T.) ;
#35095=ORIENTED_EDGE('',*,*,#25987,.T.) ;
#35096=ORIENTED_EDGE('',*,*,#26016,.F.) ;
#35097=ORIENTED_EDGE('',*,*,#26015,.F.) ;
#35098=ORIENTED_EDGE('',*,*,#26008,.F.) ;
#35099=ORIENTED_EDGE('',*,*,#26020,.F.) ;
#35100=ORIENTED_EDGE('',*,*,#25989,.F.) ;
#35101=ORIENTED_EDGE('',*,*,#26020,.T.) ;
#35102=ORIENTED_EDGE('',*,*,#25850,.F.) ;
#35103=ORIENTED_EDGE('',*,*,#25437,.T.) ;
#35104=ORIENTED_EDGE('',*,*,#26021,.T.) ;
#35105=ORIENTED_EDGE('',*,*,#25420,.T.) ;
#35106=ORIENTED_EDGE('',*,*,#26022,.T.) ;
#35107=ORIENTED_EDGE('',*,*,#26023,.F.) ;
#35108=ORIENTED_EDGE('',*,*,#26024,.F.) ;
#35109=ORIENTED_EDGE('',*,*,#26025,.T.) ;
#35110=ORIENTED_EDGE('',*,*,#26026,.T.) ;
#35111=ORIENTED_EDGE('',*,*,#25422,.T.) ;
#35112=ORIENTED_EDGE('',*,*,#26027,.F.) ;
#35113=ORIENTED_EDGE('',*,*,#26028,.F.) ;
#35114=ORIENTED_EDGE('',*,*,#26029,.F.) ;
#35115=ORIENTED_EDGE('',*,*,#26030,.F.) ;
#35116=ORIENTED_EDGE('',*,*,#25235,.T.) ;
#35117=ORIENTED_EDGE('',*,*,#26031,.F.) ;
#35118=ORIENTED_EDGE('',*,*,#25903,.F.) ;
#35119=ORIENTED_EDGE('',*,*,#26032,.F.) ;
#35120=ORIENTED_EDGE('',*,*,#25899,.F.) ;
#35121=ORIENTED_EDGE('',*,*,#26033,.F.) ;
#35122=ORIENTED_EDGE('',*,*,#26034,.F.) ;
#35123=ORIENTED_EDGE('',*,*,#26031,.T.) ;
#35124=ORIENTED_EDGE('',*,*,#25234,.T.) ;
#35125=ORIENTED_EDGE('',*,*,#26033,.T.) ;
#35126=ORIENTED_EDGE('',*,*,#25901,.T.) ;
#35127=ORIENTED_EDGE('',*,*,#25237,.T.) ;
#35128=ORIENTED_EDGE('',*,*,#26035,.F.) ;
#35129=ORIENTED_EDGE('',*,*,#25907,.F.) ;
#35130=ORIENTED_EDGE('',*,*,#26036,.F.) ;
#35131=ORIENTED_EDGE('',*,*,#26035,.T.) ;
#35132=ORIENTED_EDGE('',*,*,#25236,.T.) ;
#35133=ORIENTED_EDGE('',*,*,#26032,.T.) ;
#35134=ORIENTED_EDGE('',*,*,#25905,.T.) ;
#35135=ORIENTED_EDGE('',*,*,#25232,.T.) ;
#35136=ORIENTED_EDGE('',*,*,#26037,.F.) ;
#35137=ORIENTED_EDGE('',*,*,#26038,.F.) ;
#35138=ORIENTED_EDGE('',*,*,#26039,.F.) ;
#35139=ORIENTED_EDGE('',*,*,#26040,.F.) ;
#35140=ORIENTED_EDGE('',*,*,#26041,.F.) ;
#35141=ORIENTED_EDGE('',*,*,#25911,.F.) ;
#35142=ORIENTED_EDGE('',*,*,#26041,.T.) ;
#35143=ORIENTED_EDGE('',*,*,#25238,.T.) ;
#35144=ORIENTED_EDGE('',*,*,#26036,.T.) ;
#35145=ORIENTED_EDGE('',*,*,#25909,.T.) ;
#35146=ORIENTED_EDGE('',*,*,#25230,.T.) ;
#35147=ORIENTED_EDGE('',*,*,#26042,.F.) ;
#35148=ORIENTED_EDGE('',*,*,#26043,.F.) ;
#35149=ORIENTED_EDGE('',*,*,#26044,.F.) ;
#35150=ORIENTED_EDGE('',*,*,#25240,.T.) ;
#35151=ORIENTED_EDGE('',*,*,#26045,.F.) ;
#35152=ORIENTED_EDGE('',*,*,#26046,.F.) ;
#35153=ORIENTED_EDGE('',*,*,#26047,.F.) ;
#35154=ORIENTED_EDGE('',*,*,#26045,.T.) ;
#35155=ORIENTED_EDGE('',*,*,#25239,.T.) ;
#35156=ORIENTED_EDGE('',*,*,#26040,.T.) ;
#35157=ORIENTED_EDGE('',*,*,#25913,.T.) ;
#35158=ORIENTED_EDGE('',*,*,#25893,.T.) ;
#35159=ORIENTED_EDGE('',*,*,#26048,.T.) ;
#35160=ORIENTED_EDGE('',*,*,#26046,.T.) ;
#35161=ORIENTED_EDGE('',*,*,#25912,.T.) ;
#35162=ORIENTED_EDGE('',*,*,#25228,.T.) ;
#35163=ORIENTED_EDGE('',*,*,#26049,.F.) ;
#35164=ORIENTED_EDGE('',*,*,#26050,.F.) ;
#35165=ORIENTED_EDGE('',*,*,#26051,.F.) ;
#35166=ORIENTED_EDGE('',*,*,#26049,.T.) ;
#35167=ORIENTED_EDGE('',*,*,#25241,.T.) ;
#35168=ORIENTED_EDGE('',*,*,#26047,.T.) ;
#35169=ORIENTED_EDGE('',*,*,#26052,.T.) ;
#35170=ORIENTED_EDGE('',*,*,#26050,.T.) ;
#35171=ORIENTED_EDGE('',*,*,#26053,.T.) ;
#35172=ORIENTED_EDGE('',*,*,#26025,.F.) ;
#35173=ORIENTED_EDGE('',*,*,#26030,.T.) ;
#35174=ORIENTED_EDGE('',*,*,#26042,.T.) ;
#35175=ORIENTED_EDGE('',*,*,#25229,.T.) ;
#35176=ORIENTED_EDGE('',*,*,#26051,.T.) ;
#35177=ORIENTED_EDGE('',*,*,#26029,.T.) ;
#35178=ORIENTED_EDGE('',*,*,#26023,.T.) ;
#35179=ORIENTED_EDGE('',*,*,#26054,.T.) ;
#35180=ORIENTED_EDGE('',*,*,#26043,.T.) ;
#35181=ORIENTED_EDGE('',*,*,#26028,.T.) ;
#35182=ORIENTED_EDGE('',*,*,#26037,.T.) ;
#35183=ORIENTED_EDGE('',*,*,#25231,.T.) ;
#35184=ORIENTED_EDGE('',*,*,#26044,.T.) ;
#35185=ORIENTED_EDGE('',*,*,#26055,.T.) ;
#35186=ORIENTED_EDGE('',*,*,#26038,.T.) ;
#35187=ORIENTED_EDGE('',*,*,#26056,.T.) ;
#35188=ORIENTED_EDGE('',*,*,#25873,.F.) ;
#35189=ORIENTED_EDGE('',*,*,#25897,.T.) ;
#35190=ORIENTED_EDGE('',*,*,#26034,.T.) ;
#35191=ORIENTED_EDGE('',*,*,#25233,.T.) ;
#35192=ORIENTED_EDGE('',*,*,#26039,.T.) ;
#35193=ORIENTED_EDGE('',*,*,#25896,.T.) ;
#35194=ORIENTED_EDGE('',*,*,#25421,.T.) ;
#35195=ORIENTED_EDGE('',*,*,#26021,.F.) ;
#35196=ORIENTED_EDGE('',*,*,#26027,.T.) ;
#35197=ORIENTED_EDGE('',*,*,#26024,.T.) ;
#35198=ORIENTED_EDGE('',*,*,#26053,.F.) ;
#35199=ORIENTED_EDGE('',*,*,#26052,.F.) ;
#35200=ORIENTED_EDGE('',*,*,#26048,.F.) ;
#35201=ORIENTED_EDGE('',*,*,#26057,.F.) ;
#35202=ORIENTED_EDGE('',*,*,#26026,.F.) ;
#35203=ORIENTED_EDGE('',*,*,#26057,.T.) ;
#35204=ORIENTED_EDGE('',*,*,#25892,.F.) ;
#35205=ORIENTED_EDGE('',*,*,#25423,.T.) ;
#35206=ORIENTED_EDGE('',*,*,#25083,.T.) ;
#35207=ORIENTED_EDGE('',*,*,#26058,.F.) ;
#35208=ORIENTED_EDGE('',*,*,#26059,.F.) ;
#35209=ORIENTED_EDGE('',*,*,#26060,.F.) ;
#35210=ORIENTED_EDGE('',*,*,#25081,.T.) ;
#35211=ORIENTED_EDGE('',*,*,#26061,.F.) ;
#35212=ORIENTED_EDGE('',*,*,#26062,.F.) ;
#35213=ORIENTED_EDGE('',*,*,#26063,.F.) ;
#35214=ORIENTED_EDGE('',*,*,#26064,.T.) ;
#35215=ORIENTED_EDGE('',*,*,#25515,.T.) ;
#35216=ORIENTED_EDGE('',*,*,#26065,.T.) ;
#35217=ORIENTED_EDGE('',*,*,#25584,.T.) ;
#35218=ORIENTED_EDGE('',*,*,#26066,.T.) ;
#35219=ORIENTED_EDGE('',*,*,#26067,.T.) ;
#35220=ORIENTED_EDGE('',*,*,#26065,.F.) ;
#35221=ORIENTED_EDGE('',*,*,#25514,.T.) ;
#35222=ORIENTED_EDGE('',*,*,#26068,.T.) ;
#35223=ORIENTED_EDGE('',*,*,#25076,.T.) ;
#35224=ORIENTED_EDGE('',*,*,#26066,.F.) ;
#35225=ORIENTED_EDGE('',*,*,#25513,.T.) ;
#35226=ORIENTED_EDGE('',*,*,#26069,.T.) ;
#35227=ORIENTED_EDGE('',*,*,#25077,.T.) ;
#35228=ORIENTED_EDGE('',*,*,#26068,.F.) ;
#35229=ORIENTED_EDGE('',*,*,#26070,.T.) ;
#35230=ORIENTED_EDGE('',*,*,#26071,.T.) ;
#35231=ORIENTED_EDGE('',*,*,#25078,.T.) ;
#35232=ORIENTED_EDGE('',*,*,#26069,.F.) ;
#35233=ORIENTED_EDGE('',*,*,#26072,.T.) ;
#35234=ORIENTED_EDGE('',*,*,#26073,.T.) ;
#35235=ORIENTED_EDGE('',*,*,#25079,.T.) ;
#35236=ORIENTED_EDGE('',*,*,#26071,.F.) ;
#35237=ORIENTED_EDGE('',*,*,#26074,.T.) ;
#35238=ORIENTED_EDGE('',*,*,#26061,.T.) ;
#35239=ORIENTED_EDGE('',*,*,#25080,.T.) ;
#35240=ORIENTED_EDGE('',*,*,#26073,.F.) ;
#35241=ORIENTED_EDGE('',*,*,#26075,.T.) ;
#35242=ORIENTED_EDGE('',*,*,#25599,.T.) ;
#35243=ORIENTED_EDGE('',*,*,#25510,.T.) ;
#35244=ORIENTED_EDGE('',*,*,#26064,.F.) ;
#35245=ORIENTED_EDGE('',*,*,#25583,.T.) ;
#35246=ORIENTED_EDGE('',*,*,#26076,.T.) ;
#35247=ORIENTED_EDGE('',*,*,#25494,.T.) ;
#35248=ORIENTED_EDGE('',*,*,#25617,.F.) ;
#35249=ORIENTED_EDGE('',*,*,#25597,.T.) ;
#35250=ORIENTED_EDGE('',*,*,#26077,.T.) ;
#35251=ORIENTED_EDGE('',*,*,#25488,.T.) ;
#35252=ORIENTED_EDGE('',*,*,#26076,.F.) ;
#35253=ORIENTED_EDGE('',*,*,#25596,.T.) ;
#35254=ORIENTED_EDGE('',*,*,#26078,.T.) ;
#35255=ORIENTED_EDGE('',*,*,#25489,.T.) ;
#35256=ORIENTED_EDGE('',*,*,#26077,.F.) ;
#35257=ORIENTED_EDGE('',*,*,#26079,.T.) ;
#35258=ORIENTED_EDGE('',*,*,#26080,.T.) ;
#35259=ORIENTED_EDGE('',*,*,#25490,.T.) ;
#35260=ORIENTED_EDGE('',*,*,#26078,.F.) ;
#35261=ORIENTED_EDGE('',*,*,#25059,.T.) ;
#35262=ORIENTED_EDGE('',*,*,#26081,.T.) ;
#35263=ORIENTED_EDGE('',*,*,#26082,.T.) ;
#35264=ORIENTED_EDGE('',*,*,#26080,.F.) ;
#35265=ORIENTED_EDGE('',*,*,#25107,.T.) ;
#35266=ORIENTED_EDGE('',*,*,#26083,.T.) ;
#35267=ORIENTED_EDGE('',*,*,#26084,.T.) ;
#35268=ORIENTED_EDGE('',*,*,#26081,.F.) ;
#35269=ORIENTED_EDGE('',*,*,#25106,.T.) ;
#35270=ORIENTED_EDGE('',*,*,#26085,.T.) ;
#35271=ORIENTED_EDGE('',*,*,#26086,.T.) ;
#35272=ORIENTED_EDGE('',*,*,#26083,.F.) ;
#35273=ORIENTED_EDGE('',*,*,#25105,.T.) ;
#35274=ORIENTED_EDGE('',*,*,#26087,.T.) ;
#35275=ORIENTED_EDGE('',*,*,#26088,.T.) ;
#35276=ORIENTED_EDGE('',*,*,#26085,.F.) ;
#35277=ORIENTED_EDGE('',*,*,#25104,.T.) ;
#35278=ORIENTED_EDGE('',*,*,#26089,.T.) ;
#35279=ORIENTED_EDGE('',*,*,#26090,.T.) ;
#35280=ORIENTED_EDGE('',*,*,#26087,.F.) ;
#35281=ORIENTED_EDGE('',*,*,#25103,.T.) ;
#35282=ORIENTED_EDGE('',*,*,#26091,.T.) ;
#35283=ORIENTED_EDGE('',*,*,#26092,.T.) ;
#35284=ORIENTED_EDGE('',*,*,#26089,.F.) ;
#35285=ORIENTED_EDGE('',*,*,#25102,.T.) ;
#35286=ORIENTED_EDGE('',*,*,#26093,.T.) ;
#35287=ORIENTED_EDGE('',*,*,#26094,.T.) ;
#35288=ORIENTED_EDGE('',*,*,#26091,.F.) ;
#35289=ORIENTED_EDGE('',*,*,#25101,.T.) ;
#35290=ORIENTED_EDGE('',*,*,#26095,.T.) ;
#35291=ORIENTED_EDGE('',*,*,#26096,.T.) ;
#35292=ORIENTED_EDGE('',*,*,#26093,.F.) ;
#35293=ORIENTED_EDGE('',*,*,#25100,.T.) ;
#35294=ORIENTED_EDGE('',*,*,#26097,.T.) ;
#35295=ORIENTED_EDGE('',*,*,#26098,.T.) ;
#35296=ORIENTED_EDGE('',*,*,#26095,.F.) ;
#35297=ORIENTED_EDGE('',*,*,#25099,.T.) ;
#35298=ORIENTED_EDGE('',*,*,#26099,.T.) ;
#35299=ORIENTED_EDGE('',*,*,#26100,.T.) ;
#35300=ORIENTED_EDGE('',*,*,#26097,.F.) ;
#35301=ORIENTED_EDGE('',*,*,#25098,.T.) ;
#35302=ORIENTED_EDGE('',*,*,#26101,.T.) ;
#35303=ORIENTED_EDGE('',*,*,#26102,.T.) ;
#35304=ORIENTED_EDGE('',*,*,#26099,.F.) ;
#35305=ORIENTED_EDGE('',*,*,#25097,.T.) ;
#35306=ORIENTED_EDGE('',*,*,#26103,.T.) ;
#35307=ORIENTED_EDGE('',*,*,#26104,.T.) ;
#35308=ORIENTED_EDGE('',*,*,#26101,.F.) ;
#35309=ORIENTED_EDGE('',*,*,#25096,.T.) ;
#35310=ORIENTED_EDGE('',*,*,#26105,.T.) ;
#35311=ORIENTED_EDGE('',*,*,#26106,.T.) ;
#35312=ORIENTED_EDGE('',*,*,#26103,.F.) ;
#35313=ORIENTED_EDGE('',*,*,#25095,.T.) ;
#35314=ORIENTED_EDGE('',*,*,#26107,.T.) ;
#35315=ORIENTED_EDGE('',*,*,#26108,.T.) ;
#35316=ORIENTED_EDGE('',*,*,#26105,.F.) ;
#35317=ORIENTED_EDGE('',*,*,#25094,.T.) ;
#35318=ORIENTED_EDGE('',*,*,#26109,.T.) ;
#35319=ORIENTED_EDGE('',*,*,#26110,.T.) ;
#35320=ORIENTED_EDGE('',*,*,#26107,.F.) ;
#35321=ORIENTED_EDGE('',*,*,#25093,.T.) ;
#35322=ORIENTED_EDGE('',*,*,#26111,.T.) ;
#35323=ORIENTED_EDGE('',*,*,#26112,.T.) ;
#35324=ORIENTED_EDGE('',*,*,#26109,.F.) ;
#35325=ORIENTED_EDGE('',*,*,#25092,.T.) ;
#35326=ORIENTED_EDGE('',*,*,#26113,.T.) ;
#35327=ORIENTED_EDGE('',*,*,#26114,.T.) ;
#35328=ORIENTED_EDGE('',*,*,#26111,.F.) ;
#35329=ORIENTED_EDGE('',*,*,#25091,.T.) ;
#35330=ORIENTED_EDGE('',*,*,#26115,.T.) ;
#35331=ORIENTED_EDGE('',*,*,#26116,.T.) ;
#35332=ORIENTED_EDGE('',*,*,#26113,.F.) ;
#35333=ORIENTED_EDGE('',*,*,#25090,.T.) ;
#35334=ORIENTED_EDGE('',*,*,#26117,.T.) ;
#35335=ORIENTED_EDGE('',*,*,#26118,.T.) ;
#35336=ORIENTED_EDGE('',*,*,#26115,.F.) ;
#35337=ORIENTED_EDGE('',*,*,#25089,.T.) ;
#35338=ORIENTED_EDGE('',*,*,#26119,.T.) ;
#35339=ORIENTED_EDGE('',*,*,#26120,.T.) ;
#35340=ORIENTED_EDGE('',*,*,#26117,.F.) ;
#35341=ORIENTED_EDGE('',*,*,#25088,.T.) ;
#35342=ORIENTED_EDGE('',*,*,#26121,.T.) ;
#35343=ORIENTED_EDGE('',*,*,#26122,.T.) ;
#35344=ORIENTED_EDGE('',*,*,#26119,.F.) ;
#35345=ORIENTED_EDGE('',*,*,#25087,.T.) ;
#35346=ORIENTED_EDGE('',*,*,#26123,.T.) ;
#35347=ORIENTED_EDGE('',*,*,#26124,.T.) ;
#35348=ORIENTED_EDGE('',*,*,#26121,.F.) ;
#35349=ORIENTED_EDGE('',*,*,#25086,.T.) ;
#35350=ORIENTED_EDGE('',*,*,#26125,.T.) ;
#35351=ORIENTED_EDGE('',*,*,#26126,.T.) ;
#35352=ORIENTED_EDGE('',*,*,#26123,.F.) ;
#35353=ORIENTED_EDGE('',*,*,#25085,.T.) ;
#35354=ORIENTED_EDGE('',*,*,#26125,.F.) ;
#35355=ORIENTED_EDGE('',*,*,#25084,.T.) ;
#35356=ORIENTED_EDGE('',*,*,#26060,.T.) ;
#35357=ORIENTED_EDGE('',*,*,#26127,.T.) ;
#35358=ORIENTED_EDGE('',*,*,#26128,.T.) ;
#35359=ORIENTED_EDGE('',*,*,#26129,.T.) ;
#35360=ORIENTED_EDGE('',*,*,#25328,.T.) ;
#35361=ORIENTED_EDGE('',*,*,#26130,.T.) ;
#35362=ORIENTED_EDGE('',*,*,#26062,.T.) ;
#35363=ORIENTED_EDGE('',*,*,#26131,.T.) ;
#35364=ORIENTED_EDGE('',*,*,#26128,.F.) ;
#35365=ORIENTED_EDGE('',*,*,#26132,.T.) ;
#35366=ORIENTED_EDGE('',*,*,#26058,.T.) ;
#35367=ORIENTED_EDGE('',*,*,#25082,.T.) ;
#35368=ORIENTED_EDGE('',*,*,#26063,.T.) ;
#35369=ORIENTED_EDGE('',*,*,#26133,.T.) ;
#35370=ORIENTED_EDGE('',*,*,#26134,.T.) ;
#35371=ORIENTED_EDGE('',*,*,#26135,.T.) ;
#35372=ORIENTED_EDGE('',*,*,#26059,.T.) ;
#35373=ORIENTED_EDGE('',*,*,#26136,.T.) ;
#35374=ORIENTED_EDGE('',*,*,#25326,.T.) ;
#35375=ORIENTED_EDGE('',*,*,#26137,.T.) ;
#35376=ORIENTED_EDGE('',*,*,#26134,.F.) ;
#35377=ORIENTED_EDGE('',*,*,#26138,.T.) ;
#35378=ORIENTED_EDGE('',*,*,#26079,.F.) ;
#35379=ORIENTED_EDGE('',*,*,#25595,.T.) ;
#35380=ORIENTED_EDGE('',*,*,#26139,.F.) ;
#35381=ORIENTED_EDGE('',*,*,#26140,.F.) ;
#35382=ORIENTED_EDGE('',*,*,#25060,.T.) ;
#35383=ORIENTED_EDGE('',*,*,#26084,.F.) ;
#35384=ORIENTED_EDGE('',*,*,#26141,.F.) ;
#35385=ORIENTED_EDGE('',*,*,#26142,.F.) ;
#35386=ORIENTED_EDGE('',*,*,#26143,.F.) ;
#35387=ORIENTED_EDGE('',*,*,#26086,.F.) ;
#35388=ORIENTED_EDGE('',*,*,#26144,.T.) ;
#35389=ORIENTED_EDGE('',*,*,#26145,.F.) ;
#35390=ORIENTED_EDGE('',*,*,#26141,.T.) ;
#35391=ORIENTED_EDGE('',*,*,#26088,.F.) ;
#35392=ORIENTED_EDGE('',*,*,#26146,.F.) ;
#35393=ORIENTED_EDGE('',*,*,#26147,.F.) ;
#35394=ORIENTED_EDGE('',*,*,#26144,.F.) ;
#35395=ORIENTED_EDGE('',*,*,#26090,.F.) ;
#35396=ORIENTED_EDGE('',*,*,#26148,.T.) ;
#35397=ORIENTED_EDGE('',*,*,#26149,.F.) ;
#35398=ORIENTED_EDGE('',*,*,#26146,.T.) ;
#35399=ORIENTED_EDGE('',*,*,#26092,.F.) ;
#35400=ORIENTED_EDGE('',*,*,#26150,.F.) ;
#35401=ORIENTED_EDGE('',*,*,#26151,.F.) ;
#35402=ORIENTED_EDGE('',*,*,#26148,.F.) ;
#35403=ORIENTED_EDGE('',*,*,#26094,.F.) ;
#35404=ORIENTED_EDGE('',*,*,#26152,.F.) ;
#35405=ORIENTED_EDGE('',*,*,#26153,.F.) ;
#35406=ORIENTED_EDGE('',*,*,#26150,.T.) ;
#35407=ORIENTED_EDGE('',*,*,#26096,.F.) ;
#35408=ORIENTED_EDGE('',*,*,#26154,.F.) ;
#35409=ORIENTED_EDGE('',*,*,#26155,.F.) ;
#35410=ORIENTED_EDGE('',*,*,#26152,.T.) ;
#35411=ORIENTED_EDGE('',*,*,#26098,.F.) ;
#35412=ORIENTED_EDGE('',*,*,#26156,.T.) ;
#35413=ORIENTED_EDGE('',*,*,#26157,.F.) ;
#35414=ORIENTED_EDGE('',*,*,#26154,.T.) ;
#35415=ORIENTED_EDGE('',*,*,#26100,.F.) ;
#35416=ORIENTED_EDGE('',*,*,#26158,.F.) ;
#35417=ORIENTED_EDGE('',*,*,#26159,.F.) ;
#35418=ORIENTED_EDGE('',*,*,#26156,.F.) ;
#35419=ORIENTED_EDGE('',*,*,#26102,.F.) ;
#35420=ORIENTED_EDGE('',*,*,#26160,.T.) ;
#35421=ORIENTED_EDGE('',*,*,#26161,.F.) ;
#35422=ORIENTED_EDGE('',*,*,#26158,.T.) ;
#35423=ORIENTED_EDGE('',*,*,#26104,.F.) ;
#35424=ORIENTED_EDGE('',*,*,#26162,.F.) ;
#35425=ORIENTED_EDGE('',*,*,#26163,.F.) ;
#35426=ORIENTED_EDGE('',*,*,#26160,.F.) ;
#35427=ORIENTED_EDGE('',*,*,#26106,.F.) ;
#35428=ORIENTED_EDGE('',*,*,#26164,.T.) ;
#35429=ORIENTED_EDGE('',*,*,#26165,.F.) ;
#35430=ORIENTED_EDGE('',*,*,#26162,.T.) ;
#35431=ORIENTED_EDGE('',*,*,#26108,.F.) ;
#35432=ORIENTED_EDGE('',*,*,#26166,.F.) ;
#35433=ORIENTED_EDGE('',*,*,#26167,.F.) ;
#35434=ORIENTED_EDGE('',*,*,#26164,.F.) ;
#35435=ORIENTED_EDGE('',*,*,#26110,.F.) ;
#35436=ORIENTED_EDGE('',*,*,#26168,.F.) ;
#35437=ORIENTED_EDGE('',*,*,#26169,.F.) ;
#35438=ORIENTED_EDGE('',*,*,#26166,.T.) ;
#35439=ORIENTED_EDGE('',*,*,#26112,.F.) ;
#35440=ORIENTED_EDGE('',*,*,#26170,.F.) ;
#35441=ORIENTED_EDGE('',*,*,#26171,.F.) ;
#35442=ORIENTED_EDGE('',*,*,#26168,.T.) ;
#35443=ORIENTED_EDGE('',*,*,#26114,.F.) ;
#35444=ORIENTED_EDGE('',*,*,#26172,.T.) ;
#35445=ORIENTED_EDGE('',*,*,#26173,.F.) ;
#35446=ORIENTED_EDGE('',*,*,#26170,.T.) ;
#35447=ORIENTED_EDGE('',*,*,#26116,.F.) ;
#35448=ORIENTED_EDGE('',*,*,#26174,.F.) ;
#35449=ORIENTED_EDGE('',*,*,#26175,.F.) ;
#35450=ORIENTED_EDGE('',*,*,#26172,.F.) ;
#35451=ORIENTED_EDGE('',*,*,#26118,.F.) ;
#35452=ORIENTED_EDGE('',*,*,#26176,.T.) ;
#35453=ORIENTED_EDGE('',*,*,#26177,.F.) ;
#35454=ORIENTED_EDGE('',*,*,#26174,.T.) ;
#35455=ORIENTED_EDGE('',*,*,#26120,.F.) ;
#35456=ORIENTED_EDGE('',*,*,#26178,.F.) ;
#35457=ORIENTED_EDGE('',*,*,#26179,.F.) ;
#35458=ORIENTED_EDGE('',*,*,#26176,.F.) ;
#35459=ORIENTED_EDGE('',*,*,#26122,.F.) ;
#35460=ORIENTED_EDGE('',*,*,#26180,.T.) ;
#35461=ORIENTED_EDGE('',*,*,#26181,.F.) ;
#35462=ORIENTED_EDGE('',*,*,#26178,.T.) ;
#35463=ORIENTED_EDGE('',*,*,#26124,.F.) ;
#35464=ORIENTED_EDGE('',*,*,#26182,.F.) ;
#35465=ORIENTED_EDGE('',*,*,#26183,.F.) ;
#35466=ORIENTED_EDGE('',*,*,#26180,.F.) ;
#35467=ORIENTED_EDGE('',*,*,#26126,.F.) ;
#35468=ORIENTED_EDGE('',*,*,#26184,.T.) ;
#35469=ORIENTED_EDGE('',*,*,#26185,.F.) ;
#35470=ORIENTED_EDGE('',*,*,#26182,.T.) ;
#35471=ORIENTED_EDGE('',*,*,#26127,.F.) ;
#35472=ORIENTED_EDGE('',*,*,#26135,.F.) ;
#35473=ORIENTED_EDGE('',*,*,#26186,.F.) ;
#35474=ORIENTED_EDGE('',*,*,#26184,.F.) ;
#35475=ORIENTED_EDGE('',*,*,#26137,.F.) ;
#35476=ORIENTED_EDGE('',*,*,#25325,.T.) ;
#35477=ORIENTED_EDGE('',*,*,#26187,.F.) ;
#35478=ORIENTED_EDGE('',*,*,#26186,.T.) ;
#35479=ORIENTED_EDGE('',*,*,#26188,.T.) ;
#35480=ORIENTED_EDGE('',*,*,#26189,.T.) ;
#35481=ORIENTED_EDGE('',*,*,#26190,.T.) ;
#35482=ORIENTED_EDGE('',*,*,#26191,.T.) ;
#35483=ORIENTED_EDGE('',*,*,#26192,.T.) ;
#35484=ORIENTED_EDGE('',*,*,#26193,.T.) ;
#35485=ORIENTED_EDGE('',*,*,#26190,.F.) ;
#35486=ORIENTED_EDGE('',*,*,#26194,.T.) ;
#35487=ORIENTED_EDGE('',*,*,#26195,.T.) ;
#35488=ORIENTED_EDGE('',*,*,#26192,.F.) ;
#35489=ORIENTED_EDGE('',*,*,#25129,.T.) ;
#35490=ORIENTED_EDGE('',*,*,#26194,.F.) ;
#35491=ORIENTED_EDGE('',*,*,#26196,.T.) ;
#35492=ORIENTED_EDGE('',*,*,#26197,.F.) ;
#35493=ORIENTED_EDGE('',*,*,#25130,.T.) ;
#35494=ORIENTED_EDGE('',*,*,#26189,.F.) ;
#35495=ORIENTED_EDGE('',*,*,#26198,.F.) ;
#35496=ORIENTED_EDGE('',*,*,#26199,.F.) ;
#35497=ORIENTED_EDGE('',*,*,#26196,.F.) ;
#35498=ORIENTED_EDGE('',*,*,#26188,.F.) ;
#35499=ORIENTED_EDGE('',*,*,#26200,.T.) ;
#35500=ORIENTED_EDGE('',*,*,#26201,.T.) ;
#35501=ORIENTED_EDGE('',*,*,#26202,.T.) ;
#35502=ORIENTED_EDGE('',*,*,#26203,.F.) ;
#35503=ORIENTED_EDGE('',*,*,#26198,.T.) ;
#35504=ORIENTED_EDGE('',*,*,#26203,.T.) ;
#35505=ORIENTED_EDGE('',*,*,#26204,.T.) ;
#35506=ORIENTED_EDGE('',*,*,#26205,.T.) ;
#35507=ORIENTED_EDGE('',*,*,#26199,.T.) ;
#35508=ORIENTED_EDGE('',*,*,#26206,.T.) ;
#35509=ORIENTED_EDGE('',*,*,#26197,.T.) ;
#35510=ORIENTED_EDGE('',*,*,#26205,.F.) ;
#35511=ORIENTED_EDGE('',*,*,#26207,.T.) ;
#35512=ORIENTED_EDGE('',*,*,#26208,.F.) ;
#35513=ORIENTED_EDGE('',*,*,#25131,.T.) ;
#35514=ORIENTED_EDGE('',*,*,#26206,.F.) ;
#35515=ORIENTED_EDGE('',*,*,#26207,.F.) ;
#35516=ORIENTED_EDGE('',*,*,#26204,.F.) ;
#35517=ORIENTED_EDGE('',*,*,#26202,.F.) ;
#35518=ORIENTED_EDGE('',*,*,#26209,.T.) ;
#35519=ORIENTED_EDGE('',*,*,#26210,.F.) ;
#35520=ORIENTED_EDGE('',*,*,#25143,.T.) ;
#35521=ORIENTED_EDGE('',*,*,#26211,.F.) ;
#35522=ORIENTED_EDGE('',*,*,#26212,.F.) ;
#35523=ORIENTED_EDGE('',*,*,#26213,.F.) ;
#35524=ORIENTED_EDGE('',*,*,#26214,.F.) ;
#35525=ORIENTED_EDGE('',*,*,#26215,.F.) ;
#35526=ORIENTED_EDGE('',*,*,#25141,.T.) ;
#35527=ORIENTED_EDGE('',*,*,#26216,.F.) ;
#35528=ORIENTED_EDGE('',*,*,#26211,.T.) ;
#35529=ORIENTED_EDGE('',*,*,#25142,.T.) ;
#35530=ORIENTED_EDGE('',*,*,#26215,.T.) ;
#35531=ORIENTED_EDGE('',*,*,#26217,.T.) ;
#35532=ORIENTED_EDGE('',*,*,#26218,.F.) ;
#35533=ORIENTED_EDGE('',*,*,#26219,.F.) ;
#35534=ORIENTED_EDGE('',*,*,#25139,.T.) ;
#35535=ORIENTED_EDGE('',*,*,#26220,.F.) ;
#35536=ORIENTED_EDGE('',*,*,#26219,.T.) ;
#35537=ORIENTED_EDGE('',*,*,#26221,.T.) ;
#35538=ORIENTED_EDGE('',*,*,#26216,.T.) ;
#35539=ORIENTED_EDGE('',*,*,#25140,.T.) ;
#35540=ORIENTED_EDGE('',*,*,#26222,.F.) ;
#35541=ORIENTED_EDGE('',*,*,#26223,.F.) ;
#35542=ORIENTED_EDGE('',*,*,#25137,.T.) ;
#35543=ORIENTED_EDGE('',*,*,#26224,.F.) ;
#35544=ORIENTED_EDGE('',*,*,#26220,.T.) ;
#35545=ORIENTED_EDGE('',*,*,#25138,.T.) ;
#35546=ORIENTED_EDGE('',*,*,#26223,.T.) ;
#35547=ORIENTED_EDGE('',*,*,#26225,.T.) ;
#35548=ORIENTED_EDGE('',*,*,#26226,.F.) ;
#35549=ORIENTED_EDGE('',*,*,#26227,.F.) ;
#35550=ORIENTED_EDGE('',*,*,#25135,.T.) ;
#35551=ORIENTED_EDGE('',*,*,#26228,.F.) ;
#35552=ORIENTED_EDGE('',*,*,#26227,.T.) ;
#35553=ORIENTED_EDGE('',*,*,#26229,.T.) ;
#35554=ORIENTED_EDGE('',*,*,#26224,.T.) ;
#35555=ORIENTED_EDGE('',*,*,#25136,.T.) ;
#35556=ORIENTED_EDGE('',*,*,#25133,.T.) ;
#35557=ORIENTED_EDGE('',*,*,#26230,.F.) ;
#35558=ORIENTED_EDGE('',*,*,#26231,.F.) ;
#35559=ORIENTED_EDGE('',*,*,#26232,.F.) ;
#35560=ORIENTED_EDGE('',*,*,#26233,.T.) ;
#35561=ORIENTED_EDGE('',*,*,#26230,.T.) ;
#35562=ORIENTED_EDGE('',*,*,#25132,.F.) ;
#35563=ORIENTED_EDGE('',*,*,#26208,.T.) ;
#35564=ORIENTED_EDGE('',*,*,#25377,.T.) ;
#35565=ORIENTED_EDGE('',*,*,#26234,.T.) ;
#35566=ORIENTED_EDGE('',*,*,#26231,.T.) ;
#35567=ORIENTED_EDGE('',*,*,#26235,.T.) ;
#35568=ORIENTED_EDGE('',*,*,#26228,.T.) ;
#35569=ORIENTED_EDGE('',*,*,#25134,.T.) ;
#35570=ORIENTED_EDGE('',*,*,#26232,.T.) ;
#35571=ORIENTED_EDGE('',*,*,#26236,.T.) ;
#35572=ORIENTED_EDGE('',*,*,#25375,.T.) ;
#35573=ORIENTED_EDGE('',*,*,#26237,.T.) ;
#35574=ORIENTED_EDGE('',*,*,#26226,.T.) ;
#35575=ORIENTED_EDGE('',*,*,#26238,.T.) ;
#35576=ORIENTED_EDGE('',*,*,#25373,.T.) ;
#35577=ORIENTED_EDGE('',*,*,#26239,.T.) ;
#35578=ORIENTED_EDGE('',*,*,#26222,.T.) ;
#35579=ORIENTED_EDGE('',*,*,#26240,.T.) ;
#35580=ORIENTED_EDGE('',*,*,#25371,.T.) ;
#35581=ORIENTED_EDGE('',*,*,#26241,.T.) ;
#35582=ORIENTED_EDGE('',*,*,#26218,.T.) ;
#35583=ORIENTED_EDGE('',*,*,#26242,.T.) ;
#35584=ORIENTED_EDGE('',*,*,#25369,.T.) ;
#35585=ORIENTED_EDGE('',*,*,#26243,.T.) ;
#35586=ORIENTED_EDGE('',*,*,#26214,.T.) ;
#35587=ORIENTED_EDGE('',*,*,#26244,.T.) ;
#35588=ORIENTED_EDGE('',*,*,#25381,.T.) ;
#35589=ORIENTED_EDGE('',*,*,#26245,.T.) ;
#35590=ORIENTED_EDGE('',*,*,#26212,.T.) ;
#35591=ORIENTED_EDGE('',*,*,#26246,.T.) ;
#35592=ORIENTED_EDGE('',*,*,#25128,.F.) ;
#35593=ORIENTED_EDGE('',*,*,#26213,.T.) ;
#35594=ORIENTED_EDGE('',*,*,#26247,.T.) ;
#35595=ORIENTED_EDGE('',*,*,#26195,.F.) ;
#35596=ORIENTED_EDGE('',*,*,#26238,.F.) ;
#35597=ORIENTED_EDGE('',*,*,#26236,.F.) ;
#35598=ORIENTED_EDGE('',*,*,#26234,.F.) ;
#35599=ORIENTED_EDGE('',*,*,#25376,.F.) ;
#35600=ORIENTED_EDGE('',*,*,#26235,.F.) ;
#35601=ORIENTED_EDGE('',*,*,#26233,.F.) ;
#35602=ORIENTED_EDGE('',*,*,#26210,.T.) ;
#35603=ORIENTED_EDGE('',*,*,#25378,.F.) ;
#35604=ORIENTED_EDGE('',*,*,#26248,.F.) ;
#35605=ORIENTED_EDGE('',*,*,#26249,.F.) ;
#35606=ORIENTED_EDGE('',*,*,#26250,.F.) ;
#35607=ORIENTED_EDGE('',*,*,#25152,.T.) ;
#35608=ORIENTED_EDGE('',*,*,#26251,.F.) ;
#35609=ORIENTED_EDGE('',*,*,#26252,.F.) ;
#35610=ORIENTED_EDGE('',*,*,#26253,.F.) ;
#35611=ORIENTED_EDGE('',*,*,#26251,.T.) ;
#35612=ORIENTED_EDGE('',*,*,#25151,.T.) ;
#35613=ORIENTED_EDGE('',*,*,#26248,.T.) ;
#35614=ORIENTED_EDGE('',*,*,#26254,.T.) ;
#35615=ORIENTED_EDGE('',*,*,#25746,.F.) ;
#35616=ORIENTED_EDGE('',*,*,#26255,.T.) ;
#35617=ORIENTED_EDGE('',*,*,#26252,.T.) ;
#35618=ORIENTED_EDGE('',*,*,#26256,.T.) ;
#35619=ORIENTED_EDGE('',*,*,#25149,.T.) ;
#35620=ORIENTED_EDGE('',*,*,#26257,.F.) ;
#35621=ORIENTED_EDGE('',*,*,#26258,.F.) ;
#35622=ORIENTED_EDGE('',*,*,#26259,.F.) ;
#35623=ORIENTED_EDGE('',*,*,#25154,.T.) ;
#35624=ORIENTED_EDGE('',*,*,#26260,.F.) ;
#35625=ORIENTED_EDGE('',*,*,#25775,.F.) ;
#35626=ORIENTED_EDGE('',*,*,#26261,.F.) ;
#35627=ORIENTED_EDGE('',*,*,#26260,.T.) ;
#35628=ORIENTED_EDGE('',*,*,#25153,.T.) ;
#35629=ORIENTED_EDGE('',*,*,#26253,.T.) ;
#35630=ORIENTED_EDGE('',*,*,#26262,.T.) ;
#35631=ORIENTED_EDGE('',*,*,#26263,.F.) ;
#35632=ORIENTED_EDGE('',*,*,#26264,.F.) ;
#35633=ORIENTED_EDGE('',*,*,#25147,.T.) ;
#35634=ORIENTED_EDGE('',*,*,#26265,.F.) ;
#35635=ORIENTED_EDGE('',*,*,#26257,.T.) ;
#35636=ORIENTED_EDGE('',*,*,#25148,.T.) ;
#35637=ORIENTED_EDGE('',*,*,#26264,.T.) ;
#35638=ORIENTED_EDGE('',*,*,#26266,.T.) ;
#35639=ORIENTED_EDGE('',*,*,#25156,.T.) ;
#35640=ORIENTED_EDGE('',*,*,#26267,.F.) ;
#35641=ORIENTED_EDGE('',*,*,#25780,.F.) ;
#35642=ORIENTED_EDGE('',*,*,#26268,.F.) ;
#35643=ORIENTED_EDGE('',*,*,#26267,.T.) ;
#35644=ORIENTED_EDGE('',*,*,#25155,.T.) ;
#35645=ORIENTED_EDGE('',*,*,#26261,.T.) ;
#35646=ORIENTED_EDGE('',*,*,#25778,.T.) ;
#35647=ORIENTED_EDGE('',*,*,#26269,.F.) ;
#35648=ORIENTED_EDGE('',*,*,#26270,.F.) ;
#35649=ORIENTED_EDGE('',*,*,#25788,.F.) ;
#35650=ORIENTED_EDGE('',*,*,#25144,.T.) ;
#35651=ORIENTED_EDGE('',*,*,#26271,.F.) ;
#35652=ORIENTED_EDGE('',*,*,#25784,.F.) ;
#35653=ORIENTED_EDGE('',*,*,#26272,.F.) ;
#35654=ORIENTED_EDGE('',*,*,#26271,.T.) ;
#35655=ORIENTED_EDGE('',*,*,#25157,.T.) ;
#35656=ORIENTED_EDGE('',*,*,#26268,.T.) ;
#35657=ORIENTED_EDGE('',*,*,#25782,.T.) ;
#35658=ORIENTED_EDGE('',*,*,#26270,.T.) ;
#35659=ORIENTED_EDGE('',*,*,#25145,.T.) ;
#35660=ORIENTED_EDGE('',*,*,#26272,.T.) ;
#35661=ORIENTED_EDGE('',*,*,#25786,.T.) ;
#35662=ORIENTED_EDGE('',*,*,#26265,.T.) ;
#35663=ORIENTED_EDGE('',*,*,#25146,.T.) ;
#35664=ORIENTED_EDGE('',*,*,#26269,.T.) ;
#35665=ORIENTED_EDGE('',*,*,#25790,.T.) ;
#35666=ORIENTED_EDGE('',*,*,#25765,.F.) ;
#35667=ORIENTED_EDGE('',*,*,#26273,.T.) ;
#35668=ORIENTED_EDGE('',*,*,#26263,.T.) ;
#35669=ORIENTED_EDGE('',*,*,#25789,.T.) ;
#35670=ORIENTED_EDGE('',*,*,#25769,.F.) ;
#35671=ORIENTED_EDGE('',*,*,#26274,.T.) ;
#35672=ORIENTED_EDGE('',*,*,#26258,.T.) ;
#35673=ORIENTED_EDGE('',*,*,#26275,.T.) ;
#35674=ORIENTED_EDGE('',*,*,#26249,.T.) ;
#35675=ORIENTED_EDGE('',*,*,#25150,.T.) ;
#35676=ORIENTED_EDGE('',*,*,#26259,.T.) ;
#35677=ORIENTED_EDGE('',*,*,#26276,.T.) ;
#35678=ORIENTED_EDGE('',*,*,#25773,.F.) ;
#35679=ORIENTED_EDGE('',*,*,#26277,.T.) ;
#35680=ORIENTED_EDGE('',*,*,#26250,.T.) ;
#35681=ORIENTED_EDGE('',*,*,#26278,.T.) ;
#35682=ORIENTED_EDGE('',*,*,#25748,.F.) ;
#35683=ORIENTED_EDGE('',*,*,#25776,.F.) ;
#35684=ORIENTED_EDGE('',*,*,#26262,.F.) ;
#35685=ORIENTED_EDGE('',*,*,#26255,.F.) ;
#35686=ORIENTED_EDGE('',*,*,#25743,.F.) ;
#35687=ORIENTED_EDGE('',*,*,#26256,.F.) ;
#35688=ORIENTED_EDGE('',*,*,#26254,.F.) ;
#35689=ORIENTED_EDGE('',*,*,#26277,.F.) ;
#35690=ORIENTED_EDGE('',*,*,#26279,.T.) ;
#35691=ORIENTED_EDGE('',*,*,#26280,.T.) ;
#35692=ORIENTED_EDGE('',*,*,#26281,.T.) ;
#35693=ORIENTED_EDGE('',*,*,#26282,.T.) ;
#35694=ORIENTED_EDGE('',*,*,#26283,.T.) ;
#35695=ORIENTED_EDGE('',*,*,#26284,.T.) ;
#35696=ORIENTED_EDGE('',*,*,#26281,.F.) ;
#35697=ORIENTED_EDGE('',*,*,#26285,.T.) ;
#35698=ORIENTED_EDGE('',*,*,#25704,.F.) ;
#35699=ORIENTED_EDGE('',*,*,#25204,.T.) ;
#35700=ORIENTED_EDGE('',*,*,#26283,.F.) ;
#35701=ORIENTED_EDGE('',*,*,#26285,.F.) ;
#35702=ORIENTED_EDGE('',*,*,#26280,.F.) ;
#35703=ORIENTED_EDGE('',*,*,#26286,.F.) ;
#35704=ORIENTED_EDGE('',*,*,#26287,.T.) ;
#35705=ORIENTED_EDGE('',*,*,#25703,.F.) ;
#35706=ORIENTED_EDGE('',*,*,#26288,.T.) ;
#35707=ORIENTED_EDGE('',*,*,#26289,.T.) ;
#35708=ORIENTED_EDGE('',*,*,#26290,.T.) ;
#35709=ORIENTED_EDGE('',*,*,#26291,.T.) ;
#35710=ORIENTED_EDGE('',*,*,#26292,.T.) ;
#35711=ORIENTED_EDGE('',*,*,#26293,.T.) ;
#35712=ORIENTED_EDGE('',*,*,#26290,.F.) ;
#35713=ORIENTED_EDGE('',*,*,#26294,.T.) ;
#35714=ORIENTED_EDGE('',*,*,#25692,.T.) ;
#35715=ORIENTED_EDGE('',*,*,#26292,.F.) ;
#35716=ORIENTED_EDGE('',*,*,#25216,.T.) ;
#35717=ORIENTED_EDGE('',*,*,#26284,.F.) ;
#35718=ORIENTED_EDGE('',*,*,#25217,.T.) ;
#35719=ORIENTED_EDGE('',*,*,#26294,.F.) ;
#35720=ORIENTED_EDGE('',*,*,#26295,.T.) ;
#35721=ORIENTED_EDGE('',*,*,#26282,.F.) ;
#35722=ORIENTED_EDGE('',*,*,#26295,.F.) ;
#35723=ORIENTED_EDGE('',*,*,#26289,.F.) ;
#35724=ORIENTED_EDGE('',*,*,#26296,.F.) ;
#35725=ORIENTED_EDGE('',*,*,#25956,.F.) ;
#35726=ORIENTED_EDGE('',*,*,#26297,.F.) ;
#35727=ORIENTED_EDGE('',*,*,#25213,.T.) ;
#35728=ORIENTED_EDGE('',*,*,#26298,.F.) ;
#35729=ORIENTED_EDGE('',*,*,#25690,.F.) ;
#35730=ORIENTED_EDGE('',*,*,#25214,.T.) ;
#35731=ORIENTED_EDGE('',*,*,#26297,.T.) ;
#35732=ORIENTED_EDGE('',*,*,#25957,.T.) ;
#35733=ORIENTED_EDGE('',*,*,#25952,.F.) ;
#35734=ORIENTED_EDGE('',*,*,#26299,.F.) ;
#35735=ORIENTED_EDGE('',*,*,#25211,.T.) ;
#35736=ORIENTED_EDGE('',*,*,#26300,.F.) ;
#35737=ORIENTED_EDGE('',*,*,#26299,.T.) ;
#35738=ORIENTED_EDGE('',*,*,#25954,.T.) ;
#35739=ORIENTED_EDGE('',*,*,#26298,.T.) ;
#35740=ORIENTED_EDGE('',*,*,#25212,.T.) ;
#35741=ORIENTED_EDGE('',*,*,#25948,.F.) ;
#35742=ORIENTED_EDGE('',*,*,#26301,.F.) ;
#35743=ORIENTED_EDGE('',*,*,#25209,.T.) ;
#35744=ORIENTED_EDGE('',*,*,#26302,.F.) ;
#35745=ORIENTED_EDGE('',*,*,#26300,.T.) ;
#35746=ORIENTED_EDGE('',*,*,#25210,.T.) ;
#35747=ORIENTED_EDGE('',*,*,#26301,.T.) ;
#35748=ORIENTED_EDGE('',*,*,#25950,.T.) ;
#35749=ORIENTED_EDGE('',*,*,#25944,.F.) ;
#35750=ORIENTED_EDGE('',*,*,#26303,.F.) ;
#35751=ORIENTED_EDGE('',*,*,#25207,.T.) ;
#35752=ORIENTED_EDGE('',*,*,#26304,.F.) ;
#35753=ORIENTED_EDGE('',*,*,#26303,.T.) ;
#35754=ORIENTED_EDGE('',*,*,#25946,.T.) ;
#35755=ORIENTED_EDGE('',*,*,#26302,.T.) ;
#35756=ORIENTED_EDGE('',*,*,#25208,.T.) ;
#35757=ORIENTED_EDGE('',*,*,#25695,.F.) ;
#35758=ORIENTED_EDGE('',*,*,#25942,.T.) ;
#35759=ORIENTED_EDGE('',*,*,#26304,.T.) ;
#35760=ORIENTED_EDGE('',*,*,#25206,.T.) ;
#35761=ORIENTED_EDGE('',*,*,#26305,.T.) ;
#35762=ORIENTED_EDGE('',*,*,#26306,.T.) ;
#35763=ORIENTED_EDGE('',*,*,#26307,.T.) ;
#35764=ORIENTED_EDGE('',*,*,#26308,.T.) ;
#35765=ORIENTED_EDGE('',*,*,#26309,.T.) ;
#35766=ORIENTED_EDGE('',*,*,#26310,.T.) ;
#35767=ORIENTED_EDGE('',*,*,#26307,.F.) ;
#35768=ORIENTED_EDGE('',*,*,#26311,.T.) ;
#35769=ORIENTED_EDGE('',*,*,#26312,.T.) ;
#35770=ORIENTED_EDGE('',*,*,#26309,.F.) ;
#35771=ORIENTED_EDGE('',*,*,#25173,.T.) ;
#35772=ORIENTED_EDGE('',*,*,#26311,.F.) ;
#35773=ORIENTED_EDGE('',*,*,#26313,.T.) ;
#35774=ORIENTED_EDGE('',*,*,#26314,.F.) ;
#35775=ORIENTED_EDGE('',*,*,#25174,.T.) ;
#35776=ORIENTED_EDGE('',*,*,#26306,.F.) ;
#35777=ORIENTED_EDGE('',*,*,#26315,.F.) ;
#35778=ORIENTED_EDGE('',*,*,#26316,.F.) ;
#35779=ORIENTED_EDGE('',*,*,#26313,.F.) ;
#35780=ORIENTED_EDGE('',*,*,#26305,.F.) ;
#35781=ORIENTED_EDGE('',*,*,#26317,.T.) ;
#35782=ORIENTED_EDGE('',*,*,#26318,.T.) ;
#35783=ORIENTED_EDGE('',*,*,#26319,.T.) ;
#35784=ORIENTED_EDGE('',*,*,#26320,.F.) ;
#35785=ORIENTED_EDGE('',*,*,#26315,.T.) ;
#35786=ORIENTED_EDGE('',*,*,#26320,.T.) ;
#35787=ORIENTED_EDGE('',*,*,#26321,.T.) ;
#35788=ORIENTED_EDGE('',*,*,#26322,.T.) ;
#35789=ORIENTED_EDGE('',*,*,#26316,.T.) ;
#35790=ORIENTED_EDGE('',*,*,#26323,.T.) ;
#35791=ORIENTED_EDGE('',*,*,#26314,.T.) ;
#35792=ORIENTED_EDGE('',*,*,#26322,.F.) ;
#35793=ORIENTED_EDGE('',*,*,#26324,.T.) ;
#35794=ORIENTED_EDGE('',*,*,#26325,.F.) ;
#35795=ORIENTED_EDGE('',*,*,#25175,.T.) ;
#35796=ORIENTED_EDGE('',*,*,#26323,.F.) ;
#35797=ORIENTED_EDGE('',*,*,#26324,.F.) ;
#35798=ORIENTED_EDGE('',*,*,#26321,.F.) ;
#35799=ORIENTED_EDGE('',*,*,#26319,.F.) ;
#35800=ORIENTED_EDGE('',*,*,#26326,.T.) ;
#35801=ORIENTED_EDGE('',*,*,#25365,.T.) ;
#35802=ORIENTED_EDGE('',*,*,#25826,.T.) ;
#35803=ORIENTED_EDGE('',*,*,#26327,.F.) ;
#35804=ORIENTED_EDGE('',*,*,#26328,.F.) ;
#35805=ORIENTED_EDGE('',*,*,#26329,.F.) ;
#35806=ORIENTED_EDGE('',*,*,#25178,.T.) ;
#35807=ORIENTED_EDGE('',*,*,#26330,.F.) ;
#35808=ORIENTED_EDGE('',*,*,#26331,.F.) ;
#35809=ORIENTED_EDGE('',*,*,#26332,.F.) ;
#35810=ORIENTED_EDGE('',*,*,#25180,.T.) ;
#35811=ORIENTED_EDGE('',*,*,#26333,.F.) ;
#35812=ORIENTED_EDGE('',*,*,#26334,.F.) ;
#35813=ORIENTED_EDGE('',*,*,#26335,.F.) ;
#35814=ORIENTED_EDGE('',*,*,#25182,.T.) ;
#35815=ORIENTED_EDGE('',*,*,#26336,.F.) ;
#35816=ORIENTED_EDGE('',*,*,#26337,.F.) ;
#35817=ORIENTED_EDGE('',*,*,#26338,.F.) ;
#35818=ORIENTED_EDGE('',*,*,#25184,.T.) ;
#35819=ORIENTED_EDGE('',*,*,#26339,.F.) ;
#35820=ORIENTED_EDGE('',*,*,#25820,.F.) ;
#35821=ORIENTED_EDGE('',*,*,#25185,.T.) ;
#35822=ORIENTED_EDGE('',*,*,#26338,.T.) ;
#35823=ORIENTED_EDGE('',*,*,#26340,.T.) ;
#35824=ORIENTED_EDGE('',*,*,#25819,.F.) ;
#35825=ORIENTED_EDGE('',*,*,#25829,.T.) ;
#35826=ORIENTED_EDGE('',*,*,#26312,.F.) ;
#35827=ORIENTED_EDGE('',*,*,#25172,.F.) ;
#35828=ORIENTED_EDGE('',*,*,#26335,.T.) ;
#35829=ORIENTED_EDGE('',*,*,#26341,.T.) ;
#35830=ORIENTED_EDGE('',*,*,#26339,.T.) ;
#35831=ORIENTED_EDGE('',*,*,#25183,.T.) ;
#35832=ORIENTED_EDGE('',*,*,#25800,.F.) ;
#35833=ORIENTED_EDGE('',*,*,#26342,.T.) ;
#35834=ORIENTED_EDGE('',*,*,#26337,.T.) ;
#35835=ORIENTED_EDGE('',*,*,#26343,.T.) ;
#35836=ORIENTED_EDGE('',*,*,#26336,.T.) ;
#35837=ORIENTED_EDGE('',*,*,#25181,.T.) ;
#35838=ORIENTED_EDGE('',*,*,#26332,.T.) ;
#35839=ORIENTED_EDGE('',*,*,#26344,.T.) ;
#35840=ORIENTED_EDGE('',*,*,#25804,.F.) ;
#35841=ORIENTED_EDGE('',*,*,#26345,.T.) ;
#35842=ORIENTED_EDGE('',*,*,#26334,.T.) ;
#35843=ORIENTED_EDGE('',*,*,#26346,.T.) ;
#35844=ORIENTED_EDGE('',*,*,#26329,.T.) ;
#35845=ORIENTED_EDGE('',*,*,#26347,.T.) ;
#35846=ORIENTED_EDGE('',*,*,#26333,.T.) ;
#35847=ORIENTED_EDGE('',*,*,#25179,.T.) ;
#35848=ORIENTED_EDGE('',*,*,#25808,.F.) ;
#35849=ORIENTED_EDGE('',*,*,#26348,.T.) ;
#35850=ORIENTED_EDGE('',*,*,#26331,.T.) ;
#35851=ORIENTED_EDGE('',*,*,#26349,.T.) ;
#35852=ORIENTED_EDGE('',*,*,#25824,.F.) ;
#35853=ORIENTED_EDGE('',*,*,#26350,.T.) ;
#35854=ORIENTED_EDGE('',*,*,#26330,.T.) ;
#35855=ORIENTED_EDGE('',*,*,#25177,.T.) ;
#35856=ORIENTED_EDGE('',*,*,#25812,.F.) ;
#35857=ORIENTED_EDGE('',*,*,#26351,.T.) ;
#35858=ORIENTED_EDGE('',*,*,#26328,.T.) ;
#35859=ORIENTED_EDGE('',*,*,#26352,.T.) ;
#35860=ORIENTED_EDGE('',*,*,#25825,.F.) ;
#35861=ORIENTED_EDGE('',*,*,#25176,.F.) ;
#35862=ORIENTED_EDGE('',*,*,#26325,.T.) ;
#35863=ORIENTED_EDGE('',*,*,#26353,.T.) ;
#35864=ORIENTED_EDGE('',*,*,#25802,.F.) ;
#35865=ORIENTED_EDGE('',*,*,#26343,.F.) ;
#35866=ORIENTED_EDGE('',*,*,#26341,.F.) ;
#35867=ORIENTED_EDGE('',*,*,#26345,.F.) ;
#35868=ORIENTED_EDGE('',*,*,#25806,.F.) ;
#35869=ORIENTED_EDGE('',*,*,#26346,.F.) ;
#35870=ORIENTED_EDGE('',*,*,#26344,.F.) ;
#35871=ORIENTED_EDGE('',*,*,#26348,.F.) ;
#35872=ORIENTED_EDGE('',*,*,#25810,.F.) ;
#35873=ORIENTED_EDGE('',*,*,#26349,.F.) ;
#35874=ORIENTED_EDGE('',*,*,#26347,.F.) ;
#35875=ORIENTED_EDGE('',*,*,#26351,.F.) ;
#35876=ORIENTED_EDGE('',*,*,#25813,.F.) ;
#35877=ORIENTED_EDGE('',*,*,#26352,.F.) ;
#35878=ORIENTED_EDGE('',*,*,#26350,.F.) ;
#35879=ORIENTED_EDGE('',*,*,#25823,.F.) ;
#35880=ORIENTED_EDGE('',*,*,#25822,.F.) ;
#35881=ORIENTED_EDGE('',*,*,#26353,.F.) ;
#35882=ORIENTED_EDGE('',*,*,#26327,.T.) ;
#35883=ORIENTED_EDGE('',*,*,#25827,.F.) ;
#35884=ORIENTED_EDGE('',*,*,#25985,.F.) ;
#35885=ORIENTED_EDGE('',*,*,#25433,.T.) ;
#35886=ORIENTED_EDGE('',*,*,#25832,.F.) ;
#35887=ORIENTED_EDGE('',*,*,#26354,.T.) ;
#35888=ORIENTED_EDGE('',*,*,#26017,.F.) ;
#35889=ORIENTED_EDGE('',*,*,#26354,.F.) ;
#35890=ORIENTED_EDGE('',*,*,#26019,.F.) ;
#35891=ORIENTED_EDGE('',*,*,#26018,.F.) ;
#35892=ORIENTED_EDGE('',*,*,#26022,.F.) ;
#35893=ORIENTED_EDGE('',*,*,#25419,.T.) ;
#35894=ORIENTED_EDGE('',*,*,#25874,.F.) ;
#35895=ORIENTED_EDGE('',*,*,#26355,.T.) ;
#35896=ORIENTED_EDGE('',*,*,#26054,.F.) ;
#35897=ORIENTED_EDGE('',*,*,#26355,.F.) ;
#35898=ORIENTED_EDGE('',*,*,#26056,.F.) ;
#35899=ORIENTED_EDGE('',*,*,#26055,.F.) ;
#35900=ORIENTED_EDGE('',*,*,#25224,.T.) ;
#35901=ORIENTED_EDGE('',*,*,#26356,.F.) ;
#35902=ORIENTED_EDGE('',*,*,#26357,.F.) ;
#35903=ORIENTED_EDGE('',*,*,#26358,.F.) ;
#35904=ORIENTED_EDGE('',*,*,#26359,.F.) ;
#35905=ORIENTED_EDGE('',*,*,#26360,.F.) ;
#35906=ORIENTED_EDGE('',*,*,#25386,.T.) ;
#35907=ORIENTED_EDGE('',*,*,#26361,.F.) ;
#35908=ORIENTED_EDGE('',*,*,#25222,.T.) ;
#35909=ORIENTED_EDGE('',*,*,#26362,.F.) ;
#35910=ORIENTED_EDGE('',*,*,#26363,.F.) ;
#35911=ORIENTED_EDGE('',*,*,#26364,.F.) ;
#35912=ORIENTED_EDGE('',*,*,#26365,.F.) ;
#35913=ORIENTED_EDGE('',*,*,#26366,.F.) ;
#35914=ORIENTED_EDGE('',*,*,#25226,.T.) ;
#35915=ORIENTED_EDGE('',*,*,#26367,.F.) ;
#35916=ORIENTED_EDGE('',*,*,#25384,.T.) ;
#35917=ORIENTED_EDGE('',*,*,#26368,.F.) ;
#35918=ORIENTED_EDGE('',*,*,#26369,.F.) ;
#35919=ORIENTED_EDGE('',*,*,#26370,.F.) ;
#35920=ORIENTED_EDGE('',*,*,#26371,.F.) ;
#35921=ORIENTED_EDGE('',*,*,#26372,.F.) ;
#35922=ORIENTED_EDGE('',*,*,#25388,.T.) ;
#35923=ORIENTED_EDGE('',*,*,#26373,.F.) ;
#35924=ORIENTED_EDGE('',*,*,#25220,.T.) ;
#35925=ORIENTED_EDGE('',*,*,#26374,.F.) ;
#35926=ORIENTED_EDGE('',*,*,#26375,.F.) ;
#35927=ORIENTED_EDGE('',*,*,#26376,.F.) ;
#35928=ORIENTED_EDGE('',*,*,#26374,.T.) ;
#35929=ORIENTED_EDGE('',*,*,#25227,.T.) ;
#35930=ORIENTED_EDGE('',*,*,#26366,.T.) ;
#35931=ORIENTED_EDGE('',*,*,#26377,.T.) ;
#35932=ORIENTED_EDGE('',*,*,#26378,.F.) ;
#35933=ORIENTED_EDGE('',*,*,#26379,.F.) ;
#35934=ORIENTED_EDGE('',*,*,#25382,.T.) ;
#35935=ORIENTED_EDGE('',*,*,#26380,.F.) ;
#35936=ORIENTED_EDGE('',*,*,#26368,.T.) ;
#35937=ORIENTED_EDGE('',*,*,#25383,.T.) ;
#35938=ORIENTED_EDGE('',*,*,#26379,.T.) ;
#35939=ORIENTED_EDGE('',*,*,#26381,.T.) ;
#35940=ORIENTED_EDGE('',*,*,#26380,.T.) ;
#35941=ORIENTED_EDGE('',*,*,#25389,.T.) ;
#35942=ORIENTED_EDGE('',*,*,#26372,.T.) ;
#35943=ORIENTED_EDGE('',*,*,#26382,.T.) ;
#35944=ORIENTED_EDGE('',*,*,#26375,.T.) ;
#35945=ORIENTED_EDGE('',*,*,#26383,.T.) ;
#35946=ORIENTED_EDGE('',*,*,#26378,.T.) ;
#35947=ORIENTED_EDGE('',*,*,#26384,.T.) ;
#35948=ORIENTED_EDGE('',*,*,#26362,.T.) ;
#35949=ORIENTED_EDGE('',*,*,#25221,.T.) ;
#35950=ORIENTED_EDGE('',*,*,#26376,.T.) ;
#35951=ORIENTED_EDGE('',*,*,#26385,.T.) ;
#35952=ORIENTED_EDGE('',*,*,#26373,.T.) ;
#35953=ORIENTED_EDGE('',*,*,#25387,.T.) ;
#35954=ORIENTED_EDGE('',*,*,#26360,.T.) ;
#35955=ORIENTED_EDGE('',*,*,#26386,.T.) ;
#35956=ORIENTED_EDGE('',*,*,#26363,.T.) ;
#35957=ORIENTED_EDGE('',*,*,#26387,.T.) ;
#35958=ORIENTED_EDGE('',*,*,#26371,.T.) ;
#35959=ORIENTED_EDGE('',*,*,#26388,.T.) ;
#35960=ORIENTED_EDGE('',*,*,#26365,.T.) ;
#35961=ORIENTED_EDGE('',*,*,#26389,.T.) ;
#35962=ORIENTED_EDGE('',*,*,#26369,.T.) ;
#35963=ORIENTED_EDGE('',*,*,#26390,.T.) ;
#35964=ORIENTED_EDGE('',*,*,#26361,.T.) ;
#35965=ORIENTED_EDGE('',*,*,#25385,.T.) ;
#35966=ORIENTED_EDGE('',*,*,#26370,.T.) ;
#35967=ORIENTED_EDGE('',*,*,#26391,.T.) ;
#35968=ORIENTED_EDGE('',*,*,#26367,.T.) ;
#35969=ORIENTED_EDGE('',*,*,#25225,.T.) ;
#35970=ORIENTED_EDGE('',*,*,#26358,.T.) ;
#35971=ORIENTED_EDGE('',*,*,#26392,.T.) ;
#35972=ORIENTED_EDGE('',*,*,#26356,.T.) ;
#35973=ORIENTED_EDGE('',*,*,#25223,.T.) ;
#35974=ORIENTED_EDGE('',*,*,#26364,.T.) ;
#35975=ORIENTED_EDGE('',*,*,#26393,.T.) ;
#35976=ORIENTED_EDGE('',*,*,#26357,.T.) ;
#35977=ORIENTED_EDGE('',*,*,#26394,.T.) ;
#35978=ORIENTED_EDGE('',*,*,#26359,.T.) ;
#35979=ORIENTED_EDGE('',*,*,#26395,.T.) ;
#35980=ORIENTED_EDGE('',*,*,#26381,.F.) ;
#35981=ORIENTED_EDGE('',*,*,#26383,.F.) ;
#35982=ORIENTED_EDGE('',*,*,#26377,.F.) ;
#35983=ORIENTED_EDGE('',*,*,#26390,.F.) ;
#35984=ORIENTED_EDGE('',*,*,#26382,.F.) ;
#35985=ORIENTED_EDGE('',*,*,#26387,.F.) ;
#35986=ORIENTED_EDGE('',*,*,#26385,.F.) ;
#35987=ORIENTED_EDGE('',*,*,#26384,.F.) ;
#35988=ORIENTED_EDGE('',*,*,#26386,.F.) ;
#35989=ORIENTED_EDGE('',*,*,#26394,.F.) ;
#35990=ORIENTED_EDGE('',*,*,#26393,.F.) ;
#35991=ORIENTED_EDGE('',*,*,#26388,.F.) ;
#35992=ORIENTED_EDGE('',*,*,#26389,.F.) ;
#35993=ORIENTED_EDGE('',*,*,#26392,.F.) ;
#35994=ORIENTED_EDGE('',*,*,#26395,.F.) ;
#35995=ORIENTED_EDGE('',*,*,#26391,.F.) ;
#35996=ORIENTED_EDGE('',*,*,#25349,.T.) ;
#35997=ORIENTED_EDGE('',*,*,#26396,.T.) ;
#35998=ORIENTED_EDGE('',*,*,#26397,.T.) ;
#35999=ORIENTED_EDGE('',*,*,#26396,.F.) ;
#36000=ORIENTED_EDGE('',*,*,#26397,.F.) ;
#36001=ORIENTED_EDGE('',*,*,#26398,.T.) ;
#36002=ORIENTED_EDGE('',*,*,#26399,.F.) ;
#36003=ORIENTED_EDGE('',*,*,#26400,.F.) ;
#36004=ORIENTED_EDGE('',*,*,#26398,.F.) ;
#36005=ORIENTED_EDGE('',*,*,#25186,.T.) ;
#36006=ORIENTED_EDGE('',*,*,#26401,.T.) ;
#36007=ORIENTED_EDGE('',*,*,#26399,.T.) ;
#36008=ORIENTED_EDGE('',*,*,#26400,.T.) ;
#36009=ORIENTED_EDGE('',*,*,#26401,.F.) ;
#36010=ORIENTED_EDGE('',*,*,#26402,.T.) ;
#36011=ORIENTED_EDGE('',*,*,#26403,.T.) ;
#36012=ORIENTED_EDGE('',*,*,#26404,.T.) ;
#36013=ORIENTED_EDGE('',*,*,#26405,.T.) ;
#36014=ORIENTED_EDGE('',*,*,#26406,.T.) ;
#36015=ORIENTED_EDGE('',*,*,#26407,.T.) ;
#36016=ORIENTED_EDGE('',*,*,#26404,.F.) ;
#36017=ORIENTED_EDGE('',*,*,#26408,.T.) ;
#36018=ORIENTED_EDGE('',*,*,#26409,.F.) ;
#36019=ORIENTED_EDGE('',*,*,#25201,.T.) ;
#36020=ORIENTED_EDGE('',*,*,#26406,.F.) ;
#36021=ORIENTED_EDGE('',*,*,#26408,.F.) ;
#36022=ORIENTED_EDGE('',*,*,#26403,.F.) ;
#36023=ORIENTED_EDGE('',*,*,#26410,.F.) ;
#36024=ORIENTED_EDGE('',*,*,#26411,.T.) ;
#36025=ORIENTED_EDGE('',*,*,#25280,.T.) ;
#36026=ORIENTED_EDGE('',*,*,#25717,.T.) ;
#36027=ORIENTED_EDGE('',*,*,#25721,.F.) ;
#36028=ORIENTED_EDGE('',*,*,#26402,.F.) ;
#36029=ORIENTED_EDGE('',*,*,#26412,.T.) ;
#36030=ORIENTED_EDGE('',*,*,#26413,.F.) ;
#36031=ORIENTED_EDGE('',*,*,#26414,.T.) ;
#36032=ORIENTED_EDGE('',*,*,#26415,.T.) ;
#36033=ORIENTED_EDGE('',*,*,#26410,.T.) ;
#36034=ORIENTED_EDGE('',*,*,#26405,.F.) ;
#36035=ORIENTED_EDGE('',*,*,#26416,.F.) ;
#36036=ORIENTED_EDGE('',*,*,#26417,.F.) ;
#36037=ORIENTED_EDGE('',*,*,#26412,.F.) ;
#36038=ORIENTED_EDGE('',*,*,#26413,.T.) ;
#36039=ORIENTED_EDGE('',*,*,#26417,.T.) ;
#36040=ORIENTED_EDGE('',*,*,#26418,.T.) ;
#36041=ORIENTED_EDGE('',*,*,#26419,.T.) ;
#36042=ORIENTED_EDGE('',*,*,#26420,.T.) ;
#36043=ORIENTED_EDGE('',*,*,#26421,.T.) ;
#36044=ORIENTED_EDGE('',*,*,#26418,.F.) ;
#36045=ORIENTED_EDGE('',*,*,#26422,.T.) ;
#36046=ORIENTED_EDGE('',*,*,#26423,.T.) ;
#36047=ORIENTED_EDGE('',*,*,#26420,.F.) ;
#36048=ORIENTED_EDGE('',*,*,#25199,.T.) ;
#36049=ORIENTED_EDGE('',*,*,#26407,.F.) ;
#36050=ORIENTED_EDGE('',*,*,#25200,.T.) ;
#36051=ORIENTED_EDGE('',*,*,#26422,.F.) ;
#36052=ORIENTED_EDGE('',*,*,#26416,.T.) ;
#36053=ORIENTED_EDGE('',*,*,#25739,.F.) ;
#36054=ORIENTED_EDGE('',*,*,#26424,.F.) ;
#36055=ORIENTED_EDGE('',*,*,#25196,.T.) ;
#36056=ORIENTED_EDGE('',*,*,#26425,.F.) ;
#36057=ORIENTED_EDGE('',*,*,#25197,.T.) ;
#36058=ORIENTED_EDGE('',*,*,#26424,.T.) ;
#36059=ORIENTED_EDGE('',*,*,#25741,.T.) ;
#36060=ORIENTED_EDGE('',*,*,#26426,.T.) ;
#36061=ORIENTED_EDGE('',*,*,#25735,.F.) ;
#36062=ORIENTED_EDGE('',*,*,#26427,.F.) ;
#36063=ORIENTED_EDGE('',*,*,#25194,.T.) ;
#36064=ORIENTED_EDGE('',*,*,#26428,.F.) ;
#36065=ORIENTED_EDGE('',*,*,#26427,.T.) ;
#36066=ORIENTED_EDGE('',*,*,#25737,.T.) ;
#36067=ORIENTED_EDGE('',*,*,#26425,.T.) ;
#36068=ORIENTED_EDGE('',*,*,#25195,.T.) ;
#36069=ORIENTED_EDGE('',*,*,#25731,.F.) ;
#36070=ORIENTED_EDGE('',*,*,#26429,.F.) ;
#36071=ORIENTED_EDGE('',*,*,#25192,.T.) ;
#36072=ORIENTED_EDGE('',*,*,#26430,.F.) ;
#36073=ORIENTED_EDGE('',*,*,#26428,.T.) ;
#36074=ORIENTED_EDGE('',*,*,#25193,.T.) ;
#36075=ORIENTED_EDGE('',*,*,#26429,.T.) ;
#36076=ORIENTED_EDGE('',*,*,#25733,.T.) ;
#36077=ORIENTED_EDGE('',*,*,#25727,.F.) ;
#36078=ORIENTED_EDGE('',*,*,#26431,.F.) ;
#36079=ORIENTED_EDGE('',*,*,#25190,.T.) ;
#36080=ORIENTED_EDGE('',*,*,#26432,.F.) ;
#36081=ORIENTED_EDGE('',*,*,#26431,.T.) ;
#36082=ORIENTED_EDGE('',*,*,#25729,.T.) ;
#36083=ORIENTED_EDGE('',*,*,#26430,.T.) ;
#36084=ORIENTED_EDGE('',*,*,#25191,.T.) ;
#36085=ORIENTED_EDGE('',*,*,#25723,.F.) ;
#36086=ORIENTED_EDGE('',*,*,#26433,.F.) ;
#36087=ORIENTED_EDGE('',*,*,#25188,.T.) ;
#36088=ORIENTED_EDGE('',*,*,#26434,.F.) ;
#36089=ORIENTED_EDGE('',*,*,#26432,.T.) ;
#36090=ORIENTED_EDGE('',*,*,#25189,.T.) ;
#36091=ORIENTED_EDGE('',*,*,#26433,.T.) ;
#36092=ORIENTED_EDGE('',*,*,#25725,.T.) ;
#36093=ORIENTED_EDGE('',*,*,#25720,.T.) ;
#36094=ORIENTED_EDGE('',*,*,#26434,.T.) ;
#36095=ORIENTED_EDGE('',*,*,#25187,.F.) ;
#36096=ORIENTED_EDGE('',*,*,#26409,.T.) ;
#36097=ORIENTED_EDGE('',*,*,#26435,.T.) ;
#36098=ORIENTED_EDGE('',*,*,#26423,.F.) ;
#36099=ORIENTED_EDGE('',*,*,#25198,.F.) ;
#36100=ORIENTED_EDGE('',*,*,#26426,.F.) ;
#36101=ORIENTED_EDGE('',*,*,#25068,.T.) ;
#36102=ORIENTED_EDGE('',*,*,#26436,.T.) ;
#36103=ORIENTED_EDGE('',*,*,#26437,.T.) ;
#36104=ORIENTED_EDGE('',*,*,#26438,.T.) ;
#36105=ORIENTED_EDGE('',*,*,#26436,.F.) ;
#36106=ORIENTED_EDGE('',*,*,#25067,.T.) ;
#36107=ORIENTED_EDGE('',*,*,#25350,.F.) ;
#36108=ORIENTED_EDGE('',*,*,#26439,.T.) ;
#36109=ORIENTED_EDGE('',*,*,#26437,.F.) ;
#36110=ORIENTED_EDGE('',*,*,#26438,.F.) ;
#36111=ORIENTED_EDGE('',*,*,#26439,.F.) ;
#36112=ORIENTED_EDGE('',*,*,#25219,.T.) ;
#36113=ORIENTED_EDGE('',*,*,#26440,.T.) ;
#36114=ORIENTED_EDGE('',*,*,#26441,.T.) ;
#36115=ORIENTED_EDGE('',*,*,#26442,.T.) ;
#36116=ORIENTED_EDGE('',*,*,#26440,.F.) ;
#36117=ORIENTED_EDGE('',*,*,#25367,.F.) ;
#36118=ORIENTED_EDGE('',*,*,#26443,.T.) ;
#36119=ORIENTED_EDGE('',*,*,#26441,.F.) ;
#36120=ORIENTED_EDGE('',*,*,#26442,.F.) ;
#36121=ORIENTED_EDGE('',*,*,#26443,.F.) ;
#36122=ORIENTED_EDGE('',*,*,#25485,.F.) ;
#36123=ORIENTED_EDGE('',*,*,#25492,.T.) ;
#36124=ORIENTED_EDGE('',*,*,#26444,.T.) ;
#36125=ORIENTED_EDGE('',*,*,#25301,.T.) ;
#36126=ORIENTED_EDGE('',*,*,#26445,.T.) ;
#36127=ORIENTED_EDGE('',*,*,#25302,.T.) ;
#36128=ORIENTED_EDGE('',*,*,#26444,.F.) ;
#36129=ORIENTED_EDGE('',*,*,#26446,.T.) ;
#36130=ORIENTED_EDGE('',*,*,#26447,.T.) ;
#36131=ORIENTED_EDGE('',*,*,#25303,.T.) ;
#36132=ORIENTED_EDGE('',*,*,#26445,.F.) ;
#36133=ORIENTED_EDGE('',*,*,#26142,.T.) ;
#36134=ORIENTED_EDGE('',*,*,#26448,.T.) ;
#36135=ORIENTED_EDGE('',*,*,#25304,.T.) ;
#36136=ORIENTED_EDGE('',*,*,#26447,.F.) ;
#36137=ORIENTED_EDGE('',*,*,#26145,.T.) ;
#36138=ORIENTED_EDGE('',*,*,#26449,.T.) ;
#36139=ORIENTED_EDGE('',*,*,#25305,.T.) ;
#36140=ORIENTED_EDGE('',*,*,#26448,.F.) ;
#36141=ORIENTED_EDGE('',*,*,#26147,.T.) ;
#36142=ORIENTED_EDGE('',*,*,#26450,.T.) ;
#36143=ORIENTED_EDGE('',*,*,#25306,.T.) ;
#36144=ORIENTED_EDGE('',*,*,#26449,.F.) ;
#36145=ORIENTED_EDGE('',*,*,#26149,.T.) ;
#36146=ORIENTED_EDGE('',*,*,#26451,.T.) ;
#36147=ORIENTED_EDGE('',*,*,#25307,.T.) ;
#36148=ORIENTED_EDGE('',*,*,#26450,.F.) ;
#36149=ORIENTED_EDGE('',*,*,#26151,.T.) ;
#36150=ORIENTED_EDGE('',*,*,#26452,.T.) ;
#36151=ORIENTED_EDGE('',*,*,#25308,.T.) ;
#36152=ORIENTED_EDGE('',*,*,#26451,.F.) ;
#36153=ORIENTED_EDGE('',*,*,#26153,.T.) ;
#36154=ORIENTED_EDGE('',*,*,#26453,.T.) ;
#36155=ORIENTED_EDGE('',*,*,#25309,.T.) ;
#36156=ORIENTED_EDGE('',*,*,#26452,.F.) ;
#36157=ORIENTED_EDGE('',*,*,#26155,.T.) ;
#36158=ORIENTED_EDGE('',*,*,#26454,.T.) ;
#36159=ORIENTED_EDGE('',*,*,#25310,.T.) ;
#36160=ORIENTED_EDGE('',*,*,#26453,.F.) ;
#36161=ORIENTED_EDGE('',*,*,#26157,.T.) ;
#36162=ORIENTED_EDGE('',*,*,#26455,.T.) ;
#36163=ORIENTED_EDGE('',*,*,#25311,.T.) ;
#36164=ORIENTED_EDGE('',*,*,#26454,.F.) ;
#36165=ORIENTED_EDGE('',*,*,#26159,.T.) ;
#36166=ORIENTED_EDGE('',*,*,#26456,.T.) ;
#36167=ORIENTED_EDGE('',*,*,#25312,.T.) ;
#36168=ORIENTED_EDGE('',*,*,#26455,.F.) ;
#36169=ORIENTED_EDGE('',*,*,#26161,.T.) ;
#36170=ORIENTED_EDGE('',*,*,#26457,.T.) ;
#36171=ORIENTED_EDGE('',*,*,#25313,.T.) ;
#36172=ORIENTED_EDGE('',*,*,#26456,.F.) ;
#36173=ORIENTED_EDGE('',*,*,#26163,.T.) ;
#36174=ORIENTED_EDGE('',*,*,#26458,.T.) ;
#36175=ORIENTED_EDGE('',*,*,#25314,.T.) ;
#36176=ORIENTED_EDGE('',*,*,#26457,.F.) ;
#36177=ORIENTED_EDGE('',*,*,#26165,.T.) ;
#36178=ORIENTED_EDGE('',*,*,#26459,.T.) ;
#36179=ORIENTED_EDGE('',*,*,#25315,.T.) ;
#36180=ORIENTED_EDGE('',*,*,#26458,.F.) ;
#36181=ORIENTED_EDGE('',*,*,#26167,.T.) ;
#36182=ORIENTED_EDGE('',*,*,#26460,.T.) ;
#36183=ORIENTED_EDGE('',*,*,#25316,.T.) ;
#36184=ORIENTED_EDGE('',*,*,#26459,.F.) ;
#36185=ORIENTED_EDGE('',*,*,#26169,.T.) ;
#36186=ORIENTED_EDGE('',*,*,#26461,.T.) ;
#36187=ORIENTED_EDGE('',*,*,#25317,.T.) ;
#36188=ORIENTED_EDGE('',*,*,#26460,.F.) ;
#36189=ORIENTED_EDGE('',*,*,#26171,.T.) ;
#36190=ORIENTED_EDGE('',*,*,#26462,.T.) ;
#36191=ORIENTED_EDGE('',*,*,#25318,.T.) ;
#36192=ORIENTED_EDGE('',*,*,#26461,.F.) ;
#36193=ORIENTED_EDGE('',*,*,#26173,.T.) ;
#36194=ORIENTED_EDGE('',*,*,#26463,.T.) ;
#36195=ORIENTED_EDGE('',*,*,#25319,.T.) ;
#36196=ORIENTED_EDGE('',*,*,#26462,.F.) ;
#36197=ORIENTED_EDGE('',*,*,#26175,.T.) ;
#36198=ORIENTED_EDGE('',*,*,#26464,.T.) ;
#36199=ORIENTED_EDGE('',*,*,#25320,.T.) ;
#36200=ORIENTED_EDGE('',*,*,#26463,.F.) ;
#36201=ORIENTED_EDGE('',*,*,#26177,.T.) ;
#36202=ORIENTED_EDGE('',*,*,#26465,.T.) ;
#36203=ORIENTED_EDGE('',*,*,#25321,.T.) ;
#36204=ORIENTED_EDGE('',*,*,#26464,.F.) ;
#36205=ORIENTED_EDGE('',*,*,#26179,.T.) ;
#36206=ORIENTED_EDGE('',*,*,#26466,.T.) ;
#36207=ORIENTED_EDGE('',*,*,#25322,.T.) ;
#36208=ORIENTED_EDGE('',*,*,#26465,.F.) ;
#36209=ORIENTED_EDGE('',*,*,#26181,.T.) ;
#36210=ORIENTED_EDGE('',*,*,#26467,.T.) ;
#36211=ORIENTED_EDGE('',*,*,#25323,.T.) ;
#36212=ORIENTED_EDGE('',*,*,#26466,.F.) ;
#36213=ORIENTED_EDGE('',*,*,#26183,.T.) ;
#36214=ORIENTED_EDGE('',*,*,#26187,.T.) ;
#36215=ORIENTED_EDGE('',*,*,#25324,.T.) ;
#36216=ORIENTED_EDGE('',*,*,#26467,.F.) ;
#36217=ORIENTED_EDGE('',*,*,#26185,.T.) ;
#36218=ORIENTED_EDGE('',*,*,#26082,.F.) ;
#36219=ORIENTED_EDGE('',*,*,#26143,.T.) ;
#36220=ORIENTED_EDGE('',*,*,#26446,.F.) ;
#36221=ORIENTED_EDGE('',*,*,#25491,.T.) ;
#36222=ORIENTED_EDGE('',*,*,#26468,.T.) ;
#36223=ORIENTED_EDGE('',*,*,#26469,.T.) ;
#36224=ORIENTED_EDGE('',*,*,#25628,.F.) ;
#36225=ORIENTED_EDGE('',*,*,#25332,.T.) ;
#36226=ORIENTED_EDGE('',*,*,#26470,.T.) ;
#36227=ORIENTED_EDGE('',*,*,#26471,.T.) ;
#36228=ORIENTED_EDGE('',*,*,#26468,.F.) ;
#36229=ORIENTED_EDGE('',*,*,#25331,.T.) ;
#36230=ORIENTED_EDGE('',*,*,#26472,.T.) ;
#36231=ORIENTED_EDGE('',*,*,#26473,.T.) ;
#36232=ORIENTED_EDGE('',*,*,#26470,.F.) ;
#36233=ORIENTED_EDGE('',*,*,#25330,.T.) ;
#36234=ORIENTED_EDGE('',*,*,#26129,.F.) ;
#36235=ORIENTED_EDGE('',*,*,#26474,.T.) ;
#36236=ORIENTED_EDGE('',*,*,#26472,.F.) ;
#36237=ORIENTED_EDGE('',*,*,#25329,.T.) ;
#36238=ORIENTED_EDGE('',*,*,#25530,.T.) ;
#36239=ORIENTED_EDGE('',*,*,#26475,.T.) ;
#36240=ORIENTED_EDGE('',*,*,#26476,.T.) ;
#36241=ORIENTED_EDGE('',*,*,#26475,.F.) ;
#36242=ORIENTED_EDGE('',*,*,#26477,.F.) ;
#36243=ORIENTED_EDGE('',*,*,#26476,.F.) ;
#36244=ORIENTED_EDGE('',*,*,#26478,.T.) ;
#36245=ORIENTED_EDGE('',*,*,#26479,.T.) ;
#36246=ORIENTED_EDGE('',*,*,#26477,.T.) ;
#36247=ORIENTED_EDGE('',*,*,#26479,.F.) ;
#36248=ORIENTED_EDGE('',*,*,#26480,.T.) ;
#36249=ORIENTED_EDGE('',*,*,#26481,.F.) ;
#36250=ORIENTED_EDGE('',*,*,#26482,.T.) ;
#36251=ORIENTED_EDGE('',*,*,#26480,.F.) ;
#36252=ORIENTED_EDGE('',*,*,#26478,.F.) ;
#36253=ORIENTED_EDGE('',*,*,#26482,.F.) ;
#36254=ORIENTED_EDGE('',*,*,#26481,.T.) ;
#36255=ORIENTED_EDGE('',*,*,#26483,.T.) ;
#36256=ORIENTED_EDGE('',*,*,#26484,.T.) ;
#36257=ORIENTED_EDGE('',*,*,#26485,.T.) ;
#36258=ORIENTED_EDGE('',*,*,#26483,.F.) ;
#36259=ORIENTED_EDGE('',*,*,#26486,.T.) ;
#36260=ORIENTED_EDGE('',*,*,#26487,.T.) ;
#36261=ORIENTED_EDGE('',*,*,#26488,.T.) ;
#36262=ORIENTED_EDGE('',*,*,#26489,.T.) ;
#36263=ORIENTED_EDGE('',*,*,#26487,.F.) ;
#36264=ORIENTED_EDGE('',*,*,#26486,.F.) ;
#36265=ORIENTED_EDGE('',*,*,#26490,.T.) ;
#36266=ORIENTED_EDGE('',*,*,#26491,.F.) ;
#36267=ORIENTED_EDGE('',*,*,#26492,.F.) ;
#36268=ORIENTED_EDGE('',*,*,#26490,.F.) ;
#36269=ORIENTED_EDGE('',*,*,#26491,.T.) ;
#36270=ORIENTED_EDGE('',*,*,#26492,.T.) ;
#36271=ORIENTED_EDGE('',*,*,#26493,.T.) ;
#36272=ORIENTED_EDGE('',*,*,#26494,.T.) ;
#36273=ORIENTED_EDGE('',*,*,#26493,.F.) ;
#36274=ORIENTED_EDGE('',*,*,#26494,.F.) ;
#36275=ORIENTED_EDGE('',*,*,#26495,.F.) ;
#36276=ORIENTED_EDGE('',*,*,#26496,.T.) ;
#36277=ORIENTED_EDGE('',*,*,#26497,.T.) ;
#36278=ORIENTED_EDGE('',*,*,#26495,.T.) ;
#36279=ORIENTED_EDGE('',*,*,#26497,.F.) ;
#36280=ORIENTED_EDGE('',*,*,#26498,.T.) ;
#36281=ORIENTED_EDGE('',*,*,#26499,.T.) ;
#36282=ORIENTED_EDGE('',*,*,#26496,.F.) ;
#36283=ORIENTED_EDGE('',*,*,#26499,.F.) ;
#36284=ORIENTED_EDGE('',*,*,#26500,.T.) ;
#36285=ORIENTED_EDGE('',*,*,#26501,.T.) ;
#36286=ORIENTED_EDGE('',*,*,#26502,.T.) ;
#36287=ORIENTED_EDGE('',*,*,#26503,.T.) ;
#36288=ORIENTED_EDGE('',*,*,#26501,.F.) ;
#36289=ORIENTED_EDGE('',*,*,#26500,.F.) ;
#36290=ORIENTED_EDGE('',*,*,#26504,.T.) ;
#36291=ORIENTED_EDGE('',*,*,#26505,.F.) ;
#36292=ORIENTED_EDGE('',*,*,#26506,.F.) ;
#36293=ORIENTED_EDGE('',*,*,#26504,.F.) ;
#36294=ORIENTED_EDGE('',*,*,#25270,.T.) ;
#36295=ORIENTED_EDGE('',*,*,#26507,.T.) ;
#36296=ORIENTED_EDGE('',*,*,#26508,.T.) ;
#36297=ORIENTED_EDGE('',*,*,#26507,.F.) ;
#36298=ORIENTED_EDGE('',*,*,#26509,.F.) ;
#36299=ORIENTED_EDGE('',*,*,#26508,.F.) ;
#36300=ORIENTED_EDGE('',*,*,#26505,.T.) ;
#36301=ORIENTED_EDGE('',*,*,#26506,.T.) ;
#36302=ORIENTED_EDGE('',*,*,#26510,.T.) ;
#36303=ORIENTED_EDGE('',*,*,#26509,.T.) ;
#36304=ORIENTED_EDGE('',*,*,#26510,.F.) ;
#36305=ORIENTED_EDGE('',*,*,#26485,.F.) ;
#36306=ORIENTED_EDGE('',*,*,#26511,.T.) ;
#36307=ORIENTED_EDGE('',*,*,#25202,.T.) ;
#36308=ORIENTED_EDGE('',*,*,#26511,.F.) ;
#36309=ORIENTED_EDGE('',*,*,#26484,.F.) ;
#36310=ORIENTED_EDGE('',*,*,#26489,.F.) ;
#36311=ORIENTED_EDGE('',*,*,#26512,.T.) ;
#36312=ORIENTED_EDGE('',*,*,#25218,.T.) ;
#36313=ORIENTED_EDGE('',*,*,#26512,.F.) ;
#36314=ORIENTED_EDGE('',*,*,#26488,.F.) ;
#36315=ORIENTED_EDGE('',*,*,#26503,.F.) ;
#36316=ORIENTED_EDGE('',*,*,#26513,.T.) ;
#36317=ORIENTED_EDGE('',*,*,#25203,.T.) ;
#36318=ORIENTED_EDGE('',*,*,#26513,.F.) ;
#36319=ORIENTED_EDGE('',*,*,#26502,.F.) ;
#36320=ORIENTED_EDGE('',*,*,#25519,.F.) ;
#36321=ORIENTED_EDGE('',*,*,#26498,.F.) ;
#36322=ORIENTED_EDGE('',*,*,#26074,.F.) ;
#36323=ORIENTED_EDGE('',*,*,#26514,.T.) ;
#36324=ORIENTED_EDGE('',*,*,#26473,.F.) ;
#36325=ORIENTED_EDGE('',*,*,#26515,.T.) ;
#36326=ORIENTED_EDGE('',*,*,#26072,.F.) ;
#36327=ORIENTED_EDGE('',*,*,#26516,.F.) ;
#36328=ORIENTED_EDGE('',*,*,#26471,.F.) ;
#36329=ORIENTED_EDGE('',*,*,#26514,.F.) ;
#36330=ORIENTED_EDGE('',*,*,#26070,.F.) ;
#36331=ORIENTED_EDGE('',*,*,#25512,.T.) ;
#36332=ORIENTED_EDGE('',*,*,#26469,.F.) ;
#36333=ORIENTED_EDGE('',*,*,#26516,.T.) ;
#36334=ORIENTED_EDGE('',*,*,#26237,.F.) ;
#36335=ORIENTED_EDGE('',*,*,#25374,.T.) ;
#36336=ORIENTED_EDGE('',*,*,#26240,.F.) ;
#36337=ORIENTED_EDGE('',*,*,#26229,.F.) ;
#36338=ORIENTED_EDGE('',*,*,#26239,.F.) ;
#36339=ORIENTED_EDGE('',*,*,#25372,.F.) ;
#36340=ORIENTED_EDGE('',*,*,#26242,.F.) ;
#36341=ORIENTED_EDGE('',*,*,#26225,.F.) ;
#36342=ORIENTED_EDGE('',*,*,#26241,.F.) ;
#36343=ORIENTED_EDGE('',*,*,#25370,.T.) ;
#36344=ORIENTED_EDGE('',*,*,#26244,.F.) ;
#36345=ORIENTED_EDGE('',*,*,#26221,.F.) ;
#36346=ORIENTED_EDGE('',*,*,#26243,.F.) ;
#36347=ORIENTED_EDGE('',*,*,#25368,.F.) ;
#36348=ORIENTED_EDGE('',*,*,#26246,.F.) ;
#36349=ORIENTED_EDGE('',*,*,#26217,.F.) ;
#36350=ORIENTED_EDGE('',*,*,#25817,.F.) ;
#36351=ORIENTED_EDGE('',*,*,#26340,.F.) ;
#36352=ORIENTED_EDGE('',*,*,#26342,.F.) ;
#36353=ORIENTED_EDGE('',*,*,#25798,.F.) ;
#36354=ORIENTED_EDGE('',*,*,#26517,.T.) ;
#36355=ORIENTED_EDGE('',*,*,#26518,.T.) ;
#36356=ORIENTED_EDGE('',*,*,#26519,.T.) ;
#36357=ORIENTED_EDGE('',*,*,#26520,.T.) ;
#36358=ORIENTED_EDGE('',*,*,#26521,.T.) ;
#36359=ORIENTED_EDGE('',*,*,#26522,.T.) ;
#36360=ORIENTED_EDGE('',*,*,#26523,.T.) ;
#36361=ORIENTED_EDGE('',*,*,#26524,.T.) ;
#36362=ORIENTED_EDGE('',*,*,#26525,.T.) ;
#36363=ORIENTED_EDGE('',*,*,#26526,.T.) ;
#36364=ORIENTED_EDGE('',*,*,#26527,.T.) ;
#36365=ORIENTED_EDGE('',*,*,#26528,.T.) ;
#36366=ORIENTED_EDGE('',*,*,#26529,.T.) ;
#36367=ORIENTED_EDGE('',*,*,#26530,.T.) ;
#36368=ORIENTED_EDGE('',*,*,#26531,.T.) ;
#36369=ORIENTED_EDGE('',*,*,#26140,.T.) ;
#36370=ORIENTED_EDGE('',*,*,#26139,.T.) ;
#36371=ORIENTED_EDGE('',*,*,#26532,.T.) ;
#36372=ORIENTED_EDGE('',*,*,#26530,.F.) ;
#36373=ORIENTED_EDGE('',*,*,#26533,.T.) ;
#36374=ORIENTED_EDGE('',*,*,#26534,.T.) ;
#36375=ORIENTED_EDGE('',*,*,#25061,.T.) ;
#36376=ORIENTED_EDGE('',*,*,#26531,.F.) ;
#36377=ORIENTED_EDGE('',*,*,#26535,.T.) ;
#36378=ORIENTED_EDGE('',*,*,#25062,.T.) ;
#36379=ORIENTED_EDGE('',*,*,#26534,.F.) ;
#36380=ORIENTED_EDGE('',*,*,#26536,.T.) ;
#36381=ORIENTED_EDGE('',*,*,#26537,.T.) ;
#36382=ORIENTED_EDGE('',*,*,#25063,.T.) ;
#36383=ORIENTED_EDGE('',*,*,#26535,.F.) ;
#36384=ORIENTED_EDGE('',*,*,#25538,.T.) ;
#36385=ORIENTED_EDGE('',*,*,#26538,.T.) ;
#36386=ORIENTED_EDGE('',*,*,#25064,.T.) ;
#36387=ORIENTED_EDGE('',*,*,#26537,.F.) ;
#36388=ORIENTED_EDGE('',*,*,#26539,.T.) ;
#36389=ORIENTED_EDGE('',*,*,#26527,.F.) ;
#36390=ORIENTED_EDGE('',*,*,#25065,.T.) ;
#36391=ORIENTED_EDGE('',*,*,#26538,.F.) ;
#36392=ORIENTED_EDGE('',*,*,#26540,.T.) ;
#36393=ORIENTED_EDGE('',*,*,#26528,.F.) ;
#36394=ORIENTED_EDGE('',*,*,#26522,.F.) ;
#36395=ORIENTED_EDGE('',*,*,#25069,.T.) ;
#36396=ORIENTED_EDGE('',*,*,#25066,.T.) ;
#36397=ORIENTED_EDGE('',*,*,#26526,.F.) ;
#36398=ORIENTED_EDGE('',*,*,#26525,.F.) ;
#36399=ORIENTED_EDGE('',*,*,#25590,.T.) ;
#36400=ORIENTED_EDGE('',*,*,#26523,.F.) ;
#36401=ORIENTED_EDGE('',*,*,#26520,.F.) ;
#36402=ORIENTED_EDGE('',*,*,#26541,.T.) ;
#36403=ORIENTED_EDGE('',*,*,#26542,.T.) ;
#36404=ORIENTED_EDGE('',*,*,#25070,.T.) ;
#36405=ORIENTED_EDGE('',*,*,#26521,.F.) ;
#36406=ORIENTED_EDGE('',*,*,#26543,.T.) ;
#36407=ORIENTED_EDGE('',*,*,#25071,.T.) ;
#36408=ORIENTED_EDGE('',*,*,#26542,.F.) ;
#36409=ORIENTED_EDGE('',*,*,#26544,.T.) ;
#36410=ORIENTED_EDGE('',*,*,#26545,.T.) ;
#36411=ORIENTED_EDGE('',*,*,#25072,.T.) ;
#36412=ORIENTED_EDGE('',*,*,#26543,.F.) ;
#36413=ORIENTED_EDGE('',*,*,#25558,.T.) ;
#36414=ORIENTED_EDGE('',*,*,#26546,.T.) ;
#36415=ORIENTED_EDGE('',*,*,#25073,.T.) ;
#36416=ORIENTED_EDGE('',*,*,#26545,.F.) ;
#36417=ORIENTED_EDGE('',*,*,#26547,.T.) ;
#36418=ORIENTED_EDGE('',*,*,#26518,.F.) ;
#36419=ORIENTED_EDGE('',*,*,#25074,.T.) ;
#36420=ORIENTED_EDGE('',*,*,#26546,.F.) ;
#36421=ORIENTED_EDGE('',*,*,#26548,.T.) ;
#36422=ORIENTED_EDGE('',*,*,#26067,.F.) ;
#36423=ORIENTED_EDGE('',*,*,#25075,.T.) ;
#36424=ORIENTED_EDGE('',*,*,#26517,.F.) ;
#36425=ORIENTED_EDGE('',*,*,#25585,.T.) ;
#36426=ORIENTED_EDGE('',*,*,#26547,.F.) ;
#36427=ORIENTED_EDGE('',*,*,#25563,.T.) ;
#36428=ORIENTED_EDGE('',*,*,#26549,.T.) ;
#36429=ORIENTED_EDGE('',*,*,#26550,.T.) ;
#36430=ORIENTED_EDGE('',*,*,#26544,.F.) ;
#36431=ORIENTED_EDGE('',*,*,#26551,.T.) ;
#36432=ORIENTED_EDGE('',*,*,#26552,.T.) ;
#36433=ORIENTED_EDGE('',*,*,#25559,.T.) ;
#36434=ORIENTED_EDGE('',*,*,#26541,.F.) ;
#36435=ORIENTED_EDGE('',*,*,#26553,.F.) ;
#36436=ORIENTED_EDGE('',*,*,#26551,.F.) ;
#36437=ORIENTED_EDGE('',*,*,#26524,.F.) ;
#36438=ORIENTED_EDGE('',*,*,#25589,.T.) ;
#36439=ORIENTED_EDGE('',*,*,#26554,.F.) ;
#36440=ORIENTED_EDGE('',*,*,#26553,.T.) ;
#36441=ORIENTED_EDGE('',*,*,#26529,.F.) ;
#36442=ORIENTED_EDGE('',*,*,#26555,.T.) ;
#36443=ORIENTED_EDGE('',*,*,#26556,.F.) ;
#36444=ORIENTED_EDGE('',*,*,#25591,.T.) ;
#36445=ORIENTED_EDGE('',*,*,#26540,.F.) ;
#36446=ORIENTED_EDGE('',*,*,#26557,.F.) ;
#36447=ORIENTED_EDGE('',*,*,#26555,.F.) ;
#36448=ORIENTED_EDGE('',*,*,#26539,.F.) ;
#36449=ORIENTED_EDGE('',*,*,#25543,.T.) ;
#36450=ORIENTED_EDGE('',*,*,#26558,.T.) ;
#36451=ORIENTED_EDGE('',*,*,#26557,.T.) ;
#36452=ORIENTED_EDGE('',*,*,#26536,.F.) ;
#36453=ORIENTED_EDGE('',*,*,#26559,.T.) ;
#36454=ORIENTED_EDGE('',*,*,#26560,.T.) ;
#36455=ORIENTED_EDGE('',*,*,#25539,.T.) ;
#36456=ORIENTED_EDGE('',*,*,#26533,.F.) ;
#36457=ORIENTED_EDGE('',*,*,#26561,.F.) ;
#36458=ORIENTED_EDGE('',*,*,#26559,.F.) ;
#36459=ORIENTED_EDGE('',*,*,#26532,.F.) ;
#36460=ORIENTED_EDGE('',*,*,#25594,.T.) ;
#36461=ORIENTED_EDGE('',*,*,#26562,.F.) ;
#36462=ORIENTED_EDGE('',*,*,#26561,.T.) ;
#36463=ORIENTED_EDGE('',*,*,#26293,.F.) ;
#36464=ORIENTED_EDGE('',*,*,#25693,.F.) ;
#36465=ORIENTED_EDGE('',*,*,#26563,.F.) ;
#36466=ORIENTED_EDGE('',*,*,#26564,.F.) ;
#36467=ORIENTED_EDGE('',*,*,#26291,.F.) ;
#36468=ORIENTED_EDGE('',*,*,#25391,.F.) ;
#36469=ORIENTED_EDGE('',*,*,#26287,.F.) ;
#36470=ORIENTED_EDGE('',*,*,#26565,.F.) ;
#36471=ORIENTED_EDGE('',*,*,#26563,.T.) ;
#36472=ORIENTED_EDGE('',*,*,#26279,.F.) ;
#36473=ORIENTED_EDGE('',*,*,#26296,.T.) ;
#36474=ORIENTED_EDGE('',*,*,#26288,.F.) ;
#36475=ORIENTED_EDGE('',*,*,#26564,.T.) ;
#36476=ORIENTED_EDGE('',*,*,#26565,.T.) ;
#36477=ORIENTED_EDGE('',*,*,#26286,.T.) ;
#36478=ORIENTED_EDGE('',*,*,#26421,.F.) ;
#36479=ORIENTED_EDGE('',*,*,#26566,.F.) ;
#36480=ORIENTED_EDGE('',*,*,#26567,.F.) ;
#36481=ORIENTED_EDGE('',*,*,#26414,.F.) ;
#36482=ORIENTED_EDGE('',*,*,#26419,.F.) ;
#36483=ORIENTED_EDGE('',*,*,#25281,.F.) ;
#36484=ORIENTED_EDGE('',*,*,#26411,.F.) ;
#36485=ORIENTED_EDGE('',*,*,#26415,.F.) ;
#36486=ORIENTED_EDGE('',*,*,#26567,.T.) ;
#36487=ORIENTED_EDGE('',*,*,#26435,.F.) ;
#36488=ORIENTED_EDGE('',*,*,#25740,.F.) ;
#36489=ORIENTED_EDGE('',*,*,#25706,.F.) ;
#36490=ORIENTED_EDGE('',*,*,#25282,.F.) ;
#36491=ORIENTED_EDGE('',*,*,#26566,.T.) ;
#36492=ORIENTED_EDGE('',*,*,#26193,.F.) ;
#36493=ORIENTED_EDGE('',*,*,#26568,.F.) ;
#36494=ORIENTED_EDGE('',*,*,#26569,.F.) ;
#36495=ORIENTED_EDGE('',*,*,#26200,.F.) ;
#36496=ORIENTED_EDGE('',*,*,#26191,.F.) ;
#36497=ORIENTED_EDGE('',*,*,#25379,.F.) ;
#36498=ORIENTED_EDGE('',*,*,#26209,.F.) ;
#36499=ORIENTED_EDGE('',*,*,#26201,.F.) ;
#36500=ORIENTED_EDGE('',*,*,#26569,.T.) ;
#36501=ORIENTED_EDGE('',*,*,#26245,.F.) ;
#36502=ORIENTED_EDGE('',*,*,#25380,.F.) ;
#36503=ORIENTED_EDGE('',*,*,#26568,.T.) ;
#36504=ORIENTED_EDGE('',*,*,#26247,.F.) ;
#36505=ORIENTED_EDGE('',*,*,#26310,.F.) ;
#36506=ORIENTED_EDGE('',*,*,#25828,.F.) ;
#36507=ORIENTED_EDGE('',*,*,#25814,.F.) ;
#36508=ORIENTED_EDGE('',*,*,#25351,.T.) ;
#36509=ORIENTED_EDGE('',*,*,#26570,.F.) ;
#36510=ORIENTED_EDGE('',*,*,#26317,.F.) ;
#36511=ORIENTED_EDGE('',*,*,#26308,.F.) ;
#36512=ORIENTED_EDGE('',*,*,#25366,.F.) ;
#36513=ORIENTED_EDGE('',*,*,#26326,.F.) ;
#36514=ORIENTED_EDGE('',*,*,#26318,.F.) ;
#36515=ORIENTED_EDGE('',*,*,#26570,.T.) ;
#36516=ORIENTED_EDGE('',*,*,#25662,.F.) ;
#36517=ORIENTED_EDGE('',*,*,#25404,.F.) ;
#36518=ORIENTED_EDGE('',*,*,#25669,.F.) ;
#36519=ORIENTED_EDGE('',*,*,#25667,.F.) ;
#36520=ORIENTED_EDGE('',*,*,#25658,.F.) ;
#36521=ORIENTED_EDGE('',*,*,#25664,.F.) ;
#36522=ORIENTED_EDGE('',*,*,#25958,.F.) ;
#36523=ORIENTED_EDGE('',*,*,#25982,.F.) ;
#36524=ORIENTED_EDGE('',*,*,#25981,.F.) ;
#36525=ORIENTED_EDGE('',*,*,#25980,.F.) ;
#36526=ORIENTED_EDGE('',*,*,#25771,.F.) ;
#36527=ORIENTED_EDGE('',*,*,#26278,.F.) ;
#36528=ORIENTED_EDGE('',*,*,#26276,.F.) ;
#36529=ORIENTED_EDGE('',*,*,#26274,.F.) ;
#36530=ORIENTED_EDGE('',*,*,#25767,.F.) ;
#36531=ORIENTED_EDGE('',*,*,#26275,.F.) ;
#36532=ORIENTED_EDGE('',*,*,#26266,.F.) ;
#36533=ORIENTED_EDGE('',*,*,#26273,.F.) ;
#36534=ORIENTED_EDGE('',*,*,#26130,.F.) ;
#36535=ORIENTED_EDGE('',*,*,#25327,.F.) ;
#36536=ORIENTED_EDGE('',*,*,#26138,.F.) ;
#36537=ORIENTED_EDGE('',*,*,#26136,.F.) ;
#36538=ORIENTED_EDGE('',*,*,#26133,.F.) ;
#36539=ORIENTED_EDGE('',*,*,#26132,.F.) ;
#36540=ORIENTED_EDGE('',*,*,#26075,.F.) ;
#36541=ORIENTED_EDGE('',*,*,#26515,.F.) ;
#36542=ORIENTED_EDGE('',*,*,#26474,.F.) ;
#36543=ORIENTED_EDGE('',*,*,#26131,.F.) ;
#36544=ORIENTED_EDGE('',*,*,#25618,.T.) ;
#36545=ORIENTED_EDGE('',*,*,#25610,.T.) ;
#36546=ORIENTED_EDGE('',*,*,#26571,.F.) ;
#36547=ORIENTED_EDGE('',*,*,#25570,.F.) ;
#36548=ORIENTED_EDGE('',*,*,#25291,.F.) ;
#36549=ORIENTED_EDGE('',*,*,#25604,.T.) ;
#36550=ORIENTED_EDGE('',*,*,#26572,.F.) ;
#36551=ORIENTED_EDGE('',*,*,#25548,.F.) ;
#36552=ORIENTED_EDGE('',*,*,#25297,.F.) ;
#36553=ORIENTED_EDGE('',*,*,#26573,.F.) ;
#36554=ORIENTED_EDGE('',*,*,#25607,.T.) ;
#36555=ORIENTED_EDGE('',*,*,#26574,.F.) ;
#36556=ORIENTED_EDGE('',*,*,#25293,.F.) ;
#36557=ORIENTED_EDGE('',*,*,#25569,.F.) ;
#36558=ORIENTED_EDGE('',*,*,#26575,.F.) ;
#36559=ORIENTED_EDGE('',*,*,#25602,.F.) ;
#36560=ORIENTED_EDGE('',*,*,#25639,.T.) ;
#36561=ORIENTED_EDGE('',*,*,#25546,.F.) ;
#36562=ORIENTED_EDGE('',*,*,#25609,.F.) ;
#36563=ORIENTED_EDGE('',*,*,#25566,.F.) ;
#36564=ORIENTED_EDGE('',*,*,#26571,.T.) ;
#36565=ORIENTED_EDGE('',*,*,#25603,.F.) ;
#36566=ORIENTED_EDGE('',*,*,#25549,.F.) ;
#36567=ORIENTED_EDGE('',*,*,#26572,.T.) ;
#36568=ORIENTED_EDGE('',*,*,#25605,.T.) ;
#36569=ORIENTED_EDGE('',*,*,#26573,.T.) ;
#36570=ORIENTED_EDGE('',*,*,#25296,.T.) ;
#36571=ORIENTED_EDGE('',*,*,#25608,.F.) ;
#36572=ORIENTED_EDGE('',*,*,#26575,.T.) ;
#36573=ORIENTED_EDGE('',*,*,#25568,.F.) ;
#36574=ORIENTED_EDGE('',*,*,#25606,.F.) ;
#36575=ORIENTED_EDGE('',*,*,#25294,.T.) ;
#36576=ORIENTED_EDGE('',*,*,#26574,.T.) ;
#36577=ORIENTED_EDGE('',*,*,#25587,.T.) ;
#36578=ORIENTED_EDGE('',*,*,#26576,.T.) ;
#36579=ORIENTED_EDGE('',*,*,#26549,.F.) ;
#36580=ORIENTED_EDGE('',*,*,#25562,.T.) ;
#36581=ORIENTED_EDGE('',*,*,#25588,.T.) ;
#36582=ORIENTED_EDGE('',*,*,#25560,.T.) ;
#36583=ORIENTED_EDGE('',*,*,#26552,.F.) ;
#36584=ORIENTED_EDGE('',*,*,#26554,.T.) ;
#36585=ORIENTED_EDGE('',*,*,#25593,.T.) ;
#36586=ORIENTED_EDGE('',*,*,#25540,.T.) ;
#36587=ORIENTED_EDGE('',*,*,#26560,.F.) ;
#36588=ORIENTED_EDGE('',*,*,#26562,.T.) ;
#36589=ORIENTED_EDGE('',*,*,#25592,.T.) ;
#36590=ORIENTED_EDGE('',*,*,#26556,.T.) ;
#36591=ORIENTED_EDGE('',*,*,#26558,.F.) ;
#36592=ORIENTED_EDGE('',*,*,#25542,.T.) ;
#36593=ORIENTED_EDGE('',*,*,#26519,.F.) ;
#36594=ORIENTED_EDGE('',*,*,#26577,.T.) ;
#36595=ORIENTED_EDGE('',*,*,#26576,.F.) ;
#36596=ORIENTED_EDGE('',*,*,#25586,.T.) ;
#36597=ORIENTED_EDGE('',*,*,#26548,.F.) ;
#36598=ORIENTED_EDGE('',*,*,#26550,.F.) ;
#36599=ORIENTED_EDGE('',*,*,#26577,.F.) ;
#45494=TOROIDAL_SURFACE('',#50349,2.1,0.1) ;
#45495=TOROIDAL_SURFACE('',#50358,2.89999999999999,0.1) ;
#45496=TOROIDAL_SURFACE('',#50363,3.09999999999999,0.1) ;
#45497=TOROIDAL_SURFACE('',#50436,0.5,0.1) ;
#45498=TOROIDAL_SURFACE('',#50443,1.9,0.1) ;
#45499=TOROIDAL_SURFACE('',#50449,1.9,0.1) ;
#45500=TOROIDAL_SURFACE('',#50455,2.7,0.1) ;
#45501=TOROIDAL_SURFACE('',#50461,1.9,0.1) ;
#45502=TOROIDAL_SURFACE('',#50467,1.9,0.1) ;
#45503=TOROIDAL_SURFACE('',#50473,0.5,0.1) ;
#45504=TOROIDAL_SURFACE('',#50495,4.,1.) ;
#45505=TOROIDAL_SURFACE('',#50500,2.88,0.12) ;
#45506=TOROIDAL_SURFACE('',#50505,2.12,0.12) ;
#45507=TOROIDAL_SURFACE('',#50511,1.97000000000001,0.12) ;
#45508=TOROIDAL_SURFACE('',#50522,1.97000000000001,0.12) ;
#45509=TOROIDAL_SURFACE('',#50526,1.97,0.12) ;
#45510=TOROIDAL_SURFACE('',#50537,1.97,0.12) ;
#45511=TOROIDAL_SURFACE('',#50541,1.9,0.1) ;
#45512=TOROIDAL_SURFACE('',#50547,2.7,0.1) ;
#45513=TOROIDAL_SURFACE('',#50552,1.9,0.1) ;
#45514=TOROIDAL_SURFACE('',#50579,0.2,0.1) ;
#45515=TOROIDAL_SURFACE('',#50585,0.2,0.1) ;
#45516=TOROIDAL_SURFACE('',#50598,0.2,0.1) ;
#45517=TOROIDAL_SURFACE('',#50606,0.199999999999996,0.0999999999999934) ;
#45518=TOROIDAL_SURFACE('',#50610,0.199999999999996,0.0999999999999979) ;
#45519=TOROIDAL_SURFACE('',#50616,0.2,0.1) ;
#45520=TOROIDAL_SURFACE('',#50623,0.2,0.1) ;
#45521=TOROIDAL_SURFACE('',#50639,0.2,0.1) ;
#45522=TOROIDAL_SURFACE('',#50655,0.2,0.1) ;
#45523=TOROIDAL_SURFACE('',#50664,0.2,0.1) ;
#45524=TOROIDAL_SURFACE('',#50669,0.2,0.1) ;
#45525=TOROIDAL_SURFACE('',#50674,0.2,0.1) ;
#45526=TOROIDAL_SURFACE('',#50697,0.2,0.1) ;
#45527=TOROIDAL_SURFACE('',#50702,0.2,0.1) ;
#45528=TOROIDAL_SURFACE('',#50707,0.2,0.1) ;
#45529=TOROIDAL_SURFACE('',#50712,0.2,0.1) ;
#45530=TOROIDAL_SURFACE('',#50720,0.2,0.1) ;
#45531=TOROIDAL_SURFACE('',#50725,0.2,0.1) ;
#45532=TOROIDAL_SURFACE('',#50746,0.199999999999996,0.0999999999999934) ;
#45533=TOROIDAL_SURFACE('',#50750,0.199999999999996,0.0999999999999979) ;
#45534=TOROIDAL_SURFACE('',#50756,0.2,0.1) ;
#45535=TOROIDAL_SURFACE('',#50761,0.2,0.1) ;
#45536=TOROIDAL_SURFACE('',#50766,0.2,0.1) ;
#45537=TOROIDAL_SURFACE('',#50771,0.2,0.1) ;
#45538=TOROIDAL_SURFACE('',#50788,0.2,0.1) ;
#45539=TOROIDAL_SURFACE('',#50797,0.2,0.1) ;
#45540=TOROIDAL_SURFACE('',#50802,0.2,0.1) ;
#45541=TOROIDAL_SURFACE('',#50812,0.2,0.1) ;
#45542=TOROIDAL_SURFACE('',#50830,0.2,0.1) ;
#45543=TOROIDAL_SURFACE('',#50839,0.2,0.1) ;
#45544=TOROIDAL_SURFACE('',#50844,0.2,0.1) ;
#45545=TOROIDAL_SURFACE('',#50854,0.2,0.1) ;
#45546=TOROIDAL_SURFACE('',#50877,0.2,0.1) ;
#45547=TOROIDAL_SURFACE('',#50883,0.2,0.1) ;
#45548=TOROIDAL_SURFACE('',#50889,0.2,0.1) ;
#45549=TOROIDAL_SURFACE('',#50894,0.2,0.1) ;
#45550=TOROIDAL_SURFACE('',#50899,0.2,0.1) ;
#45551=TOROIDAL_SURFACE('',#50904,0.2,0.1) ;
#45552=TOROIDAL_SURFACE('',#50922,0.2,0.1) ;
#45553=TOROIDAL_SURFACE('',#50927,0.199999999999996,0.0999999999999934) ;
#45554=TOROIDAL_SURFACE('',#50931,0.199999999999996,0.0999999999999979) ;
#45555=TOROIDAL_SURFACE('',#50935,0.200000000000031,0.0999999999999979) ;
#45556=TOROIDAL_SURFACE('',#50942,0.199999999999996,0.0999999999999979) ;
#45557=TOROIDAL_SURFACE('',#50952,0.2,0.1) ;
#45558=TOROIDAL_SURFACE('',#50956,0.2,0.1) ;
#45559=TOROIDAL_SURFACE('',#50961,0.199999999999996,0.0999999999999979) ;
#45560=TOROIDAL_SURFACE('',#50964,0.199999999999996,0.0999999999999979) ;
#45561=TOROIDAL_SURFACE('',#50975,0.200000000000031,0.0999999999999979) ;
#45562=TOROIDAL_SURFACE('',#50979,0.199999999999996,0.0999999999999979) ;
#45563=TOROIDAL_SURFACE('',#50985,0.199999999999996,0.0999999999999979) ;
#45564=TOROIDAL_SURFACE('',#50989,0.200000000000031,0.0999999999999979) ;
#45565=TOROIDAL_SURFACE('',#51004,0.2,0.1) ;
#45566=TOROIDAL_SURFACE('',#51008,0.2,0.1) ;
#45567=TOROIDAL_SURFACE('',#51013,0.200000000000031,0.0999999999999979) ;
#45568=TOROIDAL_SURFACE('',#51020,0.199999999999996,0.0999999999999979) ;
#45569=TOROIDAL_SURFACE('',#51024,0.200000000000031,0.0999999999999979) ;
#45570=TOROIDAL_SURFACE('',#51032,0.199999999999996,0.0999999999999979) ;
#45571=TOROIDAL_SURFACE('',#51036,0.199999999999996,0.0999999999999979) ;
#45572=TOROIDAL_SURFACE('',#51042,0.200000000000031,0.0999999999999979) ;
#45573=TOROIDAL_SURFACE('',#51056,0.199999999999996,0.0999999999999979) ;
#45574=TOROIDAL_SURFACE('',#51060,0.200000000000031,0.0999999999999979) ;
#45575=TOROIDAL_SURFACE('',#51067,1.1,0.1) ;
#45576=TOROIDAL_SURFACE('',#51072,0.5,0.1) ;
#45577=TOROIDAL_SURFACE('',#51077,0.5,0.1) ;
#45578=TOROIDAL_SURFACE('',#51081,1.9,0.1) ;
#45579=TOROIDAL_SURFACE('',#51082,1.9,0.1) ;
#45580=TOROIDAL_SURFACE('',#51086,1.1,0.1) ;
#45581=TOROIDAL_SURFACE('',#51091,0.7,0.1) ;
#45582=TOROIDAL_SURFACE('',#51096,0.5,0.1) ;
#45583=TOROIDAL_SURFACE('',#51101,0.500000000000005,0.1) ;
#45584=TOROIDAL_SURFACE('',#51104,2.59999999999996,0.1) ;
#45585=TOROIDAL_SURFACE('',#51109,2.59999999999999,0.1) ;
#45586=TOROIDAL_SURFACE('',#51112,0.500000000000023,0.1) ;
#45587=TOROIDAL_SURFACE('',#51117,0.5,0.1) ;
#45588=TOROIDAL_SURFACE('',#51122,0.7,0.1) ;
#45589=TOROIDAL_SURFACE('',#51127,3.9,0.1) ;
#45590=TOROIDAL_SURFACE('',#51132,3.9,0.1) ;
#45591=TOROIDAL_SURFACE('',#51137,3.9,0.1) ;
#45592=TOROIDAL_SURFACE('',#51142,0.7,0.1) ;
#45593=TOROIDAL_SURFACE('',#51147,0.5,0.1) ;
#45594=TOROIDAL_SURFACE('',#51151,0.2,0.1) ;
#45595=TOROIDAL_SURFACE('',#51159,0.2,0.1) ;
#45596=TOROIDAL_SURFACE('',#51205,0.9,0.1) ;
#45597=TOROIDAL_SURFACE('',#51218,0.9,0.1) ;
#45598=TOROIDAL_SURFACE('',#51224,0.199999999999996,0.100000000000002) ;
#45599=TOROIDAL_SURFACE('',#51228,0.199999999999995,0.0999999999999784) ;
#45600=TOROIDAL_SURFACE('',#51233,0.199999999999987,0.0999999999999979) ;
#45601=TOROIDAL_SURFACE('',#51238,0.199999999999969,0.0999999999999847) ;
#45602=TOROIDAL_SURFACE('',#51243,0.200000000000031,0.100000000000016) ;
#45603=TOROIDAL_SURFACE('',#51248,0.200000000000031,0.0999999999999979) ;
#45604=TOROIDAL_SURFACE('',#51267,0.199999999999996,0.100000000000002) ;
#45605=TOROIDAL_SURFACE('',#51273,0.199999999999996,0.100000000000002) ;
#45606=TOROIDAL_SURFACE('',#51277,0.200000000000031,0.0999999999999979) ;
#45607=TOROIDAL_SURFACE('',#51281,0.199999999999996,0.0999999999999979) ;
#45608=TOROIDAL_SURFACE('',#51286,0.199999999999996,0.100000000000002) ;
#45609=TOROIDAL_SURFACE('',#51293,0.200000000000031,0.0999999999999979) ;
#45610=TOROIDAL_SURFACE('',#51308,0.9,0.1) ;
#45611=TOROIDAL_SURFACE('',#51317,0.900000000000001,0.1) ;
#45612=TOROIDAL_SURFACE('',#51324,0.199999999999919,0.0999999999999784) ;
#45613=TOROIDAL_SURFACE('',#51328,0.199999999999987,0.0999999999999979) ;
#45614=TOROIDAL_SURFACE('',#51332,0.199999999999982,0.099999999999991) ;
#45615=TOROIDAL_SURFACE('',#51336,0.199999999999996,0.100000000000016) ;
#45616=TOROIDAL_SURFACE('',#51344,0.9,0.1) ;
#45617=TOROIDAL_SURFACE('',#51357,0.9,0.1) ;
#45618=TOROIDAL_SURFACE('',#51363,0.200000000000031,0.100000000000016) ;
#45619=TOROIDAL_SURFACE('',#51367,0.199999999999982,0.099999999999991) ;
#45620=TOROIDAL_SURFACE('',#51371,0.199999999999987,0.0999999999999979) ;
#45621=TOROIDAL_SURFACE('',#51375,0.199999999999976,0.0999999999999847) ;
#45622=TOROIDAL_SURFACE('',#51399,0.200000000000031,0.0999999999999979) ;
#45623=TOROIDAL_SURFACE('',#51403,0.200000000000031,0.100000000000016) ;
#45624=TOROIDAL_SURFACE('',#51407,0.199999999999996,0.0999999999999979) ;
#45625=TOROIDAL_SURFACE('',#51411,0.200000000000031,0.100000000000016) ;
#45626=TOROIDAL_SURFACE('',#51415,0.200000000000031,0.0999999999999934) ;
#45627=TOROIDAL_SURFACE('',#51419,0.199999999999996,0.0999999999999979) ;
#45628=TOROIDAL_SURFACE('',#51423,0.200000000000031,0.0999999999999979) ;
#45629=TOROIDAL_SURFACE('',#51428,0.200000000000031,0.100000000000016) ;
#45630=TOROIDAL_SURFACE('',#51447,2.6,0.1) ;
#45631=TOROIDAL_SURFACE('',#51453,2.6,0.1) ;
#45632=TOROIDAL_SURFACE('',#51458,0.900000000000001,0.1) ;
#45633=TOROIDAL_SURFACE('',#51470,0.9,0.1) ;
#45634=TOROIDAL_SURFACE('',#51477,0.199999999999969,0.099999999999991) ;
#45635=TOROIDAL_SURFACE('',#51482,0.199999999999991,0.0999999999999979) ;
#45636=TOROIDAL_SURFACE('',#51486,0.199999999999969,0.0999999999999847) ;
#45637=TOROIDAL_SURFACE('',#51490,0.200000000000031,0.100000000000016) ;
#45638=TOROIDAL_SURFACE('',#51494,0.199999999999996,0.0999999999999979) ;
#45639=TOROIDAL_SURFACE('',#51500,2.6,0.1) ;
#45640=TOROIDAL_SURFACE('',#51505,2.1,0.1) ;
#45641=TOROIDAL_SURFACE('',#51512,0.7,0.1) ;
#45642=TOROIDAL_SURFACE('',#51517,0.5,0.1) ;
#45643=TOROIDAL_SURFACE('',#51521,0.500000000000005,0.1) ;
#45644=TOROIDAL_SURFACE('',#51523,2.59999999999996,0.1) ;
#45645=TOROIDAL_SURFACE('',#51527,2.59999999999999,0.1) ;
#45646=TOROIDAL_SURFACE('',#51529,0.500000000000023,0.1) ;
#45647=TOROIDAL_SURFACE('',#51533,0.5,0.1) ;
#45648=TOROIDAL_SURFACE('',#51537,0.7,0.1) ;
#45649=TOROIDAL_SURFACE('',#51541,3.9,0.1) ;
#45650=TOROIDAL_SURFACE('',#51545,3.9,0.1) ;
#45651=TOROIDAL_SURFACE('',#51549,3.9,0.1) ;
#45652=TOROIDAL_SURFACE('',#51553,0.7,0.1) ;
#45653=TOROIDAL_SURFACE('',#51557,0.5,0.1) ;
#45654=TOROIDAL_SURFACE('',#51559,0.5,0.1) ;
#45655=TOROIDAL_SURFACE('',#51564,0.5,0.1) ;
#45656=TOROIDAL_SURFACE('',#51568,2.2,0.2) ;
#45657=TOROIDAL_SURFACE('',#51573,2.6,0.2) ;
#45658=TOROIDAL_SURFACE('',#51579,3.,0.2) ;
#45659=TOROIDAL_SURFACE('',#51583,3.,0.2) ;
#45660=TOROIDAL_SURFACE('',#51591,2.6,0.2) ;
#45661=TOROIDAL_SURFACE('',#51596,2.2,0.2) ;
#45662=TOROIDAL_SURFACE('',#51601,2.99999999999999,0.2) ;
#45663=TOROIDAL_SURFACE('',#51609,2.2,0.2) ;
#45664=TOROIDAL_SURFACE('',#51614,2.59999999999999,0.2) ;
#45665=TOROIDAL_SURFACE('',#51616,4.06491106406735,1.3) ;
#45666=TOROIDAL_SURFACE('',#51618,4.06491106406736,1.3) ;
#45667=TOROIDAL_SURFACE('',#51620,4.06491106406735,1.3) ;
#46426=ADVANCED_FACE('',(#11208),#1917,.T.) ;
#46427=ADVANCED_FACE('',(#11209),#1918,.T.) ;
#46428=ADVANCED_FACE('',(#11210),#1919,.T.) ;
#46429=ADVANCED_FACE('',(#11211),#9592,.F.) ;
#46430=ADVANCED_FACE('',(#11212),#9593,.F.) ;
#46431=ADVANCED_FACE('',(#11213),#9594,.F.) ;
#46432=ADVANCED_FACE('',(#11214),#1920,.T.) ;
#46433=ADVANCED_FACE('',(#11215),#1921,.T.) ;
#46434=ADVANCED_FACE('',(#11216),#2277,.F.) ;
#46435=ADVANCED_FACE('',(#11217),#2278,.F.) ;
#46436=ADVANCED_FACE('',(#11218),#2279,.F.) ;
#46437=ADVANCED_FACE('',(#11219),#1922,.F.) ;
#46438=ADVANCED_FACE('',(#11220,#679),#2280,.T.) ;
#46439=ADVANCED_FACE('',(#11221),#9595,.F.) ;
#46440=ADVANCED_FACE('',(#11222),#9596,.F.) ;
#46441=ADVANCED_FACE('',(#11223),#9597,.F.) ;
#46442=ADVANCED_FACE('',(#11224),#1923,.T.) ;
#46443=ADVANCED_FACE('',(#11225),#1924,.T.) ;
#46444=ADVANCED_FACE('',(#11226),#1925,.T.) ;
#46445=ADVANCED_FACE('',(#11227),#1926,.T.) ;
#46446=ADVANCED_FACE('',(#11228),#9598,.F.) ;
#46447=ADVANCED_FACE('',(#11229),#1927,.T.) ;
#46448=ADVANCED_FACE('',(#11230),#9599,.F.) ;
#46449=ADVANCED_FACE('',(#11231),#9600,.F.) ;
#46450=ADVANCED_FACE('',(#11232),#9601,.F.) ;
#46451=ADVANCED_FACE('',(#11233),#9602,.F.) ;
#46452=ADVANCED_FACE('',(#11234),#1928,.T.) ;
#46453=ADVANCED_FACE('',(#11235),#1929,.T.) ;
#46454=ADVANCED_FACE('',(#11236),#1930,.T.) ;
#46455=ADVANCED_FACE('',(#11237),#1931,.T.) ;
#46456=ADVANCED_FACE('',(#11238),#1932,.T.) ;
#46457=ADVANCED_FACE('',(#11239),#1933,.T.) ;
#46458=ADVANCED_FACE('',(#11240),#1934,.F.) ;
#46459=ADVANCED_FACE('',(#11241),#1935,.F.) ;
#46460=ADVANCED_FACE('',(#11242),#2281,.F.) ;
#46461=ADVANCED_FACE('',(#11243),#2282,.F.) ;
#46462=ADVANCED_FACE('',(#11244),#2283,.F.) ;
#46463=ADVANCED_FACE('',(#11245),#1936,.F.) ;
#46464=ADVANCED_FACE('',(#11246),#1937,.F.) ;
#46465=ADVANCED_FACE('',(#11247),#1938,.F.) ;
#46466=ADVANCED_FACE('',(#11248),#1939,.F.) ;
#46467=ADVANCED_FACE('',(#11249),#2284,.F.) ;
#46468=ADVANCED_FACE('',(#11250),#1940,.F.) ;
#46469=ADVANCED_FACE('',(#11251),#9603,.T.) ;
#46470=ADVANCED_FACE('',(#11252),#9604,.T.) ;
#46471=ADVANCED_FACE('',(#11253),#1941,.F.) ;
#46472=ADVANCED_FACE('',(#11254),#9605,.T.) ;
#46473=ADVANCED_FACE('',(#11255),#1942,.F.) ;
#46474=ADVANCED_FACE('',(#11256),#1943,.F.) ;
#46475=ADVANCED_FACE('',(#11257),#1944,.F.) ;
#46476=ADVANCED_FACE('',(#11258),#2285,.T.) ;
#46477=ADVANCED_FACE('',(#11259),#9606,.F.) ;
#46478=ADVANCED_FACE('',(#11260),#9607,.F.) ;
#46479=ADVANCED_FACE('',(#11261),#9608,.F.) ;
#46480=ADVANCED_FACE('',(#11262),#2286,.F.) ;
#46481=ADVANCED_FACE('',(#11263),#2287,.F.) ;
#46482=ADVANCED_FACE('',(#11264),#2288,.F.) ;
#46483=ADVANCED_FACE('',(#11265),#9609,.F.) ;
#46484=ADVANCED_FACE('',(#11266),#9610,.F.) ;
#46485=ADVANCED_FACE('',(#11267),#9611,.F.) ;
#46486=ADVANCED_FACE('',(#11268),#9612,.F.) ;
#46487=ADVANCED_FACE('',(#11269),#2289,.F.) ;
#46488=ADVANCED_FACE('',(#11270),#2290,.F.) ;
#46489=ADVANCED_FACE('',(#11271),#2291,.F.) ;
#46490=ADVANCED_FACE('',(#11272),#9613,.F.) ;
#46491=ADVANCED_FACE('',(#11273),#9614,.F.) ;
#46492=ADVANCED_FACE('',(#11274),#9615,.F.) ;
#46493=ADVANCED_FACE('',(#11275),#2292,.F.) ;
#46494=ADVANCED_FACE('',(#11276),#2293,.F.) ;
#46495=ADVANCED_FACE('',(#11277),#2294,.F.) ;
#46496=ADVANCED_FACE('',(#11278),#9616,.T.) ;
#46497=ADVANCED_FACE('',(#11279),#1945,.F.) ;
#46498=ADVANCED_FACE('',(#11280),#1946,.F.) ;
#46499=ADVANCED_FACE('',(#11281),#9617,.T.) ;
#46500=ADVANCED_FACE('',(#11282),#1947,.F.) ;
#46501=ADVANCED_FACE('',(#11283),#1948,.F.) ;
#46502=ADVANCED_FACE('',(#11284),#1949,.F.) ;
#46503=ADVANCED_FACE('',(#11285),#1950,.F.) ;
#46504=ADVANCED_FACE('',(#11286),#1951,.F.) ;
#46505=ADVANCED_FACE('',(#11287),#9618,.T.) ;
#46506=ADVANCED_FACE('',(#11288),#9619,.T.) ;
#46507=ADVANCED_FACE('',(#11289),#9620,.T.) ;
#46508=ADVANCED_FACE('',(#11290),#9621,.T.) ;
#46509=ADVANCED_FACE('',(#11291),#1952,.F.) ;
#46510=ADVANCED_FACE('',(#11292),#9622,.T.) ;
#46511=ADVANCED_FACE('',(#11293),#1953,.F.) ;
#46512=ADVANCED_FACE('',(#11294),#1954,.F.) ;
#46513=ADVANCED_FACE('',(#11295),#1955,.F.) ;
#46514=ADVANCED_FACE('',(#11296),#9623,.T.) ;
#46515=ADVANCED_FACE('',(#11297),#1956,.F.) ;
#46516=ADVANCED_FACE('',(#11298),#1957,.F.) ;
#46517=ADVANCED_FACE('',(#11299),#1958,.F.) ;
#46518=ADVANCED_FACE('',(#11300),#1959,.F.) ;
#46519=ADVANCED_FACE('',(#11301),#2295,.F.) ;
#46520=ADVANCED_FACE('',(#11302),#2296,.F.) ;
#46521=ADVANCED_FACE('',(#11303),#2297,.F.) ;
#46522=ADVANCED_FACE('',(#11304),#2298,.F.) ;
#46523=ADVANCED_FACE('',(#11305,#680,#681,#682,#683,#684,#685,#686,#687,
#688,#689,#690,#691,#692,#693,#694,#695,#696,#697),#2299,.T.) ;
#46524=ADVANCED_FACE('',(#11306),#9624,.T.) ;
#46525=ADVANCED_FACE('',(#11307),#9625,.T.) ;
#46526=ADVANCED_FACE('',(#11308),#9626,.T.) ;
#46527=ADVANCED_FACE('',(#11309),#2300,.F.) ;
#46528=ADVANCED_FACE('',(#11310),#9627,.T.) ;
#46529=ADVANCED_FACE('',(#11311),#9628,.T.) ;
#46530=ADVANCED_FACE('',(#11312),#9629,.T.) ;
#46531=ADVANCED_FACE('',(#11313),#9630,.T.) ;
#46532=ADVANCED_FACE('',(#11314),#2301,.F.) ;
#46533=ADVANCED_FACE('',(#11315),#9631,.T.) ;
#46534=ADVANCED_FACE('',(#11316),#9632,.T.) ;
#46535=ADVANCED_FACE('',(#11317),#9633,.T.) ;
#46536=ADVANCED_FACE('',(#11318),#2302,.F.) ;
#46537=ADVANCED_FACE('',(#11319),#2303,.F.) ;
#46538=ADVANCED_FACE('',(#11320),#1960,.F.) ;
#46539=ADVANCED_FACE('',(#11321),#1961,.F.) ;
#46540=ADVANCED_FACE('',(#11322),#1962,.F.) ;
#46541=ADVANCED_FACE('',(#11323),#1963,.F.) ;
#46542=ADVANCED_FACE('',(#11324),#1964,.F.) ;
#46543=ADVANCED_FACE('',(#11325),#45494,.T.) ;
#46544=ADVANCED_FACE('',(#11326,#698),#2304,.F.) ;
#46545=ADVANCED_FACE('',(#11327),#9634,.F.) ;
#46546=ADVANCED_FACE('',(#11328),#45495,.T.) ;
#46547=ADVANCED_FACE('',(#11329),#9635,.T.) ;
#46548=ADVANCED_FACE('',(#11330),#45496,.F.) ;
#46549=ADVANCED_FACE('',(#11331,#699,#700,#701,#702,#703,#704,#705,#706,
#707,#708,#709,#710,#711,#712),#2305,.F.) ;
#46550=ADVANCED_FACE('',(#11332),#45497,.T.) ;
#46551=ADVANCED_FACE('',(#11333),#9636,.T.) ;
#46552=ADVANCED_FACE('',(#11334),#45498,.T.) ;
#46553=ADVANCED_FACE('',(#11335),#9637,.T.) ;
#46554=ADVANCED_FACE('',(#11336),#45499,.T.) ;
#46555=ADVANCED_FACE('',(#11337),#9638,.T.) ;
#46556=ADVANCED_FACE('',(#11338),#45500,.T.) ;
#46557=ADVANCED_FACE('',(#11339),#9639,.T.) ;
#46558=ADVANCED_FACE('',(#11340),#45501,.T.) ;
#46559=ADVANCED_FACE('',(#11341),#9640,.T.) ;
#46560=ADVANCED_FACE('',(#11342),#45502,.T.) ;
#46561=ADVANCED_FACE('',(#11343),#9641,.T.) ;
#46562=ADVANCED_FACE('',(#11344),#45503,.T.) ;
#46563=ADVANCED_FACE('',(#11345),#2306,.T.) ;
#46564=ADVANCED_FACE('',(#11346),#9642,.T.) ;
#46565=ADVANCED_FACE('',(#11347),#2307,.F.) ;
#46566=ADVANCED_FACE('',(#11348),#9643,.T.) ;
#46567=ADVANCED_FACE('',(#11349),#2308,.F.) ;
#46568=ADVANCED_FACE('',(#11350),#9644,.F.) ;
#46569=ADVANCED_FACE('',(#11351),#2309,.F.) ;
#46570=ADVANCED_FACE('',(#11352),#9645,.T.) ;
#46571=ADVANCED_FACE('',(#11353),#2310,.F.) ;
#46572=ADVANCED_FACE('',(#11354),#9646,.T.) ;
#46573=ADVANCED_FACE('',(#11355),#2311,.T.) ;
#46574=ADVANCED_FACE('',(#11356),#45504,.F.) ;
#46575=ADVANCED_FACE('',(#11357),#9647,.T.) ;
#46576=ADVANCED_FACE('',(#11358),#1965,.T.) ;
#46577=ADVANCED_FACE('',(#11359),#45505,.T.) ;
#46578=ADVANCED_FACE('',(#11360,#713),#2312,.F.) ;
#46579=ADVANCED_FACE('',(#11361),#45506,.T.) ;
#46580=ADVANCED_FACE('',(#11362),#9648,.F.) ;
#46581=ADVANCED_FACE('',(#11363),#45507,.T.) ;
#46582=ADVANCED_FACE('',(#11364),#9649,.F.) ;
#46583=ADVANCED_FACE('',(#11365,#714),#2313,.T.) ;
#46584=ADVANCED_FACE('',(#11366),#45508,.T.) ;
#46585=ADVANCED_FACE('',(#11367,#715),#2314,.F.) ;
#46586=ADVANCED_FACE('',(#11368),#45509,.T.) ;
#46587=ADVANCED_FACE('',(#11369),#9650,.F.) ;
#46588=ADVANCED_FACE('',(#11370,#716),#2315,.T.) ;
#46589=ADVANCED_FACE('',(#11371),#45510,.T.) ;
#46590=ADVANCED_FACE('',(#11372,#717),#2316,.F.) ;
#46591=ADVANCED_FACE('',(#11373),#45511,.T.) ;
#46592=ADVANCED_FACE('',(#11374),#9651,.T.) ;
#46593=ADVANCED_FACE('',(#11375),#45512,.T.) ;
#46594=ADVANCED_FACE('',(#11376),#9652,.T.) ;
#46595=ADVANCED_FACE('',(#11377),#45513,.T.) ;
#46596=ADVANCED_FACE('',(#11378),#2317,.T.) ;
#46597=ADVANCED_FACE('',(#11379),#9653,.T.) ;
#46598=ADVANCED_FACE('',(#11380),#2318,.F.) ;
#46599=ADVANCED_FACE('',(#11381),#9654,.T.) ;
#46600=ADVANCED_FACE('',(#11382),#9655,.F.) ;
#46601=ADVANCED_FACE('',(#11383),#1966,.T.) ;
#46602=ADVANCED_FACE('',(#11384),#1967,.T.) ;
#46603=ADVANCED_FACE('',(#11385),#9656,.F.) ;
#46604=ADVANCED_FACE('',(#11386),#1968,.T.) ;
#46605=ADVANCED_FACE('',(#11387),#9657,.F.) ;
#46606=ADVANCED_FACE('',(#11388),#9658,.T.) ;
#46607=ADVANCED_FACE('',(#11389),#45514,.T.) ;
#46608=ADVANCED_FACE('',(#11390),#9659,.T.) ;
#46609=ADVANCED_FACE('',(#11391),#45515,.T.) ;
#46610=ADVANCED_FACE('',(#11392),#9660,.T.) ;
#46611=ADVANCED_FACE('',(#11393),#9661,.F.) ;
#46612=ADVANCED_FACE('',(#11394),#9662,.T.) ;
#46613=ADVANCED_FACE('',(#11395),#2176,.T.) ;
#46614=ADVANCED_FACE('',(#11396),#9663,.T.) ;
#46615=ADVANCED_FACE('',(#11397),#45516,.T.) ;
#46616=ADVANCED_FACE('',(#11398),#2177,.T.) ;
#46617=ADVANCED_FACE('',(#11399),#9664,.T.) ;
#46618=ADVANCED_FACE('',(#11400),#45517,.T.) ;
#46619=ADVANCED_FACE('',(#11401),#45518,.T.) ;
#46620=ADVANCED_FACE('',(#11402),#9665,.T.) ;
#46621=ADVANCED_FACE('',(#11403),#9666,.T.) ;
#46622=ADVANCED_FACE('',(#11404),#45519,.F.) ;
#46623=ADVANCED_FACE('',(#11405),#9667,.F.) ;
#46624=ADVANCED_FACE('',(#11406),#9668,.F.) ;
#46625=ADVANCED_FACE('',(#11407),#45520,.F.) ;
#46626=ADVANCED_FACE('',(#11408),#9669,.T.) ;
#46627=ADVANCED_FACE('',(#11409),#2178,.T.) ;
#46628=ADVANCED_FACE('',(#11410),#9670,.T.) ;
#46629=ADVANCED_FACE('',(#11411),#2319,.F.) ;
#46630=ADVANCED_FACE('',(#11412),#9671,.T.) ;
#46631=ADVANCED_FACE('',(#11413),#9672,.T.) ;
#46632=ADVANCED_FACE('',(#11414),#2320,.F.) ;
#46633=ADVANCED_FACE('',(#11415),#45521,.F.) ;
#46634=ADVANCED_FACE('',(#11416),#9673,.F.) ;
#46635=ADVANCED_FACE('',(#11417),#1969,.T.) ;
#46636=ADVANCED_FACE('',(#11418),#9674,.T.) ;
#46637=ADVANCED_FACE('',(#11419),#2321,.F.) ;
#46638=ADVANCED_FACE('',(#11420),#1970,.T.) ;
#46639=ADVANCED_FACE('',(#11421),#9675,.F.) ;
#46640=ADVANCED_FACE('',(#11422),#45522,.F.) ;
#46641=ADVANCED_FACE('',(#11423),#2322,.F.) ;
#46642=ADVANCED_FACE('',(#11424),#9676,.T.) ;
#46643=ADVANCED_FACE('',(#11425),#9677,.T.) ;
#46644=ADVANCED_FACE('',(#11426),#45523,.T.) ;
#46645=ADVANCED_FACE('',(#11427),#9678,.T.) ;
#46646=ADVANCED_FACE('',(#11428),#45524,.T.) ;
#46647=ADVANCED_FACE('',(#11429),#9679,.T.) ;
#46648=ADVANCED_FACE('',(#11430),#45525,.T.) ;
#46649=ADVANCED_FACE('',(#11431),#9680,.T.) ;
#46650=ADVANCED_FACE('',(#11432),#2323,.F.) ;
#46651=ADVANCED_FACE('',(#11433),#9681,.F.) ;
#46652=ADVANCED_FACE('',(#11434),#2324,.F.) ;
#46653=ADVANCED_FACE('',(#11435),#9682,.F.) ;
#46654=ADVANCED_FACE('',(#11436),#2325,.T.) ;
#46655=ADVANCED_FACE('',(#11437),#9683,.F.) ;
#46656=ADVANCED_FACE('',(#11438),#2326,.F.) ;
#46657=ADVANCED_FACE('',(#11439),#9684,.F.) ;
#46658=ADVANCED_FACE('',(#11440),#2327,.T.) ;
#46659=ADVANCED_FACE('',(#11441),#9685,.F.) ;
#46660=ADVANCED_FACE('',(#11442),#2328,.F.) ;
#46661=ADVANCED_FACE('',(#11443),#9686,.T.) ;
#46662=ADVANCED_FACE('',(#11444),#45526,.T.) ;
#46663=ADVANCED_FACE('',(#11445),#9687,.T.) ;
#46664=ADVANCED_FACE('',(#11446),#45527,.T.) ;
#46665=ADVANCED_FACE('',(#11447),#9688,.T.) ;
#46666=ADVANCED_FACE('',(#11448),#45528,.T.) ;
#46667=ADVANCED_FACE('',(#11449),#9689,.T.) ;
#46668=ADVANCED_FACE('',(#11450),#45529,.T.) ;
#46669=ADVANCED_FACE('',(#11451),#9690,.T.) ;
#46670=ADVANCED_FACE('',(#11452),#9691,.T.) ;
#46671=ADVANCED_FACE('',(#11453),#45530,.T.) ;
#46672=ADVANCED_FACE('',(#11454),#9692,.T.) ;
#46673=ADVANCED_FACE('',(#11455),#45531,.T.) ;
#46674=ADVANCED_FACE('',(#11456),#9693,.T.) ;
#46675=ADVANCED_FACE('',(#11457),#2179,.T.) ;
#46676=ADVANCED_FACE('',(#11458),#2180,.T.) ;
#46677=ADVANCED_FACE('',(#11459),#9694,.F.) ;
#46678=ADVANCED_FACE('',(#11460),#2329,.F.) ;
#46679=ADVANCED_FACE('',(#11461),#9695,.F.) ;
#46680=ADVANCED_FACE('',(#11462),#2330,.F.) ;
#46681=ADVANCED_FACE('',(#11463),#9696,.F.) ;
#46682=ADVANCED_FACE('',(#11464),#2331,.F.) ;
#46683=ADVANCED_FACE('',(#11465),#9697,.T.) ;
#46684=ADVANCED_FACE('',(#11466),#2332,.F.) ;
#46685=ADVANCED_FACE('',(#11467),#45532,.T.) ;
#46686=ADVANCED_FACE('',(#11468),#45533,.T.) ;
#46687=ADVANCED_FACE('',(#11469),#9698,.T.) ;
#46688=ADVANCED_FACE('',(#11470),#45534,.T.) ;
#46689=ADVANCED_FACE('',(#11471),#9699,.T.) ;
#46690=ADVANCED_FACE('',(#11472),#45535,.T.) ;
#46691=ADVANCED_FACE('',(#11473),#9700,.T.) ;
#46692=ADVANCED_FACE('',(#11474),#45536,.T.) ;
#46693=ADVANCED_FACE('',(#11475),#9701,.T.) ;
#46694=ADVANCED_FACE('',(#11476),#45537,.T.) ;
#46695=ADVANCED_FACE('',(#11477),#9702,.T.) ;
#46696=ADVANCED_FACE('',(#11478),#9703,.T.) ;
#46697=ADVANCED_FACE('',(#11479),#9704,.F.) ;
#46698=ADVANCED_FACE('',(#11480),#1971,.T.) ;
#46699=ADVANCED_FACE('',(#11481),#9705,.F.) ;
#46700=ADVANCED_FACE('',(#11482),#1972,.T.) ;
#46701=ADVANCED_FACE('',(#11483),#9706,.T.) ;
#46702=ADVANCED_FACE('',(#11484),#2333,.F.) ;
#46703=ADVANCED_FACE('',(#11485),#45538,.T.) ;
#46704=ADVANCED_FACE('',(#11486),#9707,.T.) ;
#46705=ADVANCED_FACE('',(#11487),#9708,.T.) ;
#46706=ADVANCED_FACE('',(#11488),#45539,.T.) ;
#46707=ADVANCED_FACE('',(#11489),#9709,.T.) ;
#46708=ADVANCED_FACE('',(#11490),#45540,.T.) ;
#46709=ADVANCED_FACE('',(#11491),#9710,.T.) ;
#46710=ADVANCED_FACE('',(#11492),#2181,.T.) ;
#46711=ADVANCED_FACE('',(#11493),#9711,.T.) ;
#46712=ADVANCED_FACE('',(#11494),#45541,.T.) ;
#46713=ADVANCED_FACE('',(#11495),#2182,.T.) ;
#46714=ADVANCED_FACE('',(#11496),#2334,.F.) ;
#46715=ADVANCED_FACE('',(#11497),#9712,.T.) ;
#46716=ADVANCED_FACE('',(#11498),#2335,.F.) ;
#46717=ADVANCED_FACE('',(#11499),#9713,.F.) ;
#46718=ADVANCED_FACE('',(#11500),#2336,.F.) ;
#46719=ADVANCED_FACE('',(#11501),#9714,.F.) ;
#46720=ADVANCED_FACE('',(#11502),#2337,.F.) ;
#46721=ADVANCED_FACE('',(#11503),#9715,.T.) ;
#46722=ADVANCED_FACE('',(#11504),#2338,.F.) ;
#46723=ADVANCED_FACE('',(#11505),#45542,.T.) ;
#46724=ADVANCED_FACE('',(#11506),#9716,.T.) ;
#46725=ADVANCED_FACE('',(#11507),#9717,.T.) ;
#46726=ADVANCED_FACE('',(#11508),#45543,.T.) ;
#46727=ADVANCED_FACE('',(#11509),#9718,.T.) ;
#46728=ADVANCED_FACE('',(#11510),#45544,.T.) ;
#46729=ADVANCED_FACE('',(#11511),#9719,.T.) ;
#46730=ADVANCED_FACE('',(#11512),#2183,.T.) ;
#46731=ADVANCED_FACE('',(#11513),#9720,.T.) ;
#46732=ADVANCED_FACE('',(#11514),#45545,.T.) ;
#46733=ADVANCED_FACE('',(#11515),#2184,.T.) ;
#46734=ADVANCED_FACE('',(#11516),#2339,.F.) ;
#46735=ADVANCED_FACE('',(#11517),#9721,.T.) ;
#46736=ADVANCED_FACE('',(#11518),#2340,.F.) ;
#46737=ADVANCED_FACE('',(#11519),#9722,.F.) ;
#46738=ADVANCED_FACE('',(#11520),#2341,.F.) ;
#46739=ADVANCED_FACE('',(#11521),#9723,.F.) ;
#46740=ADVANCED_FACE('',(#11522),#2342,.F.) ;
#46741=ADVANCED_FACE('',(#11523),#9724,.T.) ;
#46742=ADVANCED_FACE('',(#11524),#2343,.F.) ;
#46743=ADVANCED_FACE('',(#11525),#9725,.T.) ;
#46744=ADVANCED_FACE('',(#11526),#9726,.T.) ;
#46745=ADVANCED_FACE('',(#11527),#45546,.T.) ;
#46746=ADVANCED_FACE('',(#11528),#2185,.T.) ;
#46747=ADVANCED_FACE('',(#11529),#2344,.F.) ;
#46748=ADVANCED_FACE('',(#11530),#9727,.T.) ;
#46749=ADVANCED_FACE('',(#11531),#45547,.T.) ;
#46750=ADVANCED_FACE('',(#11532),#2345,.F.) ;
#46751=ADVANCED_FACE('',(#11533),#9728,.T.) ;
#46752=ADVANCED_FACE('',(#11534),#45548,.T.) ;
#46753=ADVANCED_FACE('',(#11535),#9729,.T.) ;
#46754=ADVANCED_FACE('',(#11536),#45549,.T.) ;
#46755=ADVANCED_FACE('',(#11537),#9730,.T.) ;
#46756=ADVANCED_FACE('',(#11538),#45550,.T.) ;
#46757=ADVANCED_FACE('',(#11539),#9731,.T.) ;
#46758=ADVANCED_FACE('',(#11540),#45551,.T.) ;
#46759=ADVANCED_FACE('',(#11541),#9732,.T.) ;
#46760=ADVANCED_FACE('',(#11542),#2346,.F.) ;
#46761=ADVANCED_FACE('',(#11543),#9733,.F.) ;
#46762=ADVANCED_FACE('',(#11544),#2347,.T.) ;
#46763=ADVANCED_FACE('',(#11545),#9734,.F.) ;
#46764=ADVANCED_FACE('',(#11546),#2348,.F.) ;
#46765=ADVANCED_FACE('',(#11547),#9735,.F.) ;
#46766=ADVANCED_FACE('',(#11548),#2349,.T.) ;
#46767=ADVANCED_FACE('',(#11549),#9736,.F.) ;
#46768=ADVANCED_FACE('',(#11550),#2350,.F.) ;
#46769=ADVANCED_FACE('',(#11551),#9737,.F.) ;
#46770=ADVANCED_FACE('',(#11552),#45552,.T.) ;
#46771=ADVANCED_FACE('',(#11553),#2351,.F.) ;
#46772=ADVANCED_FACE('',(#11554),#45553,.T.) ;
#46773=ADVANCED_FACE('',(#11555),#9738,.F.) ;
#46774=ADVANCED_FACE('',(#11556),#45554,.T.) ;
#46775=ADVANCED_FACE('',(#11557),#45555,.T.) ;
#46776=ADVANCED_FACE('',(#11558),#9739,.T.) ;
#46777=ADVANCED_FACE('',(#11559),#9740,.F.) ;
#46778=ADVANCED_FACE('',(#11560),#9741,.T.) ;
#46779=ADVANCED_FACE('',(#11561),#45556,.T.) ;
#46780=ADVANCED_FACE('',(#11562),#9742,.T.) ;
#46781=ADVANCED_FACE('',(#11563),#9743,.T.) ;
#46782=ADVANCED_FACE('',(#11564),#9744,.F.) ;
#46783=ADVANCED_FACE('',(#11565),#9745,.T.) ;
#46784=ADVANCED_FACE('',(#11566),#2352,.F.) ;
#46785=ADVANCED_FACE('',(#11567),#9746,.T.) ;
#46786=ADVANCED_FACE('',(#11568),#45557,.T.) ;
#46787=ADVANCED_FACE('',(#11569),#45558,.T.) ;
#46788=ADVANCED_FACE('',(#11570),#2353,.F.) ;
#46789=ADVANCED_FACE('',(#11571),#45559,.T.) ;
#46790=ADVANCED_FACE('',(#11572),#45560,.T.) ;
#46791=ADVANCED_FACE('',(#11573),#9747,.T.) ;
#46792=ADVANCED_FACE('',(#11574),#2186,.T.) ;
#46793=ADVANCED_FACE('',(#11575),#2187,.T.) ;
#46794=ADVANCED_FACE('',(#11576),#9748,.T.) ;
#46795=ADVANCED_FACE('',(#11577),#45561,.T.) ;
#46796=ADVANCED_FACE('',(#11578),#45562,.T.) ;
#46797=ADVANCED_FACE('',(#11579),#9749,.T.) ;
#46798=ADVANCED_FACE('',(#11580),#9750,.F.) ;
#46799=ADVANCED_FACE('',(#11581),#45563,.T.) ;
#46800=ADVANCED_FACE('',(#11582),#45564,.T.) ;
#46801=ADVANCED_FACE('',(#11583),#9751,.T.) ;
#46802=ADVANCED_FACE('',(#11584),#9752,.F.) ;
#46803=ADVANCED_FACE('',(#11585),#9753,.T.) ;
#46804=ADVANCED_FACE('',(#11586),#9754,.F.) ;
#46805=ADVANCED_FACE('',(#11587),#9755,.T.) ;
#46806=ADVANCED_FACE('',(#11588),#9756,.F.) ;
#46807=ADVANCED_FACE('',(#11589),#9757,.T.) ;
#46808=ADVANCED_FACE('',(#11590),#9758,.T.) ;
#46809=ADVANCED_FACE('',(#11591),#9759,.T.) ;
#46810=ADVANCED_FACE('',(#11592),#2354,.F.) ;
#46811=ADVANCED_FACE('',(#11593),#9760,.T.) ;
#46812=ADVANCED_FACE('',(#11594),#45565,.T.) ;
#46813=ADVANCED_FACE('',(#11595),#45566,.T.) ;
#46814=ADVANCED_FACE('',(#11596),#2355,.F.) ;
#46815=ADVANCED_FACE('',(#11597),#45567,.T.) ;
#46816=ADVANCED_FACE('',(#11598),#2188,.T.) ;
#46817=ADVANCED_FACE('',(#11599),#9761,.T.) ;
#46818=ADVANCED_FACE('',(#11600),#45568,.T.) ;
#46819=ADVANCED_FACE('',(#11601),#9762,.T.) ;
#46820=ADVANCED_FACE('',(#11602),#45569,.T.) ;
#46821=ADVANCED_FACE('',(#11603),#2189,.T.) ;
#46822=ADVANCED_FACE('',(#11604),#9763,.T.) ;
#46823=ADVANCED_FACE('',(#11605),#45570,.T.) ;
#46824=ADVANCED_FACE('',(#11606),#45571,.T.) ;
#46825=ADVANCED_FACE('',(#11607),#9764,.T.) ;
#46826=ADVANCED_FACE('',(#11608),#9765,.F.) ;
#46827=ADVANCED_FACE('',(#11609),#45572,.T.) ;
#46828=ADVANCED_FACE('',(#11610),#9766,.T.) ;
#46829=ADVANCED_FACE('',(#11611),#9767,.F.) ;
#46830=ADVANCED_FACE('',(#11612),#9768,.T.) ;
#46831=ADVANCED_FACE('',(#11613),#9769,.F.) ;
#46832=ADVANCED_FACE('',(#11614),#9770,.T.) ;
#46833=ADVANCED_FACE('',(#11615),#9771,.F.) ;
#46834=ADVANCED_FACE('',(#11616),#9772,.T.) ;
#46835=ADVANCED_FACE('',(#11617),#9773,.T.) ;
#46836=ADVANCED_FACE('',(#11618),#2356,.F.) ;
#46837=ADVANCED_FACE('',(#11619),#9774,.T.) ;
#46838=ADVANCED_FACE('',(#11620),#45573,.T.) ;
#46839=ADVANCED_FACE('',(#11621),#45574,.T.) ;
#46840=ADVANCED_FACE('',(#11622),#9775,.T.) ;
#46841=ADVANCED_FACE('',(#11623),#45575,.T.) ;
#46842=ADVANCED_FACE('',(#11624),#9776,.T.) ;
#46843=ADVANCED_FACE('',(#11625),#45576,.T.) ;
#46844=ADVANCED_FACE('',(#11626),#9777,.T.) ;
#46845=ADVANCED_FACE('',(#11627),#45577,.T.) ;
#46846=ADVANCED_FACE('',(#11628),#9778,.T.) ;
#46847=ADVANCED_FACE('',(#11629),#45578,.T.) ;
#46848=ADVANCED_FACE('',(#11630),#45579,.T.) ;
#46849=ADVANCED_FACE('',(#11631),#9779,.T.) ;
#46850=ADVANCED_FACE('',(#11632),#45580,.T.) ;
#46851=ADVANCED_FACE('',(#11633),#9780,.T.) ;
#46852=ADVANCED_FACE('',(#11634),#45581,.T.) ;
#46853=ADVANCED_FACE('',(#11635),#9781,.T.) ;
#46854=ADVANCED_FACE('',(#11636),#45582,.T.) ;
#46855=ADVANCED_FACE('',(#11637),#9782,.T.) ;
#46856=ADVANCED_FACE('',(#11638),#45583,.T.) ;
#46857=ADVANCED_FACE('',(#11639),#45584,.T.) ;
#46858=ADVANCED_FACE('',(#11640),#9783,.T.) ;
#46859=ADVANCED_FACE('',(#11641),#45585,.T.) ;
#46860=ADVANCED_FACE('',(#11642),#45586,.T.) ;
#46861=ADVANCED_FACE('',(#11643),#9784,.T.) ;
#46862=ADVANCED_FACE('',(#11644),#45587,.T.) ;
#46863=ADVANCED_FACE('',(#11645),#9785,.T.) ;
#46864=ADVANCED_FACE('',(#11646),#45588,.T.) ;
#46865=ADVANCED_FACE('',(#11647),#9786,.T.) ;
#46866=ADVANCED_FACE('',(#11648),#45589,.T.) ;
#46867=ADVANCED_FACE('',(#11649),#9787,.T.) ;
#46868=ADVANCED_FACE('',(#11650),#45590,.T.) ;
#46869=ADVANCED_FACE('',(#11651),#9788,.T.) ;
#46870=ADVANCED_FACE('',(#11652),#45591,.T.) ;
#46871=ADVANCED_FACE('',(#11653),#9789,.T.) ;
#46872=ADVANCED_FACE('',(#11654),#45592,.T.) ;
#46873=ADVANCED_FACE('',(#11655),#9790,.T.) ;
#46874=ADVANCED_FACE('',(#11656),#45593,.T.) ;
#46875=ADVANCED_FACE('',(#11657),#9791,.T.) ;
#46876=ADVANCED_FACE('',(#11658),#45594,.F.) ;
#46877=ADVANCED_FACE('',(#11659),#9792,.F.) ;
#46878=ADVANCED_FACE('',(#11660),#9793,.T.) ;
#46879=ADVANCED_FACE('',(#11661),#9794,.F.) ;
#46880=ADVANCED_FACE('',(#11662),#45595,.F.) ;
#46881=ADVANCED_FACE('',(#11663),#9795,.T.) ;
#46882=ADVANCED_FACE('',(#11664),#2357,.T.) ;
#46883=ADVANCED_FACE('',(#11665),#9796,.T.) ;
#46884=ADVANCED_FACE('',(#11666),#2358,.T.) ;
#46885=ADVANCED_FACE('',(#11667),#9797,.T.) ;
#46886=ADVANCED_FACE('',(#11668),#9798,.F.) ;
#46887=ADVANCED_FACE('',(#11669),#2359,.T.) ;
#46888=ADVANCED_FACE('',(#11670),#9799,.F.) ;
#46889=ADVANCED_FACE('',(#11671),#9800,.T.) ;
#46890=ADVANCED_FACE('',(#11672),#2360,.T.) ;
#46891=ADVANCED_FACE('',(#11673),#9801,.T.) ;
#46892=ADVANCED_FACE('',(#11674),#2361,.T.) ;
#46893=ADVANCED_FACE('',(#11675),#9802,.F.) ;
#46894=ADVANCED_FACE('',(#11676),#2362,.T.) ;
#46895=ADVANCED_FACE('',(#11677),#9803,.T.) ;
#46896=ADVANCED_FACE('',(#11678),#2363,.T.) ;
#46897=ADVANCED_FACE('',(#11679),#9804,.T.) ;
#46898=ADVANCED_FACE('',(#11680),#2364,.T.) ;
#46899=ADVANCED_FACE('',(#11681),#9805,.T.) ;
#46900=ADVANCED_FACE('',(#11682),#2365,.T.) ;
#46901=ADVANCED_FACE('',(#11683),#9806,.F.) ;
#46902=ADVANCED_FACE('',(#11684),#2366,.T.) ;
#46903=ADVANCED_FACE('',(#11685),#9807,.T.) ;
#46904=ADVANCED_FACE('',(#11686),#2367,.F.) ;
#46905=ADVANCED_FACE('',(#11687),#9808,.T.) ;
#46906=ADVANCED_FACE('',(#11688),#9809,.T.) ;
#46907=ADVANCED_FACE('',(#11689),#45596,.T.) ;
#46908=ADVANCED_FACE('',(#11690),#9810,.T.) ;
#46909=ADVANCED_FACE('',(#11691),#9811,.T.) ;
#46910=ADVANCED_FACE('',(#11692),#2368,.T.) ;
#46911=ADVANCED_FACE('',(#11693),#2369,.F.) ;
#46912=ADVANCED_FACE('',(#11694),#9812,.T.) ;
#46913=ADVANCED_FACE('',(#11695),#45597,.T.) ;
#46914=ADVANCED_FACE('',(#11696),#9813,.T.) ;
#46915=ADVANCED_FACE('',(#11697),#2370,.T.) ;
#46916=ADVANCED_FACE('',(#11698),#45598,.T.) ;
#46917=ADVANCED_FACE('',(#11699),#45599,.T.) ;
#46918=ADVANCED_FACE('',(#11700),#9814,.T.) ;
#46919=ADVANCED_FACE('',(#11701),#45600,.T.) ;
#46920=ADVANCED_FACE('',(#11702),#9815,.T.) ;
#46921=ADVANCED_FACE('',(#11703),#45601,.T.) ;
#46922=ADVANCED_FACE('',(#11704),#9816,.T.) ;
#46923=ADVANCED_FACE('',(#11705),#45602,.T.) ;
#46924=ADVANCED_FACE('',(#11706),#9817,.T.) ;
#46925=ADVANCED_FACE('',(#11707),#45603,.T.) ;
#46926=ADVANCED_FACE('',(#11708),#9818,.T.) ;
#46927=ADVANCED_FACE('',(#11709),#9819,.F.) ;
#46928=ADVANCED_FACE('',(#11710),#9820,.T.) ;
#46929=ADVANCED_FACE('',(#11711),#9821,.F.) ;
#46930=ADVANCED_FACE('',(#11712),#9822,.F.) ;
#46931=ADVANCED_FACE('',(#11713),#9823,.F.) ;
#46932=ADVANCED_FACE('',(#11714),#9824,.F.) ;
#46933=ADVANCED_FACE('',(#11715),#9825,.F.) ;
#46934=ADVANCED_FACE('',(#11716),#9826,.T.) ;
#46935=ADVANCED_FACE('',(#11717),#2371,.F.) ;
#46936=ADVANCED_FACE('',(#11718),#2372,.F.) ;
#46937=ADVANCED_FACE('',(#11719),#2190,.T.) ;
#46938=ADVANCED_FACE('',(#11720),#45604,.T.) ;
#46939=ADVANCED_FACE('',(#11721),#9827,.T.) ;
#46940=ADVANCED_FACE('',(#11722),#9828,.F.) ;
#46941=ADVANCED_FACE('',(#11723),#45605,.T.) ;
#46942=ADVANCED_FACE('',(#11724),#45606,.T.) ;
#46943=ADVANCED_FACE('',(#11725),#9829,.T.) ;
#46944=ADVANCED_FACE('',(#11726),#45607,.T.) ;
#46945=ADVANCED_FACE('',(#11727),#9830,.T.) ;
#46946=ADVANCED_FACE('',(#11728),#45608,.T.) ;
#46947=ADVANCED_FACE('',(#11729),#9831,.T.) ;
#46948=ADVANCED_FACE('',(#11730),#2191,.T.) ;
#46949=ADVANCED_FACE('',(#11731),#45609,.T.) ;
#46950=ADVANCED_FACE('',(#11732),#9832,.T.) ;
#46951=ADVANCED_FACE('',(#11733),#9833,.T.) ;
#46952=ADVANCED_FACE('',(#11734),#9834,.T.) ;
#46953=ADVANCED_FACE('',(#11735),#9835,.F.) ;
#46954=ADVANCED_FACE('',(#11736),#9836,.F.) ;
#46955=ADVANCED_FACE('',(#11737),#9837,.T.) ;
#46956=ADVANCED_FACE('',(#11738),#9838,.T.) ;
#46957=ADVANCED_FACE('',(#11739),#2373,.F.) ;
#46958=ADVANCED_FACE('',(#11740),#2374,.F.) ;
#46959=ADVANCED_FACE('',(#11741),#9839,.T.) ;
#46960=ADVANCED_FACE('',(#11742),#45610,.T.) ;
#46961=ADVANCED_FACE('',(#11743),#9840,.T.) ;
#46962=ADVANCED_FACE('',(#11744),#2375,.T.) ;
#46963=ADVANCED_FACE('',(#11745),#9841,.T.) ;
#46964=ADVANCED_FACE('',(#11746),#45611,.T.) ;
#46965=ADVANCED_FACE('',(#11747),#9842,.T.) ;
#46966=ADVANCED_FACE('',(#11748),#9843,.T.) ;
#46967=ADVANCED_FACE('',(#11749),#2376,.T.) ;
#46968=ADVANCED_FACE('',(#11750),#45612,.T.) ;
#46969=ADVANCED_FACE('',(#11751),#9844,.T.) ;
#46970=ADVANCED_FACE('',(#11752),#45613,.T.) ;
#46971=ADVANCED_FACE('',(#11753),#9845,.T.) ;
#46972=ADVANCED_FACE('',(#11754),#45614,.T.) ;
#46973=ADVANCED_FACE('',(#11755),#9846,.T.) ;
#46974=ADVANCED_FACE('',(#11756),#45615,.T.) ;
#46975=ADVANCED_FACE('',(#11757),#9847,.T.) ;
#46976=ADVANCED_FACE('',(#11758),#9848,.T.) ;
#46977=ADVANCED_FACE('',(#11759),#9849,.T.) ;
#46978=ADVANCED_FACE('',(#11760),#45616,.T.) ;
#46979=ADVANCED_FACE('',(#11761),#9850,.T.) ;
#46980=ADVANCED_FACE('',(#11762),#9851,.T.) ;
#46981=ADVANCED_FACE('',(#11763),#2377,.T.) ;
#46982=ADVANCED_FACE('',(#11764),#2378,.F.) ;
#46983=ADVANCED_FACE('',(#11765),#9852,.T.) ;
#46984=ADVANCED_FACE('',(#11766),#45617,.T.) ;
#46985=ADVANCED_FACE('',(#11767),#9853,.T.) ;
#46986=ADVANCED_FACE('',(#11768),#2379,.T.) ;
#46987=ADVANCED_FACE('',(#11769),#45618,.T.) ;
#46988=ADVANCED_FACE('',(#11770),#45619,.T.) ;
#46989=ADVANCED_FACE('',(#11771),#45620,.T.) ;
#46990=ADVANCED_FACE('',(#11772),#45621,.T.) ;
#46991=ADVANCED_FACE('',(#11773),#9854,.T.) ;
#46992=ADVANCED_FACE('',(#11774),#9855,.T.) ;
#46993=ADVANCED_FACE('',(#11775),#9856,.T.) ;
#46994=ADVANCED_FACE('',(#11776),#9857,.F.) ;
#46995=ADVANCED_FACE('',(#11777),#9858,.T.) ;
#46996=ADVANCED_FACE('',(#11778),#9859,.F.) ;
#46997=ADVANCED_FACE('',(#11779),#9860,.T.) ;
#46998=ADVANCED_FACE('',(#11780),#9861,.F.) ;
#46999=ADVANCED_FACE('',(#11781),#9862,.T.) ;
#47000=ADVANCED_FACE('',(#11782),#9863,.F.) ;
#47001=ADVANCED_FACE('',(#11783),#9864,.T.) ;
#47002=ADVANCED_FACE('',(#11784),#2380,.T.) ;
#47003=ADVANCED_FACE('',(#11785),#2381,.F.) ;
#47004=ADVANCED_FACE('',(#11786),#2382,.T.) ;
#47005=ADVANCED_FACE('',(#11787),#2383,.F.) ;
#47006=ADVANCED_FACE('',(#11788),#2384,.F.) ;
#47007=ADVANCED_FACE('',(#11789),#9865,.T.) ;
#47008=ADVANCED_FACE('',(#11790),#2385,.F.) ;
#47009=ADVANCED_FACE('',(#11791),#9866,.T.) ;
#47010=ADVANCED_FACE('',(#11792),#2386,.F.) ;
#47011=ADVANCED_FACE('',(#11793),#45622,.T.) ;
#47012=ADVANCED_FACE('',(#11794),#45623,.T.) ;
#47013=ADVANCED_FACE('',(#11795),#45624,.T.) ;
#47014=ADVANCED_FACE('',(#11796),#45625,.T.) ;
#47015=ADVANCED_FACE('',(#11797),#45626,.T.) ;
#47016=ADVANCED_FACE('',(#11798),#45627,.T.) ;
#47017=ADVANCED_FACE('',(#11799),#45628,.T.) ;
#47018=ADVANCED_FACE('',(#11800),#9867,.T.) ;
#47019=ADVANCED_FACE('',(#11801),#45629,.T.) ;
#47020=ADVANCED_FACE('',(#11802),#9868,.T.) ;
#47021=ADVANCED_FACE('',(#11803),#9869,.T.) ;
#47022=ADVANCED_FACE('',(#11804),#9870,.F.) ;
#47023=ADVANCED_FACE('',(#11805),#9871,.T.) ;
#47024=ADVANCED_FACE('',(#11806),#9872,.T.) ;
#47025=ADVANCED_FACE('',(#11807),#9873,.F.) ;
#47026=ADVANCED_FACE('',(#11808),#9874,.F.) ;
#47027=ADVANCED_FACE('',(#11809),#9875,.T.) ;
#47028=ADVANCED_FACE('',(#11810),#9876,.T.) ;
#47029=ADVANCED_FACE('',(#11811),#9877,.T.) ;
#47030=ADVANCED_FACE('',(#11812),#9878,.F.) ;
#47031=ADVANCED_FACE('',(#11813),#2387,.F.) ;
#47032=ADVANCED_FACE('',(#11814),#2388,.F.) ;
#47033=ADVANCED_FACE('',(#11815),#2389,.F.) ;
#47034=ADVANCED_FACE('',(#11816),#2390,.F.) ;
#47035=ADVANCED_FACE('',(#11817),#45630,.T.) ;
#47036=ADVANCED_FACE('',(#11818),#9879,.F.) ;
#47037=ADVANCED_FACE('',(#11819),#45631,.T.) ;
#47038=ADVANCED_FACE('',(#11820),#9880,.T.) ;
#47039=ADVANCED_FACE('',(#11821),#45632,.T.) ;
#47040=ADVANCED_FACE('',(#11822),#9881,.T.) ;
#47041=ADVANCED_FACE('',(#11823),#2391,.T.) ;
#47042=ADVANCED_FACE('',(#11824),#2392,.F.) ;
#47043=ADVANCED_FACE('',(#11825),#2393,.T.) ;
#47044=ADVANCED_FACE('',(#11826),#9882,.T.) ;
#47045=ADVANCED_FACE('',(#11827),#45633,.T.) ;
#47046=ADVANCED_FACE('',(#11828),#9883,.T.) ;
#47047=ADVANCED_FACE('',(#11829),#9884,.T.) ;
#47048=ADVANCED_FACE('',(#11830),#45634,.T.) ;
#47049=ADVANCED_FACE('',(#11831),#9885,.T.) ;
#47050=ADVANCED_FACE('',(#11832),#45635,.T.) ;
#47051=ADVANCED_FACE('',(#11833),#9886,.T.) ;
#47052=ADVANCED_FACE('',(#11834),#45636,.T.) ;
#47053=ADVANCED_FACE('',(#11835),#9887,.T.) ;
#47054=ADVANCED_FACE('',(#11836),#45637,.T.) ;
#47055=ADVANCED_FACE('',(#11837),#9888,.T.) ;
#47056=ADVANCED_FACE('',(#11838),#45638,.T.) ;
#47057=ADVANCED_FACE('',(#11839),#9889,.T.) ;
#47058=ADVANCED_FACE('',(#11840),#9890,.T.) ;
#47059=ADVANCED_FACE('',(#11841),#9891,.T.) ;
#47060=ADVANCED_FACE('',(#11842),#45639,.T.) ;
#47061=ADVANCED_FACE('',(#11843),#9892,.F.) ;
#47062=ADVANCED_FACE('',(#11844),#45640,.T.) ;
#47063=ADVANCED_FACE('',(#11845),#9893,.F.) ;
#47064=ADVANCED_FACE('',(#11846),#9894,.T.) ;
#47065=ADVANCED_FACE('',(#11847),#45641,.T.) ;
#47066=ADVANCED_FACE('',(#11848),#9895,.T.) ;
#47067=ADVANCED_FACE('',(#11849),#45642,.T.) ;
#47068=ADVANCED_FACE('',(#11850),#9896,.T.) ;
#47069=ADVANCED_FACE('',(#11851),#45643,.T.) ;
#47070=ADVANCED_FACE('',(#11852),#45644,.T.) ;
#47071=ADVANCED_FACE('',(#11853),#9897,.T.) ;
#47072=ADVANCED_FACE('',(#11854),#45645,.T.) ;
#47073=ADVANCED_FACE('',(#11855),#45646,.T.) ;
#47074=ADVANCED_FACE('',(#11856),#9898,.T.) ;
#47075=ADVANCED_FACE('',(#11857),#45647,.T.) ;
#47076=ADVANCED_FACE('',(#11858),#9899,.T.) ;
#47077=ADVANCED_FACE('',(#11859),#45648,.T.) ;
#47078=ADVANCED_FACE('',(#11860),#9900,.T.) ;
#47079=ADVANCED_FACE('',(#11861),#45649,.T.) ;
#47080=ADVANCED_FACE('',(#11862),#9901,.T.) ;
#47081=ADVANCED_FACE('',(#11863),#45650,.T.) ;
#47082=ADVANCED_FACE('',(#11864),#9902,.T.) ;
#47083=ADVANCED_FACE('',(#11865),#45651,.T.) ;
#47084=ADVANCED_FACE('',(#11866),#9903,.T.) ;
#47085=ADVANCED_FACE('',(#11867),#45652,.T.) ;
#47086=ADVANCED_FACE('',(#11868),#9904,.T.) ;
#47087=ADVANCED_FACE('',(#11869),#45653,.T.) ;
#47088=ADVANCED_FACE('',(#11870),#9905,.F.) ;
#47089=ADVANCED_FACE('',(#11871),#45654,.T.) ;
#47090=ADVANCED_FACE('',(#11872),#9906,.T.) ;
#47091=ADVANCED_FACE('',(#11873),#45655,.T.) ;
#47092=ADVANCED_FACE('',(#11874),#9907,.T.) ;
#47093=ADVANCED_FACE('',(#11875),#45656,.T.) ;
#47094=ADVANCED_FACE('',(#11876,#718),#2394,.T.) ;
#47095=ADVANCED_FACE('',(#11877),#45657,.F.) ;
#47096=ADVANCED_FACE('',(#11878),#9908,.F.) ;
#47097=ADVANCED_FACE('',(#11879),#45658,.T.) ;
#47098=ADVANCED_FACE('',(#11880),#45659,.T.) ;
#47099=ADVANCED_FACE('',(#11881),#9909,.F.) ;
#47100=ADVANCED_FACE('',(#11882),#45660,.F.) ;
#47101=ADVANCED_FACE('',(#11883,#719),#2395,.T.) ;
#47102=ADVANCED_FACE('',(#11884),#45661,.T.) ;
#47103=ADVANCED_FACE('',(#11885),#9910,.F.) ;
#47104=ADVANCED_FACE('',(#11886),#45662,.T.) ;
#47105=ADVANCED_FACE('',(#11887),#9911,.F.) ;
#47106=ADVANCED_FACE('',(#11888),#45663,.T.) ;
#47107=ADVANCED_FACE('',(#11889,#720),#2396,.T.) ;
#47108=ADVANCED_FACE('',(#11890),#45664,.F.) ;
#47109=ADVANCED_FACE('',(#11891),#45665,.T.) ;
#47110=ADVANCED_FACE('',(#11892),#45666,.T.) ;
#47111=ADVANCED_FACE('',(#11893),#45667,.T.) ;
#47112=ADVANCED_FACE('',(#11894,#721),#2397,.F.) ;
#47113=ADVANCED_FACE('',(#11895),#9912,.T.) ;
#47114=ADVANCED_FACE('',(#11896),#2398,.T.) ;
#47115=ADVANCED_FACE('',(#11897),#9913,.T.) ;
#47116=ADVANCED_FACE('',(#11898),#2399,.T.) ;
#47117=ADVANCED_FACE('',(#11899),#2400,.F.) ;
#47118=ADVANCED_FACE('',(#11900),#2401,.T.) ;
#47119=ADVANCED_FACE('',(#11901),#2402,.F.) ;
#47120=ADVANCED_FACE('',(#11902),#2403,.F.) ;
#47121=ADVANCED_FACE('',(#11903),#1973,.F.) ;
#47122=ADVANCED_FACE('',(#11904),#1974,.F.) ;
#47123=ADVANCED_FACE('',(#11905),#1975,.F.) ;
#47124=ADVANCED_FACE('',(#11906),#1976,.F.) ;
#47125=ADVANCED_FACE('',(#11907),#9914,.T.) ;
#47126=ADVANCED_FACE('',(#11908),#1977,.F.) ;
#47127=ADVANCED_FACE('',(#11909),#9915,.T.) ;
#47128=ADVANCED_FACE('',(#11910),#1978,.F.) ;
#47129=ADVANCED_FACE('',(#11911),#9916,.T.) ;
#47130=ADVANCED_FACE('',(#11912),#9917,.T.) ;
#47131=ADVANCED_FACE('',(#11913),#9918,.T.) ;
#47132=ADVANCED_FACE('',(#11914),#1979,.F.) ;
#47133=ADVANCED_FACE('',(#11915),#9919,.T.) ;
#47134=ADVANCED_FACE('',(#11916),#1980,.F.) ;
#47135=ADVANCED_FACE('',(#11917),#9920,.T.) ;
#47136=ADVANCED_FACE('',(#11918),#9921,.T.) ;
#47137=ADVANCED_FACE('',(#11919),#9922,.F.) ;
#47138=ADVANCED_FACE('',(#11920),#9923,.F.) ;
#47139=ADVANCED_FACE('',(#11921),#2404,.T.) ;
#47140=ADVANCED_FACE('',(#11922),#9924,.T.) ;
#47141=ADVANCED_FACE('',(#11923),#9925,.T.) ;
#47142=ADVANCED_FACE('',(#11924),#2405,.T.) ;
#47143=ADVANCED_FACE('',(#11925),#9926,.F.) ;
#47144=ADVANCED_FACE('',(#11926),#9927,.F.) ;
#47145=ADVANCED_FACE('',(#11927),#2406,.T.) ;
#47146=ADVANCED_FACE('',(#11928),#9928,.T.) ;
#47147=ADVANCED_FACE('',(#11929),#2407,.T.) ;
#47148=ADVANCED_FACE('',(#11930),#2408,.T.) ;
#47149=ADVANCED_FACE('',(#11931),#2409,.F.) ;
#47150=ADVANCED_FACE('',(#11932),#2410,.T.) ;
#47151=ADVANCED_FACE('',(#11933),#2411,.T.) ;
#47152=ADVANCED_FACE('',(#11934),#2412,.F.) ;
#47153=ADVANCED_FACE('',(#11935),#2413,.T.) ;
#47154=ADVANCED_FACE('',(#11936),#2414,.T.) ;
#47155=ADVANCED_FACE('',(#11937),#2415,.F.) ;
#47156=ADVANCED_FACE('',(#11938),#2416,.T.) ;
#47157=ADVANCED_FACE('',(#11939),#2417,.T.) ;
#47158=ADVANCED_FACE('',(#11940),#2418,.F.) ;
#47159=ADVANCED_FACE('',(#11941),#2419,.F.) ;
#47160=ADVANCED_FACE('',(#11942),#2420,.F.) ;
#47161=ADVANCED_FACE('',(#11943),#2421,.F.) ;
#47162=ADVANCED_FACE('',(#11944),#2422,.F.) ;
#47163=ADVANCED_FACE('',(#11945),#2423,.F.) ;
#47164=ADVANCED_FACE('',(#11946),#9929,.T.) ;
#47165=ADVANCED_FACE('',(#11947),#9930,.T.) ;
#47166=ADVANCED_FACE('',(#11948),#9931,.T.) ;
#47167=ADVANCED_FACE('',(#11949),#1981,.F.) ;
#47168=ADVANCED_FACE('',(#11950),#1982,.F.) ;
#47169=ADVANCED_FACE('',(#11951),#1983,.F.) ;
#47170=ADVANCED_FACE('',(#11952),#2424,.F.) ;
#47171=ADVANCED_FACE('',(#11953),#1984,.F.) ;
#47172=ADVANCED_FACE('',(#11954),#2425,.F.) ;
#47173=ADVANCED_FACE('',(#11955),#1985,.T.) ;
#47174=ADVANCED_FACE('',(#11956),#1986,.T.) ;
#47175=ADVANCED_FACE('',(#11957),#1987,.T.) ;
#47176=ADVANCED_FACE('',(#11958),#1988,.T.) ;
#47177=ADVANCED_FACE('',(#11959),#9932,.T.) ;
#47178=ADVANCED_FACE('',(#11960),#2426,.T.) ;
#49059=CLOSED_SHELL('',(#46426,#46427,#46428,#46429,#46430,#46431,#46432,
#46433,#46434,#46435,#46436,#46437,#46438,#46439,#46440,#46441,#46442,#46443,
#46444,#46445,#46446,#46447,#46448,#46449,#46450,#46451,#46452,#46453,#46454,
#46455,#46456,#46457,#46458,#46459,#46460,#46461,#46462,#46463,#46464,#46465,
#46466,#46467,#46468,#46469,#46470,#46471,#46472,#46473,#46474,#46475,#46476,
#46477,#46478,#46479,#46480,#46481,#46482,#46483,#46484,#46485,#46486,#46487,
#46488,#46489,#46490,#46491,#46492,#46493,#46494,#46495,#46496,#46497,#46498,
#46499,#46500,#46501,#46502,#46503,#46504,#46505,#46506,#46507,#46508,#46509,
#46510,#46511,#46512,#46513,#46514,#46515,#46516,#46517,#46518,#46519,#46520,
#46521,#46522,#46523,#46524,#46525,#46526,#46527,#46528,#46529,#46530,#46531,
#46532,#46533,#46534,#46535,#46536,#46537,#46538,#46539,#46540,#46541,#46542,
#46543,#46544,#46545,#46546,#46547,#46548,#46549,#46550,#46551,#46552,#46553,
#46554,#46555,#46556,#46557,#46558,#46559,#46560,#46561,#46562,#46563,#46564,
#46565,#46566,#46567,#46568,#46569,#46570,#46571,#46572,#46573,#46574,#46575,
#46576,#46577,#46578,#46579,#46580,#46581,#46582,#46583,#46584,#46585,#46586,
#46587,#46588,#46589,#46590,#46591,#46592,#46593,#46594,#46595,#46596,#46597,
#46598,#46599,#46600,#46601,#46602,#46603,#46604,#46605,#46606,#46607,#46608,
#46609,#46610,#46611,#46612,#46613,#46614,#46615,#46616,#46617,#46618,#46619,
#46620,#46621,#46622,#46623,#46624,#46625,#46626,#46627,#46628,#46629,#46630,
#46631,#46632,#46633,#46634,#46635,#46636,#46637,#46638,#46639,#46640,#46641,
#46642,#46643,#46644,#46645,#46646,#46647,#46648,#46649,#46650,#46651,#46652,
#46653,#46654,#46655,#46656,#46657,#46658,#46659,#46660,#46661,#46662,#46663,
#46664,#46665,#46666,#46667,#46668,#46669,#46670,#46671,#46672,#46673,#46674,
#46675,#46676,#46677,#46678,#46679,#46680,#46681,#46682,#46683,#46684,#46685,
#46686,#46687,#46688,#46689,#46690,#46691,#46692,#46693,#46694,#46695,#46696,
#46697,#46698,#46699,#46700,#46701,#46702,#46703,#46704,#46705,#46706,#46707,
#46708,#46709,#46710,#46711,#46712,#46713,#46714,#46715,#46716,#46717,#46718,
#46719,#46720,#46721,#46722,#46723,#46724,#46725,#46726,#46727,#46728,#46729,
#46730,#46731,#46732,#46733,#46734,#46735,#46736,#46737,#46738,#46739,#46740,
#46741,#46742,#46743,#46744,#46745,#46746,#46747,#46748,#46749,#46750,#46751,
#46752,#46753,#46754,#46755,#46756,#46757,#46758,#46759,#46760,#46761,#46762,
#46763,#46764,#46765,#46766,#46767,#46768,#46769,#46770,#46771,#46772,#46773,
#46774,#46775,#46776,#46777,#46778,#46779,#46780,#46781,#46782,#46783,#46784,
#46785,#46786,#46787,#46788,#46789,#46790,#46791,#46792,#46793,#46794,#46795,
#46796,#46797,#46798,#46799,#46800,#46801,#46802,#46803,#46804,#46805,#46806,
#46807,#46808,#46809,#46810,#46811,#46812,#46813,#46814,#46815,#46816,#46817,
#46818,#46819,#46820,#46821,#46822,#46823,#46824,#46825,#46826,#46827,#46828,
#46829,#46830,#46831,#46832,#46833,#46834,#46835,#46836,#46837,#46838,#46839,
#46840,#46841,#46842,#46843,#46844,#46845,#46846,#46847,#46848,#46849,#46850,
#46851,#46852,#46853,#46854,#46855,#46856,#46857,#46858,#46859,#46860,#46861,
#46862,#46863,#46864,#46865,#46866,#46867,#46868,#46869,#46870,#46871,#46872,
#46873,#46874,#46875,#46876,#46877,#46878,#46879,#46880,#46881,#46882,#46883,
#46884,#46885,#46886,#46887,#46888,#46889,#46890,#46891,#46892,#46893,#46894,
#46895,#46896,#46897,#46898,#46899,#46900,#46901,#46902,#46903,#46904,#46905,
#46906,#46907,#46908,#46909,#46910,#46911,#46912,#46913,#46914,#46915,#46916,
#46917,#46918,#46919,#46920,#46921,#46922,#46923,#46924,#46925,#46926,#46927,
#46928,#46929,#46930,#46931,#46932,#46933,#46934,#46935,#46936,#46937,#46938,
#46939,#46940,#46941,#46942,#46943,#46944,#46945,#46946,#46947,#46948,#46949,
#46950,#46951,#46952,#46953,#46954,#46955,#46956,#46957,#46958,#46959,#46960,
#46961,#46962,#46963,#46964,#46965,#46966,#46967,#46968,#46969,#46970,#46971,
#46972,#46973,#46974,#46975,#46976,#46977,#46978,#46979,#46980,#46981,#46982,
#46983,#46984,#46985,#46986,#46987,#46988,#46989,#46990,#46991,#46992,#46993,
#46994,#46995,#46996,#46997,#46998,#46999,#47000,#47001,#47002,#47003,#47004,
#47005,#47006,#47007,#47008,#47009,#47010,#47011,#47012,#47013,#47014,#47015,
#47016,#47017,#47018,#47019,#47020,#47021,#47022,#47023,#47024,#47025,#47026,
#47027,#47028,#47029,#47030,#47031,#47032,#47033,#47034,#47035,#47036,#47037,
#47038,#47039,#47040,#47041,#47042,#47043,#47044,#47045,#47046,#47047,#47048,
#47049,#47050,#47051,#47052,#47053,#47054,#47055,#47056,#47057,#47058,#47059,
#47060,#47061,#47062,#47063,#47064,#47065,#47066,#47067,#47068,#47069,#47070,
#47071,#47072,#47073,#47074,#47075,#47076,#47077,#47078,#47079,#47080,#47081,
#47082,#47083,#47084,#47085,#47086,#47087,#47088,#47089,#47090,#47091,#47092,
#47093,#47094,#47095,#47096,#47097,#47098,#47099,#47100,#47101,#47102,#47103,
#47104,#47105,#47106,#47107,#47108,#47109,#47110,#47111,#47112,#47113,#47114,
#47115,#47116,#47117,#47118,#47119,#47120,#47121,#47122,#47123,#47124,#47125,
#47126,#47127,#47128,#47129,#47130,#47131,#47132,#47133,#47134,#47135,#47136,
#47137,#47138,#47139,#47140,#47141,#47142,#47143,#47144,#47145,#47146,#47147,
#47148,#47149,#47150,#47151,#47152,#47153,#47154,#47155,#47156,#47157,#47158,
#47159,#47160,#47161,#47162,#47163,#47164,#47165,#47166,#47167,#47168,#47169,
#47170,#47171,#47172,#47173,#47174,#47175,#47176,#47177,#47178)) ;
#50164=AXIS2_PLACEMENT_3D('',#79197,#57096,#57097) ;
#50165=AXIS2_PLACEMENT_3D('',#79541,#57098,#57099) ;
#50166=AXIS2_PLACEMENT_3D('',#79545,#57101,#57102) ;
#50167=AXIS2_PLACEMENT_3D('',#79547,#57104,#57105) ;
#50168=AXIS2_PLACEMENT_3D('',#79552,#57108,#57109) ;
#50169=AXIS2_PLACEMENT_3D('',#79553,#57110,#57111) ;
#50170=AXIS2_PLACEMENT_3D('',#79726,#57114,#57115) ;
#50171=AXIS2_PLACEMENT_3D('',#79732,#57119,#57120) ;
#50172=AXIS2_PLACEMENT_3D('',#79736,#57123,#57124) ;
#50173=AXIS2_PLACEMENT_3D('',#79758,#57128,#57129) ;
#50174=AXIS2_PLACEMENT_3D('',#79872,#57138,#57139) ;
#50175=AXIS2_PLACEMENT_3D('',#79874,#57140,#57141) ;
#50176=AXIS2_PLACEMENT_3D('',#79899,#57143,#57144) ;
#50177=AXIS2_PLACEMENT_3D('',#79901,#57145,#57146) ;
#50178=AXIS2_PLACEMENT_3D('',#79903,#57148,#57149) ;
#50179=AXIS2_PLACEMENT_3D('',#80157,#57151,#57152) ;
#50180=AXIS2_PLACEMENT_3D('',#80263,#57153,#57154) ;
#50181=AXIS2_PLACEMENT_3D('',#80267,#57156,#57157) ;
#50182=AXIS2_PLACEMENT_3D('',#80268,#57158,#57159) ;
#50183=AXIS2_PLACEMENT_3D('',#80331,#57160,#57161) ;
#50184=AXIS2_PLACEMENT_3D('',#80333,#57162,#57163) ;
#50185=AXIS2_PLACEMENT_3D('',#80335,#57165,#57166) ;
#50186=AXIS2_PLACEMENT_3D('',#80338,#57168,#57169) ;
#50187=AXIS2_PLACEMENT_3D('',#80339,#57170,#57171) ;
#50188=AXIS2_PLACEMENT_3D('',#80342,#57173,#57174) ;
#50189=AXIS2_PLACEMENT_3D('',#80343,#57175,#57176) ;
#50190=AXIS2_PLACEMENT_3D('',#80868,#57181,#57182) ;
#50191=AXIS2_PLACEMENT_3D('',#80872,#57185,#57186) ;
#50192=AXIS2_PLACEMENT_3D('',#80876,#57189,#57190) ;
#50193=AXIS2_PLACEMENT_3D('',#80980,#57197,#57198) ;
#50194=AXIS2_PLACEMENT_3D('',#81071,#57201,#57202) ;
#50195=AXIS2_PLACEMENT_3D('',#81091,#57204,#57205) ;
#50196=AXIS2_PLACEMENT_3D('',#81092,#57206,#57207) ;
#50197=AXIS2_PLACEMENT_3D('',#81118,#57209,#57210) ;
#50198=AXIS2_PLACEMENT_3D('',#81227,#57211,#57212) ;
#50199=AXIS2_PLACEMENT_3D('',#81516,#57214,#57215) ;
#50200=AXIS2_PLACEMENT_3D('',#81517,#57216,#57217) ;
#50201=AXIS2_PLACEMENT_3D('',#81522,#57219,#57220) ;
#50202=AXIS2_PLACEMENT_3D('',#81525,#57222,#57223) ;
#50203=AXIS2_PLACEMENT_3D('',#81526,#57224,#57225) ;
#50204=AXIS2_PLACEMENT_3D('',#81531,#57228,#57229) ;
#50205=AXIS2_PLACEMENT_3D('',#81532,#57230,#57231) ;
#50206=AXIS2_PLACEMENT_3D('',#81535,#57234,#57235) ;
#50207=AXIS2_PLACEMENT_3D('',#81541,#57239,#57240) ;
#50208=AXIS2_PLACEMENT_3D('',#81545,#57243,#57244) ;
#50209=AXIS2_PLACEMENT_3D('',#81546,#57245,#57246) ;
#50210=AXIS2_PLACEMENT_3D('',#81551,#57248,#57249) ;
#50211=AXIS2_PLACEMENT_3D('',#81554,#57251,#57252) ;
#50212=AXIS2_PLACEMENT_3D('',#81555,#57253,#57254) ;
#50213=AXIS2_PLACEMENT_3D('',#81560,#57257,#57258) ;
#50214=AXIS2_PLACEMENT_3D('',#81561,#57259,#57260) ;
#50215=AXIS2_PLACEMENT_3D('',#81566,#57263,#57264) ;
#50216=AXIS2_PLACEMENT_3D('',#81567,#57265,#57266) ;
#50217=AXIS2_PLACEMENT_3D('',#81570,#57269,#57270) ;
#50218=AXIS2_PLACEMENT_3D('',#81576,#57274,#57275) ;
#50219=AXIS2_PLACEMENT_3D('',#81580,#57278,#57279) ;
#50220=AXIS2_PLACEMENT_3D('',#81581,#57280,#57281) ;
#50221=AXIS2_PLACEMENT_3D('',#81586,#57283,#57284) ;
#50222=AXIS2_PLACEMENT_3D('',#81589,#57286,#57287) ;
#50223=AXIS2_PLACEMENT_3D('',#81590,#57288,#57289) ;
#50224=AXIS2_PLACEMENT_3D('',#81595,#57292,#57293) ;
#50225=AXIS2_PLACEMENT_3D('',#81596,#57294,#57295) ;
#50226=AXIS2_PLACEMENT_3D('',#81599,#57298,#57299) ;
#50227=AXIS2_PLACEMENT_3D('',#81605,#57303,#57304) ;
#50228=AXIS2_PLACEMENT_3D('',#81609,#57307,#57308) ;
#50229=AXIS2_PLACEMENT_3D('',#81610,#57309,#57310) ;
#50230=AXIS2_PLACEMENT_3D('',#81634,#57312,#57313) ;
#50231=AXIS2_PLACEMENT_3D('',#81791,#57314,#57315) ;
#50232=AXIS2_PLACEMENT_3D('',#81793,#57316,#57317) ;
#50233=AXIS2_PLACEMENT_3D('',#81796,#57319,#57320) ;
#50234=AXIS2_PLACEMENT_3D('',#82250,#57321,#57322) ;
#50235=AXIS2_PLACEMENT_3D('',#82254,#57324,#57325) ;
#50236=AXIS2_PLACEMENT_3D('',#82257,#57327,#57328) ;
#50237=AXIS2_PLACEMENT_3D('',#82258,#57329,#57330) ;
#50238=AXIS2_PLACEMENT_3D('',#82262,#57332,#57333) ;
#50239=AXIS2_PLACEMENT_3D('',#82264,#57335,#57336) ;
#50240=AXIS2_PLACEMENT_3D('',#82268,#57338,#57339) ;
#50241=AXIS2_PLACEMENT_3D('',#82270,#57341,#57342) ;
#50242=AXIS2_PLACEMENT_3D('',#82304,#57345,#57346) ;
#50243=AXIS2_PLACEMENT_3D('',#82326,#57347,#57348) ;
#50244=AXIS2_PLACEMENT_3D('',#82500,#57350,#57351) ;
#50245=AXIS2_PLACEMENT_3D('',#82547,#57358,#57359) ;
#50246=AXIS2_PLACEMENT_3D('',#82549,#57361,#57362) ;
#50247=AXIS2_PLACEMENT_3D('',#82551,#57364,#57365) ;
#50248=AXIS2_PLACEMENT_3D('',#82553,#57367,#57368) ;
#50249=AXIS2_PLACEMENT_3D('',#82554,#57369,#57370) ;
#50250=AXIS2_PLACEMENT_3D('',#82563,#57374,#57375) ;
#50251=AXIS2_PLACEMENT_3D('',#82567,#57377,#57378) ;
#50252=AXIS2_PLACEMENT_3D('',#82573,#57381,#57382) ;
#50253=AXIS2_PLACEMENT_3D('',#82574,#57383,#57384) ;
#50254=AXIS2_PLACEMENT_3D('',#82580,#57387,#57388) ;
#50255=AXIS2_PLACEMENT_3D('',#82584,#57390,#57391) ;
#50256=AXIS2_PLACEMENT_3D('',#82592,#57395,#57396) ;
#50257=AXIS2_PLACEMENT_3D('',#82596,#57398,#57399) ;
#50258=AXIS2_PLACEMENT_3D('',#82600,#57401,#57402) ;
#50259=AXIS2_PLACEMENT_3D('',#82604,#57404,#57405) ;
#50260=AXIS2_PLACEMENT_3D('',#82608,#57407,#57408) ;
#50261=AXIS2_PLACEMENT_3D('',#82612,#57410,#57411) ;
#50262=AXIS2_PLACEMENT_3D('',#82616,#57413,#57414) ;
#50263=AXIS2_PLACEMENT_3D('',#82620,#57416,#57417) ;
#50264=AXIS2_PLACEMENT_3D('',#82624,#57419,#57420) ;
#50265=AXIS2_PLACEMENT_3D('',#82628,#57422,#57423) ;
#50266=AXIS2_PLACEMENT_3D('',#82632,#57425,#57426) ;
#50267=AXIS2_PLACEMENT_3D('',#82636,#57428,#57429) ;
#50268=AXIS2_PLACEMENT_3D('',#82638,#57430,#57431) ;
#50269=AXIS2_PLACEMENT_3D('',#82642,#57433,#57434) ;
#50270=AXIS2_PLACEMENT_3D('',#82644,#57435,#57436) ;
#50271=AXIS2_PLACEMENT_3D('',#82648,#57438,#57439) ;
#50272=AXIS2_PLACEMENT_3D('',#82651,#57441,#57442) ;
#50273=AXIS2_PLACEMENT_3D('',#82666,#57449,#57450) ;
#50274=AXIS2_PLACEMENT_3D('',#82670,#57452,#57453) ;
#50275=AXIS2_PLACEMENT_3D('',#82674,#57455,#57456) ;
#50276=AXIS2_PLACEMENT_3D('',#82680,#57459,#57460) ;
#50277=AXIS2_PLACEMENT_3D('',#82684,#57462,#57463) ;
#50278=AXIS2_PLACEMENT_3D('',#82690,#57466,#57467) ;
#50279=AXIS2_PLACEMENT_3D('',#82704,#57474,#57475) ;
#50280=AXIS2_PLACEMENT_3D('',#82708,#57477,#57478) ;
#50281=AXIS2_PLACEMENT_3D('',#82712,#57480,#57481) ;
#50282=AXIS2_PLACEMENT_3D('',#82716,#57483,#57484) ;
#50283=AXIS2_PLACEMENT_3D('',#82720,#57486,#57487) ;
#50284=AXIS2_PLACEMENT_3D('',#82723,#57489,#57490) ;
#50285=AXIS2_PLACEMENT_3D('',#82726,#57491,#57492) ;
#50286=AXIS2_PLACEMENT_3D('',#82732,#57495,#57496) ;
#50287=AXIS2_PLACEMENT_3D('',#82736,#57498,#57499) ;
#50288=AXIS2_PLACEMENT_3D('',#82742,#57502,#57503) ;
#50289=AXIS2_PLACEMENT_3D('',#82746,#57505,#57506) ;
#50290=AXIS2_PLACEMENT_3D('',#82750,#57508,#57509) ;
#50291=AXIS2_PLACEMENT_3D('',#82754,#57511,#57512) ;
#50292=AXIS2_PLACEMENT_3D('',#82760,#57515,#57516) ;
#50293=AXIS2_PLACEMENT_3D('',#82764,#57518,#57519) ;
#50294=AXIS2_PLACEMENT_3D('',#82770,#57522,#57523) ;
#50295=AXIS2_PLACEMENT_3D('',#82774,#57525,#57526) ;
#50296=AXIS2_PLACEMENT_3D('',#82778,#57528,#57529) ;
#50297=AXIS2_PLACEMENT_3D('',#82794,#57537,#57538) ;
#50298=AXIS2_PLACEMENT_3D('',#82798,#57540,#57541) ;
#50299=AXIS2_PLACEMENT_3D('',#82802,#57543,#57544) ;
#50300=AXIS2_PLACEMENT_3D('',#82806,#57546,#57547) ;
#50301=AXIS2_PLACEMENT_3D('',#82809,#57549,#57550) ;
#50302=AXIS2_PLACEMENT_3D('',#82814,#57552,#57553) ;
#50303=AXIS2_PLACEMENT_3D('',#82818,#57555,#57556) ;
#50304=AXIS2_PLACEMENT_3D('',#82822,#57558,#57559) ;
#50305=AXIS2_PLACEMENT_3D('',#82826,#57561,#57562) ;
#50306=AXIS2_PLACEMENT_3D('',#82830,#57564,#57565) ;
#50307=AXIS2_PLACEMENT_3D('',#82841,#57571,#57572) ;
#50308=AXIS2_PLACEMENT_3D('',#82843,#57573,#57574) ;
#50309=AXIS2_PLACEMENT_3D('',#82852,#57578,#57579) ;
#50310=AXIS2_PLACEMENT_3D('',#82856,#57581,#57582) ;
#50311=AXIS2_PLACEMENT_3D('',#82860,#57584,#57585) ;
#50312=AXIS2_PLACEMENT_3D('',#82864,#57587,#57588) ;
#50313=AXIS2_PLACEMENT_3D('',#82873,#57593,#57594) ;
#50314=AXIS2_PLACEMENT_3D('',#82875,#57595,#57596) ;
#50315=AXIS2_PLACEMENT_3D('',#82878,#57597,#57598) ;
#50316=AXIS2_PLACEMENT_3D('',#82882,#57600,#57601) ;
#50317=AXIS2_PLACEMENT_3D('',#82886,#57603,#57604) ;
#50318=AXIS2_PLACEMENT_3D('',#82890,#57606,#57607) ;
#50319=AXIS2_PLACEMENT_3D('',#82894,#57609,#57610) ;
#50320=AXIS2_PLACEMENT_3D('',#82898,#57612,#57613) ;
#50321=AXIS2_PLACEMENT_3D('',#82902,#57615,#57616) ;
#50322=AXIS2_PLACEMENT_3D('',#82908,#57619,#57620) ;
#50323=AXIS2_PLACEMENT_3D('',#82912,#57622,#57623) ;
#50324=AXIS2_PLACEMENT_3D('',#82918,#57626,#57627) ;
#50325=AXIS2_PLACEMENT_3D('',#82928,#57633,#57634) ;
#50326=AXIS2_PLACEMENT_3D('',#82929,#57635,#57636) ;
#50327=AXIS2_PLACEMENT_3D('',#82930,#57637,#57638) ;
#50328=AXIS2_PLACEMENT_3D('',#82931,#57639,#57640) ;
#50329=AXIS2_PLACEMENT_3D('',#82932,#57641,#57642) ;
#50330=AXIS2_PLACEMENT_3D('',#82933,#57643,#57644) ;
#50331=AXIS2_PLACEMENT_3D('',#82935,#57646,#57647) ;
#50332=AXIS2_PLACEMENT_3D('',#82936,#57648,#57649) ;
#50333=AXIS2_PLACEMENT_3D('',#82937,#57650,#57651) ;
#50334=AXIS2_PLACEMENT_3D('',#82938,#57652,#57653) ;
#50335=AXIS2_PLACEMENT_3D('',#82939,#57654,#57655) ;
#50336=AXIS2_PLACEMENT_3D('',#82940,#57656,#57657) ;
#50337=AXIS2_PLACEMENT_3D('',#82941,#57658,#57659) ;
#50338=AXIS2_PLACEMENT_3D('',#82944,#57661,#57662) ;
#50339=AXIS2_PLACEMENT_3D('',#82945,#57663,#57664) ;
#50340=AXIS2_PLACEMENT_3D('',#82947,#57666,#57667) ;
#50341=AXIS2_PLACEMENT_3D('',#82949,#57669,#57670) ;
#50342=AXIS2_PLACEMENT_3D('',#82950,#57671,#57672) ;
#50343=AXIS2_PLACEMENT_3D('',#82951,#57673,#57674) ;
#50344=AXIS2_PLACEMENT_3D('',#82952,#57675,#57676) ;
#50345=AXIS2_PLACEMENT_3D('',#82953,#57677,#57678) ;
#50346=AXIS2_PLACEMENT_3D('',#82954,#57679,#57680) ;
#50347=AXIS2_PLACEMENT_3D('',#82956,#57682,#57683) ;
#50348=AXIS2_PLACEMENT_3D('',#82957,#57684,#57685) ;
#50349=AXIS2_PLACEMENT_3D('',#83011,#57689,#57690) ;
#50350=AXIS2_PLACEMENT_3D('',#83014,#57691,#57692) ;
#50351=AXIS2_PLACEMENT_3D('',#83016,#57693,#57694) ;
#50352=AXIS2_PLACEMENT_3D('',#83017,#57695,#57696) ;
#50353=AXIS2_PLACEMENT_3D('',#83018,#57697,#57698) ;
#50354=AXIS2_PLACEMENT_3D('',#83019,#57699,#57700) ;
#50355=AXIS2_PLACEMENT_3D('',#83021,#57701,#57702) ;
#50356=AXIS2_PLACEMENT_3D('',#83022,#57703,#57704) ;
#50357=AXIS2_PLACEMENT_3D('',#83025,#57706,#57707) ;
#50358=AXIS2_PLACEMENT_3D('',#83026,#57708,#57709) ;
#50359=AXIS2_PLACEMENT_3D('',#83028,#57710,#57711) ;
#50360=AXIS2_PLACEMENT_3D('',#83029,#57712,#57713) ;
#50361=AXIS2_PLACEMENT_3D('',#83030,#57714,#57715) ;
#50362=AXIS2_PLACEMENT_3D('',#83032,#57716,#57717) ;
#50363=AXIS2_PLACEMENT_3D('',#83034,#57719,#57720) ;
#50364=AXIS2_PLACEMENT_3D('',#83036,#57721,#57722) ;
#50365=AXIS2_PLACEMENT_3D('',#83037,#57723,#57724) ;
#50366=AXIS2_PLACEMENT_3D('',#83038,#57725,#57726) ;
#50367=AXIS2_PLACEMENT_3D('',#83043,#57728,#57729) ;
#50368=AXIS2_PLACEMENT_3D('',#83055,#57735,#57736) ;
#50369=AXIS2_PLACEMENT_3D('',#83059,#57738,#57739) ;
#50370=AXIS2_PLACEMENT_3D('',#83063,#57741,#57742) ;
#50371=AXIS2_PLACEMENT_3D('',#83069,#57745,#57746) ;
#50372=AXIS2_PLACEMENT_3D('',#83073,#57748,#57749) ;
#50373=AXIS2_PLACEMENT_3D('',#83081,#57753,#57754) ;
#50374=AXIS2_PLACEMENT_3D('',#83085,#57756,#57757) ;
#50375=AXIS2_PLACEMENT_3D('',#83091,#57760,#57761) ;
#50376=AXIS2_PLACEMENT_3D('',#83095,#57763,#57764) ;
#50377=AXIS2_PLACEMENT_3D('',#83099,#57766,#57767) ;
#50378=AXIS2_PLACEMENT_3D('',#83101,#57768,#57769) ;
#50379=AXIS2_PLACEMENT_3D('',#83105,#57771,#57772) ;
#50380=AXIS2_PLACEMENT_3D('',#83107,#57773,#57774) ;
#50381=AXIS2_PLACEMENT_3D('',#83111,#57776,#57777) ;
#50382=AXIS2_PLACEMENT_3D('',#83115,#57779,#57780) ;
#50383=AXIS2_PLACEMENT_3D('',#83119,#57782,#57783) ;
#50384=AXIS2_PLACEMENT_3D('',#83123,#57785,#57786) ;
#50385=AXIS2_PLACEMENT_3D('',#83127,#57788,#57789) ;
#50386=AXIS2_PLACEMENT_3D('',#83131,#57791,#57792) ;
#50387=AXIS2_PLACEMENT_3D('',#83135,#57794,#57795) ;
#50388=AXIS2_PLACEMENT_3D('',#83157,#57799,#57800) ;
#50389=AXIS2_PLACEMENT_3D('',#83161,#57802,#57803) ;
#50390=AXIS2_PLACEMENT_3D('',#83164,#57805,#57806) ;
#50391=AXIS2_PLACEMENT_3D('',#83171,#57809,#57810) ;
#50392=AXIS2_PLACEMENT_3D('',#83175,#57812,#57813) ;
#50393=AXIS2_PLACEMENT_3D('',#83181,#57816,#57817) ;
#50394=AXIS2_PLACEMENT_3D('',#83185,#57819,#57820) ;
#50395=AXIS2_PLACEMENT_3D('',#83189,#57822,#57823) ;
#50396=AXIS2_PLACEMENT_3D('',#83192,#57825,#57826) ;
#50397=AXIS2_PLACEMENT_3D('',#83194,#57827,#57828) ;
#50398=AXIS2_PLACEMENT_3D('',#83196,#57829,#57830) ;
#50399=AXIS2_PLACEMENT_3D('',#83203,#57833,#57834) ;
#50400=AXIS2_PLACEMENT_3D('',#83207,#57836,#57837) ;
#50401=AXIS2_PLACEMENT_3D('',#83211,#57839,#57840) ;
#50402=AXIS2_PLACEMENT_3D('',#83215,#57842,#57843) ;
#50403=AXIS2_PLACEMENT_3D('',#83219,#57845,#57846) ;
#50404=AXIS2_PLACEMENT_3D('',#83223,#57848,#57849) ;
#50405=AXIS2_PLACEMENT_3D('',#83230,#57853,#57854) ;
#50406=AXIS2_PLACEMENT_3D('',#83235,#57856,#57857) ;
#50407=AXIS2_PLACEMENT_3D('',#83239,#57859,#57860) ;
#50408=AXIS2_PLACEMENT_3D('',#83243,#57862,#57863) ;
#50409=AXIS2_PLACEMENT_3D('',#83247,#57865,#57866) ;
#50410=AXIS2_PLACEMENT_3D('',#83251,#57868,#57869) ;
#50411=AXIS2_PLACEMENT_3D('',#83258,#57873,#57874) ;
#50412=AXIS2_PLACEMENT_3D('',#83261,#57875,#57876) ;
#50413=AXIS2_PLACEMENT_3D('',#83265,#57878,#57879) ;
#50414=AXIS2_PLACEMENT_3D('',#83269,#57881,#57882) ;
#50415=AXIS2_PLACEMENT_3D('',#83273,#57884,#57885) ;
#50416=AXIS2_PLACEMENT_3D('',#83292,#57891,#57892) ;
#50417=AXIS2_PLACEMENT_3D('',#83296,#57894,#57895) ;
#50418=AXIS2_PLACEMENT_3D('',#83300,#57897,#57898) ;
#50419=AXIS2_PLACEMENT_3D('',#83304,#57900,#57901) ;
#50420=AXIS2_PLACEMENT_3D('',#83328,#57906,#57907) ;
#50421=AXIS2_PLACEMENT_3D('',#83332,#57909,#57910) ;
#50422=AXIS2_PLACEMENT_3D('',#83336,#57912,#57913) ;
#50423=AXIS2_PLACEMENT_3D('',#83340,#57915,#57916) ;
#50424=AXIS2_PLACEMENT_3D('',#83353,#57919,#57920) ;
#50425=AXIS2_PLACEMENT_3D('',#83357,#57922,#57923) ;
#50426=AXIS2_PLACEMENT_3D('',#83361,#57925,#57926) ;
#50427=AXIS2_PLACEMENT_3D('',#83365,#57928,#57929) ;
#50428=AXIS2_PLACEMENT_3D('',#83371,#57932,#57933) ;
#50429=AXIS2_PLACEMENT_3D('',#83375,#57935,#57936) ;
#50430=AXIS2_PLACEMENT_3D('',#83381,#57939,#57940) ;
#50431=AXIS2_PLACEMENT_3D('',#83385,#57942,#57943) ;
#50432=AXIS2_PLACEMENT_3D('',#83389,#57945,#57946) ;
#50433=AXIS2_PLACEMENT_3D('',#83393,#57948,#57949) ;
#50434=AXIS2_PLACEMENT_3D('',#83399,#57952,#57953) ;
#50435=AXIS2_PLACEMENT_3D('',#83403,#57955,#57956) ;
#50436=AXIS2_PLACEMENT_3D('',#83426,#57959,#57960) ;
#50437=AXIS2_PLACEMENT_3D('',#83429,#57961,#57962) ;
#50438=AXIS2_PLACEMENT_3D('',#83430,#57963,#57964) ;
#50439=AXIS2_PLACEMENT_3D('',#83432,#57965,#57966) ;
#50440=AXIS2_PLACEMENT_3D('',#83433,#57967,#57968) ;
#50441=AXIS2_PLACEMENT_3D('',#83434,#57969,#57970) ;
#50442=AXIS2_PLACEMENT_3D('',#83437,#57971,#57972) ;
#50443=AXIS2_PLACEMENT_3D('',#83440,#57975,#57976) ;
#50444=AXIS2_PLACEMENT_3D('',#83443,#57977,#57978) ;
#50445=AXIS2_PLACEMENT_3D('',#83444,#57979,#57980) ;
#50446=AXIS2_PLACEMENT_3D('',#83445,#57981,#57982) ;
#50447=AXIS2_PLACEMENT_3D('',#83446,#57983,#57984) ;
#50448=AXIS2_PLACEMENT_3D('',#83449,#57985,#57986) ;
#50449=AXIS2_PLACEMENT_3D('',#83452,#57989,#57990) ;
#50450=AXIS2_PLACEMENT_3D('',#83455,#57991,#57992) ;
#50451=AXIS2_PLACEMENT_3D('',#83456,#57993,#57994) ;
#50452=AXIS2_PLACEMENT_3D('',#83457,#57995,#57996) ;
#50453=AXIS2_PLACEMENT_3D('',#83458,#57997,#57998) ;
#50454=AXIS2_PLACEMENT_3D('',#83461,#57999,#58000) ;
#50455=AXIS2_PLACEMENT_3D('',#83464,#58003,#58004) ;
#50456=AXIS2_PLACEMENT_3D('',#83467,#58005,#58006) ;
#50457=AXIS2_PLACEMENT_3D('',#83468,#58007,#58008) ;
#50458=AXIS2_PLACEMENT_3D('',#83469,#58009,#58010) ;
#50459=AXIS2_PLACEMENT_3D('',#83470,#58011,#58012) ;
#50460=AXIS2_PLACEMENT_3D('',#83473,#58013,#58014) ;
#50461=AXIS2_PLACEMENT_3D('',#83476,#58017,#58018) ;
#50462=AXIS2_PLACEMENT_3D('',#83479,#58019,#58020) ;
#50463=AXIS2_PLACEMENT_3D('',#83480,#58021,#58022) ;
#50464=AXIS2_PLACEMENT_3D('',#83481,#58023,#58024) ;
#50465=AXIS2_PLACEMENT_3D('',#83482,#58025,#58026) ;
#50466=AXIS2_PLACEMENT_3D('',#83485,#58027,#58028) ;
#50467=AXIS2_PLACEMENT_3D('',#83488,#58031,#58032) ;
#50468=AXIS2_PLACEMENT_3D('',#83491,#58033,#58034) ;
#50469=AXIS2_PLACEMENT_3D('',#83492,#58035,#58036) ;
#50470=AXIS2_PLACEMENT_3D('',#83493,#58037,#58038) ;
#50471=AXIS2_PLACEMENT_3D('',#83494,#58039,#58040) ;
#50472=AXIS2_PLACEMENT_3D('',#83497,#58041,#58042) ;
#50473=AXIS2_PLACEMENT_3D('',#83500,#58045,#58046) ;
#50474=AXIS2_PLACEMENT_3D('',#83502,#58047,#58048) ;
#50475=AXIS2_PLACEMENT_3D('',#83503,#58049,#58050) ;
#50476=AXIS2_PLACEMENT_3D('',#83504,#58051,#58052) ;
#50477=AXIS2_PLACEMENT_3D('',#83505,#58053,#58054) ;
#50478=AXIS2_PLACEMENT_3D('',#83511,#58057,#58058) ;
#50479=AXIS2_PLACEMENT_3D('',#83517,#58062,#58063) ;
#50480=AXIS2_PLACEMENT_3D('',#83520,#58065,#58066) ;
#50481=AXIS2_PLACEMENT_3D('',#83521,#58067,#58068) ;
#50482=AXIS2_PLACEMENT_3D('',#83525,#58071,#58072) ;
#50483=AXIS2_PLACEMENT_3D('',#83528,#58074,#58075) ;
#50484=AXIS2_PLACEMENT_3D('',#83529,#58076,#58077) ;
#50485=AXIS2_PLACEMENT_3D('',#83533,#58080,#58081) ;
#50486=AXIS2_PLACEMENT_3D('',#83536,#58083,#58084) ;
#50487=AXIS2_PLACEMENT_3D('',#83537,#58085,#58086) ;
#50488=AXIS2_PLACEMENT_3D('',#83541,#58089,#58090) ;
#50489=AXIS2_PLACEMENT_3D('',#83544,#58092,#58093) ;
#50490=AXIS2_PLACEMENT_3D('',#83545,#58094,#58095) ;
#50491=AXIS2_PLACEMENT_3D('',#83549,#58098,#58099) ;
#50492=AXIS2_PLACEMENT_3D('',#83552,#58101,#58102) ;
#50493=AXIS2_PLACEMENT_3D('',#83553,#58103,#58104) ;
#50494=AXIS2_PLACEMENT_3D('',#83561,#58108,#58109) ;
#50495=AXIS2_PLACEMENT_3D('',#83563,#58111,#58112) ;
#50496=AXIS2_PLACEMENT_3D('',#83565,#58113,#58114) ;
#50497=AXIS2_PLACEMENT_3D('',#83566,#58115,#58116) ;
#50498=AXIS2_PLACEMENT_3D('',#83567,#58117,#58118) ;
#50499=AXIS2_PLACEMENT_3D('',#83570,#58120,#58121) ;
#50500=AXIS2_PLACEMENT_3D('',#83687,#58123,#58124) ;
#50501=AXIS2_PLACEMENT_3D('',#83689,#58125,#58126) ;
#50502=AXIS2_PLACEMENT_3D('',#83690,#58127,#58128) ;
#50503=AXIS2_PLACEMENT_3D('',#83691,#58129,#58130) ;
#50504=AXIS2_PLACEMENT_3D('',#83693,#58131,#58132) ;
#50505=AXIS2_PLACEMENT_3D('',#83694,#58133,#58134) ;
#50506=AXIS2_PLACEMENT_3D('',#83697,#58135,#58136) ;
#50507=AXIS2_PLACEMENT_3D('',#83698,#58137,#58138) ;
#50508=AXIS2_PLACEMENT_3D('',#83699,#58139,#58140) ;
#50509=AXIS2_PLACEMENT_3D('',#83700,#58141,#58142) ;
#50510=AXIS2_PLACEMENT_3D('',#83703,#58144,#58145) ;
#50511=AXIS2_PLACEMENT_3D('',#83704,#58146,#58147) ;
#50512=AXIS2_PLACEMENT_3D('',#83706,#58148,#58149) ;
#50513=AXIS2_PLACEMENT_3D('',#83708,#58150,#58151) ;
#50514=AXIS2_PLACEMENT_3D('',#83710,#58152,#58153) ;
#50515=AXIS2_PLACEMENT_3D('',#83711,#58154,#58155) ;
#50516=AXIS2_PLACEMENT_3D('',#83712,#58156,#58157) ;
#50517=AXIS2_PLACEMENT_3D('',#83716,#58159,#58160) ;
#50518=AXIS2_PLACEMENT_3D('',#83717,#58161,#58162) ;
#50519=AXIS2_PLACEMENT_3D('',#83718,#58163,#58164) ;
#50520=AXIS2_PLACEMENT_3D('',#83725,#58167,#58168) ;
#50521=AXIS2_PLACEMENT_3D('',#83729,#58170,#58171) ;
#50522=AXIS2_PLACEMENT_3D('',#83731,#58173,#58174) ;
#50523=AXIS2_PLACEMENT_3D('',#83733,#58175,#58176) ;
#50524=AXIS2_PLACEMENT_3D('',#83734,#58177,#58178) ;
#50525=AXIS2_PLACEMENT_3D('',#83735,#58179,#58180) ;
#50526=AXIS2_PLACEMENT_3D('',#83753,#58184,#58185) ;
#50527=AXIS2_PLACEMENT_3D('',#83755,#58186,#58187) ;
#50528=AXIS2_PLACEMENT_3D('',#83757,#58188,#58189) ;
#50529=AXIS2_PLACEMENT_3D('',#83759,#58190,#58191) ;
#50530=AXIS2_PLACEMENT_3D('',#83760,#58192,#58193) ;
#50531=AXIS2_PLACEMENT_3D('',#83761,#58194,#58195) ;
#50532=AXIS2_PLACEMENT_3D('',#83765,#58197,#58198) ;
#50533=AXIS2_PLACEMENT_3D('',#83766,#58199,#58200) ;
#50534=AXIS2_PLACEMENT_3D('',#83767,#58201,#58202) ;
#50535=AXIS2_PLACEMENT_3D('',#83774,#58205,#58206) ;
#50536=AXIS2_PLACEMENT_3D('',#83778,#58208,#58209) ;
#50537=AXIS2_PLACEMENT_3D('',#83780,#58211,#58212) ;
#50538=AXIS2_PLACEMENT_3D('',#83782,#58213,#58214) ;
#50539=AXIS2_PLACEMENT_3D('',#83783,#58215,#58216) ;
#50540=AXIS2_PLACEMENT_3D('',#83784,#58217,#58218) ;
#50541=AXIS2_PLACEMENT_3D('',#83802,#58222,#58223) ;
#50542=AXIS2_PLACEMENT_3D('',#83804,#58224,#58225) ;
#50543=AXIS2_PLACEMENT_3D('',#83806,#58226,#58227) ;
#50544=AXIS2_PLACEMENT_3D('',#83807,#58228,#58229) ;
#50545=AXIS2_PLACEMENT_3D('',#83808,#58230,#58231) ;
#50546=AXIS2_PLACEMENT_3D('',#83810,#58232,#58233) ;
#50547=AXIS2_PLACEMENT_3D('',#83812,#58235,#58236) ;
#50548=AXIS2_PLACEMENT_3D('',#83814,#58237,#58238) ;
#50549=AXIS2_PLACEMENT_3D('',#83815,#58239,#58240) ;
#50550=AXIS2_PLACEMENT_3D('',#83816,#58241,#58242) ;
#50551=AXIS2_PLACEMENT_3D('',#83818,#58243,#58244) ;
#50552=AXIS2_PLACEMENT_3D('',#83820,#58246,#58247) ;
#50553=AXIS2_PLACEMENT_3D('',#83822,#58248,#58249) ;
#50554=AXIS2_PLACEMENT_3D('',#83823,#58250,#58251) ;
#50555=AXIS2_PLACEMENT_3D('',#83824,#58252,#58253) ;
#50556=AXIS2_PLACEMENT_3D('',#83828,#58255,#58256) ;
#50557=AXIS2_PLACEMENT_3D('',#83890,#58266,#58267) ;
#50558=AXIS2_PLACEMENT_3D('',#83892,#58269,#58270) ;
#50559=AXIS2_PLACEMENT_3D('',#83893,#58271,#58272) ;
#50560=AXIS2_PLACEMENT_3D('',#83894,#58273,#58274) ;
#50561=AXIS2_PLACEMENT_3D('',#83898,#58276,#58277) ;
#50562=AXIS2_PLACEMENT_3D('',#83937,#58278,#58279) ;
#50563=AXIS2_PLACEMENT_3D('',#83942,#58282,#58283) ;
#50564=AXIS2_PLACEMENT_3D('',#83981,#58284,#58285) ;
#50565=AXIS2_PLACEMENT_3D('',#83985,#58287,#58288) ;
#50566=AXIS2_PLACEMENT_3D('',#84000,#58291,#58292) ;
#50567=AXIS2_PLACEMENT_3D('',#84001,#58293,#58294) ;
#50568=AXIS2_PLACEMENT_3D('',#84002,#58295,#58296) ;
#50569=AXIS2_PLACEMENT_3D('',#84016,#58297,#58298) ;
#50570=AXIS2_PLACEMENT_3D('',#84038,#58299,#58300) ;
#50571=AXIS2_PLACEMENT_3D('',#84039,#58301,#58302) ;
#50572=AXIS2_PLACEMENT_3D('',#84061,#58303,#58304) ;
#50573=AXIS2_PLACEMENT_3D('',#84081,#58305,#58306) ;
#50574=AXIS2_PLACEMENT_3D('',#84083,#58307,#58308) ;
#50575=AXIS2_PLACEMENT_3D('',#84110,#58310,#58311) ;
#50576=AXIS2_PLACEMENT_3D('',#84116,#58312,#58313) ;
#50577=AXIS2_PLACEMENT_3D('',#84117,#58314,#58315) ;
#50578=AXIS2_PLACEMENT_3D('',#84118,#58316,#58317) ;
#50579=AXIS2_PLACEMENT_3D('',#84119,#58318,#58319) ;
#50580=AXIS2_PLACEMENT_3D('',#84121,#58320,#58321) ;
#50581=AXIS2_PLACEMENT_3D('',#84123,#58322,#58323) ;
#50582=AXIS2_PLACEMENT_3D('',#84124,#58324,#58325) ;
#50583=AXIS2_PLACEMENT_3D('',#84125,#58326,#58327) ;
#50584=AXIS2_PLACEMENT_3D('',#84127,#58328,#58329) ;
#50585=AXIS2_PLACEMENT_3D('',#84129,#58331,#58332) ;
#50586=AXIS2_PLACEMENT_3D('',#84131,#58333,#58334) ;
#50587=AXIS2_PLACEMENT_3D('',#84132,#58335,#58336) ;
#50588=AXIS2_PLACEMENT_3D('',#84133,#58337,#58338) ;
#50589=AXIS2_PLACEMENT_3D('',#84135,#58339,#58340) ;
#50590=AXIS2_PLACEMENT_3D('',#84137,#58342,#58343) ;
#50591=AXIS2_PLACEMENT_3D('',#84150,#58344,#58345) ;
#50592=AXIS2_PLACEMENT_3D('',#84156,#58346,#58347) ;
#50593=AXIS2_PLACEMENT_3D('',#84158,#58348,#58349) ;
#50594=AXIS2_PLACEMENT_3D('',#84160,#58350,#58351) ;
#50595=AXIS2_PLACEMENT_3D('',#84161,#58352,#58353) ;
#50596=AXIS2_PLACEMENT_3D('',#84162,#58354,#58355) ;
#50597=AXIS2_PLACEMENT_3D('',#84164,#58356,#58357) ;
#50598=AXIS2_PLACEMENT_3D('',#84166,#58359,#58360) ;
#50599=AXIS2_PLACEMENT_3D('',#84168,#58361,#58362) ;
#50600=AXIS2_PLACEMENT_3D('',#84169,#58363,#58364) ;
#50601=AXIS2_PLACEMENT_3D('',#84170,#58365,#58366) ;
#50602=AXIS2_PLACEMENT_3D('',#84173,#58367,#58368) ;
#50603=AXIS2_PLACEMENT_3D('',#84174,#58369,#58370) ;
#50604=AXIS2_PLACEMENT_3D('',#84175,#58371,#58372) ;
#50605=AXIS2_PLACEMENT_3D('',#84176,#58373,#58374) ;
#50606=AXIS2_PLACEMENT_3D('',#84179,#58377,#58378) ;
#50607=AXIS2_PLACEMENT_3D('',#84181,#58379,#58380) ;
#50608=AXIS2_PLACEMENT_3D('',#84183,#58381,#58382) ;
#50609=AXIS2_PLACEMENT_3D('',#84184,#58383,#58384) ;
#50610=AXIS2_PLACEMENT_3D('',#84185,#58385,#58386) ;
#50611=AXIS2_PLACEMENT_3D('',#84188,#58387,#58388) ;
#50612=AXIS2_PLACEMENT_3D('',#84189,#58389,#58390) ;
#50613=AXIS2_PLACEMENT_3D('',#84190,#58391,#58392) ;
#50614=AXIS2_PLACEMENT_3D('',#84191,#58393,#58394) ;
#50615=AXIS2_PLACEMENT_3D('',#84193,#58396,#58397) ;
#50616=AXIS2_PLACEMENT_3D('',#84195,#58399,#58400) ;
#50617=AXIS2_PLACEMENT_3D('',#84198,#58401,#58402) ;
#50618=AXIS2_PLACEMENT_3D('',#84199,#58403,#58404) ;
#50619=AXIS2_PLACEMENT_3D('',#84200,#58405,#58406) ;
#50620=AXIS2_PLACEMENT_3D('',#84201,#58407,#58408) ;
#50621=AXIS2_PLACEMENT_3D('',#84204,#58411,#58412) ;
#50622=AXIS2_PLACEMENT_3D('',#84207,#58413,#58414) ;
#50623=AXIS2_PLACEMENT_3D('',#84210,#58417,#58418) ;
#50624=AXIS2_PLACEMENT_3D('',#84211,#58419,#58420) ;
#50625=AXIS2_PLACEMENT_3D('',#84212,#58421,#58422) ;
#50626=AXIS2_PLACEMENT_3D('',#84213,#58423,#58424) ;
#50627=AXIS2_PLACEMENT_3D('',#84215,#58425,#58426) ;
#50628=AXIS2_PLACEMENT_3D('',#84217,#58428,#58429) ;
#50629=AXIS2_PLACEMENT_3D('',#84219,#58430,#58431) ;
#50630=AXIS2_PLACEMENT_3D('',#84220,#58432,#58433) ;
#50631=AXIS2_PLACEMENT_3D('',#84221,#58434,#58435) ;
#50632=AXIS2_PLACEMENT_3D('',#84224,#58437,#58438) ;
#50633=AXIS2_PLACEMENT_3D('',#84225,#58439,#58440) ;
#50634=AXIS2_PLACEMENT_3D('',#84227,#58442,#58443) ;
#50635=AXIS2_PLACEMENT_3D('',#84230,#58445,#58446) ;
#50636=AXIS2_PLACEMENT_3D('',#84231,#58447,#58448) ;
#50637=AXIS2_PLACEMENT_3D('',#84235,#58450,#58451) ;
#50638=AXIS2_PLACEMENT_3D('',#84237,#58453,#58454) ;
#50639=AXIS2_PLACEMENT_3D('',#84239,#58456,#58457) ;
#50640=AXIS2_PLACEMENT_3D('',#84242,#58458,#58459) ;
#50641=AXIS2_PLACEMENT_3D('',#84243,#58460,#58461) ;
#50642=AXIS2_PLACEMENT_3D('',#84244,#58462,#58463) ;
#50643=AXIS2_PLACEMENT_3D('',#84245,#58464,#58465) ;
#50644=AXIS2_PLACEMENT_3D('',#84248,#58466,#58467) ;
#50645=AXIS2_PLACEMENT_3D('',#84271,#58470,#58471) ;
#50646=AXIS2_PLACEMENT_3D('',#84272,#58472,#58473) ;
#50647=AXIS2_PLACEMENT_3D('',#84273,#58474,#58475) ;
#50648=AXIS2_PLACEMENT_3D('',#84276,#58477,#58478) ;
#50649=AXIS2_PLACEMENT_3D('',#84277,#58479,#58480) ;
#50650=AXIS2_PLACEMENT_3D('',#84301,#58482,#58483) ;
#50651=AXIS2_PLACEMENT_3D('',#84302,#58484,#58485) ;
#50652=AXIS2_PLACEMENT_3D('',#84303,#58486,#58487) ;
#50653=AXIS2_PLACEMENT_3D('',#84304,#58488,#58489) ;
#50654=AXIS2_PLACEMENT_3D('',#84307,#58490,#58491) ;
#50655=AXIS2_PLACEMENT_3D('',#84310,#58494,#58495) ;
#50656=AXIS2_PLACEMENT_3D('',#84311,#58496,#58497) ;
#50657=AXIS2_PLACEMENT_3D('',#84312,#58498,#58499) ;
#50658=AXIS2_PLACEMENT_3D('',#84313,#58500,#58501) ;
#50659=AXIS2_PLACEMENT_3D('',#84317,#58504,#58505) ;
#50660=AXIS2_PLACEMENT_3D('',#84318,#58506,#58507) ;
#50661=AXIS2_PLACEMENT_3D('',#84319,#58508,#58509) ;
#50662=AXIS2_PLACEMENT_3D('',#84321,#58510,#58511) ;
#50663=AXIS2_PLACEMENT_3D('',#84323,#58512,#58513) ;
#50664=AXIS2_PLACEMENT_3D('',#84325,#58515,#58516) ;
#50665=AXIS2_PLACEMENT_3D('',#84327,#58517,#58518) ;
#50666=AXIS2_PLACEMENT_3D('',#84328,#58519,#58520) ;
#50667=AXIS2_PLACEMENT_3D('',#84329,#58521,#58522) ;
#50668=AXIS2_PLACEMENT_3D('',#84331,#58523,#58524) ;
#50669=AXIS2_PLACEMENT_3D('',#84333,#58526,#58527) ;
#50670=AXIS2_PLACEMENT_3D('',#84335,#58528,#58529) ;
#50671=AXIS2_PLACEMENT_3D('',#84336,#58530,#58531) ;
#50672=AXIS2_PLACEMENT_3D('',#84337,#58532,#58533) ;
#50673=AXIS2_PLACEMENT_3D('',#84339,#58534,#58535) ;
#50674=AXIS2_PLACEMENT_3D('',#84341,#58537,#58538) ;
#50675=AXIS2_PLACEMENT_3D('',#84342,#58539,#58540) ;
#50676=AXIS2_PLACEMENT_3D('',#84343,#58541,#58542) ;
#50677=AXIS2_PLACEMENT_3D('',#84345,#58543,#58544) ;
#50678=AXIS2_PLACEMENT_3D('',#84347,#58546,#58547) ;
#50679=AXIS2_PLACEMENT_3D('',#84353,#58551,#58552) ;
#50680=AXIS2_PLACEMENT_3D('',#84356,#58554,#58555) ;
#50681=AXIS2_PLACEMENT_3D('',#84357,#58556,#58557) ;
#50682=AXIS2_PLACEMENT_3D('',#84361,#58560,#58561) ;
#50683=AXIS2_PLACEMENT_3D('',#84364,#58563,#58564) ;
#50684=AXIS2_PLACEMENT_3D('',#84365,#58565,#58566) ;
#50685=AXIS2_PLACEMENT_3D('',#84369,#58569,#58570) ;
#50686=AXIS2_PLACEMENT_3D('',#84372,#58572,#58573) ;
#50687=AXIS2_PLACEMENT_3D('',#84373,#58574,#58575) ;
#50688=AXIS2_PLACEMENT_3D('',#84377,#58578,#58579) ;
#50689=AXIS2_PLACEMENT_3D('',#84380,#58581,#58582) ;
#50690=AXIS2_PLACEMENT_3D('',#84381,#58583,#58584) ;
#50691=AXIS2_PLACEMENT_3D('',#84385,#58587,#58588) ;
#50692=AXIS2_PLACEMENT_3D('',#84388,#58590,#58591) ;
#50693=AXIS2_PLACEMENT_3D('',#84389,#58592,#58593) ;
#50694=AXIS2_PLACEMENT_3D('',#84393,#58596,#58597) ;
#50695=AXIS2_PLACEMENT_3D('',#84395,#58598,#58599) ;
#50696=AXIS2_PLACEMENT_3D('',#84398,#58601,#58602) ;
#50697=AXIS2_PLACEMENT_3D('',#84399,#58603,#58604) ;
#50698=AXIS2_PLACEMENT_3D('',#84401,#58605,#58606) ;
#50699=AXIS2_PLACEMENT_3D('',#84402,#58607,#58608) ;
#50700=AXIS2_PLACEMENT_3D('',#84403,#58609,#58610) ;
#50701=AXIS2_PLACEMENT_3D('',#84405,#58611,#58612) ;
#50702=AXIS2_PLACEMENT_3D('',#84407,#58614,#58615) ;
#50703=AXIS2_PLACEMENT_3D('',#84409,#58616,#58617) ;
#50704=AXIS2_PLACEMENT_3D('',#84410,#58618,#58619) ;
#50705=AXIS2_PLACEMENT_3D('',#84411,#58620,#58621) ;
#50706=AXIS2_PLACEMENT_3D('',#84413,#58622,#58623) ;
#50707=AXIS2_PLACEMENT_3D('',#84415,#58625,#58626) ;
#50708=AXIS2_PLACEMENT_3D('',#84417,#58627,#58628) ;
#50709=AXIS2_PLACEMENT_3D('',#84418,#58629,#58630) ;
#50710=AXIS2_PLACEMENT_3D('',#84419,#58631,#58632) ;
#50711=AXIS2_PLACEMENT_3D('',#84421,#58633,#58634) ;
#50712=AXIS2_PLACEMENT_3D('',#84423,#58636,#58637) ;
#50713=AXIS2_PLACEMENT_3D('',#84425,#58638,#58639) ;
#50714=AXIS2_PLACEMENT_3D('',#84426,#58640,#58641) ;
#50715=AXIS2_PLACEMENT_3D('',#84427,#58642,#58643) ;
#50716=AXIS2_PLACEMENT_3D('',#84429,#58644,#58645) ;
#50717=AXIS2_PLACEMENT_3D('',#84431,#58647,#58648) ;
#50718=AXIS2_PLACEMENT_3D('',#84433,#58649,#58650) ;
#50719=AXIS2_PLACEMENT_3D('',#84436,#58652,#58653) ;
#50720=AXIS2_PLACEMENT_3D('',#84437,#58654,#58655) ;
#50721=AXIS2_PLACEMENT_3D('',#84439,#58656,#58657) ;
#50722=AXIS2_PLACEMENT_3D('',#84440,#58658,#58659) ;
#50723=AXIS2_PLACEMENT_3D('',#84441,#58660,#58661) ;
#50724=AXIS2_PLACEMENT_3D('',#84443,#58662,#58663) ;
#50725=AXIS2_PLACEMENT_3D('',#84445,#58665,#58666) ;
#50726=AXIS2_PLACEMENT_3D('',#84447,#58667,#58668) ;
#50727=AXIS2_PLACEMENT_3D('',#84448,#58669,#58670) ;
#50728=AXIS2_PLACEMENT_3D('',#84449,#58671,#58672) ;
#50729=AXIS2_PLACEMENT_3D('',#84451,#58673,#58674) ;
#50730=AXIS2_PLACEMENT_3D('',#84453,#58676,#58677) ;
#50731=AXIS2_PLACEMENT_3D('',#84454,#58678,#58679) ;
#50732=AXIS2_PLACEMENT_3D('',#84455,#58680,#58681) ;
#50733=AXIS2_PLACEMENT_3D('',#84456,#58682,#58683) ;
#50734=AXIS2_PLACEMENT_3D('',#84457,#58684,#58685) ;
#50735=AXIS2_PLACEMENT_3D('',#84461,#58687,#58688) ;
#50736=AXIS2_PLACEMENT_3D('',#84463,#58690,#58691) ;
#50737=AXIS2_PLACEMENT_3D('',#84467,#58694,#58695) ;
#50738=AXIS2_PLACEMENT_3D('',#84470,#58697,#58698) ;
#50739=AXIS2_PLACEMENT_3D('',#84471,#58699,#58700) ;
#50740=AXIS2_PLACEMENT_3D('',#84475,#58703,#58704) ;
#50741=AXIS2_PLACEMENT_3D('',#84478,#58706,#58707) ;
#50742=AXIS2_PLACEMENT_3D('',#84479,#58708,#58709) ;
#50743=AXIS2_PLACEMENT_3D('',#84483,#58712,#58713) ;
#50744=AXIS2_PLACEMENT_3D('',#84486,#58715,#58716) ;
#50745=AXIS2_PLACEMENT_3D('',#84487,#58717,#58718) ;
#50746=AXIS2_PLACEMENT_3D('',#84491,#58721,#58722) ;
#50747=AXIS2_PLACEMENT_3D('',#84493,#58723,#58724) ;
#50748=AXIS2_PLACEMENT_3D('',#84495,#58725,#58726) ;
#50749=AXIS2_PLACEMENT_3D('',#84496,#58727,#58728) ;
#50750=AXIS2_PLACEMENT_3D('',#84497,#58729,#58730) ;
#50751=AXIS2_PLACEMENT_3D('',#84500,#58731,#58732) ;
#50752=AXIS2_PLACEMENT_3D('',#84501,#58733,#58734) ;
#50753=AXIS2_PLACEMENT_3D('',#84502,#58735,#58736) ;
#50754=AXIS2_PLACEMENT_3D('',#84503,#58737,#58738) ;
#50755=AXIS2_PLACEMENT_3D('',#84505,#58739,#58740) ;
#50756=AXIS2_PLACEMENT_3D('',#84507,#58742,#58743) ;
#50757=AXIS2_PLACEMENT_3D('',#84509,#58744,#58745) ;
#50758=AXIS2_PLACEMENT_3D('',#84510,#58746,#58747) ;
#50759=AXIS2_PLACEMENT_3D('',#84511,#58748,#58749) ;
#50760=AXIS2_PLACEMENT_3D('',#84513,#58750,#58751) ;
#50761=AXIS2_PLACEMENT_3D('',#84515,#58753,#58754) ;
#50762=AXIS2_PLACEMENT_3D('',#84517,#58755,#58756) ;
#50763=AXIS2_PLACEMENT_3D('',#84518,#58757,#58758) ;
#50764=AXIS2_PLACEMENT_3D('',#84519,#58759,#58760) ;
#50765=AXIS2_PLACEMENT_3D('',#84521,#58761,#58762) ;
#50766=AXIS2_PLACEMENT_3D('',#84523,#58764,#58765) ;
#50767=AXIS2_PLACEMENT_3D('',#84525,#58766,#58767) ;
#50768=AXIS2_PLACEMENT_3D('',#84526,#58768,#58769) ;
#50769=AXIS2_PLACEMENT_3D('',#84527,#58770,#58771) ;
#50770=AXIS2_PLACEMENT_3D('',#84529,#58772,#58773) ;
#50771=AXIS2_PLACEMENT_3D('',#84531,#58775,#58776) ;
#50772=AXIS2_PLACEMENT_3D('',#84533,#58777,#58778) ;
#50773=AXIS2_PLACEMENT_3D('',#84534,#58779,#58780) ;
#50774=AXIS2_PLACEMENT_3D('',#84535,#58781,#58782) ;
#50775=AXIS2_PLACEMENT_3D('',#84537,#58784,#58785) ;
#50776=AXIS2_PLACEMENT_3D('',#84539,#58786,#58787) ;
#50777=AXIS2_PLACEMENT_3D('',#84541,#58789,#58790) ;
#50778=AXIS2_PLACEMENT_3D('',#84544,#58791,#58792) ;
#50779=AXIS2_PLACEMENT_3D('',#84567,#58795,#58796) ;
#50780=AXIS2_PLACEMENT_3D('',#84568,#58797,#58798) ;
#50781=AXIS2_PLACEMENT_3D('',#84569,#58799,#58800) ;
#50782=AXIS2_PLACEMENT_3D('',#84572,#58801,#58802) ;
#50783=AXIS2_PLACEMENT_3D('',#84595,#58805,#58806) ;
#50784=AXIS2_PLACEMENT_3D('',#84596,#58807,#58808) ;
#50785=AXIS2_PLACEMENT_3D('',#84597,#58809,#58810) ;
#50786=AXIS2_PLACEMENT_3D('',#84599,#58811,#58812) ;
#50787=AXIS2_PLACEMENT_3D('',#84601,#58814,#58815) ;
#50788=AXIS2_PLACEMENT_3D('',#84605,#58818,#58819) ;
#50789=AXIS2_PLACEMENT_3D('',#84607,#58820,#58821) ;
#50790=AXIS2_PLACEMENT_3D('',#84609,#58822,#58823) ;
#50791=AXIS2_PLACEMENT_3D('',#84610,#58824,#58825) ;
#50792=AXIS2_PLACEMENT_3D('',#84611,#58826,#58827) ;
#50793=AXIS2_PLACEMENT_3D('',#84613,#58828,#58829) ;
#50794=AXIS2_PLACEMENT_3D('',#84615,#58831,#58832) ;
#50795=AXIS2_PLACEMENT_3D('',#84617,#58833,#58834) ;
#50796=AXIS2_PLACEMENT_3D('',#84620,#58836,#58837) ;
#50797=AXIS2_PLACEMENT_3D('',#84621,#58838,#58839) ;
#50798=AXIS2_PLACEMENT_3D('',#84623,#58840,#58841) ;
#50799=AXIS2_PLACEMENT_3D('',#84624,#58842,#58843) ;
#50800=AXIS2_PLACEMENT_3D('',#84625,#58844,#58845) ;
#50801=AXIS2_PLACEMENT_3D('',#84627,#58846,#58847) ;
#50802=AXIS2_PLACEMENT_3D('',#84629,#58849,#58850) ;
#50803=AXIS2_PLACEMENT_3D('',#84631,#58851,#58852) ;
#50804=AXIS2_PLACEMENT_3D('',#84632,#58853,#58854) ;
#50805=AXIS2_PLACEMENT_3D('',#84633,#58855,#58856) ;
#50806=AXIS2_PLACEMENT_3D('',#84635,#58857,#58858) ;
#50807=AXIS2_PLACEMENT_3D('',#84637,#58860,#58861) ;
#50808=AXIS2_PLACEMENT_3D('',#84638,#58862,#58863) ;
#50809=AXIS2_PLACEMENT_3D('',#84639,#58864,#58865) ;
#50810=AXIS2_PLACEMENT_3D('',#84641,#58866,#58867) ;
#50811=AXIS2_PLACEMENT_3D('',#84644,#58869,#58870) ;
#50812=AXIS2_PLACEMENT_3D('',#84645,#58871,#58872) ;
#50813=AXIS2_PLACEMENT_3D('',#84647,#58873,#58874) ;
#50814=AXIS2_PLACEMENT_3D('',#84648,#58875,#58876) ;
#50815=AXIS2_PLACEMENT_3D('',#84649,#58877,#58878) ;
#50816=AXIS2_PLACEMENT_3D('',#84650,#58879,#58880) ;
#50817=AXIS2_PLACEMENT_3D('',#84651,#58881,#58882) ;
#50818=AXIS2_PLACEMENT_3D('',#84657,#58886,#58887) ;
#50819=AXIS2_PLACEMENT_3D('',#84660,#58889,#58890) ;
#50820=AXIS2_PLACEMENT_3D('',#84661,#58891,#58892) ;
#50821=AXIS2_PLACEMENT_3D('',#84665,#58895,#58896) ;
#50822=AXIS2_PLACEMENT_3D('',#84668,#58898,#58899) ;
#50823=AXIS2_PLACEMENT_3D('',#84669,#58900,#58901) ;
#50824=AXIS2_PLACEMENT_3D('',#84673,#58904,#58905) ;
#50825=AXIS2_PLACEMENT_3D('',#84676,#58907,#58908) ;
#50826=AXIS2_PLACEMENT_3D('',#84677,#58909,#58910) ;
#50827=AXIS2_PLACEMENT_3D('',#84681,#58913,#58914) ;
#50828=AXIS2_PLACEMENT_3D('',#84684,#58916,#58917) ;
#50829=AXIS2_PLACEMENT_3D('',#84685,#58918,#58919) ;
#50830=AXIS2_PLACEMENT_3D('',#84689,#58922,#58923) ;
#50831=AXIS2_PLACEMENT_3D('',#84691,#58924,#58925) ;
#50832=AXIS2_PLACEMENT_3D('',#84693,#58926,#58927) ;
#50833=AXIS2_PLACEMENT_3D('',#84694,#58928,#58929) ;
#50834=AXIS2_PLACEMENT_3D('',#84695,#58930,#58931) ;
#50835=AXIS2_PLACEMENT_3D('',#84697,#58932,#58933) ;
#50836=AXIS2_PLACEMENT_3D('',#84699,#58935,#58936) ;
#50837=AXIS2_PLACEMENT_3D('',#84701,#58937,#58938) ;
#50838=AXIS2_PLACEMENT_3D('',#84704,#58940,#58941) ;
#50839=AXIS2_PLACEMENT_3D('',#84705,#58942,#58943) ;
#50840=AXIS2_PLACEMENT_3D('',#84707,#58944,#58945) ;
#50841=AXIS2_PLACEMENT_3D('',#84708,#58946,#58947) ;
#50842=AXIS2_PLACEMENT_3D('',#84709,#58948,#58949) ;
#50843=AXIS2_PLACEMENT_3D('',#84711,#58950,#58951) ;
#50844=AXIS2_PLACEMENT_3D('',#84713,#58953,#58954) ;
#50845=AXIS2_PLACEMENT_3D('',#84715,#58955,#58956) ;
#50846=AXIS2_PLACEMENT_3D('',#84716,#58957,#58958) ;
#50847=AXIS2_PLACEMENT_3D('',#84717,#58959,#58960) ;
#50848=AXIS2_PLACEMENT_3D('',#84719,#58961,#58962) ;
#50849=AXIS2_PLACEMENT_3D('',#84721,#58964,#58965) ;
#50850=AXIS2_PLACEMENT_3D('',#84722,#58966,#58967) ;
#50851=AXIS2_PLACEMENT_3D('',#84723,#58968,#58969) ;
#50852=AXIS2_PLACEMENT_3D('',#84725,#58970,#58971) ;
#50853=AXIS2_PLACEMENT_3D('',#84728,#58973,#58974) ;
#50854=AXIS2_PLACEMENT_3D('',#84729,#58975,#58976) ;
#50855=AXIS2_PLACEMENT_3D('',#84731,#58977,#58978) ;
#50856=AXIS2_PLACEMENT_3D('',#84732,#58979,#58980) ;
#50857=AXIS2_PLACEMENT_3D('',#84733,#58981,#58982) ;
#50858=AXIS2_PLACEMENT_3D('',#84734,#58983,#58984) ;
#50859=AXIS2_PLACEMENT_3D('',#84735,#58985,#58986) ;
#50860=AXIS2_PLACEMENT_3D('',#84741,#58990,#58991) ;
#50861=AXIS2_PLACEMENT_3D('',#84744,#58993,#58994) ;
#50862=AXIS2_PLACEMENT_3D('',#84745,#58995,#58996) ;
#50863=AXIS2_PLACEMENT_3D('',#84749,#58999,#59000) ;
#50864=AXIS2_PLACEMENT_3D('',#84752,#59002,#59003) ;
#50865=AXIS2_PLACEMENT_3D('',#84753,#59004,#59005) ;
#50866=AXIS2_PLACEMENT_3D('',#84757,#59008,#59009) ;
#50867=AXIS2_PLACEMENT_3D('',#84760,#59011,#59012) ;
#50868=AXIS2_PLACEMENT_3D('',#84761,#59013,#59014) ;
#50869=AXIS2_PLACEMENT_3D('',#84765,#59017,#59018) ;
#50870=AXIS2_PLACEMENT_3D('',#84768,#59020,#59021) ;
#50871=AXIS2_PLACEMENT_3D('',#84769,#59022,#59023) ;
#50872=AXIS2_PLACEMENT_3D('',#84773,#59026,#59027) ;
#50873=AXIS2_PLACEMENT_3D('',#84774,#59028,#59029) ;
#50874=AXIS2_PLACEMENT_3D('',#84775,#59030,#59031) ;
#50875=AXIS2_PLACEMENT_3D('',#84777,#59032,#59033) ;
#50876=AXIS2_PLACEMENT_3D('',#84779,#59035,#59036) ;
#50877=AXIS2_PLACEMENT_3D('',#84780,#59037,#59038) ;
#50878=AXIS2_PLACEMENT_3D('',#84782,#59039,#59040) ;
#50879=AXIS2_PLACEMENT_3D('',#84783,#59041,#59042) ;
#50880=AXIS2_PLACEMENT_3D('',#84784,#59043,#59044) ;
#50881=AXIS2_PLACEMENT_3D('',#84785,#59045,#59046) ;
#50882=AXIS2_PLACEMENT_3D('',#84787,#59048,#59049) ;
#50883=AXIS2_PLACEMENT_3D('',#84789,#59051,#59052) ;
#50884=AXIS2_PLACEMENT_3D('',#84791,#59053,#59054) ;
#50885=AXIS2_PLACEMENT_3D('',#84792,#59055,#59056) ;
#50886=AXIS2_PLACEMENT_3D('',#84793,#59057,#59058) ;
#50887=AXIS2_PLACEMENT_3D('',#84794,#59059,#59060) ;
#50888=AXIS2_PLACEMENT_3D('',#84797,#59062,#59063) ;
#50889=AXIS2_PLACEMENT_3D('',#84798,#59064,#59065) ;
#50890=AXIS2_PLACEMENT_3D('',#84800,#59066,#59067) ;
#50891=AXIS2_PLACEMENT_3D('',#84801,#59068,#59069) ;
#50892=AXIS2_PLACEMENT_3D('',#84802,#59070,#59071) ;
#50893=AXIS2_PLACEMENT_3D('',#84804,#59072,#59073) ;
#50894=AXIS2_PLACEMENT_3D('',#84806,#59075,#59076) ;
#50895=AXIS2_PLACEMENT_3D('',#84808,#59077,#59078) ;
#50896=AXIS2_PLACEMENT_3D('',#84809,#59079,#59080) ;
#50897=AXIS2_PLACEMENT_3D('',#84810,#59081,#59082) ;
#50898=AXIS2_PLACEMENT_3D('',#84812,#59083,#59084) ;
#50899=AXIS2_PLACEMENT_3D('',#84814,#59086,#59087) ;
#50900=AXIS2_PLACEMENT_3D('',#84816,#59088,#59089) ;
#50901=AXIS2_PLACEMENT_3D('',#84817,#59090,#59091) ;
#50902=AXIS2_PLACEMENT_3D('',#84818,#59092,#59093) ;
#50903=AXIS2_PLACEMENT_3D('',#84820,#59094,#59095) ;
#50904=AXIS2_PLACEMENT_3D('',#84822,#59097,#59098) ;
#50905=AXIS2_PLACEMENT_3D('',#84824,#59099,#59100) ;
#50906=AXIS2_PLACEMENT_3D('',#84825,#59101,#59102) ;
#50907=AXIS2_PLACEMENT_3D('',#84826,#59103,#59104) ;
#50908=AXIS2_PLACEMENT_3D('',#84828,#59106,#59107) ;
#50909=AXIS2_PLACEMENT_3D('',#84832,#59110,#59111) ;
#50910=AXIS2_PLACEMENT_3D('',#84835,#59113,#59114) ;
#50911=AXIS2_PLACEMENT_3D('',#84836,#59115,#59116) ;
#50912=AXIS2_PLACEMENT_3D('',#84840,#59119,#59120) ;
#50913=AXIS2_PLACEMENT_3D('',#84843,#59122,#59123) ;
#50914=AXIS2_PLACEMENT_3D('',#84844,#59124,#59125) ;
#50915=AXIS2_PLACEMENT_3D('',#84848,#59128,#59129) ;
#50916=AXIS2_PLACEMENT_3D('',#84851,#59131,#59132) ;
#50917=AXIS2_PLACEMENT_3D('',#84852,#59133,#59134) ;
#50918=AXIS2_PLACEMENT_3D('',#84856,#59137,#59138) ;
#50919=AXIS2_PLACEMENT_3D('',#84859,#59140,#59141) ;
#50920=AXIS2_PLACEMENT_3D('',#84860,#59142,#59143) ;
#50921=AXIS2_PLACEMENT_3D('',#84862,#59145,#59146) ;
#50922=AXIS2_PLACEMENT_3D('',#84864,#59148,#59149) ;
#50923=AXIS2_PLACEMENT_3D('',#84866,#59150,#59151) ;
#50924=AXIS2_PLACEMENT_3D('',#84868,#59152,#59153) ;
#50925=AXIS2_PLACEMENT_3D('',#84869,#59154,#59155) ;
#50926=AXIS2_PLACEMENT_3D('',#84870,#59156,#59157) ;
#50927=AXIS2_PLACEMENT_3D('',#84878,#59162,#59163) ;
#50928=AXIS2_PLACEMENT_3D('',#84880,#59164,#59165) ;
#50929=AXIS2_PLACEMENT_3D('',#84881,#59166,#59167) ;
#50930=AXIS2_PLACEMENT_3D('',#84882,#59168,#59169) ;
#50931=AXIS2_PLACEMENT_3D('',#84884,#59171,#59172) ;
#50932=AXIS2_PLACEMENT_3D('',#84885,#59173,#59174) ;
#50933=AXIS2_PLACEMENT_3D('',#84887,#59175,#59176) ;
#50934=AXIS2_PLACEMENT_3D('',#84888,#59177,#59178) ;
#50935=AXIS2_PLACEMENT_3D('',#84889,#59179,#59180) ;
#50936=AXIS2_PLACEMENT_3D('',#84891,#59181,#59182) ;
#50937=AXIS2_PLACEMENT_3D('',#84892,#59183,#59184) ;
#50938=AXIS2_PLACEMENT_3D('',#84893,#59185,#59186) ;
#50939=AXIS2_PLACEMENT_3D('',#84894,#59187,#59188) ;
#50940=AXIS2_PLACEMENT_3D('',#84896,#59190,#59191) ;
#50941=AXIS2_PLACEMENT_3D('',#84898,#59193,#59194) ;
#50942=AXIS2_PLACEMENT_3D('',#84899,#59195,#59196) ;
#50943=AXIS2_PLACEMENT_3D('',#84901,#59197,#59198) ;
#50944=AXIS2_PLACEMENT_3D('',#84902,#59199,#59200) ;
#50945=AXIS2_PLACEMENT_3D('',#84903,#59201,#59202) ;
#50946=AXIS2_PLACEMENT_3D('',#84904,#59203,#59204) ;
#50947=AXIS2_PLACEMENT_3D('',#84905,#59205,#59206) ;
#50948=AXIS2_PLACEMENT_3D('',#84907,#59208,#59209) ;
#50949=AXIS2_PLACEMENT_3D('',#84909,#59211,#59212) ;
#50950=AXIS2_PLACEMENT_3D('',#84911,#59214,#59215) ;
#50951=AXIS2_PLACEMENT_3D('',#84913,#59217,#59218) ;
#50952=AXIS2_PLACEMENT_3D('',#84914,#59219,#59220) ;
#50953=AXIS2_PLACEMENT_3D('',#84916,#59221,#59222) ;
#50954=AXIS2_PLACEMENT_3D('',#84918,#59223,#59224) ;
#50955=AXIS2_PLACEMENT_3D('',#84919,#59225,#59226) ;
#50956=AXIS2_PLACEMENT_3D('',#84920,#59227,#59228) ;
#50957=AXIS2_PLACEMENT_3D('',#84922,#59229,#59230) ;
#50958=AXIS2_PLACEMENT_3D('',#84924,#59231,#59232) ;
#50959=AXIS2_PLACEMENT_3D('',#84925,#59233,#59234) ;
#50960=AXIS2_PLACEMENT_3D('',#84926,#59235,#59236) ;
#50961=AXIS2_PLACEMENT_3D('',#84933,#59241,#59242) ;
#50962=AXIS2_PLACEMENT_3D('',#84934,#59243,#59244) ;
#50963=AXIS2_PLACEMENT_3D('',#84935,#59245,#59246) ;
#50964=AXIS2_PLACEMENT_3D('',#84936,#59247,#59248) ;
#50965=AXIS2_PLACEMENT_3D('',#84937,#59249,#59250) ;
#50966=AXIS2_PLACEMENT_3D('',#84938,#59251,#59252) ;
#50967=AXIS2_PLACEMENT_3D('',#84939,#59253,#59254) ;
#50968=AXIS2_PLACEMENT_3D('',#84940,#59255,#59256) ;
#50969=AXIS2_PLACEMENT_3D('',#84941,#59257,#59258) ;
#50970=AXIS2_PLACEMENT_3D('',#84942,#59259,#59260) ;
#50971=AXIS2_PLACEMENT_3D('',#84943,#59261,#59262) ;
#50972=AXIS2_PLACEMENT_3D('',#84944,#59263,#59264) ;
#50973=AXIS2_PLACEMENT_3D('',#84945,#59265,#59266) ;
#50974=AXIS2_PLACEMENT_3D('',#84946,#59267,#59268) ;
#50975=AXIS2_PLACEMENT_3D('',#84947,#59269,#59270) ;
#50976=AXIS2_PLACEMENT_3D('',#84949,#59271,#59272) ;
#50977=AXIS2_PLACEMENT_3D('',#84950,#59273,#59274) ;
#50978=AXIS2_PLACEMENT_3D('',#84951,#59275,#59276) ;
#50979=AXIS2_PLACEMENT_3D('',#84952,#59277,#59278) ;
#50980=AXIS2_PLACEMENT_3D('',#84953,#59279,#59280) ;
#50981=AXIS2_PLACEMENT_3D('',#84955,#59281,#59282) ;
#50982=AXIS2_PLACEMENT_3D('',#84956,#59283,#59284) ;
#50983=AXIS2_PLACEMENT_3D('',#84957,#59285,#59286) ;
#50984=AXIS2_PLACEMENT_3D('',#84958,#59287,#59288) ;
#50985=AXIS2_PLACEMENT_3D('',#84960,#59290,#59291) ;
#50986=AXIS2_PLACEMENT_3D('',#84961,#59292,#59293) ;
#50987=AXIS2_PLACEMENT_3D('',#84963,#59294,#59295) ;
#50988=AXIS2_PLACEMENT_3D('',#84964,#59296,#59297) ;
#50989=AXIS2_PLACEMENT_3D('',#84965,#59298,#59299) ;
#50990=AXIS2_PLACEMENT_3D('',#84967,#59300,#59301) ;
#50991=AXIS2_PLACEMENT_3D('',#84968,#59302,#59303) ;
#50992=AXIS2_PLACEMENT_3D('',#84969,#59304,#59305) ;
#50993=AXIS2_PLACEMENT_3D('',#84970,#59306,#59307) ;
#50994=AXIS2_PLACEMENT_3D('',#84972,#59309,#59310) ;
#50995=AXIS2_PLACEMENT_3D('',#84974,#59312,#59313) ;
#50996=AXIS2_PLACEMENT_3D('',#84975,#59314,#59315) ;
#50997=AXIS2_PLACEMENT_3D('',#84977,#59317,#59318) ;
#50998=AXIS2_PLACEMENT_3D('',#84979,#59320,#59321) ;
#50999=AXIS2_PLACEMENT_3D('',#84981,#59323,#59324) ;
#51000=AXIS2_PLACEMENT_3D('',#84982,#59325,#59326) ;
#51001=AXIS2_PLACEMENT_3D('',#84983,#59327,#59328) ;
#51002=AXIS2_PLACEMENT_3D('',#84984,#59329,#59330) ;
#51003=AXIS2_PLACEMENT_3D('',#84986,#59332,#59333) ;
#51004=AXIS2_PLACEMENT_3D('',#84987,#59334,#59335) ;
#51005=AXIS2_PLACEMENT_3D('',#84989,#59336,#59337) ;
#51006=AXIS2_PLACEMENT_3D('',#84991,#59338,#59339) ;
#51007=AXIS2_PLACEMENT_3D('',#84992,#59340,#59341) ;
#51008=AXIS2_PLACEMENT_3D('',#84993,#59342,#59343) ;
#51009=AXIS2_PLACEMENT_3D('',#84995,#59344,#59345) ;
#51010=AXIS2_PLACEMENT_3D('',#84997,#59346,#59347) ;
#51011=AXIS2_PLACEMENT_3D('',#84998,#59348,#59349) ;
#51012=AXIS2_PLACEMENT_3D('',#84999,#59350,#59351) ;
#51013=AXIS2_PLACEMENT_3D('',#85006,#59356,#59357) ;
#51014=AXIS2_PLACEMENT_3D('',#85007,#59358,#59359) ;
#51015=AXIS2_PLACEMENT_3D('',#85008,#59360,#59361) ;
#51016=AXIS2_PLACEMENT_3D('',#85009,#59362,#59363) ;
#51017=AXIS2_PLACEMENT_3D('',#85010,#59364,#59365) ;
#51018=AXIS2_PLACEMENT_3D('',#85011,#59366,#59367) ;
#51019=AXIS2_PLACEMENT_3D('',#85012,#59368,#59369) ;
#51020=AXIS2_PLACEMENT_3D('',#85013,#59370,#59371) ;
#51021=AXIS2_PLACEMENT_3D('',#85014,#59372,#59373) ;
#51022=AXIS2_PLACEMENT_3D('',#85015,#59374,#59375) ;
#51023=AXIS2_PLACEMENT_3D('',#85016,#59376,#59377) ;
#51024=AXIS2_PLACEMENT_3D('',#85017,#59378,#59379) ;
#51025=AXIS2_PLACEMENT_3D('',#85019,#59380,#59381) ;
#51026=AXIS2_PLACEMENT_3D('',#85020,#59382,#59383) ;
#51027=AXIS2_PLACEMENT_3D('',#85021,#59384,#59385) ;
#51028=AXIS2_PLACEMENT_3D('',#85022,#59386,#59387) ;
#51029=AXIS2_PLACEMENT_3D('',#85023,#59388,#59389) ;
#51030=AXIS2_PLACEMENT_3D('',#85024,#59390,#59391) ;
#51031=AXIS2_PLACEMENT_3D('',#85025,#59392,#59393) ;
#51032=AXIS2_PLACEMENT_3D('',#85026,#59394,#59395) ;
#51033=AXIS2_PLACEMENT_3D('',#85027,#59396,#59397) ;
#51034=AXIS2_PLACEMENT_3D('',#85029,#59398,#59399) ;
#51035=AXIS2_PLACEMENT_3D('',#85030,#59400,#59401) ;
#51036=AXIS2_PLACEMENT_3D('',#85031,#59402,#59403) ;
#51037=AXIS2_PLACEMENT_3D('',#85032,#59404,#59405) ;
#51038=AXIS2_PLACEMENT_3D('',#85034,#59406,#59407) ;
#51039=AXIS2_PLACEMENT_3D('',#85035,#59408,#59409) ;
#51040=AXIS2_PLACEMENT_3D('',#85036,#59410,#59411) ;
#51041=AXIS2_PLACEMENT_3D('',#85037,#59412,#59413) ;
#51042=AXIS2_PLACEMENT_3D('',#85039,#59415,#59416) ;
#51043=AXIS2_PLACEMENT_3D('',#85041,#59417,#59418) ;
#51044=AXIS2_PLACEMENT_3D('',#85042,#59419,#59420) ;
#51045=AXIS2_PLACEMENT_3D('',#85043,#59421,#59422) ;
#51046=AXIS2_PLACEMENT_3D('',#85044,#59423,#59424) ;
#51047=AXIS2_PLACEMENT_3D('',#85046,#59426,#59427) ;
#51048=AXIS2_PLACEMENT_3D('',#85048,#59429,#59430) ;
#51049=AXIS2_PLACEMENT_3D('',#85049,#59431,#59432) ;
#51050=AXIS2_PLACEMENT_3D('',#85051,#59434,#59435) ;
#51051=AXIS2_PLACEMENT_3D('',#85053,#59437,#59438) ;
#51052=AXIS2_PLACEMENT_3D('',#85055,#59440,#59441) ;
#51053=AXIS2_PLACEMENT_3D('',#85056,#59442,#59443) ;
#51054=AXIS2_PLACEMENT_3D('',#85057,#59444,#59445) ;
#51055=AXIS2_PLACEMENT_3D('',#85059,#59447,#59448) ;
#51056=AXIS2_PLACEMENT_3D('',#85060,#59449,#59450) ;
#51057=AXIS2_PLACEMENT_3D('',#85062,#59451,#59452) ;
#51058=AXIS2_PLACEMENT_3D('',#85064,#59453,#59454) ;
#51059=AXIS2_PLACEMENT_3D('',#85065,#59455,#59456) ;
#51060=AXIS2_PLACEMENT_3D('',#85066,#59457,#59458) ;
#51061=AXIS2_PLACEMENT_3D('',#85068,#59459,#59460) ;
#51062=AXIS2_PLACEMENT_3D('',#85070,#59461,#59462) ;
#51063=AXIS2_PLACEMENT_3D('',#85071,#59463,#59464) ;
#51064=AXIS2_PLACEMENT_3D('',#85072,#59465,#59466) ;
#51065=AXIS2_PLACEMENT_3D('',#85073,#59467,#59468) ;
#51066=AXIS2_PLACEMENT_3D('',#85074,#59469,#59470) ;
#51067=AXIS2_PLACEMENT_3D('',#85075,#59471,#59472) ;
#51068=AXIS2_PLACEMENT_3D('',#85076,#59473,#59474) ;
#51069=AXIS2_PLACEMENT_3D('',#85077,#59475,#59476) ;
#51070=AXIS2_PLACEMENT_3D('',#85078,#59477,#59478) ;
#51071=AXIS2_PLACEMENT_3D('',#85079,#59479,#59480) ;
#51072=AXIS2_PLACEMENT_3D('',#85080,#59481,#59482) ;
#51073=AXIS2_PLACEMENT_3D('',#85082,#59483,#59484) ;
#51074=AXIS2_PLACEMENT_3D('',#85083,#59485,#59486) ;
#51075=AXIS2_PLACEMENT_3D('',#85084,#59487,#59488) ;
#51076=AXIS2_PLACEMENT_3D('',#85086,#59489,#59490) ;
#51077=AXIS2_PLACEMENT_3D('',#85088,#59492,#59493) ;
#51078=AXIS2_PLACEMENT_3D('',#85090,#59494,#59495) ;
#51079=AXIS2_PLACEMENT_3D('',#85091,#59496,#59497) ;
#51080=AXIS2_PLACEMENT_3D('',#85092,#59498,#59499) ;
#51081=AXIS2_PLACEMENT_3D('',#85094,#59501,#59502) ;
#51082=AXIS2_PLACEMENT_3D('',#85095,#59503,#59504) ;
#51083=AXIS2_PLACEMENT_3D('',#85096,#59505,#59506) ;
#51084=AXIS2_PLACEMENT_3D('',#85097,#59507,#59508) ;
#51085=AXIS2_PLACEMENT_3D('',#85098,#59509,#59510) ;
#51086=AXIS2_PLACEMENT_3D('',#85099,#59511,#59512) ;
#51087=AXIS2_PLACEMENT_3D('',#85100,#59513,#59514) ;
#51088=AXIS2_PLACEMENT_3D('',#85101,#59515,#59516) ;
#51089=AXIS2_PLACEMENT_3D('',#85102,#59517,#59518) ;
#51090=AXIS2_PLACEMENT_3D('',#85103,#59519,#59520) ;
#51091=AXIS2_PLACEMENT_3D('',#85104,#59521,#59522) ;
#51092=AXIS2_PLACEMENT_3D('',#85106,#59523,#59524) ;
#51093=AXIS2_PLACEMENT_3D('',#85107,#59525,#59526) ;
#51094=AXIS2_PLACEMENT_3D('',#85108,#59527,#59528) ;
#51095=AXIS2_PLACEMENT_3D('',#85110,#59529,#59530) ;
#51096=AXIS2_PLACEMENT_3D('',#85112,#59532,#59533) ;
#51097=AXIS2_PLACEMENT_3D('',#85114,#59534,#59535) ;
#51098=AXIS2_PLACEMENT_3D('',#85115,#59536,#59537) ;
#51099=AXIS2_PLACEMENT_3D('',#85116,#59538,#59539) ;
#51100=AXIS2_PLACEMENT_3D('',#85118,#59540,#59541) ;
#51101=AXIS2_PLACEMENT_3D('',#85120,#59543,#59544) ;
#51102=AXIS2_PLACEMENT_3D('',#85122,#59545,#59546) ;
#51103=AXIS2_PLACEMENT_3D('',#85123,#59547,#59548) ;
#51104=AXIS2_PLACEMENT_3D('',#85124,#59549,#59550) ;
#51105=AXIS2_PLACEMENT_3D('',#85126,#59551,#59552) ;
#51106=AXIS2_PLACEMENT_3D('',#85127,#59553,#59554) ;
#51107=AXIS2_PLACEMENT_3D('',#85128,#59555,#59556) ;
#51108=AXIS2_PLACEMENT_3D('',#85130,#59557,#59558) ;
#51109=AXIS2_PLACEMENT_3D('',#85132,#59560,#59561) ;
#51110=AXIS2_PLACEMENT_3D('',#85134,#59562,#59563) ;
#51111=AXIS2_PLACEMENT_3D('',#85135,#59564,#59565) ;
#51112=AXIS2_PLACEMENT_3D('',#85136,#59566,#59567) ;
#51113=AXIS2_PLACEMENT_3D('',#85138,#59568,#59569) ;
#51114=AXIS2_PLACEMENT_3D('',#85139,#59570,#59571) ;
#51115=AXIS2_PLACEMENT_3D('',#85140,#59572,#59573) ;
#51116=AXIS2_PLACEMENT_3D('',#85142,#59574,#59575) ;
#51117=AXIS2_PLACEMENT_3D('',#85144,#59577,#59578) ;
#51118=AXIS2_PLACEMENT_3D('',#85146,#59579,#59580) ;
#51119=AXIS2_PLACEMENT_3D('',#85147,#59581,#59582) ;
#51120=AXIS2_PLACEMENT_3D('',#85148,#59583,#59584) ;
#51121=AXIS2_PLACEMENT_3D('',#85150,#59585,#59586) ;
#51122=AXIS2_PLACEMENT_3D('',#85152,#59588,#59589) ;
#51123=AXIS2_PLACEMENT_3D('',#85154,#59590,#59591) ;
#51124=AXIS2_PLACEMENT_3D('',#85155,#59592,#59593) ;
#51125=AXIS2_PLACEMENT_3D('',#85156,#59594,#59595) ;
#51126=AXIS2_PLACEMENT_3D('',#85158,#59596,#59597) ;
#51127=AXIS2_PLACEMENT_3D('',#85160,#59599,#59600) ;
#51128=AXIS2_PLACEMENT_3D('',#85162,#59601,#59602) ;
#51129=AXIS2_PLACEMENT_3D('',#85163,#59603,#59604) ;
#51130=AXIS2_PLACEMENT_3D('',#85164,#59605,#59606) ;
#51131=AXIS2_PLACEMENT_3D('',#85166,#59607,#59608) ;
#51132=AXIS2_PLACEMENT_3D('',#85168,#59610,#59611) ;
#51133=AXIS2_PLACEMENT_3D('',#85170,#59612,#59613) ;
#51134=AXIS2_PLACEMENT_3D('',#85171,#59614,#59615) ;
#51135=AXIS2_PLACEMENT_3D('',#85172,#59616,#59617) ;
#51136=AXIS2_PLACEMENT_3D('',#85174,#59618,#59619) ;
#51137=AXIS2_PLACEMENT_3D('',#85176,#59621,#59622) ;
#51138=AXIS2_PLACEMENT_3D('',#85178,#59623,#59624) ;
#51139=AXIS2_PLACEMENT_3D('',#85179,#59625,#59626) ;
#51140=AXIS2_PLACEMENT_3D('',#85180,#59627,#59628) ;
#51141=AXIS2_PLACEMENT_3D('',#85182,#59629,#59630) ;
#51142=AXIS2_PLACEMENT_3D('',#85184,#59632,#59633) ;
#51143=AXIS2_PLACEMENT_3D('',#85186,#59634,#59635) ;
#51144=AXIS2_PLACEMENT_3D('',#85187,#59636,#59637) ;
#51145=AXIS2_PLACEMENT_3D('',#85188,#59638,#59639) ;
#51146=AXIS2_PLACEMENT_3D('',#85190,#59640,#59641) ;
#51147=AXIS2_PLACEMENT_3D('',#85192,#59643,#59644) ;
#51148=AXIS2_PLACEMENT_3D('',#85194,#59645,#59646) ;
#51149=AXIS2_PLACEMENT_3D('',#85195,#59647,#59648) ;
#51150=AXIS2_PLACEMENT_3D('',#85196,#59649,#59650) ;
#51151=AXIS2_PLACEMENT_3D('',#85198,#59652,#59653) ;
#51152=AXIS2_PLACEMENT_3D('',#85201,#59654,#59655) ;
#51153=AXIS2_PLACEMENT_3D('',#85202,#59656,#59657) ;
#51154=AXIS2_PLACEMENT_3D('',#85203,#59658,#59659) ;
#51155=AXIS2_PLACEMENT_3D('',#85204,#59660,#59661) ;
#51156=AXIS2_PLACEMENT_3D('',#85207,#59664,#59665) ;
#51157=AXIS2_PLACEMENT_3D('',#85209,#59667,#59668) ;
#51158=AXIS2_PLACEMENT_3D('',#85212,#59669,#59670) ;
#51159=AXIS2_PLACEMENT_3D('',#85215,#59673,#59674) ;
#51160=AXIS2_PLACEMENT_3D('',#85216,#59675,#59676) ;
#51161=AXIS2_PLACEMENT_3D('',#85217,#59677,#59678) ;
#51162=AXIS2_PLACEMENT_3D('',#85218,#59679,#59680) ;
#51163=AXIS2_PLACEMENT_3D('',#85220,#59681,#59682) ;
#51164=AXIS2_PLACEMENT_3D('',#85221,#59683,#59684) ;
#51165=AXIS2_PLACEMENT_3D('',#85222,#59685,#59686) ;
#51166=AXIS2_PLACEMENT_3D('',#85228,#59690,#59691) ;
#51167=AXIS2_PLACEMENT_3D('',#85231,#59693,#59694) ;
#51168=AXIS2_PLACEMENT_3D('',#85232,#59695,#59696) ;
#51169=AXIS2_PLACEMENT_3D('',#85236,#59699,#59700) ;
#51170=AXIS2_PLACEMENT_3D('',#85239,#59702,#59703) ;
#51171=AXIS2_PLACEMENT_3D('',#85240,#59704,#59705) ;
#51172=AXIS2_PLACEMENT_3D('',#85243,#59707,#59708) ;
#51173=AXIS2_PLACEMENT_3D('',#85244,#59709,#59710) ;
#51174=AXIS2_PLACEMENT_3D('',#85248,#59713,#59714) ;
#51175=AXIS2_PLACEMENT_3D('',#85251,#59716,#59717) ;
#51176=AXIS2_PLACEMENT_3D('',#85252,#59718,#59719) ;
#51177=AXIS2_PLACEMENT_3D('',#85255,#59721,#59722) ;
#51178=AXIS2_PLACEMENT_3D('',#85256,#59723,#59724) ;
#51179=AXIS2_PLACEMENT_3D('',#85260,#59727,#59728) ;
#51180=AXIS2_PLACEMENT_3D('',#85263,#59730,#59731) ;
#51181=AXIS2_PLACEMENT_3D('',#85264,#59732,#59733) ;
#51182=AXIS2_PLACEMENT_3D('',#85268,#59736,#59737) ;
#51183=AXIS2_PLACEMENT_3D('',#85271,#59739,#59740) ;
#51184=AXIS2_PLACEMENT_3D('',#85272,#59741,#59742) ;
#51185=AXIS2_PLACEMENT_3D('',#85276,#59745,#59746) ;
#51186=AXIS2_PLACEMENT_3D('',#85279,#59748,#59749) ;
#51187=AXIS2_PLACEMENT_3D('',#85280,#59750,#59751) ;
#51188=AXIS2_PLACEMENT_3D('',#85284,#59754,#59755) ;
#51189=AXIS2_PLACEMENT_3D('',#85287,#59757,#59758) ;
#51190=AXIS2_PLACEMENT_3D('',#85288,#59759,#59760) ;
#51191=AXIS2_PLACEMENT_3D('',#85292,#59763,#59764) ;
#51192=AXIS2_PLACEMENT_3D('',#85295,#59766,#59767) ;
#51193=AXIS2_PLACEMENT_3D('',#85296,#59768,#59769) ;
#51194=AXIS2_PLACEMENT_3D('',#85300,#59772,#59773) ;
#51195=AXIS2_PLACEMENT_3D('',#85303,#59775,#59776) ;
#51196=AXIS2_PLACEMENT_3D('',#85304,#59777,#59778) ;
#51197=AXIS2_PLACEMENT_3D('',#85308,#59781,#59782) ;
#51198=AXIS2_PLACEMENT_3D('',#85311,#59784,#59785) ;
#51199=AXIS2_PLACEMENT_3D('',#85312,#59786,#59787) ;
#51200=AXIS2_PLACEMENT_3D('',#85314,#59789,#59790) ;
#51201=AXIS2_PLACEMENT_3D('',#85315,#59791,#59792) ;
#51202=AXIS2_PLACEMENT_3D('',#85316,#59793,#59794) ;
#51203=AXIS2_PLACEMENT_3D('',#85319,#59795,#59796) ;
#51204=AXIS2_PLACEMENT_3D('',#85323,#59798,#59799) ;
#51205=AXIS2_PLACEMENT_3D('',#85325,#59801,#59802) ;
#51206=AXIS2_PLACEMENT_3D('',#85327,#59803,#59804) ;
#51207=AXIS2_PLACEMENT_3D('',#85328,#59805,#59806) ;
#51208=AXIS2_PLACEMENT_3D('',#85329,#59807,#59808) ;
#51209=AXIS2_PLACEMENT_3D('',#85330,#59809,#59810) ;
#51210=AXIS2_PLACEMENT_3D('',#85331,#59811,#59812) ;
#51211=AXIS2_PLACEMENT_3D('',#85332,#59813,#59814) ;
#51212=AXIS2_PLACEMENT_3D('',#85335,#59816,#59817) ;
#51213=AXIS2_PLACEMENT_3D('',#85336,#59818,#59819) ;
#51214=AXIS2_PLACEMENT_3D('',#85340,#59822,#59823) ;
#51215=AXIS2_PLACEMENT_3D('',#85347,#59827,#59828) ;
#51216=AXIS2_PLACEMENT_3D('',#85348,#59829,#59830) ;
#51217=AXIS2_PLACEMENT_3D('',#85351,#59832,#59833) ;
#51218=AXIS2_PLACEMENT_3D('',#85352,#59834,#59835) ;
#51219=AXIS2_PLACEMENT_3D('',#85354,#59836,#59837) ;
#51220=AXIS2_PLACEMENT_3D('',#85355,#59838,#59839) ;
#51221=AXIS2_PLACEMENT_3D('',#85356,#59840,#59841) ;
#51222=AXIS2_PLACEMENT_3D('',#85357,#59842,#59843) ;
#51223=AXIS2_PLACEMENT_3D('',#85358,#59844,#59845) ;
#51224=AXIS2_PLACEMENT_3D('',#85361,#59848,#59849) ;
#51225=AXIS2_PLACEMENT_3D('',#85363,#59850,#59851) ;
#51226=AXIS2_PLACEMENT_3D('',#85365,#59852,#59853) ;
#51227=AXIS2_PLACEMENT_3D('',#85366,#59854,#59855) ;
#51228=AXIS2_PLACEMENT_3D('',#85367,#59856,#59857) ;
#51229=AXIS2_PLACEMENT_3D('',#85370,#59858,#59859) ;
#51230=AXIS2_PLACEMENT_3D('',#85371,#59860,#59861) ;
#51231=AXIS2_PLACEMENT_3D('',#85372,#59862,#59863) ;
#51232=AXIS2_PLACEMENT_3D('',#85373,#59864,#59865) ;
#51233=AXIS2_PLACEMENT_3D('',#85375,#59867,#59868) ;
#51234=AXIS2_PLACEMENT_3D('',#85378,#59869,#59870) ;
#51235=AXIS2_PLACEMENT_3D('',#85379,#59871,#59872) ;
#51236=AXIS2_PLACEMENT_3D('',#85380,#59873,#59874) ;
#51237=AXIS2_PLACEMENT_3D('',#85381,#59875,#59876) ;
#51238=AXIS2_PLACEMENT_3D('',#85383,#59878,#59879) ;
#51239=AXIS2_PLACEMENT_3D('',#85386,#59880,#59881) ;
#51240=AXIS2_PLACEMENT_3D('',#85387,#59882,#59883) ;
#51241=AXIS2_PLACEMENT_3D('',#85388,#59884,#59885) ;
#51242=AXIS2_PLACEMENT_3D('',#85389,#59886,#59887) ;
#51243=AXIS2_PLACEMENT_3D('',#85391,#59889,#59890) ;
#51244=AXIS2_PLACEMENT_3D('',#85394,#59891,#59892) ;
#51245=AXIS2_PLACEMENT_3D('',#85395,#59893,#59894) ;
#51246=AXIS2_PLACEMENT_3D('',#85396,#59895,#59896) ;
#51247=AXIS2_PLACEMENT_3D('',#85397,#59897,#59898) ;
#51248=AXIS2_PLACEMENT_3D('',#85399,#59900,#59901) ;
#51249=AXIS2_PLACEMENT_3D('',#85401,#59902,#59903) ;
#51250=AXIS2_PLACEMENT_3D('',#85403,#59904,#59905) ;
#51251=AXIS2_PLACEMENT_3D('',#85404,#59906,#59907) ;
#51252=AXIS2_PLACEMENT_3D('',#85405,#59908,#59909) ;
#51253=AXIS2_PLACEMENT_3D('',#85407,#59911,#59912) ;
#51254=AXIS2_PLACEMENT_3D('',#85410,#59915,#59916) ;
#51255=AXIS2_PLACEMENT_3D('',#85412,#59918,#59919) ;
#51256=AXIS2_PLACEMENT_3D('',#85415,#59922,#59923) ;
#51257=AXIS2_PLACEMENT_3D('',#85418,#59926,#59927) ;
#51258=AXIS2_PLACEMENT_3D('',#85421,#59930,#59931) ;
#51259=AXIS2_PLACEMENT_3D('',#85424,#59934,#59935) ;
#51260=AXIS2_PLACEMENT_3D('',#85427,#59938,#59939) ;
#51261=AXIS2_PLACEMENT_3D('',#85429,#59941,#59942) ;
#51262=AXIS2_PLACEMENT_3D('',#85430,#59943,#59944) ;
#51263=AXIS2_PLACEMENT_3D('',#85431,#59945,#59946) ;
#51264=AXIS2_PLACEMENT_3D('',#85433,#59947,#59948) ;
#51265=AXIS2_PLACEMENT_3D('',#85435,#59949,#59950) ;
#51266=AXIS2_PLACEMENT_3D('',#85436,#59951,#59952) ;
#51267=AXIS2_PLACEMENT_3D('',#85437,#59953,#59954) ;
#51268=AXIS2_PLACEMENT_3D('',#85439,#59955,#59956) ;
#51269=AXIS2_PLACEMENT_3D('',#85441,#59957,#59958) ;
#51270=AXIS2_PLACEMENT_3D('',#85442,#59959,#59960) ;
#51271=AXIS2_PLACEMENT_3D('',#85443,#59961,#59962) ;
#51272=AXIS2_PLACEMENT_3D('',#85445,#59964,#59965) ;
#51273=AXIS2_PLACEMENT_3D('',#85448,#59968,#59969) ;
#51274=AXIS2_PLACEMENT_3D('',#85450,#59970,#59971) ;
#51275=AXIS2_PLACEMENT_3D('',#85452,#59972,#59973) ;
#51276=AXIS2_PLACEMENT_3D('',#85453,#59974,#59975) ;
#51277=AXIS2_PLACEMENT_3D('',#85454,#59976,#59977) ;
#51278=AXIS2_PLACEMENT_3D('',#85455,#59978,#59979) ;
#51279=AXIS2_PLACEMENT_3D('',#85456,#59980,#59981) ;
#51280=AXIS2_PLACEMENT_3D('',#85457,#59982,#59983) ;
#51281=AXIS2_PLACEMENT_3D('',#85459,#59985,#59986) ;
#51282=AXIS2_PLACEMENT_3D('',#85461,#59987,#59988) ;
#51283=AXIS2_PLACEMENT_3D('',#85462,#59989,#59990) ;
#51284=AXIS2_PLACEMENT_3D('',#85463,#59991,#59992) ;
#51285=AXIS2_PLACEMENT_3D('',#85464,#59993,#59994) ;
#51286=AXIS2_PLACEMENT_3D('',#85466,#59996,#59997) ;
#51287=AXIS2_PLACEMENT_3D('',#85467,#59998,#59999) ;
#51288=AXIS2_PLACEMENT_3D('',#85468,#60000,#60001) ;
#51289=AXIS2_PLACEMENT_3D('',#85469,#60002,#60003) ;
#51290=AXIS2_PLACEMENT_3D('',#85470,#60004,#60005) ;
#51291=AXIS2_PLACEMENT_3D('',#85471,#60006,#60007) ;
#51292=AXIS2_PLACEMENT_3D('',#85472,#60008,#60009) ;
#51293=AXIS2_PLACEMENT_3D('',#85473,#60010,#60011) ;
#51294=AXIS2_PLACEMENT_3D('',#85474,#60012,#60013) ;
#51295=AXIS2_PLACEMENT_3D('',#85475,#60014,#60015) ;
#51296=AXIS2_PLACEMENT_3D('',#85476,#60016,#60017) ;
#51297=AXIS2_PLACEMENT_3D('',#85477,#60018,#60019) ;
#51298=AXIS2_PLACEMENT_3D('',#85478,#60020,#60021) ;
#51299=AXIS2_PLACEMENT_3D('',#85479,#60022,#60023) ;
#51300=AXIS2_PLACEMENT_3D('',#85481,#60025,#60026) ;
#51301=AXIS2_PLACEMENT_3D('',#85484,#60029,#60030) ;
#51302=AXIS2_PLACEMENT_3D('',#85486,#60032,#60033) ;
#51303=AXIS2_PLACEMENT_3D('',#85489,#60036,#60037) ;
#51304=AXIS2_PLACEMENT_3D('',#85490,#60038,#60039) ;
#51305=AXIS2_PLACEMENT_3D('',#85491,#60040,#60041) ;
#51306=AXIS2_PLACEMENT_3D('',#85494,#60042,#60043) ;
#51307=AXIS2_PLACEMENT_3D('',#85498,#60045,#60046) ;
#51308=AXIS2_PLACEMENT_3D('',#85500,#60048,#60049) ;
#51309=AXIS2_PLACEMENT_3D('',#85501,#60050,#60051) ;
#51310=AXIS2_PLACEMENT_3D('',#85502,#60052,#60053) ;
#51311=AXIS2_PLACEMENT_3D('',#85503,#60054,#60055) ;
#51312=AXIS2_PLACEMENT_3D('',#85504,#60056,#60057) ;
#51313=AXIS2_PLACEMENT_3D('',#85505,#60058,#60059) ;
#51314=AXIS2_PLACEMENT_3D('',#85509,#60062,#60063) ;
#51315=AXIS2_PLACEMENT_3D('',#85512,#60064,#60065) ;
#51316=AXIS2_PLACEMENT_3D('',#85516,#60067,#60068) ;
#51317=AXIS2_PLACEMENT_3D('',#85518,#60070,#60071) ;
#51318=AXIS2_PLACEMENT_3D('',#85519,#60072,#60073) ;
#51319=AXIS2_PLACEMENT_3D('',#85520,#60074,#60075) ;
#51320=AXIS2_PLACEMENT_3D('',#85521,#60076,#60077) ;
#51321=AXIS2_PLACEMENT_3D('',#85522,#60078,#60079) ;
#51322=AXIS2_PLACEMENT_3D('',#85523,#60080,#60081) ;
#51323=AXIS2_PLACEMENT_3D('',#85525,#60083,#60084) ;
#51324=AXIS2_PLACEMENT_3D('',#85527,#60086,#60087) ;
#51325=AXIS2_PLACEMENT_3D('',#85528,#60088,#60089) ;
#51326=AXIS2_PLACEMENT_3D('',#85529,#60090,#60091) ;
#51327=AXIS2_PLACEMENT_3D('',#85530,#60092,#60093) ;
#51328=AXIS2_PLACEMENT_3D('',#85531,#60094,#60095) ;
#51329=AXIS2_PLACEMENT_3D('',#85532,#60096,#60097) ;
#51330=AXIS2_PLACEMENT_3D('',#85533,#60098,#60099) ;
#51331=AXIS2_PLACEMENT_3D('',#85534,#60100,#60101) ;
#51332=AXIS2_PLACEMENT_3D('',#85535,#60102,#60103) ;
#51333=AXIS2_PLACEMENT_3D('',#85536,#60104,#60105) ;
#51334=AXIS2_PLACEMENT_3D('',#85537,#60106,#60107) ;
#51335=AXIS2_PLACEMENT_3D('',#85538,#60108,#60109) ;
#51336=AXIS2_PLACEMENT_3D('',#85539,#60110,#60111) ;
#51337=AXIS2_PLACEMENT_3D('',#85540,#60112,#60113) ;
#51338=AXIS2_PLACEMENT_3D('',#85541,#60114,#60115) ;
#51339=AXIS2_PLACEMENT_3D('',#85542,#60116,#60117) ;
#51340=AXIS2_PLACEMENT_3D('',#85543,#60118,#60119) ;
#51341=AXIS2_PLACEMENT_3D('',#85544,#60120,#60121) ;
#51342=AXIS2_PLACEMENT_3D('',#85547,#60122,#60123) ;
#51343=AXIS2_PLACEMENT_3D('',#85551,#60125,#60126) ;
#51344=AXIS2_PLACEMENT_3D('',#85553,#60128,#60129) ;
#51345=AXIS2_PLACEMENT_3D('',#85554,#60130,#60131) ;
#51346=AXIS2_PLACEMENT_3D('',#85555,#60132,#60133) ;
#51347=AXIS2_PLACEMENT_3D('',#85556,#60134,#60135) ;
#51348=AXIS2_PLACEMENT_3D('',#85557,#60136,#60137) ;
#51349=AXIS2_PLACEMENT_3D('',#85558,#60138,#60139) ;
#51350=AXIS2_PLACEMENT_3D('',#85559,#60140,#60141) ;
#51351=AXIS2_PLACEMENT_3D('',#85562,#60143,#60144) ;
#51352=AXIS2_PLACEMENT_3D('',#85563,#60145,#60146) ;
#51353=AXIS2_PLACEMENT_3D('',#85567,#60149,#60150) ;
#51354=AXIS2_PLACEMENT_3D('',#85574,#60154,#60155) ;
#51355=AXIS2_PLACEMENT_3D('',#85575,#60156,#60157) ;
#51356=AXIS2_PLACEMENT_3D('',#85578,#60159,#60160) ;
#51357=AXIS2_PLACEMENT_3D('',#85579,#60161,#60162) ;
#51358=AXIS2_PLACEMENT_3D('',#85581,#60163,#60164) ;
#51359=AXIS2_PLACEMENT_3D('',#85582,#60165,#60166) ;
#51360=AXIS2_PLACEMENT_3D('',#85583,#60167,#60168) ;
#51361=AXIS2_PLACEMENT_3D('',#85584,#60169,#60170) ;
#51362=AXIS2_PLACEMENT_3D('',#85585,#60171,#60172) ;
#51363=AXIS2_PLACEMENT_3D('',#85588,#60175,#60176) ;
#51364=AXIS2_PLACEMENT_3D('',#85591,#60177,#60178) ;
#51365=AXIS2_PLACEMENT_3D('',#85592,#60179,#60180) ;
#51366=AXIS2_PLACEMENT_3D('',#85593,#60181,#60182) ;
#51367=AXIS2_PLACEMENT_3D('',#85594,#60183,#60184) ;
#51368=AXIS2_PLACEMENT_3D('',#85597,#60185,#60186) ;
#51369=AXIS2_PLACEMENT_3D('',#85598,#60187,#60188) ;
#51370=AXIS2_PLACEMENT_3D('',#85599,#60189,#60190) ;
#51371=AXIS2_PLACEMENT_3D('',#85600,#60191,#60192) ;
#51372=AXIS2_PLACEMENT_3D('',#85603,#60193,#60194) ;
#51373=AXIS2_PLACEMENT_3D('',#85604,#60195,#60196) ;
#51374=AXIS2_PLACEMENT_3D('',#85605,#60197,#60198) ;
#51375=AXIS2_PLACEMENT_3D('',#85606,#60199,#60200) ;
#51376=AXIS2_PLACEMENT_3D('',#85609,#60201,#60202) ;
#51377=AXIS2_PLACEMENT_3D('',#85610,#60203,#60204) ;
#51378=AXIS2_PLACEMENT_3D('',#85611,#60205,#60206) ;
#51379=AXIS2_PLACEMENT_3D('',#85612,#60207,#60208) ;
#51380=AXIS2_PLACEMENT_3D('',#85614,#60210,#60211) ;
#51381=AXIS2_PLACEMENT_3D('',#85615,#60212,#60213) ;
#51382=AXIS2_PLACEMENT_3D('',#85617,#60215,#60216) ;
#51383=AXIS2_PLACEMENT_3D('',#85620,#60219,#60220) ;
#51384=AXIS2_PLACEMENT_3D('',#85622,#60222,#60223) ;
#51385=AXIS2_PLACEMENT_3D('',#85625,#60226,#60227) ;
#51386=AXIS2_PLACEMENT_3D('',#85627,#60229,#60230) ;
#51387=AXIS2_PLACEMENT_3D('',#85630,#60233,#60234) ;
#51388=AXIS2_PLACEMENT_3D('',#85632,#60236,#60237) ;
#51389=AXIS2_PLACEMENT_3D('',#85635,#60240,#60241) ;
#51390=AXIS2_PLACEMENT_3D('',#85637,#60243,#60244) ;
#51391=AXIS2_PLACEMENT_3D('',#85638,#60245,#60246) ;
#51392=AXIS2_PLACEMENT_3D('',#85639,#60247,#60248) ;
#51393=AXIS2_PLACEMENT_3D('',#85640,#60249,#60250) ;
#51394=AXIS2_PLACEMENT_3D('',#85641,#60251,#60252) ;
#51395=AXIS2_PLACEMENT_3D('',#85642,#60253,#60254) ;
#51396=AXIS2_PLACEMENT_3D('',#85644,#60256,#60257) ;
#51397=AXIS2_PLACEMENT_3D('',#85645,#60258,#60259) ;
#51398=AXIS2_PLACEMENT_3D('',#85647,#60261,#60262) ;
#51399=AXIS2_PLACEMENT_3D('',#85648,#60263,#60264) ;
#51400=AXIS2_PLACEMENT_3D('',#85650,#60265,#60266) ;
#51401=AXIS2_PLACEMENT_3D('',#85652,#60267,#60268) ;
#51402=AXIS2_PLACEMENT_3D('',#85653,#60269,#60270) ;
#51403=AXIS2_PLACEMENT_3D('',#85654,#60271,#60272) ;
#51404=AXIS2_PLACEMENT_3D('',#85657,#60273,#60274) ;
#51405=AXIS2_PLACEMENT_3D('',#85658,#60275,#60276) ;
#51406=AXIS2_PLACEMENT_3D('',#85659,#60277,#60278) ;
#51407=AXIS2_PLACEMENT_3D('',#85660,#60279,#60280) ;
#51408=AXIS2_PLACEMENT_3D('',#85662,#60281,#60282) ;
#51409=AXIS2_PLACEMENT_3D('',#85664,#60283,#60284) ;
#51410=AXIS2_PLACEMENT_3D('',#85665,#60285,#60286) ;
#51411=AXIS2_PLACEMENT_3D('',#85666,#60287,#60288) ;
#51412=AXIS2_PLACEMENT_3D('',#85669,#60289,#60290) ;
#51413=AXIS2_PLACEMENT_3D('',#85670,#60291,#60292) ;
#51414=AXIS2_PLACEMENT_3D('',#85671,#60293,#60294) ;
#51415=AXIS2_PLACEMENT_3D('',#85672,#60295,#60296) ;
#51416=AXIS2_PLACEMENT_3D('',#85674,#60297,#60298) ;
#51417=AXIS2_PLACEMENT_3D('',#85676,#60299,#60300) ;
#51418=AXIS2_PLACEMENT_3D('',#85677,#60301,#60302) ;
#51419=AXIS2_PLACEMENT_3D('',#85678,#60303,#60304) ;
#51420=AXIS2_PLACEMENT_3D('',#85681,#60305,#60306) ;
#51421=AXIS2_PLACEMENT_3D('',#85682,#60307,#60308) ;
#51422=AXIS2_PLACEMENT_3D('',#85683,#60309,#60310) ;
#51423=AXIS2_PLACEMENT_3D('',#85684,#60311,#60312) ;
#51424=AXIS2_PLACEMENT_3D('',#85686,#60313,#60314) ;
#51425=AXIS2_PLACEMENT_3D('',#85688,#60315,#60316) ;
#51426=AXIS2_PLACEMENT_3D('',#85689,#60317,#60318) ;
#51427=AXIS2_PLACEMENT_3D('',#85690,#60319,#60320) ;
#51428=AXIS2_PLACEMENT_3D('',#85692,#60322,#60323) ;
#51429=AXIS2_PLACEMENT_3D('',#85695,#60324,#60325) ;
#51430=AXIS2_PLACEMENT_3D('',#85696,#60326,#60327) ;
#51431=AXIS2_PLACEMENT_3D('',#85697,#60328,#60329) ;
#51432=AXIS2_PLACEMENT_3D('',#85698,#60330,#60331) ;
#51433=AXIS2_PLACEMENT_3D('',#85700,#60333,#60334) ;
#51434=AXIS2_PLACEMENT_3D('',#85702,#60336,#60337) ;
#51435=AXIS2_PLACEMENT_3D('',#85705,#60340,#60341) ;
#51436=AXIS2_PLACEMENT_3D('',#85707,#60343,#60344) ;
#51437=AXIS2_PLACEMENT_3D('',#85709,#60346,#60347) ;
#51438=AXIS2_PLACEMENT_3D('',#85712,#60350,#60351) ;
#51439=AXIS2_PLACEMENT_3D('',#85715,#60354,#60355) ;
#51440=AXIS2_PLACEMENT_3D('',#85717,#60357,#60358) ;
#51441=AXIS2_PLACEMENT_3D('',#85719,#60360,#60361) ;
#51442=AXIS2_PLACEMENT_3D('',#85721,#60363,#60364) ;
#51443=AXIS2_PLACEMENT_3D('',#85724,#60367,#60368) ;
#51444=AXIS2_PLACEMENT_3D('',#85725,#60369,#60370) ;
#51445=AXIS2_PLACEMENT_3D('',#85726,#60371,#60372) ;
#51446=AXIS2_PLACEMENT_3D('',#85727,#60373,#60374) ;
#51447=AXIS2_PLACEMENT_3D('',#85728,#60375,#60376) ;
#51448=AXIS2_PLACEMENT_3D('',#85730,#60377,#60378) ;
#51449=AXIS2_PLACEMENT_3D('',#85731,#60379,#60380) ;
#51450=AXIS2_PLACEMENT_3D('',#85732,#60381,#60382) ;
#51451=AXIS2_PLACEMENT_3D('',#85736,#60384,#60385) ;
#51452=AXIS2_PLACEMENT_3D('',#85737,#60386,#60387) ;
#51453=AXIS2_PLACEMENT_3D('',#85738,#60388,#60389) ;
#51454=AXIS2_PLACEMENT_3D('',#85739,#60390,#60391) ;
#51455=AXIS2_PLACEMENT_3D('',#85740,#60392,#60393) ;
#51456=AXIS2_PLACEMENT_3D('',#85743,#60394,#60395) ;
#51457=AXIS2_PLACEMENT_3D('',#85747,#60397,#60398) ;
#51458=AXIS2_PLACEMENT_3D('',#85749,#60400,#60401) ;
#51459=AXIS2_PLACEMENT_3D('',#85750,#60402,#60403) ;
#51460=AXIS2_PLACEMENT_3D('',#85751,#60404,#60405) ;
#51461=AXIS2_PLACEMENT_3D('',#85752,#60406,#60407) ;
#51462=AXIS2_PLACEMENT_3D('',#85753,#60408,#60409) ;
#51463=AXIS2_PLACEMENT_3D('',#85754,#60410,#60411) ;
#51464=AXIS2_PLACEMENT_3D('',#85755,#60412,#60413) ;
#51465=AXIS2_PLACEMENT_3D('',#85759,#60416,#60417) ;
#51466=AXIS2_PLACEMENT_3D('',#85763,#60419,#60420) ;
#51467=AXIS2_PLACEMENT_3D('',#85767,#60423,#60424) ;
#51468=AXIS2_PLACEMENT_3D('',#85771,#60427,#60428) ;
#51469=AXIS2_PLACEMENT_3D('',#85773,#60429,#60430) ;
#51470=AXIS2_PLACEMENT_3D('',#85775,#60432,#60433) ;
#51471=AXIS2_PLACEMENT_3D('',#85777,#60434,#60435) ;
#51472=AXIS2_PLACEMENT_3D('',#85778,#60436,#60437) ;
#51473=AXIS2_PLACEMENT_3D('',#85779,#60438,#60439) ;
#51474=AXIS2_PLACEMENT_3D('',#85780,#60440,#60441) ;
#51475=AXIS2_PLACEMENT_3D('',#85781,#60442,#60443) ;
#51476=AXIS2_PLACEMENT_3D('',#85782,#60444,#60445) ;
#51477=AXIS2_PLACEMENT_3D('',#85783,#60446,#60447) ;
#51478=AXIS2_PLACEMENT_3D('',#85784,#60448,#60449) ;
#51479=AXIS2_PLACEMENT_3D('',#85785,#60450,#60451) ;
#51480=AXIS2_PLACEMENT_3D('',#85786,#60452,#60453) ;
#51481=AXIS2_PLACEMENT_3D('',#85787,#60454,#60455) ;
#51482=AXIS2_PLACEMENT_3D('',#85788,#60456,#60457) ;
#51483=AXIS2_PLACEMENT_3D('',#85789,#60458,#60459) ;
#51484=AXIS2_PLACEMENT_3D('',#85790,#60460,#60461) ;
#51485=AXIS2_PLACEMENT_3D('',#85791,#60462,#60463) ;
#51486=AXIS2_PLACEMENT_3D('',#85792,#60464,#60465) ;
#51487=AXIS2_PLACEMENT_3D('',#85793,#60466,#60467) ;
#51488=AXIS2_PLACEMENT_3D('',#85794,#60468,#60469) ;
#51489=AXIS2_PLACEMENT_3D('',#85795,#60470,#60471) ;
#51490=AXIS2_PLACEMENT_3D('',#85796,#60472,#60473) ;
#51491=AXIS2_PLACEMENT_3D('',#85797,#60474,#60475) ;
#51492=AXIS2_PLACEMENT_3D('',#85798,#60476,#60477) ;
#51493=AXIS2_PLACEMENT_3D('',#85799,#60478,#60479) ;
#51494=AXIS2_PLACEMENT_3D('',#85800,#60480,#60481) ;
#51495=AXIS2_PLACEMENT_3D('',#85801,#60482,#60483) ;
#51496=AXIS2_PLACEMENT_3D('',#85802,#60484,#60485) ;
#51497=AXIS2_PLACEMENT_3D('',#85803,#60486,#60487) ;
#51498=AXIS2_PLACEMENT_3D('',#85804,#60488,#60489) ;
#51499=AXIS2_PLACEMENT_3D('',#85805,#60490,#60491) ;
#51500=AXIS2_PLACEMENT_3D('',#85807,#60493,#60494) ;
#51501=AXIS2_PLACEMENT_3D('',#85809,#60495,#60496) ;
#51502=AXIS2_PLACEMENT_3D('',#85811,#60497,#60498) ;
#51503=AXIS2_PLACEMENT_3D('',#85812,#60499,#60500) ;
#51504=AXIS2_PLACEMENT_3D('',#85813,#60501,#60502) ;
#51505=AXIS2_PLACEMENT_3D('',#85815,#60504,#60505) ;
#51506=AXIS2_PLACEMENT_3D('',#85817,#60506,#60507) ;
#51507=AXIS2_PLACEMENT_3D('',#85819,#60508,#60509) ;
#51508=AXIS2_PLACEMENT_3D('',#85820,#60510,#60511) ;
#51509=AXIS2_PLACEMENT_3D('',#85821,#60512,#60513) ;
#51510=AXIS2_PLACEMENT_3D('',#85823,#60515,#60516) ;
#51511=AXIS2_PLACEMENT_3D('',#85824,#60517,#60518) ;
#51512=AXIS2_PLACEMENT_3D('',#85825,#60519,#60520) ;
#51513=AXIS2_PLACEMENT_3D('',#85826,#60521,#60522) ;
#51514=AXIS2_PLACEMENT_3D('',#85827,#60523,#60524) ;
#51515=AXIS2_PLACEMENT_3D('',#85828,#60525,#60526) ;
#51516=AXIS2_PLACEMENT_3D('',#85829,#60527,#60528) ;
#51517=AXIS2_PLACEMENT_3D('',#85830,#60529,#60530) ;
#51518=AXIS2_PLACEMENT_3D('',#85831,#60531,#60532) ;
#51519=AXIS2_PLACEMENT_3D('',#85832,#60533,#60534) ;
#51520=AXIS2_PLACEMENT_3D('',#85833,#60535,#60536) ;
#51521=AXIS2_PLACEMENT_3D('',#85834,#60537,#60538) ;
#51522=AXIS2_PLACEMENT_3D('',#85835,#60539,#60540) ;
#51523=AXIS2_PLACEMENT_3D('',#85836,#60541,#60542) ;
#51524=AXIS2_PLACEMENT_3D('',#85837,#60543,#60544) ;
#51525=AXIS2_PLACEMENT_3D('',#85838,#60545,#60546) ;
#51526=AXIS2_PLACEMENT_3D('',#85839,#60547,#60548) ;
#51527=AXIS2_PLACEMENT_3D('',#85840,#60549,#60550) ;
#51528=AXIS2_PLACEMENT_3D('',#85841,#60551,#60552) ;
#51529=AXIS2_PLACEMENT_3D('',#85842,#60553,#60554) ;
#51530=AXIS2_PLACEMENT_3D('',#85843,#60555,#60556) ;
#51531=AXIS2_PLACEMENT_3D('',#85844,#60557,#60558) ;
#51532=AXIS2_PLACEMENT_3D('',#85845,#60559,#60560) ;
#51533=AXIS2_PLACEMENT_3D('',#85846,#60561,#60562) ;
#51534=AXIS2_PLACEMENT_3D('',#85847,#60563,#60564) ;
#51535=AXIS2_PLACEMENT_3D('',#85848,#60565,#60566) ;
#51536=AXIS2_PLACEMENT_3D('',#85849,#60567,#60568) ;
#51537=AXIS2_PLACEMENT_3D('',#85850,#60569,#60570) ;
#51538=AXIS2_PLACEMENT_3D('',#85851,#60571,#60572) ;
#51539=AXIS2_PLACEMENT_3D('',#85852,#60573,#60574) ;
#51540=AXIS2_PLACEMENT_3D('',#85853,#60575,#60576) ;
#51541=AXIS2_PLACEMENT_3D('',#85854,#60577,#60578) ;
#51542=AXIS2_PLACEMENT_3D('',#85855,#60579,#60580) ;
#51543=AXIS2_PLACEMENT_3D('',#85856,#60581,#60582) ;
#51544=AXIS2_PLACEMENT_3D('',#85857,#60583,#60584) ;
#51545=AXIS2_PLACEMENT_3D('',#85858,#60585,#60586) ;
#51546=AXIS2_PLACEMENT_3D('',#85859,#60587,#60588) ;
#51547=AXIS2_PLACEMENT_3D('',#85860,#60589,#60590) ;
#51548=AXIS2_PLACEMENT_3D('',#85861,#60591,#60592) ;
#51549=AXIS2_PLACEMENT_3D('',#85862,#60593,#60594) ;
#51550=AXIS2_PLACEMENT_3D('',#85863,#60595,#60596) ;
#51551=AXIS2_PLACEMENT_3D('',#85864,#60597,#60598) ;
#51552=AXIS2_PLACEMENT_3D('',#85865,#60599,#60600) ;
#51553=AXIS2_PLACEMENT_3D('',#85866,#60601,#60602) ;
#51554=AXIS2_PLACEMENT_3D('',#85867,#60603,#60604) ;
#51555=AXIS2_PLACEMENT_3D('',#85868,#60605,#60606) ;
#51556=AXIS2_PLACEMENT_3D('',#85869,#60607,#60608) ;
#51557=AXIS2_PLACEMENT_3D('',#85870,#60609,#60610) ;
#51558=AXIS2_PLACEMENT_3D('',#85871,#60611,#60612) ;
#51559=AXIS2_PLACEMENT_3D('',#85872,#60613,#60614) ;
#51560=AXIS2_PLACEMENT_3D('',#85874,#60615,#60616) ;
#51561=AXIS2_PLACEMENT_3D('',#85875,#60617,#60618) ;
#51562=AXIS2_PLACEMENT_3D('',#85876,#60619,#60620) ;
#51563=AXIS2_PLACEMENT_3D('',#85878,#60621,#60622) ;
#51564=AXIS2_PLACEMENT_3D('',#85880,#60624,#60625) ;
#51565=AXIS2_PLACEMENT_3D('',#85882,#60626,#60627) ;
#51566=AXIS2_PLACEMENT_3D('',#85883,#60628,#60629) ;
#51567=AXIS2_PLACEMENT_3D('',#85884,#60630,#60631) ;
#51568=AXIS2_PLACEMENT_3D('',#85886,#60633,#60634) ;
#51569=AXIS2_PLACEMENT_3D('',#85888,#60635,#60636) ;
#51570=AXIS2_PLACEMENT_3D('',#85889,#60637,#60638) ;
#51571=AXIS2_PLACEMENT_3D('',#85890,#60639,#60640) ;
#51572=AXIS2_PLACEMENT_3D('',#85892,#60641,#60642) ;
#51573=AXIS2_PLACEMENT_3D('',#85893,#60643,#60644) ;
#51574=AXIS2_PLACEMENT_3D('',#85896,#60645,#60646) ;
#51575=AXIS2_PLACEMENT_3D('',#85897,#60647,#60648) ;
#51576=AXIS2_PLACEMENT_3D('',#85898,#60649,#60650) ;
#51577=AXIS2_PLACEMENT_3D('',#85899,#60651,#60652) ;
#51578=AXIS2_PLACEMENT_3D('',#85901,#60653,#60654) ;
#51579=AXIS2_PLACEMENT_3D('',#85903,#60656,#60657) ;
#51580=AXIS2_PLACEMENT_3D('',#85905,#60658,#60659) ;
#51581=AXIS2_PLACEMENT_3D('',#85907,#60660,#60661) ;
#51582=AXIS2_PLACEMENT_3D('',#85908,#60662,#60663) ;
#51583=AXIS2_PLACEMENT_3D('',#85909,#60664,#60665) ;
#51584=AXIS2_PLACEMENT_3D('',#85911,#60666,#60667) ;
#51585=AXIS2_PLACEMENT_3D('',#85913,#60668,#60669) ;
#51586=AXIS2_PLACEMENT_3D('',#85915,#60670,#60671) ;
#51587=AXIS2_PLACEMENT_3D('',#85916,#60672,#60673) ;
#51588=AXIS2_PLACEMENT_3D('',#85917,#60674,#60675) ;
#51589=AXIS2_PLACEMENT_3D('',#85921,#60677,#60678) ;
#51590=AXIS2_PLACEMENT_3D('',#85922,#60679,#60680) ;
#51591=AXIS2_PLACEMENT_3D('',#85923,#60681,#60682) ;
#51592=AXIS2_PLACEMENT_3D('',#85925,#60683,#60684) ;
#51593=AXIS2_PLACEMENT_3D('',#85926,#60685,#60686) ;
#51594=AXIS2_PLACEMENT_3D('',#85927,#60687,#60688) ;
#51595=AXIS2_PLACEMENT_3D('',#85929,#60689,#60690) ;
#51596=AXIS2_PLACEMENT_3D('',#85930,#60691,#60692) ;
#51597=AXIS2_PLACEMENT_3D('',#85932,#60693,#60694) ;
#51598=AXIS2_PLACEMENT_3D('',#85933,#60695,#60696) ;
#51599=AXIS2_PLACEMENT_3D('',#85934,#60697,#60698) ;
#51600=AXIS2_PLACEMENT_3D('',#85936,#60699,#60700) ;
#51601=AXIS2_PLACEMENT_3D('',#85938,#60702,#60703) ;
#51602=AXIS2_PLACEMENT_3D('',#85940,#60704,#60705) ;
#51603=AXIS2_PLACEMENT_3D('',#85942,#60706,#60707) ;
#51604=AXIS2_PLACEMENT_3D('',#85944,#60708,#60709) ;
#51605=AXIS2_PLACEMENT_3D('',#85945,#60710,#60711) ;
#51606=AXIS2_PLACEMENT_3D('',#85946,#60712,#60713) ;
#51607=AXIS2_PLACEMENT_3D('',#85950,#60715,#60716) ;
#51608=AXIS2_PLACEMENT_3D('',#85951,#60717,#60718) ;
#51609=AXIS2_PLACEMENT_3D('',#85952,#60719,#60720) ;
#51610=AXIS2_PLACEMENT_3D('',#85954,#60721,#60722) ;
#51611=AXIS2_PLACEMENT_3D('',#85955,#60723,#60724) ;
#51612=AXIS2_PLACEMENT_3D('',#85956,#60725,#60726) ;
#51613=AXIS2_PLACEMENT_3D('',#85958,#60727,#60728) ;
#51614=AXIS2_PLACEMENT_3D('',#85959,#60729,#60730) ;
#51615=AXIS2_PLACEMENT_3D('',#85960,#60731,#60732) ;
#51616=AXIS2_PLACEMENT_3D('',#85961,#60733,#60734) ;
#51617=AXIS2_PLACEMENT_3D('',#85962,#60735,#60736) ;
#51618=AXIS2_PLACEMENT_3D('',#85963,#60737,#60738) ;
#51619=AXIS2_PLACEMENT_3D('',#85964,#60739,#60740) ;
#51620=AXIS2_PLACEMENT_3D('',#85965,#60741,#60742) ;
#51621=AXIS2_PLACEMENT_3D('',#85966,#60743,#60744) ;
#51622=AXIS2_PLACEMENT_3D('',#85967,#60745,#60746) ;
#51623=AXIS2_PLACEMENT_3D('',#85968,#60747,#60748) ;
#51624=AXIS2_PLACEMENT_3D('',#85971,#60751,#60752) ;
#51625=AXIS2_PLACEMENT_3D('',#85973,#60754,#60755) ;
#51626=AXIS2_PLACEMENT_3D('',#85974,#60756,#60757) ;
#51627=AXIS2_PLACEMENT_3D('',#85975,#60758,#60759) ;
#51628=AXIS2_PLACEMENT_3D('',#85976,#60760,#60761) ;
#51629=AXIS2_PLACEMENT_3D('',#85977,#60762,#60763) ;
#51630=AXIS2_PLACEMENT_3D('',#85978,#60764,#60765) ;
#51631=AXIS2_PLACEMENT_3D('',#86009,#60766,#60767) ;
#51632=AXIS2_PLACEMENT_3D('',#86011,#60768,#60769) ;
#51633=AXIS2_PLACEMENT_3D('',#86012,#60770,#60771) ;
#51634=AXIS2_PLACEMENT_3D('',#86040,#60772,#60773) ;
#51635=AXIS2_PLACEMENT_3D('',#86041,#60774,#60775) ;
#51636=AXIS2_PLACEMENT_3D('',#86043,#60776,#60777) ;
#51637=AXIS2_PLACEMENT_3D('',#86044,#60778,#60779) ;
#51638=AXIS2_PLACEMENT_3D('',#86045,#60780,#60781) ;
#51639=AXIS2_PLACEMENT_3D('',#86072,#60782,#60783) ;
#51640=AXIS2_PLACEMENT_3D('',#86073,#60784,#60785) ;
#51641=AXIS2_PLACEMENT_3D('',#86075,#60786,#60787) ;
#51642=AXIS2_PLACEMENT_3D('',#86077,#60788,#60789) ;
#51643=AXIS2_PLACEMENT_3D('',#86078,#60790,#60791) ;
#51644=AXIS2_PLACEMENT_3D('',#86106,#60792,#60793) ;
#51645=AXIS2_PLACEMENT_3D('',#86107,#60794,#60795) ;
#51646=AXIS2_PLACEMENT_3D('',#86108,#60796,#60797) ;
#51647=AXIS2_PLACEMENT_3D('',#86109,#60798,#60799) ;
#51648=AXIS2_PLACEMENT_3D('',#86112,#60801,#60802) ;
#51649=AXIS2_PLACEMENT_3D('',#86143,#60803,#60804) ;
#51650=AXIS2_PLACEMENT_3D('',#86144,#60805,#60806) ;
#51651=AXIS2_PLACEMENT_3D('',#86145,#60807,#60808) ;
#51652=AXIS2_PLACEMENT_3D('',#86146,#60809,#60810) ;
#51653=AXIS2_PLACEMENT_3D('',#86173,#60811,#60812) ;
#51654=AXIS2_PLACEMENT_3D('',#86174,#60813,#60814) ;
#51655=AXIS2_PLACEMENT_3D('',#86175,#60815,#60816) ;
#51656=AXIS2_PLACEMENT_3D('',#86177,#60818,#60819) ;
#51657=AXIS2_PLACEMENT_3D('',#86178,#60820,#60821) ;
#51658=AXIS2_PLACEMENT_3D('',#86181,#60823,#60824) ;
#51659=AXIS2_PLACEMENT_3D('',#86212,#60825,#60826) ;
#51660=AXIS2_PLACEMENT_3D('',#86213,#60827,#60828) ;
#51661=AXIS2_PLACEMENT_3D('',#86214,#60829,#60830) ;
#51662=AXIS2_PLACEMENT_3D('',#86215,#60831,#60832) ;
#51663=AXIS2_PLACEMENT_3D('',#86242,#60833,#60834) ;
#51664=AXIS2_PLACEMENT_3D('',#86243,#60835,#60836) ;
#51665=AXIS2_PLACEMENT_3D('',#86244,#60837,#60838) ;
#51666=AXIS2_PLACEMENT_3D('',#86246,#60840,#60841) ;
#51667=AXIS2_PLACEMENT_3D('',#86247,#60842,#60843) ;
#51668=AXIS2_PLACEMENT_3D('',#86249,#60844,#60845) ;
#51669=AXIS2_PLACEMENT_3D('',#86251,#60847,#60848) ;
#51670=AXIS2_PLACEMENT_3D('',#86254,#60850,#60851) ;
#51671=AXIS2_PLACEMENT_3D('',#86255,#60852,#60853) ;
#51672=AXIS2_PLACEMENT_3D('',#86257,#60855,#60856) ;
#51673=AXIS2_PLACEMENT_3D('',#86258,#60857,#60858) ;
#51674=AXIS2_PLACEMENT_3D('',#86259,#60859,#60860) ;
#51675=AXIS2_PLACEMENT_3D('',#86262,#60862,#60863) ;
#51676=AXIS2_PLACEMENT_3D('',#86263,#60864,#60865) ;
#51677=AXIS2_PLACEMENT_3D('',#86265,#60867,#60868) ;
#51678=AXIS2_PLACEMENT_3D('',#86266,#60869,#60870) ;
#51679=AXIS2_PLACEMENT_3D('',#86267,#60871,#60872) ;
#51680=AXIS2_PLACEMENT_3D('',#86270,#60874,#60875) ;
#51681=AXIS2_PLACEMENT_3D('',#86271,#60876,#60877) ;
#51682=AXIS2_PLACEMENT_3D('',#86273,#60879,#60880) ;
#51683=AXIS2_PLACEMENT_3D('',#86274,#60881,#60882) ;
#51684=AXIS2_PLACEMENT_3D('',#86275,#60883,#60884) ;
#51685=AXIS2_PLACEMENT_3D('',#86279,#60887,#60888) ;
#51686=AXIS2_PLACEMENT_3D('',#86281,#60890,#60891) ;
#51687=AXIS2_PLACEMENT_3D('',#86282,#60892,#60893) ;
#51688=AXIS2_PLACEMENT_3D('',#86285,#60896,#60897) ;
#51689=AXIS2_PLACEMENT_3D('',#86286,#60898,#60899) ;
#51690=AXIS2_PLACEMENT_3D('',#86287,#60900,#60901) ;
#51691=AXIS2_PLACEMENT_3D('',#86290,#60904,#60905) ;
#51692=AXIS2_PLACEMENT_3D('',#86291,#60906,#60907) ;
#51693=AXIS2_PLACEMENT_3D('',#86292,#60908,#60909) ;
#51694=AXIS2_PLACEMENT_3D('',#86294,#60911,#60912) ;
#51695=AXIS2_PLACEMENT_3D('',#86295,#60913,#60914) ;
#51696=AXIS2_PLACEMENT_3D('',#86296,#60915,#60916) ;
#51697=AXIS2_PLACEMENT_3D('',#86297,#60917,#60918) ;
#51698=AXIS2_PLACEMENT_3D('',#86298,#60919,#60920) ;
#51699=AXIS2_PLACEMENT_3D('',#86299,#60921,#60922) ;
#51700=AXIS2_PLACEMENT_3D('',#86300,#60923,#60924) ;
#51701=AXIS2_PLACEMENT_3D('',#86301,#60925,#60926) ;
#51702=AXIS2_PLACEMENT_3D('',#86307,#60927,#60928) ;
#51703=AXIS2_PLACEMENT_3D('',#86314,#60930,#60931) ;
#51704=AXIS2_PLACEMENT_3D('',#86396,#60933,#60934) ;
#51705=AXIS2_PLACEMENT_3D('',#86422,#60935,#60936) ;
#51706=AXIS2_PLACEMENT_3D('',#86453,#60937,#60938) ;
#51707=AXIS2_PLACEMENT_3D('',#86539,#60939,#60940) ;
#51708=AXIS2_PLACEMENT_3D('',#86541,#60942,#60943) ;
#57096=DIRECTION('axis',(0.,0.,1.)) ;
#57097=DIRECTION('refdir',(1.,0.,0.)) ;
#57098=DIRECTION('center_axis',(1.,0.,0.)) ;
#57099=DIRECTION('ref_axis',(0.,0.707106781186574,-0.707106781186521)) ;
#57100=DIRECTION('',(1.,0.,0.)) ;
#57101=DIRECTION('center_axis',(0.707106781186574,0.707106781186521,0.)) ;
#57102=DIRECTION('ref_axis',(-0.707106781186521,0.707106781186574,0.)) ;
#57103=DIRECTION('',(-1.,0.,0.)) ;
#57104=DIRECTION('center_axis',(0.,1.,0.)) ;
#57105=DIRECTION('ref_axis',(-0.707106781186574,0.,-0.707106781186521)) ;
#57106=DIRECTION('',(0.,-1.,0.)) ;
#57107=DIRECTION('',(0.,1.,0.)) ;
#57108=DIRECTION('center_axis',(-0.707106781186574,0.707106781186521,0.)) ;
#57109=DIRECTION('ref_axis',(-0.707106781186521,-0.707106781186574,0.)) ;
#57110=DIRECTION('center_axis',(-1.,0.,0.)) ;
#57111=DIRECTION('ref_axis',(0.,-0.707106781186574,-0.707106781186521)) ;
#57112=DIRECTION('',(1.,0.,0.)) ;
#57113=DIRECTION('',(-1.,0.,0.)) ;
#57114=DIRECTION('center_axis',(0.,1.,0.)) ;
#57115=DIRECTION('ref_axis',(1.,0.,0.)) ;
#57116=DIRECTION('',(0.,0.,-1.)) ;
#57117=DIRECTION('',(1.,0.,1.51760508056877E-16)) ;
#57118=DIRECTION('',(0.,0.,-1.)) ;
#57119=DIRECTION('center_axis',(-1.,0.,0.)) ;
#57120=DIRECTION('ref_axis',(0.,1.,0.)) ;
#57121=DIRECTION('',(0.,0.,-1.)) ;
#57122=DIRECTION('',(0.,1.,5.60383084497428E-34)) ;
#57123=DIRECTION('center_axis',(0.,-1.,0.)) ;
#57124=DIRECTION('ref_axis',(-1.,0.,0.)) ;
#57125=DIRECTION('',(0.,0.,-1.)) ;
#57126=DIRECTION('',(-1.,0.,-1.51760508056877E-16)) ;
#57127=DIRECTION('',(0.,0.,-1.)) ;
#57128=DIRECTION('center_axis',(0.,0.,1.)) ;
#57129=DIRECTION('ref_axis',(-1.,0.,0.)) ;
#57130=DIRECTION('',(1.,0.,0.)) ;
#57131=DIRECTION('',(0.536696284465946,-0.843775502275604,0.)) ;
#57132=DIRECTION('',(1.,0.,0.)) ;
#57133=DIRECTION('',(-0.538514312398237,0.842616363087173,0.)) ;
#57134=DIRECTION('',(-1.,0.,0.)) ;
#57135=DIRECTION('',(0.,-1.,0.)) ;
#57136=DIRECTION('',(1.,0.,0.)) ;
#57137=DIRECTION('',(0.,1.,0.)) ;
#57138=DIRECTION('center_axis',(-0.538514312398237,0.842616363087172,0.)) ;
#57139=DIRECTION('ref_axis',(-0.595819744277688,-0.380787122062806,-0.707106781186545)) ;
#57140=DIRECTION('center_axis',(0.480356996202705,0.877073062064452,0.)) ;
#57141=DIRECTION('ref_axis',(0.877073062064452,-0.480356996202705,0.)) ;
#57142=DIRECTION('',(0.538514312398237,-0.842616363087173,0.)) ;
#57143=DIRECTION('center_axis',(1.,0.,0.)) ;
#57144=DIRECTION('ref_axis',(0.,0.707106781186574,-0.707106781186521)) ;
#57145=DIRECTION('center_axis',(0.876554700080465,-0.481302251986053,0.)) ;
#57146=DIRECTION('ref_axis',(-0.481302251986053,-0.876554700080465,0.)) ;
#57147=DIRECTION('',(-1.,0.,0.)) ;
#57148=DIRECTION('center_axis',(0.536696284465946,-0.843775502275604,0.)) ;
#57149=DIRECTION('ref_axis',(0.596639379458124,0.379501582183469,-0.707106781186596)) ;
#57150=DIRECTION('',(-0.536696284465946,0.843775502275604,0.)) ;
#57151=DIRECTION('center_axis',(0.999980832705611,-0.00587550485991174,
-0.00195260442350964)) ;
#57152=DIRECTION('ref_axis',(-0.00195251174417658,2.1509854887887E-5,-0.99999809361579)) ;
#57153=DIRECTION('center_axis',(1.,0.,0.)) ;
#57154=DIRECTION('ref_axis',(0.,0.707106781186574,-0.707106781186521)) ;
#57155=DIRECTION('',(-1.,0.,0.)) ;
#57156=DIRECTION('center_axis',(-0.999999985503101,-0.000120403056781265,
-0.000120403083049754)) ;
#57157=DIRECTION('ref_axis',(0.000120401111956324,1.63776238757342E-5,-0.999999992617673)) ;
#57158=DIRECTION('center_axis',(0.707106781186574,0.707106781186521,0.)) ;
#57159=DIRECTION('ref_axis',(-0.707106781186521,0.707106781186574,0.)) ;
#57160=DIRECTION('center_axis',(0.,1.,0.)) ;
#57161=DIRECTION('ref_axis',(-0.707106781186574,0.,-0.707106781186521)) ;
#57162=DIRECTION('center_axis',(0.707106781186574,0.707106781186521,0.)) ;
#57163=DIRECTION('ref_axis',(0.707106781186521,-0.707106781186574,0.)) ;
#57164=DIRECTION('',(0.,-1.,0.)) ;
#57165=DIRECTION('center_axis',(1.,0.,0.)) ;
#57166=DIRECTION('ref_axis',(0.,0.707106781186574,-0.707106781186521)) ;
#57167=DIRECTION('',(-1.,0.,0.)) ;
#57168=DIRECTION('center_axis',(0.707106781186574,-0.707106781186521,0.)) ;
#57169=DIRECTION('ref_axis',(-0.707106781186521,-0.707106781186574,0.)) ;
#57170=DIRECTION('center_axis',(0.,-1.,0.)) ;
#57171=DIRECTION('ref_axis',(0.707106781186574,0.,-0.707106781186521)) ;
#57172=DIRECTION('',(0.,1.,0.)) ;
#57173=DIRECTION('center_axis',(-0.707106781186574,-0.707106781186521,0.)) ;
#57174=DIRECTION('ref_axis',(-0.707106781186521,0.707106781186574,0.)) ;
#57175=DIRECTION('center_axis',(-1.,0.,0.)) ;
#57176=DIRECTION('ref_axis',(0.,-0.707106781186574,-0.707106781186521)) ;
#57177=DIRECTION('',(1.,0.,0.)) ;
#57178=DIRECTION('',(0.,0.,-1.)) ;
#57179=DIRECTION('',(0.,0.,-1.)) ;
#57180=DIRECTION('',(0.,0.,-1.)) ;
#57181=DIRECTION('center_axis',(-0.842616363087172,-0.538514312398237,0.)) ;
#57182=DIRECTION('ref_axis',(-0.538514312398237,0.842616363087172,0.)) ;
#57183=DIRECTION('',(0.,0.,-1.)) ;
#57184=DIRECTION('',(-0.538514312398237,0.842616363087173,-8.17252056454565E-17)) ;
#57185=DIRECTION('center_axis',(0.,1.,0.)) ;
#57186=DIRECTION('ref_axis',(1.,0.,0.)) ;
#57187=DIRECTION('',(0.,0.,-1.)) ;
#57188=DIRECTION('',(1.,0.,1.51760508056877E-16)) ;
#57189=DIRECTION('center_axis',(0.843775502275604,0.536696284465946,0.)) ;
#57190=DIRECTION('ref_axis',(0.536696284465946,-0.843775502275604,0.)) ;
#57191=DIRECTION('',(0.,0.,-1.)) ;
#57192=DIRECTION('',(0.536696284465946,-0.843775502275604,8.14493008027904E-17)) ;
#57193=DIRECTION('',(0.,0.,-1.)) ;
#57194=DIRECTION('',(0.,0.,-1.)) ;
#57195=DIRECTION('',(0.,0.,-1.)) ;
#57196=DIRECTION('',(0.,0.,-1.)) ;
#57197=DIRECTION('center_axis',(0.,1.,0.)) ;
#57198=DIRECTION('ref_axis',(1.,0.,0.)) ;
#57199=DIRECTION('',(0.,0.,-1.)) ;
#57200=DIRECTION('',(1.,0.,1.51760508056877E-16)) ;
#57201=DIRECTION('center_axis',(-1.,0.,-1.51760508056877E-16)) ;
#57202=DIRECTION('ref_axis',(-1.07310884363333E-16,0.707106781186547,0.707106781186547)) ;
#57203=DIRECTION('',(1.,0.,1.51760508056877E-16)) ;
#57204=DIRECTION('center_axis',(-0.707106781186574,0.707106781186521,0.)) ;
#57205=DIRECTION('ref_axis',(0.707106781186521,0.707106781186574,2.14621768726675E-16)) ;
#57206=DIRECTION('center_axis',(1.,0.,1.51760508056877E-16)) ;
#57207=DIRECTION('ref_axis',(-1.07310884363333E-16,-0.707106781186547,0.707106781186547)) ;
#57208=DIRECTION('',(-1.,0.,-1.51760508056877E-16)) ;
#57209=DIRECTION('center_axis',(-0.707106781186574,-0.707106781186521,0.)) ;
#57210=DIRECTION('ref_axis',(-0.707106781186521,0.707106781186574,-2.14621768726675E-16)) ;
#57211=DIRECTION('center_axis',(0.,1.,5.60383084497428E-34)) ;
#57212=DIRECTION('ref_axis',(0.707106781186547,-3.96250679110365E-34,0.707106781186547)) ;
#57213=DIRECTION('',(0.,-1.,-5.60383084497428E-34)) ;
#57214=DIRECTION('center_axis',(-1.51760508056877E-16,-5.60383084497428E-34,
1.)) ;
#57215=DIRECTION('ref_axis',(1.,1.81422958079369E-66,1.51760508056877E-16)) ;
#57216=DIRECTION('center_axis',(0.707106781186552,0.707106781186543,0.)) ;
#57217=DIRECTION('ref_axis',(-0.500000000000041,0.500000000000047,-0.707106781186485)) ;
#57218=DIRECTION('',(0.707106781186552,0.707106781186543,0.)) ;
#57219=DIRECTION('center_axis',(1.,-5.23364152894628E-14,-7.40148683083437E-14)) ;
#57220=DIRECTION('ref_axis',(-5.23364152894683E-14,-1.,-7.40148683083368E-14)) ;
#57221=DIRECTION('',(-0.707106781186552,-0.707106781186543,0.)) ;
#57222=DIRECTION('center_axis',(-0.38268343236509,0.923879532511287,0.)) ;
#57223=DIRECTION('ref_axis',(0.923879532511287,0.38268343236509,0.)) ;
#57224=DIRECTION('center_axis',(0.707106781186552,-0.707106781186543,0.)) ;
#57225=DIRECTION('ref_axis',(0.499999999999936,0.499999999999943,-0.707106781186633)) ;
#57226=DIRECTION('',(-0.707106781186552,0.707106781186543,0.)) ;
#57227=DIRECTION('',(0.707106781186552,-0.707106781186543,0.)) ;
#57228=DIRECTION('center_axis',(-0.38268343236508,-0.923879532511291,0.)) ;
#57229=DIRECTION('ref_axis',(-0.923879532511291,0.38268343236508,0.)) ;
#57230=DIRECTION('center_axis',(-1.,0.,0.)) ;
#57231=DIRECTION('ref_axis',(0.,-0.707106781186574,-0.707106781186521)) ;
#57232=DIRECTION('',(1.,0.,0.)) ;
#57233=DIRECTION('',(-1.,0.,0.)) ;
#57234=DIRECTION('center_axis',(0.,-1.,0.)) ;
#57235=DIRECTION('ref_axis',(-1.,0.,-1.77819390572528E-34)) ;
#57236=DIRECTION('',(0.,0.,-1.)) ;
#57237=DIRECTION('',(-1.,0.,-1.51760508056877E-16)) ;
#57238=DIRECTION('',(0.,0.,-1.)) ;
#57239=DIRECTION('center_axis',(-0.707106781186543,0.707106781186552,0.)) ;
#57240=DIRECTION('ref_axis',(0.707106781186552,0.707106781186543,1.25737296900294E-34)) ;
#57241=DIRECTION('',(0.,0.,-1.)) ;
#57242=DIRECTION('',(0.707106781186552,0.707106781186543,1.07310884363334E-16)) ;
#57243=DIRECTION('center_axis',(0.,0.,-1.)) ;
#57244=DIRECTION('ref_axis',(-1.,0.,0.)) ;
#57245=DIRECTION('center_axis',(0.,1.,0.)) ;
#57246=DIRECTION('ref_axis',(-0.707106781186521,0.,-0.707106781186574)) ;
#57247=DIRECTION('',(0.,1.,0.)) ;
#57248=DIRECTION('center_axis',(0.7071067811866,0.707106781186495,0.)) ;
#57249=DIRECTION('ref_axis',(0.707106781186495,-0.7071067811866,0.)) ;
#57250=DIRECTION('',(0.,-1.,0.)) ;
#57251=DIRECTION('center_axis',(-0.707106781186495,0.7071067811866,0.)) ;
#57252=DIRECTION('ref_axis',(0.7071067811866,0.707106781186495,0.)) ;
#57253=DIRECTION('center_axis',(1.,0.,0.)) ;
#57254=DIRECTION('ref_axis',(0.,0.707106781186574,-0.707106781186521)) ;
#57255=DIRECTION('',(-1.,0.,0.)) ;
#57256=DIRECTION('',(1.,0.,0.)) ;
#57257=DIRECTION('center_axis',(0.707106781186574,-0.707106781186521,0.)) ;
#57258=DIRECTION('ref_axis',(-0.707106781186521,-0.707106781186574,0.)) ;
#57259=DIRECTION('center_axis',(0.,-1.,0.)) ;
#57260=DIRECTION('ref_axis',(0.707106781186574,0.,-0.707106781186521)) ;
#57261=DIRECTION('',(0.,1.,0.)) ;
#57262=DIRECTION('',(0.,-1.,0.)) ;
#57263=DIRECTION('center_axis',(-0.707106781186469,-0.707106781186626,0.)) ;
#57264=DIRECTION('ref_axis',(-0.707106781186626,0.707106781186469,0.)) ;
#57265=DIRECTION('center_axis',(-1.,0.,0.)) ;
#57266=DIRECTION('ref_axis',(0.,-0.707106781186574,-0.707106781186521)) ;
#57267=DIRECTION('',(1.,0.,0.)) ;
#57268=DIRECTION('',(-1.,0.,0.)) ;
#57269=DIRECTION('center_axis',(0.,-1.,0.)) ;
#57270=DIRECTION('ref_axis',(-1.,0.,0.)) ;
#57271=DIRECTION('',(0.,0.,-1.)) ;
#57272=DIRECTION('',(-1.,0.,-1.51760508056877E-16)) ;
#57273=DIRECTION('',(0.,0.,-1.)) ;
#57274=DIRECTION('center_axis',(-1.,0.,0.)) ;
#57275=DIRECTION('ref_axis',(0.,1.,0.)) ;
#57276=DIRECTION('',(0.,0.,-1.)) ;
#57277=DIRECTION('',(0.,1.,5.60383084497428E-34)) ;
#57278=DIRECTION('center_axis',(0.,0.,-1.)) ;
#57279=DIRECTION('ref_axis',(-1.,0.,0.)) ;
#57280=DIRECTION('center_axis',(-0.707106781186552,0.707106781186543,0.)) ;
#57281=DIRECTION('ref_axis',(-0.499999999999936,-0.499999999999943,-0.707106781186633)) ;
#57282=DIRECTION('',(-0.707106781186552,0.707106781186543,0.)) ;
#57283=DIRECTION('center_axis',(0.38268343236508,0.923879532511291,0.)) ;
#57284=DIRECTION('ref_axis',(0.923879532511291,-0.38268343236508,0.)) ;
#57285=DIRECTION('',(0.707106781186552,-0.707106781186543,0.)) ;
#57286=DIRECTION('center_axis',(-1.,5.23364152894628E-14,-7.40148683083437E-14)) ;
#57287=DIRECTION('ref_axis',(5.23364152894683E-14,1.,-7.40148683083368E-14)) ;
#57288=DIRECTION('center_axis',(1.,0.,0.)) ;
#57289=DIRECTION('ref_axis',(0.,0.707106781186574,-0.707106781186521)) ;
#57290=DIRECTION('',(-1.,0.,0.)) ;
#57291=DIRECTION('',(1.,0.,0.)) ;
#57292=DIRECTION('center_axis',(0.38268343236509,-0.923879532511287,0.)) ;
#57293=DIRECTION('ref_axis',(-0.923879532511287,-0.38268343236509,0.)) ;
#57294=DIRECTION('center_axis',(-0.707106781186552,-0.707106781186543,0.)) ;
#57295=DIRECTION('ref_axis',(0.500000000000041,-0.500000000000047,-0.707106781186485)) ;
#57296=DIRECTION('',(0.707106781186552,0.707106781186543,0.)) ;
#57297=DIRECTION('',(-0.707106781186552,-0.707106781186543,0.)) ;
#57298=DIRECTION('center_axis',(0.707106781186543,-0.707106781186552,0.)) ;
#57299=DIRECTION('ref_axis',(-0.707106781186552,-0.707106781186543,-1.25737296900294E-34)) ;
#57300=DIRECTION('',(0.,0.,-1.)) ;
#57301=DIRECTION('',(-0.707106781186552,-0.707106781186543,-1.07310884363334E-16)) ;
#57302=DIRECTION('',(0.,0.,-1.)) ;
#57303=DIRECTION('center_axis',(-0.707106781186543,-0.707106781186552,0.)) ;
#57304=DIRECTION('ref_axis',(-0.707106781186552,0.707106781186543,-1.25737296900294E-34)) ;
#57305=DIRECTION('',(0.,0.,-1.)) ;
#57306=DIRECTION('',(-0.707106781186552,0.707106781186543,-1.07310884363334E-16)) ;
#57307=DIRECTION('center_axis',(0.,0.,-1.)) ;
#57308=DIRECTION('ref_axis',(-1.,0.,0.)) ;
#57309=DIRECTION('center_axis',(-0.538514312398237,0.842616363087172,-8.17252056454566E-17)) ;
#57310=DIRECTION('ref_axis',(0.595819744277703,0.380787122062815,0.707106781186527)) ;
#57311=DIRECTION('',(0.538514312398237,-0.842616363087173,8.17252056454565E-17)) ;
#57312=DIRECTION('center_axis',(0.48035699620269,0.87707306206446,0.)) ;
#57313=DIRECTION('ref_axis',(-0.87707306206446,0.48035699620269,-1.73030634072448E-16)) ;
#57314=DIRECTION('center_axis',(0.536696284465946,-0.843775502275604,8.14493008027904E-17)) ;
#57315=DIRECTION('ref_axis',(-0.596639379458102,-0.379501582183455,0.707106781186622)) ;
#57316=DIRECTION('center_axis',(-0.538364893193227,0.842709511753463,-0.00198004476873555)) ;
#57317=DIRECTION('ref_axis',(-0.0010804597739936,0.00165936097387972,0.999998039561996)) ;
#57318=DIRECTION('',(-0.536696284465946,0.843775502275604,-8.14493008027904E-17)) ;
#57319=DIRECTION('center_axis',(0.87655470008041,-0.481302251986153,0.)) ;
#57320=DIRECTION('ref_axis',(0.481302251986153,0.87655470008041,-1.69226926461802E-16)) ;
#57321=DIRECTION('center_axis',(0.,1.,5.60383084497428E-34)) ;
#57322=DIRECTION('ref_axis',(0.707106781186547,-3.96250679110365E-34,0.707106781186547)) ;
#57323=DIRECTION('',(0.,1.,5.60383084497428E-34)) ;
#57324=DIRECTION('center_axis',(-0.707106781186574,-0.707106781186521,0.)) ;
#57325=DIRECTION('ref_axis',(0.707106781186521,-0.707106781186574,-7.92501358220702E-34)) ;
#57326=DIRECTION('',(0.,-1.,-5.60383084497428E-34)) ;
#57327=DIRECTION('center_axis',(0.707106781186574,0.707106781186521,0.)) ;
#57328=DIRECTION('ref_axis',(0.707106781186521,-0.707106781186574,-7.92501358220702E-34)) ;
#57329=DIRECTION('center_axis',(-1.,0.,-1.51760508056877E-16)) ;
#57330=DIRECTION('ref_axis',(-1.07310884363333E-16,0.707106781186547,0.707106781186547)) ;
#57331=DIRECTION('',(1.,0.,1.51760508056877E-16)) ;
#57332=DIRECTION('center_axis',(-0.707106781186574,-0.707106781186521,0.)) ;
#57333=DIRECTION('ref_axis',(0.707106781186521,-0.707106781186574,2.14621768726675E-16)) ;
#57334=DIRECTION('',(-1.,0.,-1.51760508056877E-16)) ;
#57335=DIRECTION('center_axis',(0.,-1.,-5.60383084497428E-34)) ;
#57336=DIRECTION('ref_axis',(-0.707106781186547,-3.96250679110365E-34,0.707106781186547)) ;
#57337=DIRECTION('',(0.,1.,5.60383084497428E-34)) ;
#57338=DIRECTION('center_axis',(0.707106781186574,-0.707106781186521,0.)) ;
#57339=DIRECTION('ref_axis',(0.707106781186521,0.707106781186574,7.92501358220702E-34)) ;
#57340=DIRECTION('',(0.,-1.,-5.60383084497428E-34)) ;
#57341=DIRECTION('center_axis',(1.,0.,1.51760508056877E-16)) ;
#57342=DIRECTION('ref_axis',(-1.07310884363333E-16,-0.707106781186547,0.707106781186547)) ;
#57343=DIRECTION('',(1.,0.,1.51760508056877E-16)) ;
#57344=DIRECTION('',(-1.,0.,-1.51760508056877E-16)) ;
#57345=DIRECTION('center_axis',(-0.999999927776723,-0.000360666211120845,
0.000119860056843106)) ;
#57346=DIRECTION('ref_axis',(0.000119860035380113,8.11099348877999E-8,0.999999992816783)) ;
#57347=DIRECTION('center_axis',(1.,0.,1.51760508056877E-16)) ;
#57348=DIRECTION('ref_axis',(-1.07310884363333E-16,-0.707106781186547,0.707106781186547)) ;
#57349=DIRECTION('',(-1.,0.,-1.51760508056877E-16)) ;
#57350=DIRECTION('center_axis',(1.,0.,1.51760508056877E-16)) ;
#57351=DIRECTION('ref_axis',(-1.07310884363333E-16,-0.707106781186547,0.707106781186547)) ;
#57352=DIRECTION('',(-1.,0.,-1.51760508056877E-16)) ;
#57353=DIRECTION('',(0.,0.,-1.)) ;
#57354=DIRECTION('',(0.,0.,-1.)) ;
#57355=DIRECTION('',(0.,0.,-1.)) ;
#57356=DIRECTION('',(0.,0.,-1.)) ;
#57357=DIRECTION('',(0.,0.,-1.)) ;
#57358=DIRECTION('center_axis',(0.,-1.,0.)) ;
#57359=DIRECTION('ref_axis',(-1.,0.,0.)) ;
#57360=DIRECTION('',(0.,0.,-1.)) ;
#57361=DIRECTION('center_axis',(1.,0.,0.)) ;
#57362=DIRECTION('ref_axis',(0.,-1.,0.)) ;
#57363=DIRECTION('',(0.,0.,-1.)) ;
#57364=DIRECTION('center_axis',(0.,1.,0.)) ;
#57365=DIRECTION('ref_axis',(1.,0.,0.)) ;
#57366=DIRECTION('',(0.,0.,-1.)) ;
#57367=DIRECTION('center_axis',(-1.,0.,0.)) ;
#57368=DIRECTION('ref_axis',(0.,1.,0.)) ;
#57369=DIRECTION('center_axis',(-1.51760508056877E-16,-5.60383084497428E-34,
1.)) ;
#57370=DIRECTION('ref_axis',(1.,1.81422958079369E-66,1.51760508056877E-16)) ;
#57371=DIRECTION('',(0.,-1.,-5.60383084497428E-34)) ;
#57372=DIRECTION('',(1.,0.,1.51760508056877E-16)) ;
#57373=DIRECTION('',(0.,1.,5.60383084497428E-34)) ;
#57374=DIRECTION('center_axis',(-1.51760508056877E-16,-5.60383084497428E-34,
1.)) ;
#57375=DIRECTION('ref_axis',(1.99707445226891E-15,-1.,3.02516650419242E-31)) ;
#57376=DIRECTION('',(1.,-3.19495806435525E-17,1.51760508056877E-16)) ;
#57377=DIRECTION('center_axis',(-1.51760508056877E-16,-5.60383084497428E-34,
1.)) ;
#57378=DIRECTION('ref_axis',(1.75742551799664E-15,-1.,2.66147406398793E-31)) ;
#57379=DIRECTION('',(0.,-1.,-5.60383084497428E-34)) ;
#57380=DIRECTION('',(1.,0.,1.51760508056877E-16)) ;
#57381=DIRECTION('center_axis',(-1.51760508056877E-16,-5.60383084497428E-34,
1.)) ;
#57382=DIRECTION('ref_axis',(1.,2.24153233798966E-35,1.51760508056877E-16)) ;
#57383=DIRECTION('center_axis',(-1.51760508056877E-16,-5.60383084497428E-34,
1.)) ;
#57384=DIRECTION('ref_axis',(1.,2.24153233798966E-35,1.51760508056877E-16)) ;
#57385=DIRECTION('',(1.,0.,1.51760508056877E-16)) ;
#57386=DIRECTION('',(0.,1.,5.60383084497428E-34)) ;
#57387=DIRECTION('center_axis',(-1.51760508056877E-16,-5.60383084497428E-34,
1.)) ;
#57388=DIRECTION('ref_axis',(9.58595737089076E-16,-1.,1.44916592997297E-31)) ;
#57389=DIRECTION('',(1.,-3.19495806435525E-17,1.51760508056877E-16)) ;
#57390=DIRECTION('center_axis',(-1.51760508056877E-16,-5.60383084497428E-34,
1.)) ;
#57391=DIRECTION('ref_axis',(1.35801062754286E-15,-1.,2.05531999698045E-31)) ;
#57392=DIRECTION('',(0.,-1.,-5.60383084497428E-34)) ;
#57393=DIRECTION('',(1.,0.,1.51760508056877E-16)) ;
#57394=DIRECTION('',(-2.22044604925031E-16,1.,-3.31372189702139E-32)) ;
#57395=DIRECTION('center_axis',(1.51760508056877E-16,5.60383084497428E-34,
-1.)) ;
#57396=DIRECTION('ref_axis',(-0.70710678118657,-0.707106781186525,-1.07310884363337E-16)) ;
#57397=DIRECTION('',(-1.,0.,-1.51760508056877E-16)) ;
#57398=DIRECTION('center_axis',(1.51760508056877E-16,5.60383084497428E-34,
-1.)) ;
#57399=DIRECTION('ref_axis',(0.707106781186573,-0.707106781186522,1.07310884363337E-16)) ;
#57400=DIRECTION('',(2.33146835171284E-14,-1.,3.53768783266021E-30)) ;
#57401=DIRECTION('center_axis',(-1.51760508056877E-16,-5.60383084497428E-34,
1.)) ;
#57402=DIRECTION('ref_axis',(-0.707106781186485,0.70710678118661,-1.07310884363324E-16)) ;
#57403=DIRECTION('',(-1.,0.,-1.51760508056877E-16)) ;
#57404=DIRECTION('center_axis',(-1.51760508056877E-16,-5.60383084497428E-34,
1.)) ;
#57405=DIRECTION('ref_axis',(0.70710678118661,0.707106781186485,1.07310884363343E-16)) ;
#57406=DIRECTION('',(2.22044604925032E-15,1.,3.37536403631613E-31)) ;
#57407=DIRECTION('center_axis',(1.51760508056877E-16,5.60383084497428E-34,
-1.)) ;
#57408=DIRECTION('ref_axis',(-0.707106781186548,-0.707106781186548,-1.07310884363333E-16)) ;
#57409=DIRECTION('',(-1.,0.,-1.51760508056877E-16)) ;
#57410=DIRECTION('center_axis',(-1.51760508056877E-16,-5.60383084497428E-34,
1.)) ;
#57411=DIRECTION('ref_axis',(0.707106781186547,0.707106781186547,1.07310884363333E-16)) ;
#57412=DIRECTION('',(5.25359141716359E-35,1.,5.60383084497428E-34)) ;
#57413=DIRECTION('center_axis',(1.51760508056877E-16,5.60383084497428E-34,
-1.)) ;
#57414=DIRECTION('ref_axis',(-0.953716950748229,-0.300705799504266,-1.44736568988007E-16)) ;
#57415=DIRECTION('',(-0.573576436351042,0.819152044288994,-8.70462513900874E-17)) ;
#57416=DIRECTION('center_axis',(1.51760508056877E-16,5.60383084497428E-34,
-1.)) ;
#57417=DIRECTION('ref_axis',(-0.53729960834682,-0.843391445812888,-8.15408615414745E-17)) ;
#57418=DIRECTION('',(-0.984807753012209,0.173648177666924,-1.49454924935485E-16)) ;
#57419=DIRECTION('center_axis',(1.51760508056877E-16,5.60383084497428E-34,
-1.)) ;
#57420=DIRECTION('ref_axis',(0.642787609686539,-0.766044443118978,9.75497742186947E-17)) ;
#57421=DIRECTION('',(5.23472275150178E-15,-1.,7.93863801220309E-31)) ;
#57422=DIRECTION('center_axis',(-1.51760508056877E-16,-5.60383084497428E-34,
1.)) ;
#57423=DIRECTION('ref_axis',(-0.923879532511313,0.382683432365025,-1.40208427237267E-16)) ;
#57424=DIRECTION('',(-0.707106781186521,-0.707106781186574,-1.0731088436333E-16)) ;
#57425=DIRECTION('center_axis',(1.51760508056877E-16,5.60383084497428E-34,
-1.)) ;
#57426=DIRECTION('ref_axis',(0.923879532511288,-0.382683432365087,1.40208427237263E-16)) ;
#57427=DIRECTION('',(6.83214169000096E-16,-1.,1.03124546314615E-31)) ;
#57428=DIRECTION('center_axis',(1.51760508056877E-16,5.60383084497428E-34,
-1.)) ;
#57429=DIRECTION('ref_axis',(0.718421208107098,0.695608343640254,1.09027967541169E-16)) ;
#57430=DIRECTION('center_axis',(-1.51760508056877E-16,-5.60383084497428E-34,
1.)) ;
#57431=DIRECTION('ref_axis',(-0.718421208107092,-0.69560834364026,-1.09027967541168E-16)) ;
#57432=DIRECTION('',(0.,-1.,-5.60383084497428E-34)) ;
#57433=DIRECTION('center_axis',(-1.51760508056877E-16,-5.60383084497428E-34,
1.)) ;
#57434=DIRECTION('ref_axis',(-0.718421208107087,0.695608343640265,-1.09027967541167E-16)) ;
#57435=DIRECTION('center_axis',(1.51760508056877E-16,5.60383084497428E-34,
-1.)) ;
#57436=DIRECTION('ref_axis',(0.718421208107084,-0.695608343640269,1.09027967541166E-16)) ;
#57437=DIRECTION('',(6.83214169000096E-16,-1.,1.03124546314615E-31)) ;
#57438=DIRECTION('center_axis',(1.51760508056877E-16,5.60383084497428E-34,
-1.)) ;
#57439=DIRECTION('ref_axis',(0.923879532511263,0.382683432365148,1.40208427237259E-16)) ;
#57440=DIRECTION('',(0.707106781186615,-0.70710678118648,1.07310884363344E-16)) ;
#57441=DIRECTION('center_axis',(-1.51760508056877E-16,-5.60383084497428E-34,
1.)) ;
#57442=DIRECTION('ref_axis',(-0.923879532511263,-0.382683432365148,-1.40208427237259E-16)) ;
#57443=DIRECTION('',(-0.707106781186552,-0.707106781186543,-1.07310884363334E-16)) ;
#57444=DIRECTION('',(-0.707106781186552,0.707106781186543,-1.07310884363334E-16)) ;
#57445=DIRECTION('',(1.,0.,1.51760508056877E-16)) ;
#57446=DIRECTION('',(0.707106781186552,-0.707106781186543,1.07310884363334E-16)) ;
#57447=DIRECTION('',(-1.,0.,-1.51760508056877E-16)) ;
#57448=DIRECTION('',(0.707106781186552,0.707106781186543,1.07310884363334E-16)) ;
#57449=DIRECTION('center_axis',(-1.51760508056877E-16,-5.60383084497428E-34,
1.)) ;
#57450=DIRECTION('ref_axis',(0.707106781186485,-0.70710678118661,1.07310884363324E-16)) ;
#57451=DIRECTION('',(1.,0.,1.51760508056877E-16)) ;
#57452=DIRECTION('center_axis',(-1.51760508056877E-16,-5.60383084497428E-34,
1.)) ;
#57453=DIRECTION('ref_axis',(-0.707106781186359,-0.707106781186736,-1.07310884363305E-16)) ;
#57454=DIRECTION('',(0.,-1.,-5.60383084497428E-34)) ;
#57455=DIRECTION('center_axis',(-1.51760508056877E-16,-5.60383084497428E-34,
1.)) ;
#57456=DIRECTION('ref_axis',(-0.707106781186485,0.70710678118661,-1.07310884363324E-16)) ;
#57457=DIRECTION('',(-1.,0.,-1.51760508056877E-16)) ;
#57458=DIRECTION('',(0.,-1.,-5.60383084497428E-34)) ;
#57459=DIRECTION('center_axis',(-1.51760508056877E-16,-5.60383084497428E-34,
1.)) ;
#57460=DIRECTION('ref_axis',(-0.707106781186485,0.70710678118661,-1.07310884363324E-16)) ;
#57461=DIRECTION('',(-1.,0.,-1.51760508056877E-16)) ;
#57462=DIRECTION('center_axis',(-1.51760508056877E-16,-5.60383084497428E-34,
1.)) ;
#57463=DIRECTION('ref_axis',(0.70710678118661,0.707106781186485,1.07310884363343E-16)) ;
#57464=DIRECTION('',(0.,1.,5.60383084497428E-34)) ;
#57465=DIRECTION('',(-1.,0.,-1.51760508056877E-16)) ;
#57466=DIRECTION('center_axis',(-1.51760508056877E-16,-5.60383084497428E-34,
1.)) ;
#57467=DIRECTION('ref_axis',(0.707106781186359,0.707106781186736,1.07310884363305E-16)) ;
#57468=DIRECTION('',(0.,1.,5.60383084497428E-34)) ;
#57469=DIRECTION('',(-7.105427357601E-15,-1.,-1.07888364883526E-30)) ;
#57470=DIRECTION('',(1.,0.,1.51760508056877E-16)) ;
#57471=DIRECTION('',(-3.17206578464329E-15,1.,-4.80833931982806E-31)) ;
#57472=DIRECTION('',(-1.,3.55271367880051E-14,-1.51760508056877E-16)) ;
#57473=DIRECTION('',(-7.105427357601E-15,-1.,-1.07888364883526E-30)) ;
#57474=DIRECTION('center_axis',(-1.51760508056877E-16,-5.60383084497428E-34,
1.)) ;
#57475=DIRECTION('ref_axis',(0.707106781186485,-0.70710678118661,1.07310884363324E-16)) ;
#57476=DIRECTION('',(1.,-7.10542735760144E-15,1.51760508056877E-16)) ;
#57477=DIRECTION('center_axis',(-1.51760508056877E-16,-5.60383084497428E-34,
1.)) ;
#57478=DIRECTION('ref_axis',(-0.382683432365031,-0.923879532511311,-5.80762321206666E-17)) ;
#57479=DIRECTION('',(0.707106781186544,-0.707106781186551,1.07310884363333E-16)) ;
#57480=DIRECTION('center_axis',(-1.51760508056877E-16,-5.60383084497428E-34,
1.)) ;
#57481=DIRECTION('ref_axis',(-0.92387953251129,-0.382683432365082,-1.40208427237263E-16)) ;
#57482=DIRECTION('',(-3.73034936274055E-14,-1.,-5.66175752827605E-30)) ;
#57483=DIRECTION('center_axis',(-1.51760508056877E-16,-5.60383084497428E-34,
1.)) ;
#57484=DIRECTION('ref_axis',(-0.923879532511297,0.382683432365065,-1.40208427237264E-16)) ;
#57485=DIRECTION('',(-0.707106781186563,-0.707106781186532,-1.07310884363336E-16)) ;
#57486=DIRECTION('center_axis',(-1.51760508056877E-16,-5.60383084497428E-34,
1.)) ;
#57487=DIRECTION('ref_axis',(-0.382683432365031,0.923879532511311,-5.80762321206666E-17)) ;
#57488=DIRECTION('',(-1.,0.,-1.51760508056877E-16)) ;
#57489=DIRECTION('center_axis',(-1.51760508056877E-16,-5.60383084497428E-34,
1.)) ;
#57490=DIRECTION('ref_axis',(0.707106781186359,0.707106781186736,1.07310884363305E-16)) ;
#57491=DIRECTION('center_axis',(-1.51760508056877E-16,-5.60383084497428E-34,
1.)) ;
#57492=DIRECTION('ref_axis',(-0.707106781186485,0.70710678118661,-1.07310884363324E-16)) ;
#57493=DIRECTION('',(-1.,0.,-1.51760508056877E-16)) ;
#57494=DIRECTION('',(0.,-1.,-5.60383084497428E-34)) ;
#57495=DIRECTION('center_axis',(-1.51760508056877E-16,-5.60383084497428E-34,
1.)) ;
#57496=DIRECTION('ref_axis',(-0.707106781186485,0.70710678118661,-1.07310884363324E-16)) ;
#57497=DIRECTION('',(-1.,0.,-1.51760508056877E-16)) ;
#57498=DIRECTION('center_axis',(-1.51760508056877E-16,-5.60383084497428E-34,
1.)) ;
#57499=DIRECTION('ref_axis',(0.70710678118661,0.707106781186485,1.07310884363343E-16)) ;
#57500=DIRECTION('',(0.,1.,5.60383084497428E-34)) ;
#57501=DIRECTION('',(-1.,0.,-1.51760508056877E-16)) ;
#57502=DIRECTION('center_axis',(-1.51760508056877E-16,-5.60383084497428E-34,
1.)) ;
#57503=DIRECTION('ref_axis',(0.707106781186359,0.707106781186736,1.07310884363305E-16)) ;
#57504=DIRECTION('',(0.,1.,5.60383084497428E-34)) ;
#57505=DIRECTION('center_axis',(-1.51760508056877E-16,-5.60383084497428E-34,
1.)) ;
#57506=DIRECTION('ref_axis',(0.707106781186485,-0.70710678118661,1.07310884363324E-16)) ;
#57507=DIRECTION('',(1.,0.,1.51760508056877E-16)) ;
#57508=DIRECTION('center_axis',(-1.51760508056877E-16,-5.60383084497428E-34,
1.)) ;
#57509=DIRECTION('ref_axis',(-0.707106781186359,-0.707106781186736,-1.07310884363305E-16)) ;
#57510=DIRECTION('',(0.,-1.,-5.60383084497428E-34)) ;
#57511=DIRECTION('center_axis',(-1.51760508056877E-16,-5.60383084497428E-34,
1.)) ;
#57512=DIRECTION('ref_axis',(-0.873151649036935,0.487448661690728,-1.32509937868545E-16)) ;
#57513=DIRECTION('',(-1.,0.,-1.51760508056877E-16)) ;
#57514=DIRECTION('',(0.,-1.,-5.60383084497428E-34)) ;
#57515=DIRECTION('center_axis',(-1.51760508056877E-16,-5.60383084497428E-34,
1.)) ;
#57516=DIRECTION('ref_axis',(-0.707106781186485,0.70710678118661,-1.07310884363324E-16)) ;
#57517=DIRECTION('',(-1.,0.,-1.51760508056877E-16)) ;
#57518=DIRECTION('center_axis',(-1.51760508056877E-16,-5.60383084497428E-34,
1.)) ;
#57519=DIRECTION('ref_axis',(0.70710678118661,0.707106781186485,1.07310884363343E-16)) ;
#57520=DIRECTION('',(0.,1.,5.60383084497428E-34)) ;
#57521=DIRECTION('',(-1.,0.,-1.51760508056877E-16)) ;
#57522=DIRECTION('center_axis',(-1.51760508056877E-16,-5.60383084497428E-34,
1.)) ;
#57523=DIRECTION('ref_axis',(0.707106781186359,0.707106781186736,1.07310884363305E-16)) ;
#57524=DIRECTION('',(0.,1.,5.60383084497428E-34)) ;
#57525=DIRECTION('center_axis',(-1.51760508056877E-16,-5.60383084497428E-34,
1.)) ;
#57526=DIRECTION('ref_axis',(0.707106781186485,-0.70710678118661,1.07310884363324E-16)) ;
#57527=DIRECTION('',(1.,0.,1.51760508056877E-16)) ;
#57528=DIRECTION('center_axis',(-1.51760508056877E-16,-5.60383084497428E-34,
1.)) ;
#57529=DIRECTION('ref_axis',(-0.707106781186359,-0.707106781186736,-1.07310884363305E-16)) ;
#57530=DIRECTION('',(0.,-1.,-5.60383084497428E-34)) ;
#57531=DIRECTION('',(-7.105427357601E-15,-1.,-1.07888364883526E-30)) ;
#57532=DIRECTION('',(1.,0.,1.51760508056877E-16)) ;
#57533=DIRECTION('',(-3.17206578464327E-15,1.,-4.80833931982803E-31)) ;
#57534=DIRECTION('',(-1.,3.55271367880051E-14,-1.51760508056877E-16)) ;
#57535=DIRECTION('',(-7.105427357601E-15,-1.,-1.07888364883526E-30)) ;
#57536=DIRECTION('',(1.,-7.10542735760144E-15,1.51760508056877E-16)) ;
#57537=DIRECTION('center_axis',(-1.51760508056877E-16,-5.60383084497428E-34,
1.)) ;
#57538=DIRECTION('ref_axis',(-0.382683432365004,-0.923879532511322,-5.80762321206626E-17)) ;
#57539=DIRECTION('',(0.707106781186575,-0.70710678118652,1.07310884363338E-16)) ;
#57540=DIRECTION('center_axis',(-1.51760508056877E-16,-5.60383084497428E-34,
1.)) ;
#57541=DIRECTION('ref_axis',(-0.92387953251129,-0.382683432365082,-1.40208427237263E-16)) ;
#57542=DIRECTION('',(-3.73034936274055E-14,-1.,-5.66175752827605E-30)) ;
#57543=DIRECTION('center_axis',(-1.51760508056877E-16,-5.60383084497428E-34,
1.)) ;
#57544=DIRECTION('ref_axis',(-0.92387953251129,0.382683432365082,-1.40208427237263E-16)) ;
#57545=DIRECTION('',(-0.707106781186563,-0.707106781186532,-1.07310884363336E-16)) ;
#57546=DIRECTION('center_axis',(-1.51760508056877E-16,-5.60383084497428E-34,
1.)) ;
#57547=DIRECTION('ref_axis',(-0.382683432365031,0.923879532511311,-5.80762321206666E-17)) ;
#57548=DIRECTION('',(-1.,0.,-1.51760508056877E-16)) ;
#57549=DIRECTION('center_axis',(-1.51760508056877E-16,-5.60383084497428E-34,
1.)) ;
#57550=DIRECTION('ref_axis',(1.,2.24153233798966E-35,1.51760508056877E-16)) ;
#57551=DIRECTION('',(-1.1311821873082E-49,1.,5.60383084497428E-34)) ;
#57552=DIRECTION('center_axis',(-1.51760508056877E-16,-5.60383084497428E-34,
1.)) ;
#57553=DIRECTION('ref_axis',(-0.707106781186485,0.70710678118661,-1.07310884363324E-16)) ;
#57554=DIRECTION('',(-1.,0.,-1.51760508056877E-16)) ;
#57555=DIRECTION('center_axis',(-1.51760508056877E-16,-5.60383084497428E-34,
1.)) ;
#57556=DIRECTION('ref_axis',(0.382683432365058,0.9238795325113,5.80762321206707E-17)) ;
#57557=DIRECTION('',(-0.707106781186555,0.70710678118654,-1.07310884363335E-16)) ;
#57558=DIRECTION('center_axis',(-1.51760508056877E-16,-5.60383084497428E-34,
1.)) ;
#57559=DIRECTION('ref_axis',(0.923879532511287,0.38268343236509,1.40208427237263E-16)) ;
#57560=DIRECTION('',(-1.1311821873082E-49,1.,5.60383084497428E-34)) ;
#57561=DIRECTION('center_axis',(-1.51760508056877E-16,-5.60383084497428E-34,
1.)) ;
#57562=DIRECTION('ref_axis',(0.923879532511283,-0.382683432365099,1.40208427237262E-16)) ;
#57563=DIRECTION('',(0.707106781186555,0.70710678118654,1.07310884363335E-16)) ;
#57564=DIRECTION('center_axis',(-1.51760508056877E-16,-5.60383084497428E-34,
1.)) ;
#57565=DIRECTION('ref_axis',(0.382683432365031,-0.923879532511311,5.80762321206666E-17)) ;
#57566=DIRECTION('',(1.,0.,1.51760508056877E-16)) ;
#57567=DIRECTION('',(-1.1311821873082E-49,1.,5.60383084497428E-34)) ;
#57568=DIRECTION('',(-1.,-3.55271367880051E-14,-1.51760508056877E-16)) ;
#57569=DIRECTION('',(0.,-1.,-5.60383084497428E-34)) ;
#57570=DIRECTION('',(1.,0.,1.51760508056877E-16)) ;
#57571=DIRECTION('center_axis',(-1.4923676700635E-16,0.,1.)) ;
#57572=DIRECTION('ref_axis',(-1.,0.,-1.4923676700635E-16)) ;
#57573=DIRECTION('center_axis',(-1.4923676700635E-16,0.,1.)) ;
#57574=DIRECTION('ref_axis',(-1.,0.,-1.4923676700635E-16)) ;
#57575=DIRECTION('',(1.,1.77635683940026E-14,1.51760508056877E-16)) ;
#57576=DIRECTION('',(0.,1.,5.60383084497428E-34)) ;
#57577=DIRECTION('',(-1.,0.,-1.51760508056877E-16)) ;
#57578=DIRECTION('center_axis',(-1.51760508056877E-16,-5.60383084497428E-34,
1.)) ;
#57579=DIRECTION('ref_axis',(0.38268343236499,0.923879532511328,5.80762321206604E-17)) ;
#57580=DIRECTION('',(-0.707106781186555,0.70710678118654,-1.07310884363335E-16)) ;
#57581=DIRECTION('center_axis',(-1.51760508056877E-16,-5.60383084497428E-34,
1.)) ;
#57582=DIRECTION('ref_axis',(0.92387953251129,0.382683432365082,1.40208427237263E-16)) ;
#57583=DIRECTION('',(0.,1.,5.60383084497428E-34)) ;
#57584=DIRECTION('center_axis',(-1.51760508056877E-16,-5.60383084497428E-34,
1.)) ;
#57585=DIRECTION('ref_axis',(0.92387953251129,-0.382683432365082,1.40208427237263E-16)) ;
#57586=DIRECTION('',(0.707106781186555,0.70710678118654,1.07310884363335E-16)) ;
#57587=DIRECTION('center_axis',(-1.51760508056877E-16,-5.60383084497428E-34,
1.)) ;
#57588=DIRECTION('ref_axis',(0.382683432365017,-0.923879532511317,5.80762321206645E-17)) ;
#57589=DIRECTION('',(1.,0.,1.51760508056877E-16)) ;
#57590=DIRECTION('',(0.,1.,5.60383084497428E-34)) ;
#57591=DIRECTION('',(-1.,0.,-1.51760508056877E-16)) ;
#57592=DIRECTION('',(-3.17206578464331E-15,-1.,-4.81954698151804E-31)) ;
#57593=DIRECTION('center_axis',(-1.4923676700635E-16,0.,1.)) ;
#57594=DIRECTION('ref_axis',(-1.,0.,-1.4923676700635E-16)) ;
#57595=DIRECTION('center_axis',(-1.51760508056877E-16,-5.60383084497428E-34,
1.)) ;
#57596=DIRECTION('ref_axis',(1.,2.80191542248707E-35,1.51760508056877E-16)) ;
#57597=DIRECTION('center_axis',(-1.51760508056877E-16,-5.60383084497428E-34,
1.)) ;
#57598=DIRECTION('ref_axis',(-0.707106781186469,0.707106781186626,-1.07310884363322E-16)) ;
#57599=DIRECTION('',(-1.,0.,-1.51760508056877E-16)) ;
#57600=DIRECTION('center_axis',(-1.51760508056877E-16,-5.60383084497428E-34,
1.)) ;
#57601=DIRECTION('ref_axis',(0.707106781186485,0.70710678118661,1.07310884363324E-16)) ;
#57602=DIRECTION('',(-1.11022302462516E-15,1.,-1.67927627189059E-31)) ;
#57603=DIRECTION('center_axis',(-1.51760508056877E-16,-5.60383084497428E-34,
1.)) ;
#57604=DIRECTION('ref_axis',(0.707106781186485,-0.70710678118661,1.07310884363324E-16)) ;
#57605=DIRECTION('',(1.,0.,1.51760508056877E-16)) ;
#57606=DIRECTION('center_axis',(-1.51760508056877E-16,-5.60383084497428E-34,
1.)) ;
#57607=DIRECTION('ref_axis',(-0.707106781186485,-0.70710678118661,-1.07310884363324E-16)) ;
#57608=DIRECTION('',(-5.55111512312578E-16,-1.,-8.48043882212758E-32)) ;
#57609=DIRECTION('center_axis',(-1.51760508056877E-16,-5.60383084497428E-34,
1.)) ;
#57610=DIRECTION('ref_axis',(0.707106781186485,-0.70710678118661,1.07310884363324E-16)) ;
#57611=DIRECTION('',(1.,0.,1.51760508056877E-16)) ;
#57612=DIRECTION('center_axis',(-1.51760508056877E-16,-5.60383084497428E-34,
1.)) ;
#57613=DIRECTION('ref_axis',(-0.707106781186359,-0.707106781186736,-1.07310884363305E-16)) ;
#57614=DIRECTION('',(0.,-1.,-5.60383084497428E-34)) ;
#57615=DIRECTION('center_axis',(-1.51760508056877E-16,-5.60383084497428E-34,
1.)) ;
#57616=DIRECTION('ref_axis',(-0.707106781186485,0.70710678118661,-1.07310884363324E-16)) ;
#57617=DIRECTION('',(-1.,0.,-1.51760508056877E-16)) ;
#57618=DIRECTION('',(0.,-1.,-5.60383084497428E-34)) ;
#57619=DIRECTION('center_axis',(-1.51760508056877E-16,-5.60383084497428E-34,
1.)) ;
#57620=DIRECTION('ref_axis',(-0.707106781186485,0.70710678118661,-1.07310884363324E-16)) ;
#57621=DIRECTION('',(-1.,0.,-1.51760508056877E-16)) ;
#57622=DIRECTION('center_axis',(-1.51760508056877E-16,-5.60383084497428E-34,
1.)) ;
#57623=DIRECTION('ref_axis',(0.70710678118661,0.707106781186485,1.07310884363343E-16)) ;
#57624=DIRECTION('',(0.,1.,5.60383084497428E-34)) ;
#57625=DIRECTION('',(-1.,0.,-1.51760508056877E-16)) ;
#57626=DIRECTION('center_axis',(-1.51760508056877E-16,-5.60383084497428E-34,
1.)) ;
#57627=DIRECTION('ref_axis',(0.707106781186359,0.707106781186736,1.07310884363305E-16)) ;
#57628=DIRECTION('',(0.,1.,5.60383084497428E-34)) ;
#57629=DIRECTION('',(0.,-1.,-5.60383084497428E-34)) ;
#57630=DIRECTION('',(-1.,0.,-1.51760508056877E-16)) ;
#57631=DIRECTION('',(0.,1.,5.60383084497428E-34)) ;
#57632=DIRECTION('',(1.,0.,1.51760508056877E-16)) ;
#57633=DIRECTION('center_axis',(0.707106781186552,0.707106781186543,1.07310884363334E-16)) ;
#57634=DIRECTION('ref_axis',(0.499999999999936,-0.499999999999943,0.707106781186633)) ;
#57635=DIRECTION('center_axis',(-0.38268343236509,0.923879532511287,0.)) ;
#57636=DIRECTION('ref_axis',(-0.923879532511287,-0.38268343236509,-1.16152464241352E-16)) ;
#57637=DIRECTION('center_axis',(-1.,-5.23364152894628E-14,0.)) ;
#57638=DIRECTION('ref_axis',(5.23364152894628E-14,-1.,-1.51760508056887E-16)) ;
#57639=DIRECTION('center_axis',(-1.,0.,-1.51760508056877E-16)) ;
#57640=DIRECTION('ref_axis',(-1.07310884363329E-16,0.707106781186574,0.707106781186521)) ;
#57641=DIRECTION('center_axis',(-0.38268343236511,-0.923879532511278,0.)) ;
#57642=DIRECTION('ref_axis',(0.923879532511278,-0.38268343236511,1.64264390233177E-16)) ;
#57643=DIRECTION('center_axis',(0.707106781186552,-0.707106781186543,1.07310884363334E-16)) ;
#57644=DIRECTION('ref_axis',(-0.500000000000041,-0.500000000000047,0.707106781186485)) ;
#57645=DIRECTION('',(0.707106781186552,-0.707106781186543,1.07310884363334E-16)) ;
#57646=DIRECTION('center_axis',(0.707106781186543,0.707106781186552,0.)) ;
#57647=DIRECTION('ref_axis',(0.707106781186552,-0.707106781186543,1.25737296900294E-34)) ;
#57648=DIRECTION('center_axis',(0.,1.,5.60383084497428E-34)) ;
#57649=DIRECTION('ref_axis',(0.707106781186521,-3.9625067911038E-34,0.707106781186574)) ;
#57650=DIRECTION('center_axis',(-0.707106781186574,0.707106781186521,0.)) ;
#57651=DIRECTION('ref_axis',(-0.707106781186521,-0.707106781186574,-7.92501358220702E-34)) ;
#57652=DIRECTION('center_axis',(-0.707106781186574,-0.707106781186521,0.)) ;
#57653=DIRECTION('ref_axis',(0.707106781186521,-0.707106781186574,-7.92501358220702E-34)) ;
#57654=DIRECTION('center_axis',(-1.,0.,-1.51760508056877E-16)) ;
#57655=DIRECTION('ref_axis',(-1.07310884363329E-16,0.707106781186574,0.707106781186521)) ;
#57656=DIRECTION('center_axis',(-0.707106781186574,-0.707106781186521,0.)) ;
#57657=DIRECTION('ref_axis',(0.707106781186521,-0.707106781186574,2.14621768726675E-16)) ;
#57658=DIRECTION('center_axis',(0.,-1.,-5.60383084497428E-34)) ;
#57659=DIRECTION('ref_axis',(-0.707106781186574,-3.96250679110351E-34,0.707106781186521)) ;
#57660=DIRECTION('',(0.,-1.,-5.60383084497428E-34)) ;
#57661=DIRECTION('center_axis',(0.707106781186574,-0.707106781186521,0.)) ;
#57662=DIRECTION('ref_axis',(0.707106781186521,0.707106781186574,7.92501358220702E-34)) ;
#57663=DIRECTION('center_axis',(1.,0.,1.51760508056877E-16)) ;
#57664=DIRECTION('ref_axis',(-1.07310884363329E-16,-0.707106781186574,0.707106781186521)) ;
#57665=DIRECTION('',(1.,0.,1.51760508056877E-16)) ;
#57666=DIRECTION('center_axis',(0.,1.,0.)) ;
#57667=DIRECTION('ref_axis',(1.,0.,0.)) ;
#57668=DIRECTION('',(0.,0.,-1.)) ;
#57669=DIRECTION('center_axis',(-0.707106781186552,0.707106781186543,-1.07310884363334E-16)) ;
#57670=DIRECTION('ref_axis',(0.499999999999936,0.499999999999943,0.707106781186633)) ;
#57671=DIRECTION('center_axis',(-1.,-5.23364152894628E-14,7.40148683083464E-14)) ;
#57672=DIRECTION('ref_axis',(5.23364152894683E-14,-1.,7.41666288163964E-14)) ;
#57673=DIRECTION('center_axis',(-0.3826834323651,-0.923879532511283,0.)) ;
#57674=DIRECTION('ref_axis',(0.923879532511282,-0.3826834323651,1.16152464241351E-16)) ;
#57675=DIRECTION('center_axis',(-0.707106781186552,-0.707106781186543,-1.07310884363334E-16)) ;
#57676=DIRECTION('ref_axis',(-0.500000000000041,0.500000000000047,0.707106781186485)) ;
#57677=DIRECTION('center_axis',(0.38268343236508,-0.923879532511291,0.)) ;
#57678=DIRECTION('ref_axis',(0.923879532511291,0.38268343236508,1.16152464241352E-16)) ;
#57679=DIRECTION('center_axis',(1.,0.,1.51760508056877E-16)) ;
#57680=DIRECTION('ref_axis',(-1.07310884363329E-16,-0.707106781186574,0.707106781186521)) ;
#57681=DIRECTION('',(1.,0.,1.51760508056877E-16)) ;
#57682=DIRECTION('center_axis',(0.,1.,0.)) ;
#57683=DIRECTION('ref_axis',(1.,0.,1.77819390572528E-34)) ;
#57684=DIRECTION('center_axis',(1.,0.,0.)) ;
#57685=DIRECTION('ref_axis',(0.,-1.,0.)) ;
#57686=DIRECTION('',(0.,0.,-1.)) ;
#57687=DIRECTION('',(0.,0.,-1.)) ;
#57688=DIRECTION('',(0.,0.,-1.)) ;
#57689=DIRECTION('center_axis',(1.4923676700635E-16,0.,-1.)) ;
#57690=DIRECTION('ref_axis',(-1.,0.,0.)) ;
#57691=DIRECTION('center_axis',(-1.4923676700635E-16,0.,1.)) ;
#57692=DIRECTION('ref_axis',(1.,0.,1.4923676700635E-16)) ;
#57693=DIRECTION('center_axis',(0.,-1.,0.)) ;
#57694=DIRECTION('ref_axis',(1.,0.,0.)) ;
#57695=DIRECTION('center_axis',(1.4923676700635E-16,0.,-1.)) ;
#57696=DIRECTION('ref_axis',(1.,0.,1.4923676700635E-16)) ;
#57697=DIRECTION('center_axis',(-1.4923676700635E-16,0.,1.)) ;
#57698=DIRECTION('ref_axis',(1.,0.,1.4923676700635E-16)) ;
#57699=DIRECTION('center_axis',(-1.4923676700635E-16,0.,1.)) ;
#57700=DIRECTION('ref_axis',(1.,0.,1.4923676700635E-16)) ;
#57701=DIRECTION('center_axis',(-1.4923676700635E-16,0.,1.)) ;
#57702=DIRECTION('ref_axis',(1.,0.,1.4923676700635E-16)) ;
#57703=DIRECTION('center_axis',(0.,0.,1.)) ;
#57704=DIRECTION('ref_axis',(1.,0.,0.)) ;
#57705=DIRECTION('',(0.,0.,1.)) ;
#57706=DIRECTION('center_axis',(1.4923676700635E-16,0.,-1.)) ;
#57707=DIRECTION('ref_axis',(1.,0.,1.4923676700635E-16)) ;
#57708=DIRECTION('center_axis',(-1.4923676700635E-16,0.,1.)) ;
#57709=DIRECTION('ref_axis',(1.,0.,0.)) ;
#57710=DIRECTION('center_axis',(1.4923676700635E-16,0.,-1.)) ;
#57711=DIRECTION('ref_axis',(1.,0.,1.4923676700635E-16)) ;
#57712=DIRECTION('center_axis',(0.,-1.,0.)) ;
#57713=DIRECTION('ref_axis',(-1.,0.,0.)) ;
#57714=DIRECTION('center_axis',(0.,0.,1.)) ;
#57715=DIRECTION('ref_axis',(1.,0.,0.)) ;
#57716=DIRECTION('center_axis',(-1.51760508056877E-16,-5.60383084497428E-34,
1.)) ;
#57717=DIRECTION('ref_axis',(1.,1.86794361499138E-35,1.51760508056877E-16)) ;
#57718=DIRECTION('',(0.,0.,-1.)) ;
#57719=DIRECTION('center_axis',(-1.51760508056877E-16,-5.60383084497428E-34,
1.)) ;
#57720=DIRECTION('ref_axis',(1.,0.,0.)) ;
#57721=DIRECTION('center_axis',(1.51760508056877E-16,5.60383084497428E-34,
-1.)) ;
#57722=DIRECTION('ref_axis',(1.,1.86794361499138E-35,1.51760508056877E-16)) ;
#57723=DIRECTION('center_axis',(0.,1.,5.60383084497428E-34)) ;
#57724=DIRECTION('ref_axis',(-1.,0.,0.)) ;
#57725=DIRECTION('center_axis',(-1.51760508056877E-16,-5.60383084497428E-34,
1.)) ;
#57726=DIRECTION('ref_axis',(1.,1.81422958079369E-66,1.51760508056877E-16)) ;
#57727=DIRECTION('',(-1.,0.,-1.51760508056877E-16)) ;
#57728=DIRECTION('center_axis',(1.51760508056877E-16,5.60383084497428E-34,
-1.)) ;
#57729=DIRECTION('ref_axis',(-0.707106781186614,0.707106781186481,-1.07310884363344E-16)) ;
#57730=DIRECTION('',(-1.1311821873082E-49,1.,5.60383084497428E-34)) ;
#57731=DIRECTION('',(-1.,0.,-1.51760508056877E-16)) ;
#57732=DIRECTION('',(1.1311821873082E-49,-1.,-5.60383084497428E-34)) ;
#57733=DIRECTION('',(1.1311821873082E-49,-1.,-5.60383084497428E-34)) ;
#57734=DIRECTION('',(-1.,0.,-1.51760508056877E-16)) ;
#57735=DIRECTION('center_axis',(1.51760508056877E-16,5.60383084497428E-34,
-1.)) ;
#57736=DIRECTION('ref_axis',(0.382683432365032,-0.923879532511311,5.80762321206668E-17)) ;
#57737=DIRECTION('',(-0.707106781186555,-0.70710678118654,-1.07310884363335E-16)) ;
#57738=DIRECTION('center_axis',(1.51760508056877E-16,5.60383084497428E-34,
-1.)) ;
#57739=DIRECTION('ref_axis',(0.923879532511313,-0.382683432365025,1.40208427237267E-16)) ;
#57740=DIRECTION('',(1.1311821873082E-49,-1.,-5.60383084497428E-34)) ;
#57741=DIRECTION('center_axis',(1.51760508056877E-16,5.60383084497428E-34,
-1.)) ;
#57742=DIRECTION('ref_axis',(0.923879532511313,0.382683432365025,1.40208427237267E-16)) ;
#57743=DIRECTION('',(0.707106781186555,-0.70710678118654,1.07310884363335E-16)) ;
#57744=DIRECTION('',(-1.,0.,-1.51760508056877E-16)) ;
#57745=DIRECTION('center_axis',(-1.51760508056877E-16,-5.60383084497428E-34,
1.)) ;
#57746=DIRECTION('ref_axis',(1.19824467136135E-15,-1.,1.81285837017747E-31)) ;
#57747=DIRECTION('',(1.,-3.19495806435525E-17,1.51760508056877E-16)) ;
#57748=DIRECTION('center_axis',(-1.51760508056877E-16,-5.60383084497428E-34,
1.)) ;
#57749=DIRECTION('ref_axis',(8.7871275899832E-16,-1.,1.32793511657148E-31)) ;
#57750=DIRECTION('',(0.,1.,5.60383084497428E-34)) ;
#57751=DIRECTION('',(-1.,0.,-1.51760508056877E-16)) ;
#57752=DIRECTION('',(0.,1.,5.60383084497428E-34)) ;
#57753=DIRECTION('center_axis',(-1.51760508056877E-16,-5.60383084497428E-34,
1.)) ;
#57754=DIRECTION('ref_axis',(1.67754253990588E-15,-1.,2.54024325058643E-31)) ;
#57755=DIRECTION('',(1.,-3.19495806435525E-17,1.51760508056877E-16)) ;
#57756=DIRECTION('center_axis',(-1.51760508056877E-16,-5.60383084497428E-34,
1.)) ;
#57757=DIRECTION('ref_axis',(7.18946802816807E-16,-1.,1.08547348976849E-31)) ;
#57758=DIRECTION('',(-1.,0.,-1.51760508056877E-16)) ;
#57759=DIRECTION('',(0.,1.,5.60383084497428E-34)) ;
#57760=DIRECTION('center_axis',(1.51760508056877E-16,5.60383084497428E-34,
-1.)) ;
#57761=DIRECTION('ref_axis',(-0.923879532511284,-0.382683432365097,-1.40208427237262E-16)) ;
#57762=DIRECTION('',(-0.707106781186615,0.70710678118648,-1.07310884363344E-16)) ;
#57763=DIRECTION('center_axis',(-1.51760508056877E-16,-5.60383084497428E-34,
1.)) ;
#57764=DIRECTION('ref_axis',(0.923879532511263,0.382683432365148,1.40208427237259E-16)) ;
#57765=DIRECTION('',(-6.83214169000096E-16,1.,-1.03124546314615E-31)) ;
#57766=DIRECTION('center_axis',(-1.51760508056877E-16,-5.60383084497428E-34,
1.)) ;
#57767=DIRECTION('ref_axis',(0.718421208107084,-0.695608343640269,1.09027967541166E-16)) ;
#57768=DIRECTION('center_axis',(1.51760508056877E-16,5.60383084497428E-34,
-1.)) ;
#57769=DIRECTION('ref_axis',(-0.718421208107087,0.695608343640265,-1.09027967541167E-16)) ;
#57770=DIRECTION('',(0.,1.,5.60383084497428E-34)) ;
#57771=DIRECTION('center_axis',(1.51760508056877E-16,5.60383084497428E-34,
-1.)) ;
#57772=DIRECTION('ref_axis',(-0.718421208107092,-0.69560834364026,-1.09027967541168E-16)) ;
#57773=DIRECTION('center_axis',(-1.51760508056877E-16,-5.60383084497428E-34,
1.)) ;
#57774=DIRECTION('ref_axis',(0.718421208107098,0.695608343640254,1.09027967541169E-16)) ;
#57775=DIRECTION('',(-6.83214169000096E-16,1.,-1.03124546314615E-31)) ;
#57776=DIRECTION('center_axis',(-1.51760508056877E-16,-5.60383084497428E-34,
1.)) ;
#57777=DIRECTION('ref_axis',(0.923879532511288,-0.382683432365087,1.40208427237263E-16)) ;
#57778=DIRECTION('',(0.707106781186521,0.707106781186574,1.0731088436333E-16)) ;
#57779=DIRECTION('center_axis',(1.51760508056877E-16,5.60383084497428E-34,
-1.)) ;
#57780=DIRECTION('ref_axis',(-0.923879532511292,0.382683432365076,-1.40208427237264E-16)) ;
#57781=DIRECTION('',(-5.23472275150178E-15,1.,-7.93863801220309E-31)) ;
#57782=DIRECTION('center_axis',(-1.51760508056877E-16,-5.60383084497428E-34,
1.)) ;
#57783=DIRECTION('ref_axis',(0.642787609686539,-0.766044443118978,9.75497742186947E-17)) ;
#57784=DIRECTION('',(0.984807753012209,-0.173648177666924,1.49454924935485E-16)) ;
#57785=DIRECTION('center_axis',(-1.51760508056877E-16,-5.60383084497428E-34,
1.)) ;
#57786=DIRECTION('ref_axis',(-0.537299608346822,-0.843391445812887,-8.15408615414747E-17)) ;
#57787=DIRECTION('',(0.573576436351042,-0.819152044288994,8.70462513900874E-17)) ;
#57788=DIRECTION('center_axis',(-1.51760508056877E-16,-5.60383084497428E-34,
1.)) ;
#57789=DIRECTION('ref_axis',(-0.953716950748229,-0.300705799504266,-1.44736568988007E-16)) ;
#57790=DIRECTION('',(-5.25359141716359E-35,-1.,-5.60383084497428E-34)) ;
#57791=DIRECTION('center_axis',(1.51760508056877E-16,5.60383084497428E-34,
-1.)) ;
#57792=DIRECTION('ref_axis',(0.707106781186547,0.707106781186547,1.07310884363333E-16)) ;
#57793=DIRECTION('',(1.,0.,1.51760508056877E-16)) ;
#57794=DIRECTION('center_axis',(-1.51760508056877E-16,-5.60383084497428E-34,
1.)) ;
#57795=DIRECTION('ref_axis',(-0.707106781186548,-0.707106781186548,-1.07310884363333E-16)) ;
#57796=DIRECTION('',(-2.22044604925032E-15,-1.,-3.37536403631613E-31)) ;
#57797=DIRECTION('',(-1.,0.,-1.51760508056877E-16)) ;
#57798=DIRECTION('',(-2.33146835171284E-14,1.,-3.53768783266021E-30)) ;
#57799=DIRECTION('center_axis',(-1.51760508056877E-16,-5.60383084497428E-34,
1.)) ;
#57800=DIRECTION('ref_axis',(0.707106781186544,-0.707106781186551,1.07310884363333E-16)) ;
#57801=DIRECTION('',(1.,0.,1.51760508056877E-16)) ;
#57802=DIRECTION('center_axis',(-1.51760508056877E-16,-5.60383084497428E-34,
1.)) ;
#57803=DIRECTION('ref_axis',(-0.70710678118657,-0.707106781186525,-1.07310884363337E-16)) ;
#57804=DIRECTION('',(2.22044604925031E-16,-1.,3.31372189702139E-32)) ;
#57805=DIRECTION('center_axis',(1.51760508056877E-16,5.60383084497428E-34,
-1.)) ;
#57806=DIRECTION('ref_axis',(1.,1.86794361499143E-34,1.51760508056877E-16)) ;
#57807=DIRECTION('',(1.,0.,1.51760508056877E-16)) ;
#57808=DIRECTION('',(0.,-1.,-5.60383084497428E-34)) ;
#57809=DIRECTION('center_axis',(1.51760508056877E-16,5.60383084497428E-34,
-1.)) ;
#57810=DIRECTION('ref_axis',(0.707106781186592,0.707106781186503,1.0731088436334E-16)) ;
#57811=DIRECTION('',(1.,0.,1.51760508056877E-16)) ;
#57812=DIRECTION('center_axis',(1.51760508056877E-16,5.60383084497428E-34,
-1.)) ;
#57813=DIRECTION('ref_axis',(-0.707106781186592,0.707106781186503,-1.0731088436334E-16)) ;
#57814=DIRECTION('',(0.,1.,5.60383084497428E-34)) ;
#57815=DIRECTION('',(1.,0.,1.51760508056877E-16)) ;
#57816=DIRECTION('center_axis',(1.51760508056877E-16,5.60383084497428E-34,
-1.)) ;
#57817=DIRECTION('ref_axis',(-0.707106781186592,0.707106781186503,-1.0731088436334E-16)) ;
#57818=DIRECTION('',(0.,1.,5.60383084497428E-34)) ;
#57819=DIRECTION('center_axis',(1.51760508056877E-16,5.60383084497428E-34,
-1.)) ;
#57820=DIRECTION('ref_axis',(-0.707106781186592,-0.707106781186503,-1.0731088436334E-16)) ;
#57821=DIRECTION('',(-1.,0.,-1.51760508056877E-16)) ;
#57822=DIRECTION('center_axis',(1.51760508056877E-16,5.60383084497428E-34,
-1.)) ;
#57823=DIRECTION('ref_axis',(0.707106781186592,-0.707106781186503,1.0731088436334E-16)) ;
#57824=DIRECTION('',(0.,-1.,-5.60383084497428E-34)) ;
#57825=DIRECTION('center_axis',(1.51760508056877E-16,5.60383084497428E-34,
-1.)) ;
#57826=DIRECTION('ref_axis',(0.707106781186592,0.707106781186503,1.0731088436334E-16)) ;
#57827=DIRECTION('center_axis',(1.51760508056877E-16,5.60383084497428E-34,
-1.)) ;
#57828=DIRECTION('ref_axis',(1.,-2.24153233798967E-35,1.51760508056877E-16)) ;
#57829=DIRECTION('center_axis',(-1.51760508056877E-16,-5.60383084497428E-34,
1.)) ;
#57830=DIRECTION('ref_axis',(1.,-8.50440216098095E-50,1.51760508056877E-16)) ;
#57831=DIRECTION('',(-1.,0.,-1.51760508056877E-16)) ;
#57832=DIRECTION('',(-7.105427357601E-15,-1.,-1.07888364883526E-30)) ;
#57833=DIRECTION('center_axis',(1.51760508056877E-16,5.60383084497428E-34,
-1.)) ;
#57834=DIRECTION('ref_axis',(0.707106781186359,0.707106781186736,1.07310884363305E-16)) ;
#57835=DIRECTION('',(1.,0.,1.51760508056877E-16)) ;
#57836=DIRECTION('center_axis',(1.51760508056877E-16,5.60383084497428E-34,
-1.)) ;
#57837=DIRECTION('ref_axis',(-0.38268343236507,0.923879532511295,-5.80762321206726E-17)) ;
#57838=DIRECTION('',(0.707106781186563,0.707106781186532,1.07310884363336E-16)) ;
#57839=DIRECTION('center_axis',(1.51760508056877E-16,5.60383084497428E-34,
-1.)) ;
#57840=DIRECTION('ref_axis',(-0.923879532511313,0.382683432365025,-1.40208427237267E-16)) ;
#57841=DIRECTION('',(3.73034936274055E-14,1.,5.66175752827605E-30)) ;
#57842=DIRECTION('center_axis',(1.51760508056877E-16,5.60383084497428E-34,
-1.)) ;
#57843=DIRECTION('ref_axis',(-0.923879532511313,-0.382683432365025,-1.40208427237267E-16)) ;
#57844=DIRECTION('',(-0.707106781186575,0.70710678118652,-1.07310884363338E-16)) ;
#57845=DIRECTION('center_axis',(1.51760508056877E-16,5.60383084497428E-34,
-1.)) ;
#57846=DIRECTION('ref_axis',(-0.382683432364994,-0.923879532511326,-5.8076232120661E-17)) ;
#57847=DIRECTION('',(-1.,7.10542735760144E-15,-1.51760508056877E-16)) ;
#57848=DIRECTION('center_axis',(1.51760508056877E-16,5.60383084497428E-34,
-1.)) ;
#57849=DIRECTION('ref_axis',(0.707106781186485,-0.70710678118661,1.07310884363324E-16)) ;
#57850=DIRECTION('',(-7.105427357601E-15,-1.,-1.07888364883526E-30)) ;
#57851=DIRECTION('',(1.,-3.55271367880051E-14,1.51760508056877E-16)) ;
#57852=DIRECTION('',(7.105427357601E-15,1.,1.07888364883526E-30)) ;
#57853=DIRECTION('center_axis',(-1.51760508056877E-16,-5.60383084497428E-34,
1.)) ;
#57854=DIRECTION('ref_axis',(1.,-8.50440216098095E-50,1.51760508056877E-16)) ;
#57855=DIRECTION('',(-1.,0.,-1.51760508056877E-16)) ;
#57856=DIRECTION('center_axis',(1.51760508056877E-16,5.60383084497428E-34,
-1.)) ;
#57857=DIRECTION('ref_axis',(-0.382683432365099,0.923879532511283,-5.80762321206769E-17)) ;
#57858=DIRECTION('',(0.707106781186563,0.707106781186532,1.07310884363336E-16)) ;
#57859=DIRECTION('center_axis',(1.51760508056877E-16,5.60383084497428E-34,
-1.)) ;
#57860=DIRECTION('ref_axis',(-0.923879532511297,0.382683432365065,-1.40208427237264E-16)) ;
#57861=DIRECTION('',(-3.73034936274055E-14,-1.,-5.66175752827605E-30)) ;
#57862=DIRECTION('center_axis',(1.51760508056877E-16,5.60383084497428E-34,
-1.)) ;
#57863=DIRECTION('ref_axis',(-0.923879532511297,-0.382683432365065,-1.40208427237264E-16)) ;
#57864=DIRECTION('',(-0.707106781186544,0.707106781186551,-1.07310884363333E-16)) ;
#57865=DIRECTION('center_axis',(1.51760508056877E-16,5.60383084497428E-34,
-1.)) ;
#57866=DIRECTION('ref_axis',(-0.382683432365045,-0.923879532511305,-5.80762321206688E-17)) ;
#57867=DIRECTION('',(1.,-7.10542735760144E-15,1.51760508056877E-16)) ;
#57868=DIRECTION('center_axis',(1.51760508056877E-16,5.60383084497428E-34,
-1.)) ;
#57869=DIRECTION('ref_axis',(0.707106781186548,-0.707106781186548,1.07310884363333E-16)) ;
#57870=DIRECTION('',(7.105427357601E-15,1.,1.07888364883526E-30)) ;
#57871=DIRECTION('',(7.105427357601E-15,1.,1.07888364883526E-30)) ;
#57872=DIRECTION('',(7.105427357601E-15,1.,1.07888364883526E-30)) ;
#57873=DIRECTION('center_axis',(1.51760508056877E-16,5.60383084497428E-34,
-1.)) ;
#57874=DIRECTION('ref_axis',(0.707106781186296,0.707106781186799,1.07310884363295E-16)) ;
#57875=DIRECTION('center_axis',(1.51760508056877E-16,5.60383084497428E-34,
-1.)) ;
#57876=DIRECTION('ref_axis',(-0.707106781186469,0.707106781186626,-1.07310884363321E-16)) ;
#57877=DIRECTION('',(5.55111512312578E-16,1.,8.48043882212758E-32)) ;
#57878=DIRECTION('center_axis',(1.51760508056877E-16,5.60383084497428E-34,
-1.)) ;
#57879=DIRECTION('ref_axis',(-0.707106781186485,-0.70710678118661,-1.07310884363324E-16)) ;
#57880=DIRECTION('',(-1.,0.,-1.51760508056877E-16)) ;
#57881=DIRECTION('center_axis',(1.51760508056877E-16,5.60383084497428E-34,
-1.)) ;
#57882=DIRECTION('ref_axis',(0.707106781186485,-0.70710678118661,1.07310884363324E-16)) ;
#57883=DIRECTION('',(1.11022302462516E-15,-1.,1.67927627189059E-31)) ;
#57884=DIRECTION('center_axis',(1.51760508056877E-16,5.60383084497428E-34,
-1.)) ;
#57885=DIRECTION('ref_axis',(0.707106781186485,0.70710678118661,1.07310884363324E-16)) ;
#57886=DIRECTION('',(1.,0.,1.51760508056877E-16)) ;
#57887=DIRECTION('',(0.,-1.,-5.60383084497428E-34)) ;
#57888=DIRECTION('',(0.,-1.,-5.60383084497428E-34)) ;
#57889=DIRECTION('',(0.,-1.,-5.60383084497428E-34)) ;
#57890=DIRECTION('',(-1.,0.,-1.51760508056877E-16)) ;
#57891=DIRECTION('center_axis',(1.51760508056877E-16,5.60383084497428E-34,
-1.)) ;
#57892=DIRECTION('ref_axis',(0.382683432364994,-0.923879532511326,5.8076232120661E-17)) ;
#57893=DIRECTION('',(-0.707106781186555,-0.70710678118654,-1.07310884363335E-16)) ;
#57894=DIRECTION('center_axis',(1.51760508056877E-16,5.60383084497428E-34,
-1.)) ;
#57895=DIRECTION('ref_axis',(0.923879532511313,-0.382683432365025,1.40208427237267E-16)) ;
#57896=DIRECTION('',(0.,-1.,-5.60383084497428E-34)) ;
#57897=DIRECTION('center_axis',(1.51760508056877E-16,5.60383084497428E-34,
-1.)) ;
#57898=DIRECTION('ref_axis',(0.923879532511313,0.382683432365025,1.40208427237267E-16)) ;
#57899=DIRECTION('',(0.707106781186555,-0.70710678118654,1.07310884363335E-16)) ;
#57900=DIRECTION('center_axis',(1.51760508056877E-16,5.60383084497428E-34,
-1.)) ;
#57901=DIRECTION('ref_axis',(0.382683432364994,0.923879532511326,5.8076232120661E-17)) ;
#57902=DIRECTION('',(1.,0.,1.51760508056877E-16)) ;
#57903=DIRECTION('',(-1.,0.,-1.51760508056877E-16)) ;
#57904=DIRECTION('',(0.,1.,5.60383084497428E-34)) ;
#57905=DIRECTION('',(1.,0.,1.51760508056877E-16)) ;
#57906=DIRECTION('center_axis',(1.51760508056877E-16,5.60383084497428E-34,
-1.)) ;
#57907=DIRECTION('ref_axis',(-0.87315164903695,0.487448661690701,-1.32509937868548E-16)) ;
#57908=DIRECTION('',(0.,1.,5.60383084497428E-34)) ;
#57909=DIRECTION('center_axis',(1.51760508056877E-16,5.60383084497428E-34,
-1.)) ;
#57910=DIRECTION('ref_axis',(-0.707106781186359,-0.707106781186736,-1.07310884363305E-16)) ;
#57911=DIRECTION('',(-1.,0.,-1.51760508056877E-16)) ;
#57912=DIRECTION('center_axis',(1.51760508056877E-16,5.60383084497428E-34,
-1.)) ;
#57913=DIRECTION('ref_axis',(0.873151649036935,-0.487448661690728,1.32509937868545E-16)) ;
#57914=DIRECTION('',(0.,-1.,-5.60383084497428E-34)) ;
#57915=DIRECTION('center_axis',(1.51760508056877E-16,5.60383084497428E-34,
-1.)) ;
#57916=DIRECTION('ref_axis',(0.873151649036842,0.487448661690894,1.32509937868531E-16)) ;
#57917=DIRECTION('',(1.,0.,1.51760508056877E-16)) ;
#57918=DIRECTION('',(0.,-1.,-5.60383084497428E-34)) ;
#57919=DIRECTION('center_axis',(1.51760508056877E-16,5.60383084497428E-34,
-1.)) ;
#57920=DIRECTION('ref_axis',(-0.87315164903695,0.487448661690701,-1.32509937868548E-16)) ;
#57921=DIRECTION('',(0.,1.,5.60383084497428E-34)) ;
#57922=DIRECTION('center_axis',(1.51760508056877E-16,5.60383084497428E-34,
-1.)) ;
#57923=DIRECTION('ref_axis',(-0.873151649036905,-0.487448661690782,-1.32509937868541E-16)) ;
#57924=DIRECTION('',(-1.,0.,-1.51760508056877E-16)) ;
#57925=DIRECTION('center_axis',(1.51760508056877E-16,5.60383084497428E-34,
-1.)) ;
#57926=DIRECTION('ref_axis',(0.873151649036766,-0.48744866169103,1.3250993786852E-16)) ;
#57927=DIRECTION('',(0.,-1.,-5.60383084497428E-34)) ;
#57928=DIRECTION('center_axis',(1.51760508056877E-16,5.60383084497428E-34,
-1.)) ;
#57929=DIRECTION('ref_axis',(0.873151649036827,0.487448661690921,1.32509937868529E-16)) ;
#57930=DIRECTION('',(1.,0.,1.51760508056877E-16)) ;
#57931=DIRECTION('',(0.,-1.,-5.60383084497428E-34)) ;
#57932=DIRECTION('center_axis',(1.51760508056877E-16,5.60383084497428E-34,
-1.)) ;
#57933=DIRECTION('ref_axis',(0.707106781186592,0.707106781186503,1.0731088436334E-16)) ;
#57934=DIRECTION('',(1.,0.,1.51760508056877E-16)) ;
#57935=DIRECTION('center_axis',(1.51760508056877E-16,5.60383084497428E-34,
-1.)) ;
#57936=DIRECTION('ref_axis',(-0.707106781186636,0.707106781186459,-1.07310884363347E-16)) ;
#57937=DIRECTION('',(0.,1.,5.60383084497428E-34)) ;
#57938=DIRECTION('',(1.,0.,1.51760508056877E-16)) ;
#57939=DIRECTION('center_axis',(1.51760508056877E-16,5.60383084497428E-34,
-1.)) ;
#57940=DIRECTION('ref_axis',(-0.87315164903695,0.487448661690701,-1.32509937868548E-16)) ;
#57941=DIRECTION('',(0.,1.,5.60383084497428E-34)) ;
#57942=DIRECTION('center_axis',(1.51760508056877E-16,5.60383084497428E-34,
-1.)) ;
#57943=DIRECTION('ref_axis',(-0.873151649036905,-0.487448661690782,-1.32509937868541E-16)) ;
#57944=DIRECTION('',(-1.,0.,-1.51760508056877E-16)) ;
#57945=DIRECTION('center_axis',(1.51760508056877E-16,5.60383084497428E-34,
-1.)) ;
#57946=DIRECTION('ref_axis',(0.873151649036766,-0.48744866169103,1.3250993786852E-16)) ;
#57947=DIRECTION('',(0.,-1.,-5.60383084497428E-34)) ;
#57948=DIRECTION('center_axis',(1.51760508056877E-16,5.60383084497428E-34,
-1.)) ;
#57949=DIRECTION('ref_axis',(0.873151649036935,0.487448661690728,1.32509937868545E-16)) ;
#57950=DIRECTION('',(1.,0.,1.51760508056877E-16)) ;
#57951=DIRECTION('',(0.,-1.,-5.60383084497428E-34)) ;
#57952=DIRECTION('center_axis',(1.51760508056877E-16,5.60383084497428E-34,
-1.)) ;
#57953=DIRECTION('ref_axis',(0.707106781186592,0.707106781186503,1.0731088436334E-16)) ;
#57954=DIRECTION('',(1.,0.,1.51760508056877E-16)) ;
#57955=DIRECTION('center_axis',(1.51760508056877E-16,5.60383084497428E-34,
-1.)) ;
#57956=DIRECTION('ref_axis',(-0.707106781186592,0.707106781186503,-1.0731088436334E-16)) ;
#57957=DIRECTION('',(0.,1.,5.60383084497428E-34)) ;
#57958=DIRECTION('',(1.,0.,1.51760508056877E-16)) ;
#57959=DIRECTION('center_axis',(-1.,-2.22044604925031E-16,0.)) ;
#57960=DIRECTION('ref_axis',(0.,0.,1.)) ;
#57961=DIRECTION('center_axis',(0.,0.,1.)) ;
#57962=DIRECTION('ref_axis',(-1.,0.,0.)) ;
#57963=DIRECTION('center_axis',(-1.,0.,-1.11022302462517E-14)) ;
#57964=DIRECTION('ref_axis',(-1.11022302462517E-14,0.,1.)) ;
#57965=DIRECTION('center_axis',(0.,1.,0.)) ;
#57966=DIRECTION('ref_axis',(-0.707106781186548,0.,-0.707106781186548)) ;
#57967=DIRECTION('center_axis',(-1.,-2.22044604925031E-16,0.)) ;
#57968=DIRECTION('ref_axis',(-1.47241706008224E-16,0.663117692312033,0.748515147570685)) ;
#57969=DIRECTION('center_axis',(0.,0.,1.)) ;
#57970=DIRECTION('ref_axis',(-0.707106781186391,-0.707106781186704,0.)) ;
#57971=DIRECTION('center_axis',(0.,0.,1.)) ;
#57972=DIRECTION('ref_axis',(-1.,0.,0.)) ;
#57973=DIRECTION('',(0.,0.,1.)) ;
#57974=DIRECTION('',(0.,0.,-1.)) ;
#57975=DIRECTION('center_axis',(0.,1.,0.)) ;
#57976=DIRECTION('ref_axis',(0.,0.,1.)) ;
#57977=DIRECTION('center_axis',(-1.,0.,-4.44089209850043E-14)) ;
#57978=DIRECTION('ref_axis',(4.44089209850043E-14,0.,-1.)) ;
#57979=DIRECTION('center_axis',(0.,1.,0.)) ;
#57980=DIRECTION('ref_axis',(-0.707106781186549,0.,-0.707106781186546)) ;
#57981=DIRECTION('center_axis',(0.,-1.,0.)) ;
#57982=DIRECTION('ref_axis',(-0.707106781186549,0.,-0.707106781186546)) ;
#57983=DIRECTION('center_axis',(-1.,0.,-1.51760508056877E-16)) ;
#57984=DIRECTION('ref_axis',(1.07310884363305E-16,-0.707106781186736,-0.707106781186359)) ;
#57985=DIRECTION('center_axis',(-1.,0.,0.)) ;
#57986=DIRECTION('ref_axis',(0.,0.,-1.)) ;
#57987=DIRECTION('',(-1.,0.,-1.51760508056877E-16)) ;
#57988=DIRECTION('',(1.,0.,1.51760508056877E-16)) ;
#57989=DIRECTION('center_axis',(0.,1.,0.)) ;
#57990=DIRECTION('ref_axis',(0.,0.,1.)) ;
#57991=DIRECTION('center_axis',(0.,0.,-1.)) ;
#57992=DIRECTION('ref_axis',(1.,0.,0.)) ;
#57993=DIRECTION('center_axis',(0.,1.,0.)) ;
#57994=DIRECTION('ref_axis',(0.707106781186548,0.,-0.707106781186548)) ;
#57995=DIRECTION('center_axis',(0.,-1.,0.)) ;
#57996=DIRECTION('ref_axis',(0.707106781186548,0.,-0.707106781186548)) ;
#57997=DIRECTION('center_axis',(-8.7076315656875E-16,0.,1.)) ;
#57998=DIRECTION('ref_axis',(0.707106781186391,-0.707106781186704,6.1572253281703E-16)) ;
#57999=DIRECTION('center_axis',(0.,0.,-1.)) ;
#58000=DIRECTION('ref_axis',(1.,0.,0.)) ;
#58001=DIRECTION('',(8.7076315656875E-16,0.,-1.)) ;
#58002=DIRECTION('',(-8.7076315656875E-16,0.,1.)) ;
#58003=DIRECTION('center_axis',(0.,1.,0.)) ;
#58004=DIRECTION('ref_axis',(0.,0.,1.)) ;
#58005=DIRECTION('center_axis',(0.,0.,1.)) ;
#58006=DIRECTION('ref_axis',(-1.,0.,0.)) ;
#58007=DIRECTION('center_axis',(0.,-1.,0.)) ;
#58008=DIRECTION('ref_axis',(0.,0.,1.)) ;
#58009=DIRECTION('center_axis',(0.,1.,0.)) ;
#58010=DIRECTION('ref_axis',(0.,0.,1.)) ;
#58011=DIRECTION('center_axis',(0.,0.,-1.)) ;
#58012=DIRECTION('ref_axis',(-0.707106781186359,-0.707106781186736,0.)) ;
#58013=DIRECTION('center_axis',(0.,0.,1.)) ;
#58014=DIRECTION('ref_axis',(-1.,0.,0.)) ;
#58015=DIRECTION('',(0.,0.,1.)) ;
#58016=DIRECTION('',(0.,0.,-1.)) ;
#58017=DIRECTION('center_axis',(0.,1.,0.)) ;
#58018=DIRECTION('ref_axis',(0.,0.,1.)) ;
#58019=DIRECTION('center_axis',(-1.,0.,0.)) ;
#58020=DIRECTION('ref_axis',(0.,0.,-1.)) ;
#58021=DIRECTION('center_axis',(0.,1.,0.)) ;
#58022=DIRECTION('ref_axis',(-0.707106781186548,0.,-0.707106781186548)) ;
#58023=DIRECTION('center_axis',(0.,-1.,0.)) ;
#58024=DIRECTION('ref_axis',(-0.707106781186548,0.,-0.707106781186548)) ;
#58025=DIRECTION('center_axis',(-1.,0.,-1.51760508056877E-16)) ;
#58026=DIRECTION('ref_axis',(1.07310884363305E-16,-0.707106781186736,-0.707106781186359)) ;
#58027=DIRECTION('center_axis',(-1.,0.,0.)) ;
#58028=DIRECTION('ref_axis',(0.,0.,-1.)) ;
#58029=DIRECTION('',(-1.,0.,-1.51760508056877E-16)) ;
#58030=DIRECTION('',(1.,0.,1.51760508056877E-16)) ;
#58031=DIRECTION('center_axis',(0.,1.,0.)) ;
#58032=DIRECTION('ref_axis',(0.,0.,1.)) ;
#58033=DIRECTION('center_axis',(0.,0.,-1.)) ;
#58034=DIRECTION('ref_axis',(1.,0.,0.)) ;
#58035=DIRECTION('center_axis',(0.,1.,0.)) ;
#58036=DIRECTION('ref_axis',(0.707106781186549,0.,-0.707106781186546)) ;
#58037=DIRECTION('center_axis',(0.,-1.,0.)) ;
#58038=DIRECTION('ref_axis',(0.707106781186549,0.,-0.707106781186547)) ;
#58039=DIRECTION('center_axis',(0.,0.,-1.)) ;
#58040=DIRECTION('ref_axis',(0.707106781186359,-0.707106781186736,0.)) ;
#58041=DIRECTION('center_axis',(0.,0.,-1.)) ;
#58042=DIRECTION('ref_axis',(1.,0.,0.)) ;
#58043=DIRECTION('',(0.,0.,-1.)) ;
#58044=DIRECTION('',(0.,0.,1.)) ;
#58045=DIRECTION('center_axis',(1.,0.,0.)) ;
#58046=DIRECTION('ref_axis',(0.,0.,-1.)) ;
#58047=DIRECTION('center_axis',(1.,0.,0.)) ;
#58048=DIRECTION('ref_axis',(0.,0.663117692312022,0.748515147570694)) ;
#58049=DIRECTION('center_axis',(0.,1.,0.)) ;
#58050=DIRECTION('ref_axis',(0.707106781186548,0.,-0.707106781186548)) ;
#58051=DIRECTION('center_axis',(1.,0.,0.)) ;
#58052=DIRECTION('ref_axis',(0.,1.,0.)) ;
#58053=DIRECTION('center_axis',(1.,0.,0.)) ;
#58054=DIRECTION('ref_axis',(0.,1.,0.)) ;
#58055=DIRECTION('',(0.,-1.,-5.60383084497428E-34)) ;
#58056=DIRECTION('',(0.,0.,-1.)) ;
#58057=DIRECTION('center_axis',(-1.,0.,0.)) ;
#58058=DIRECTION('ref_axis',(0.,0.707106781186538,0.707106781186557)) ;
#58059=DIRECTION('',(0.,1.,5.60383084497428E-34)) ;
#58060=DIRECTION('',(0.,0.,1.)) ;
#58061=DIRECTION('',(0.,-1.,-5.60383084497428E-34)) ;
#58062=DIRECTION('center_axis',(0.,-1.,-5.60383084497428E-34)) ;
#58063=DIRECTION('ref_axis',(0.707106781186549,3.96250679110365E-34,-0.707106781186546)) ;
#58064=DIRECTION('',(0.,1.,5.60383084497428E-34)) ;
#58065=DIRECTION('center_axis',(0.,1.,0.)) ;
#58066=DIRECTION('ref_axis',(0.707106781186549,0.,-0.707106781186547)) ;
#58067=DIRECTION('center_axis',(-1.51760508056877E-16,-5.60383084497428E-34,
1.)) ;
#58068=DIRECTION('ref_axis',(1.,1.81422958079369E-66,1.51760508056877E-16)) ;
#58069=DIRECTION('',(0.,-1.,-5.60383084497428E-34)) ;
#58070=DIRECTION('',(-1.,0.,-1.51760508056877E-16)) ;
#58071=DIRECTION('center_axis',(0.,1.,5.60383084497428E-34)) ;
#58072=DIRECTION('ref_axis',(-0.707106781186546,3.96250679110366E-34,-0.707106781186549)) ;
#58073=DIRECTION('',(0.,1.,5.60383084497428E-34)) ;
#58074=DIRECTION('center_axis',(0.,1.,0.)) ;
#58075=DIRECTION('ref_axis',(-0.810015401063436,0.,-0.586408603313459)) ;
#58076=DIRECTION('center_axis',(1.,0.,0.)) ;
#58077=DIRECTION('ref_axis',(0.,0.,1.)) ;
#58078=DIRECTION('',(0.,1.,0.)) ;
#58079=DIRECTION('',(0.,0.,1.)) ;
#58080=DIRECTION('center_axis',(0.,-1.,0.)) ;
#58081=DIRECTION('ref_axis',(-1.,0.,0.)) ;
#58082=DIRECTION('',(0.,1.,0.)) ;
#58083=DIRECTION('center_axis',(0.,-1.,0.)) ;
#58084=DIRECTION('ref_axis',(0.,0.,1.)) ;
#58085=DIRECTION('center_axis',(-1.,0.,-8.7076315656875E-16)) ;
#58086=DIRECTION('ref_axis',(8.7076315656875E-16,0.,-1.)) ;
#58087=DIRECTION('',(4.87960943544713E-49,-1.,-5.60383084497428E-34)) ;
#58088=DIRECTION('',(8.7076315656875E-16,0.,-1.)) ;
#58089=DIRECTION('center_axis',(4.87960943544713E-49,-1.,-5.60383084497428E-34)) ;
#58090=DIRECTION('ref_axis',(0.707106781186548,3.96250679110366E-34,-0.707106781186548)) ;
#58091=DIRECTION('',(-4.87960943544713E-49,1.,5.60383084497428E-34)) ;
#58092=DIRECTION('center_axis',(0.,1.,0.)) ;
#58093=DIRECTION('ref_axis',(0.810015401063433,0.,-0.586408603313462)) ;
#58094=DIRECTION('center_axis',(-1.51760508056877E-16,-5.60383084497428E-34,
1.)) ;
#58095=DIRECTION('ref_axis',(1.,1.81422958079369E-66,1.51760508056877E-16)) ;
#58096=DIRECTION('',(2.22044604925031E-16,-1.,3.31372189702139E-32)) ;
#58097=DIRECTION('',(-1.,0.,-1.51760508056877E-16)) ;
#58098=DIRECTION('center_axis',(-2.22044604925031E-16,1.,-3.31372189702139E-32)) ;
#58099=DIRECTION('ref_axis',(-0.707106781186546,-1.57009245868377E-16,-0.707106781186549)) ;
#58100=DIRECTION('',(-2.22044604925031E-16,1.,-3.31372189702139E-32)) ;
#58101=DIRECTION('center_axis',(0.,1.,0.)) ;
#58102=DIRECTION('ref_axis',(-0.707106781186549,0.,-0.707106781186546)) ;
#58103=DIRECTION('center_axis',(-1.,-2.22044604925031E-16,0.)) ;
#58104=DIRECTION('ref_axis',(2.22044604925031E-16,-1.,3.31372189702139E-32)) ;
#58105=DIRECTION('',(-2.22044604925031E-16,1.,-3.31372189702139E-32)) ;
#58106=DIRECTION('',(0.,0.,-1.)) ;
#58107=DIRECTION('',(2.22044604925031E-16,-1.,3.31372189702139E-32)) ;
#58108=DIRECTION('center_axis',(1.,2.22044604925031E-16,0.)) ;
#58109=DIRECTION('ref_axis',(-1.57009245868375E-16,0.707106781186538,0.707106781186557)) ;
#58110=DIRECTION('',(0.,0.,1.)) ;
#58111=DIRECTION('center_axis',(-1.51760508056877E-16,-5.60383084497428E-34,
1.)) ;
#58112=DIRECTION('ref_axis',(1.,0.,0.)) ;
#58113=DIRECTION('center_axis',(0.,1.,5.60383084497428E-34)) ;
#58114=DIRECTION('ref_axis',(-1.,0.,0.)) ;
#58115=DIRECTION('center_axis',(-1.51760508056877E-16,-5.60383084497428E-34,
1.)) ;
#58116=DIRECTION('ref_axis',(1.,1.86794361499143E-34,1.51760508056877E-16)) ;
#58117=DIRECTION('center_axis',(0.,0.,1.)) ;
#58118=DIRECTION('ref_axis',(1.,0.,0.)) ;
#58119=DIRECTION('',(0.,0.,-1.)) ;
#58120=DIRECTION('center_axis',(-1.4923676700635E-16,0.,1.)) ;
#58121=DIRECTION('ref_axis',(1.,0.,1.4923676700635E-16)) ;
#58122=DIRECTION('',(0.000396813558216815,-0.999999921269497,0.)) ;
#58123=DIRECTION('center_axis',(-1.4923676700635E-16,0.,1.)) ;
#58124=DIRECTION('ref_axis',(1.,0.,0.)) ;
#58125=DIRECTION('center_axis',(0.,-1.,0.)) ;
#58126=DIRECTION('ref_axis',(-1.,0.,0.)) ;
#58127=DIRECTION('center_axis',(-1.4923676700635E-16,0.,1.)) ;
#58128=DIRECTION('ref_axis',(1.,0.,1.4923676700635E-16)) ;
#58129=DIRECTION('center_axis',(-1.4923676700635E-16,0.,1.)) ;
#58130=DIRECTION('ref_axis',(1.,0.,1.4923676700635E-16)) ;
#58131=DIRECTION('center_axis',(1.4923676700635E-16,0.,-1.)) ;
#58132=DIRECTION('ref_axis',(1.,0.,1.4923676700635E-16)) ;
#58133=DIRECTION('center_axis',(1.4923676700635E-16,0.,-1.)) ;
#58134=DIRECTION('ref_axis',(-1.,0.,0.)) ;
#58135=DIRECTION('center_axis',(-1.4923676700635E-16,0.,1.)) ;
#58136=DIRECTION('ref_axis',(1.,0.,1.4923676700635E-16)) ;
#58137=DIRECTION('center_axis',(0.,-1.,0.)) ;
#58138=DIRECTION('ref_axis',(1.,0.,0.)) ;
#58139=DIRECTION('center_axis',(-1.4923676700635E-16,0.,1.)) ;
#58140=DIRECTION('ref_axis',(1.,0.,1.4923676700635E-16)) ;
#58141=DIRECTION('center_axis',(0.,0.,1.)) ;
#58142=DIRECTION('ref_axis',(1.,0.,0.)) ;
#58143=DIRECTION('',(0.,0.,1.)) ;
#58144=DIRECTION('center_axis',(1.4923676700635E-16,0.,-1.)) ;
#58145=DIRECTION('ref_axis',(1.,0.,1.4923676700635E-16)) ;
#58146=DIRECTION('center_axis',(0.,-0.97854978498675,-0.206010481049838)) ;
#58147=DIRECTION('ref_axis',(0.,0.206010481049828,-0.978549784986752)) ;
#58148=DIRECTION('center_axis',(0.,0.97854978498675,0.206010481049838)) ;
#58149=DIRECTION('ref_axis',(-1.,9.47139866158082E-17,-4.49891436425098E-16)) ;
#58150=DIRECTION('center_axis',(-1.,0.,0.)) ;
#58151=DIRECTION('ref_axis',(0.,-0.206010481049841,0.978549784986749)) ;
#58152=DIRECTION('center_axis',(0.,-0.97854978498675,-0.206010481049838)) ;
#58153=DIRECTION('ref_axis',(-1.,9.47139866158082E-17,-4.49891436425098E-16)) ;
#58154=DIRECTION('center_axis',(0.,-0.97854978498675,-0.206010481049838)) ;
#58155=DIRECTION('ref_axis',(-1.,9.47139866158082E-17,-4.49891436425098E-16)) ;
#58156=DIRECTION('center_axis',(0.,-0.97854978498675,-0.206010481049839)) ;
#58157=DIRECTION('ref_axis',(-1.,0.,0.)) ;
#58158=DIRECTION('',(0.,-0.97854978498675,-0.206010481049839)) ;
#58159=DIRECTION('center_axis',(0.,0.97854978498675,0.206010481049838)) ;
#58160=DIRECTION('ref_axis',(-1.,-9.47139866158082E-17,4.49891436425098E-16)) ;
#58161=DIRECTION('center_axis',(0.,0.97854978498675,0.206010481049838)) ;
#58162=DIRECTION('ref_axis',(-1.,-9.47139866158082E-17,4.49891436425098E-16)) ;
#58163=DIRECTION('center_axis',(0.,0.97854978498675,0.206010481049838)) ;
#58164=DIRECTION('ref_axis',(0.,-0.206010481049838,0.97854978498675)) ;
#58165=DIRECTION('',(-1.,3.19495806435525E-17,-1.51760508056877E-16)) ;
#58166=DIRECTION('',(0.,-0.206010481049838,0.97854978498675)) ;
#58167=DIRECTION('center_axis',(0.,0.97854978498675,0.206010481049838)) ;
#58168=DIRECTION('ref_axis',(2.85896974219543E-17,0.206010481049838,-0.97854978498675)) ;
#58169=DIRECTION('',(-1.,0.,-1.4923676700635E-16)) ;
#58170=DIRECTION('center_axis',(0.,0.97854978498675,0.206010481049838)) ;
#58171=DIRECTION('ref_axis',(-1.42948487109771E-17,0.206010481049838,-0.97854978498675)) ;
#58172=DIRECTION('',(0.,0.206010481049838,-0.97854978498675)) ;
#58173=DIRECTION('center_axis',(0.,0.97854978498675,0.206010481049838)) ;
#58174=DIRECTION('ref_axis',(0.,-0.206010481049828,0.978549784986752)) ;
#58175=DIRECTION('center_axis',(0.,-0.97854978498675,-0.206010481049838)) ;
#58176=DIRECTION('ref_axis',(-1.,-9.47139866158082E-17,4.49891436425098E-16)) ;
#58177=DIRECTION('center_axis',(-1.,0.,0.)) ;
#58178=DIRECTION('ref_axis',(0.,0.206010481049841,-0.978549784986749)) ;
#58179=DIRECTION('center_axis',(0.,0.97854978498675,0.206010481049838)) ;
#58180=DIRECTION('ref_axis',(0.,-0.206010481049838,0.97854978498675)) ;
#58181=DIRECTION('',(0.,-0.206010481049838,0.97854978498675)) ;
#58182=DIRECTION('',(0.,0.206010481049838,-0.97854978498675)) ;
#58183=DIRECTION('',(-1.,0.,0.)) ;
#58184=DIRECTION('center_axis',(0.,-0.97854978498675,-0.206010481049838)) ;
#58185=DIRECTION('ref_axis',(0.,0.206010481049829,-0.978549784986752)) ;
#58186=DIRECTION('center_axis',(0.,0.97854978498675,0.206010481049838)) ;
#58187=DIRECTION('ref_axis',(-1.,-3.89103363082382E-16,1.84824097464135E-15)) ;
#58188=DIRECTION('center_axis',(-1.,0.,0.)) ;
#58189=DIRECTION('ref_axis',(0.,-0.206010481049842,0.978549784986749)) ;
#58190=DIRECTION('center_axis',(0.,-0.97854978498675,-0.206010481049838)) ;
#58191=DIRECTION('ref_axis',(-1.,-3.89103363082383E-16,1.84824097464135E-15)) ;
#58192=DIRECTION('center_axis',(0.,-0.97854978498675,-0.206010481049838)) ;
#58193=DIRECTION('ref_axis',(-1.,-3.89103363082383E-16,1.84824097464135E-15)) ;
#58194=DIRECTION('center_axis',(0.,-0.97854978498675,-0.206010481049839)) ;
#58195=DIRECTION('ref_axis',(-1.,0.,0.)) ;
#58196=DIRECTION('',(0.,-0.97854978498675,-0.206010481049839)) ;
#58197=DIRECTION('center_axis',(0.,0.97854978498675,0.206010481049838)) ;
#58198=DIRECTION('ref_axis',(-1.,-9.47139866158086E-17,4.498914364251E-16)) ;
#58199=DIRECTION('center_axis',(0.,0.97854978498675,0.206010481049838)) ;
#58200=DIRECTION('ref_axis',(-1.,-9.47139866158086E-17,4.498914364251E-16)) ;
#58201=DIRECTION('center_axis',(0.,0.97854978498675,0.206010481049838)) ;
#58202=DIRECTION('ref_axis',(0.,-0.206010481049838,0.97854978498675)) ;
#58203=DIRECTION('',(-1.,3.19495806435525E-17,-1.51760508056877E-16)) ;
#58204=DIRECTION('',(0.,-0.206010481049838,0.97854978498675)) ;
#58205=DIRECTION('center_axis',(0.,0.97854978498675,0.206010481049838)) ;
#58206=DIRECTION('ref_axis',(1.42948487109771E-17,0.206010481049838,-0.97854978498675)) ;
#58207=DIRECTION('',(-1.,0.,-1.4923676700635E-16)) ;
#58208=DIRECTION('center_axis',(0.,0.97854978498675,0.206010481049838)) ;
#58209=DIRECTION('ref_axis',(-1.42948487109771E-17,0.206010481049838,-0.97854978498675)) ;
#58210=DIRECTION('',(0.,0.206010481049838,-0.97854978498675)) ;
#58211=DIRECTION('center_axis',(0.,0.97854978498675,0.206010481049838)) ;
#58212=DIRECTION('ref_axis',(0.,-0.206010481049829,0.978549784986752)) ;
#58213=DIRECTION('center_axis',(0.,-0.97854978498675,-0.206010481049838)) ;
#58214=DIRECTION('ref_axis',(-1.,-9.47139866158086E-17,4.498914364251E-16)) ;
#58215=DIRECTION('center_axis',(-1.,0.,0.)) ;
#58216=DIRECTION('ref_axis',(0.,0.206010481049842,-0.978549784986749)) ;
#58217=DIRECTION('center_axis',(0.,0.97854978498675,0.206010481049838)) ;
#58218=DIRECTION('ref_axis',(0.,-0.206010481049838,0.97854978498675)) ;
#58219=DIRECTION('',(-1.,0.,0.)) ;
#58220=DIRECTION('',(0.,-0.206010481049838,0.97854978498675)) ;
#58221=DIRECTION('',(0.,0.206010481049838,-0.97854978498675)) ;
#58222=DIRECTION('center_axis',(0.,-1.,0.)) ;
#58223=DIRECTION('ref_axis',(0.,0.,-1.)) ;
#58224=DIRECTION('center_axis',(1.,0.,0.)) ;
#58225=DIRECTION('ref_axis',(0.,0.,-1.)) ;
#58226=DIRECTION('center_axis',(0.,-1.,0.)) ;
#58227=DIRECTION('ref_axis',(0.810015401063433,0.,-0.586408603313462)) ;
#58228=DIRECTION('center_axis',(0.,0.,-1.)) ;
#58229=DIRECTION('ref_axis',(0.,1.,0.)) ;
#58230=DIRECTION('center_axis',(8.7076315656875E-16,0.,-1.)) ;
#58231=DIRECTION('ref_axis',(0.707106781186391,0.707106781186704,6.1572253281703E-16)) ;
#58232=DIRECTION('center_axis',(0.,0.,-1.)) ;
#58233=DIRECTION('ref_axis',(0.,1.,0.)) ;
#58234=DIRECTION('',(-8.7076315656875E-16,0.,1.)) ;
#58235=DIRECTION('center_axis',(0.,-1.,0.)) ;
#58236=DIRECTION('ref_axis',(0.,0.,1.)) ;
#58237=DIRECTION('center_axis',(0.,0.,1.)) ;
#58238=DIRECTION('ref_axis',(0.,1.,0.)) ;
#58239=DIRECTION('center_axis',(0.,1.,0.)) ;
#58240=DIRECTION('ref_axis',(0.,0.,1.)) ;
#58241=DIRECTION('center_axis',(0.,0.,1.)) ;
#58242=DIRECTION('ref_axis',(-0.707106781186359,0.707106781186736,0.)) ;
#58243=DIRECTION('center_axis',(0.,0.,1.)) ;
#58244=DIRECTION('ref_axis',(0.,1.,0.)) ;
#58245=DIRECTION('',(0.,0.,-1.)) ;
#58246=DIRECTION('center_axis',(0.,-1.,0.)) ;
#58247=DIRECTION('ref_axis',(0.,0.,-1.)) ;
#58248=DIRECTION('center_axis',(-1.,0.,0.)) ;
#58249=DIRECTION('ref_axis',(0.,1.,0.)) ;
#58250=DIRECTION('center_axis',(0.,-1.,0.)) ;
#58251=DIRECTION('ref_axis',(-0.810015401063435,0.,-0.586408603313459)) ;
#58252=DIRECTION('center_axis',(0.,1.,0.)) ;
#58253=DIRECTION('ref_axis',(-1.,0.,-1.4923676700635E-16)) ;
#58254=DIRECTION('',(1.,0.,1.51760508056877E-16)) ;
#58255=DIRECTION('center_axis',(0.,-1.,0.)) ;
#58256=DIRECTION('ref_axis',(-0.707106781186549,0.,-0.707106781186546)) ;
#58257=DIRECTION('',(0.,0.,-1.)) ;
#58258=DIRECTION('',(-1.,0.,-1.51760508056877E-16)) ;
#58259=DIRECTION('',(0.,0.,1.)) ;
#58260=DIRECTION('',(0.,0.,-1.)) ;
#58261=DIRECTION('',(-1.,0.,-1.51760508056877E-16)) ;
#58262=DIRECTION('',(0.,0.,1.)) ;
#58263=DIRECTION('',(0.,0.,-1.)) ;
#58264=DIRECTION('',(-1.,0.,-1.51760508056877E-16)) ;
#58265=DIRECTION('',(0.,0.,1.)) ;
#58266=DIRECTION('center_axis',(0.,-1.,0.)) ;
#58267=DIRECTION('ref_axis',(0.707106781186549,0.,-0.707106781186546)) ;
#58268=DIRECTION('',(1.,0.,1.51760508056877E-16)) ;
#58269=DIRECTION('center_axis',(1.,0.,1.51760508056877E-16)) ;
#58270=DIRECTION('ref_axis',(1.07310884363343E-16,0.707106781186485,-0.70710678118661)) ;
#58271=DIRECTION('center_axis',(-1.,0.,-4.44089209850043E-14)) ;
#58272=DIRECTION('ref_axis',(0.,1.,0.)) ;
#58273=DIRECTION('center_axis',(0.,1.,0.)) ;
#58274=DIRECTION('ref_axis',(-1.,0.,-1.4923676700635E-16)) ;
#58275=DIRECTION('',(1.,0.,1.51760508056877E-16)) ;
#58276=DIRECTION('center_axis',(0.,-1.,0.)) ;
#58277=DIRECTION('ref_axis',(-3.36349381434756E-17,0.,-1.)) ;
#58278=DIRECTION('center_axis',(0.,-1.,0.)) ;
#58279=DIRECTION('ref_axis',(0.,0.,-1.)) ;
#58280=DIRECTION('',(0.,0.,-1.)) ;
#58281=DIRECTION('',(0.,0.,-1.)) ;
#58282=DIRECTION('center_axis',(0.,-1.,0.)) ;
#58283=DIRECTION('ref_axis',(0.,0.,-1.)) ;
#58284=DIRECTION('center_axis',(0.,-1.,0.)) ;
#58285=DIRECTION('ref_axis',(3.36349381434756E-17,0.,-1.)) ;
#58286=DIRECTION('',(1.,0.,1.51760508056877E-16)) ;
#58287=DIRECTION('center_axis',(0.,-1.,0.)) ;
#58288=DIRECTION('ref_axis',(1.,0.,3.92523114670939E-16)) ;
#58289=DIRECTION('',(1.,0.,1.51760508056877E-16)) ;
#58290=DIRECTION('',(1.,0.,1.51760508056877E-16)) ;
#58291=DIRECTION('center_axis',(1.,0.,1.51760508056877E-16)) ;
#58292=DIRECTION('ref_axis',(1.07310884363343E-16,0.707106781186485,-0.70710678118661)) ;
#58293=DIRECTION('center_axis',(-1.,0.,0.)) ;
#58294=DIRECTION('ref_axis',(0.,1.,0.)) ;
#58295=DIRECTION('center_axis',(-1.,0.,-1.51760508056877E-16)) ;
#58296=DIRECTION('ref_axis',(-1.07310884363324E-16,0.70710678118661,0.707106781186485)) ;
#58297=DIRECTION('center_axis',(-1.,0.,0.)) ;
#58298=DIRECTION('ref_axis',(0.,0.,1.)) ;
#58299=DIRECTION('center_axis',(-0.996538840142805,0.,0.0831284553377041)) ;
#58300=DIRECTION('ref_axis',(0.0828427124744576,0.0828427124744687,0.993113372168428)) ;
#58301=DIRECTION('center_axis',(0.554700196225257,0.832050294337825,-2.46336371845354E-14)) ;
#58302=DIRECTION('ref_axis',(0.832050294337825,-0.554700196225257,1.77197583952116E-30)) ;
#58303=DIRECTION('center_axis',(-1.,1.11022302462518E-14,-2.26623325918295E-15)) ;
#58304=DIRECTION('ref_axis',(-3.546880840987E-30,0.19999999999989,0.979795897113294)) ;
#58305=DIRECTION('center_axis',(-1.,0.,-1.51760508056877E-16)) ;
#58306=DIRECTION('ref_axis',(-9.59817728648186E-17,0.774596669241454,0.632455532033712)) ;
#58307=DIRECTION('center_axis',(-1.,0.,0.)) ;
#58308=DIRECTION('ref_axis',(0.,0.199999999999984,0.979795897113275)) ;
#58309=DIRECTION('',(-1.,0.,-1.51760508056877E-16)) ;
#58310=DIRECTION('center_axis',(-1.,0.,6.66133814775093E-14)) ;
#58311=DIRECTION('ref_axis',(6.66133814775093E-14,0.,1.)) ;
#58312=DIRECTION('center_axis',(-1.,0.,-1.51760508056877E-16)) ;
#58313=DIRECTION('ref_axis',(-1.07310884363324E-16,0.70710678118661,0.707106781186485)) ;
#58314=DIRECTION('center_axis',(2.22044604925031E-16,-1.,3.31372189702139E-32)) ;
#58315=DIRECTION('ref_axis',(-0.707106781186548,-1.57009245868377E-16,-0.707106781186548)) ;
#58316=DIRECTION('center_axis',(0.,1.,0.)) ;
#58317=DIRECTION('ref_axis',(0.,0.,-1.)) ;
#58318=DIRECTION('center_axis',(1.51760508056877E-16,5.60383084497428E-34,
-1.)) ;
#58319=DIRECTION('ref_axis',(-1.,0.,0.)) ;
#58320=DIRECTION('center_axis',(1.,0.,0.)) ;
#58321=DIRECTION('ref_axis',(0.,-1.,4.44089209849993E-14)) ;
#58322=DIRECTION('center_axis',(-1.51760508056877E-16,-5.60383084497428E-34,
1.)) ;
#58323=DIRECTION('ref_axis',(-0.707106781186614,0.707106781186481,-1.07310884363344E-16)) ;
#58324=DIRECTION('center_axis',(0.,1.,0.)) ;
#58325=DIRECTION('ref_axis',(1.,0.,0.)) ;
#58326=DIRECTION('center_axis',(-1.,0.,-1.51760508056877E-16)) ;
#58327=DIRECTION('ref_axis',(1.07310884363343E-16,-0.707106781186485,-0.70710678118661)) ;
#58328=DIRECTION('center_axis',(1.,0.,0.)) ;
#58329=DIRECTION('ref_axis',(0.,-1.,0.)) ;
#58330=DIRECTION('',(-1.,0.,-1.51760508056877E-16)) ;
#58331=DIRECTION('center_axis',(1.51760508056877E-16,5.60383084497428E-34,
-1.)) ;
#58332=DIRECTION('ref_axis',(-1.,0.,0.)) ;
#58333=DIRECTION('center_axis',(0.707106781186592,-0.707106781186503,0.)) ;
#58334=DIRECTION('ref_axis',(-0.707106781186503,-0.707106781186592,-4.44089209850158E-14)) ;
#58335=DIRECTION('center_axis',(-1.51760508056877E-16,-5.60383084497428E-34,
1.)) ;
#58336=DIRECTION('ref_axis',(0.382683432364956,0.923879532511342,5.80762321206553E-17)) ;
#58337=DIRECTION('center_axis',(0.707106781186555,-0.70710678118654,1.07310884363335E-16)) ;
#58338=DIRECTION('ref_axis',(-0.499999999999962,-0.499999999999972,-0.707106781186594)) ;
#58339=DIRECTION('center_axis',(0.707106781186437,-0.707106781186659,0.)) ;
#58340=DIRECTION('ref_axis',(-0.707106781186659,-0.707106781186437,0.)) ;
#58341=DIRECTION('',(-0.707106781186555,0.70710678118654,-1.07310884363335E-16)) ;
#58342=DIRECTION('center_axis',(-1.,0.,-1.51760508056877E-16)) ;
#58343=DIRECTION('ref_axis',(-1.07310884363324E-16,0.70710678118661,0.707106781186485)) ;
#58344=DIRECTION('center_axis',(0.,-0.206010481049838,0.97854978498675)) ;
#58345=DIRECTION('ref_axis',(0.707106781186543,-0.691939188692773,-0.145671408145844)) ;
#58346=DIRECTION('center_axis',(-0.816496580927833,-0.40824829046381,0.408248290463703)) ;
#58347=DIRECTION('ref_axis',(0.577350269189448,-0.577350269189946,0.577350269189484)) ;
#58348=DIRECTION('center_axis',(-3.55271367880058E-13,-1.,0.)) ;
#58349=DIRECTION('ref_axis',(0.,0.,1.)) ;
#58350=DIRECTION('center_axis',(1.,0.,0.)) ;
#58351=DIRECTION('ref_axis',(0.,-1.,0.)) ;
#58352=DIRECTION('center_axis',(0.,0.,1.)) ;
#58353=DIRECTION('ref_axis',(1.,0.,0.)) ;
#58354=DIRECTION('center_axis',(1.,0.,1.51760508056877E-16)) ;
#58355=DIRECTION('ref_axis',(-1.07310884363343E-16,-0.707106781186485,0.70710678118661)) ;
#58356=DIRECTION('center_axis',(1.,0.,0.)) ;
#58357=DIRECTION('ref_axis',(0.,0.,1.)) ;
#58358=DIRECTION('',(1.,0.,1.51760508056877E-16)) ;
#58359=DIRECTION('center_axis',(-1.51760508056877E-16,-5.60383084497428E-34,
1.)) ;
#58360=DIRECTION('ref_axis',(1.,0.,0.)) ;
#58361=DIRECTION('center_axis',(0.,1.,0.)) ;
#58362=DIRECTION('ref_axis',(0.707106781186548,0.,0.707106781186548)) ;
#58363=DIRECTION('center_axis',(0.,0.,1.)) ;
#58364=DIRECTION('ref_axis',(0.,1.,0.)) ;
#58365=DIRECTION('center_axis',(-0.81649658092775,-0.408248290463875,-0.408248290463804)) ;
#58366=DIRECTION('ref_axis',(0.577350269189602,-0.577350269189744,-0.577350269189531)) ;
#58367=DIRECTION('center_axis',(0.,0.,-1.)) ;
#58368=DIRECTION('ref_axis',(1.,0.,0.)) ;
#58369=DIRECTION('center_axis',(1.,0.,1.51760508056877E-16)) ;
#58370=DIRECTION('ref_axis',(1.07310884363347E-16,-0.707106781186459,-0.707106781186636)) ;
#58371=DIRECTION('center_axis',(0.,-1.,-5.60383084497428E-34)) ;
#58372=DIRECTION('ref_axis',(0.707106781186547,3.96250679110365E-34,-0.707106781186547)) ;
#58373=DIRECTION('center_axis',(0.,0.,1.)) ;
#58374=DIRECTION('ref_axis',(0.70710678118661,-0.707106781186485,0.)) ;
#58375=DIRECTION('',(0.,0.,1.)) ;
#58376=DIRECTION('',(0.,0.,-1.)) ;
#58377=DIRECTION('center_axis',(0.,0.,1.)) ;
#58378=DIRECTION('ref_axis',(1.,0.,0.)) ;
#58379=DIRECTION('center_axis',(-1.,0.,0.)) ;
#58380=DIRECTION('ref_axis',(0.,-1.,0.)) ;
#58381=DIRECTION('center_axis',(0.,0.,-1.)) ;
#58382=DIRECTION('ref_axis',(1.,0.,0.)) ;
#58383=DIRECTION('center_axis',(0.,-1.,0.)) ;
#58384=DIRECTION('ref_axis',(0.,0.,1.)) ;
#58385=DIRECTION('center_axis',(0.,0.,-1.)) ;
#58386=DIRECTION('ref_axis',(-1.,0.,0.)) ;
#58387=DIRECTION('center_axis',(4.44089209850072E-14,0.,-1.)) ;
#58388=DIRECTION('ref_axis',(0.,1.,0.)) ;
#58389=DIRECTION('center_axis',(1.,0.,0.)) ;
#58390=DIRECTION('ref_axis',(0.,0.,1.)) ;
#58391=DIRECTION('center_axis',(0.,-1.,0.)) ;
#58392=DIRECTION('ref_axis',(1.,0.,0.)) ;
#58393=DIRECTION('center_axis',(1.,0.,1.51760508056877E-16)) ;
#58394=DIRECTION('ref_axis',(-1.07310884363343E-16,-0.707106781186485,0.70710678118661)) ;
#58395=DIRECTION('',(1.,0.,1.51760508056877E-16)) ;
#58396=DIRECTION('center_axis',(0.,1.,5.60383084497428E-34)) ;
#58397=DIRECTION('ref_axis',(0.707106781186548,-3.96250679110365E-34,0.707106781186548)) ;
#58398=DIRECTION('',(0.,1.,5.60383084497428E-34)) ;
#58399=DIRECTION('center_axis',(0.,-1.,0.)) ;
#58400=DIRECTION('ref_axis',(0.,0.,-1.)) ;
#58401=DIRECTION('center_axis',(0.,0.,1.)) ;
#58402=DIRECTION('ref_axis',(0.,1.,0.)) ;
#58403=DIRECTION('center_axis',(0.,1.,0.)) ;
#58404=DIRECTION('ref_axis',(0.707106781186548,0.,-0.707106781186548)) ;
#58405=DIRECTION('center_axis',(0.,-1.,0.)) ;
#58406=DIRECTION('ref_axis',(0.707106781186548,0.,-0.707106781186548)) ;
#58407=DIRECTION('center_axis',(0.,0.,1.)) ;
#58408=DIRECTION('ref_axis',(-0.70710678118661,0.707106781186485,0.)) ;
#58409=DIRECTION('',(0.,0.,-1.)) ;
#58410=DIRECTION('',(0.,0.,1.)) ;
#58411=DIRECTION('center_axis',(0.,0.,1.)) ;
#58412=DIRECTION('ref_axis',(0.70710678118661,0.707106781186485,0.)) ;
#58413=DIRECTION('center_axis',(0.,0.,-1.)) ;
#58414=DIRECTION('ref_axis',(0.,1.,0.)) ;
#58415=DIRECTION('',(0.,0.,1.)) ;
#58416=DIRECTION('',(0.,0.,-1.)) ;
#58417=DIRECTION('center_axis',(0.,-1.,0.)) ;
#58418=DIRECTION('ref_axis',(0.,0.,-1.)) ;
#58419=DIRECTION('center_axis',(0.,1.,0.)) ;
#58420=DIRECTION('ref_axis',(-0.707106781186548,0.,-0.707106781186548)) ;
#58421=DIRECTION('center_axis',(0.,-1.,0.)) ;
#58422=DIRECTION('ref_axis',(-0.707106781186548,0.,-0.707106781186548)) ;
#58423=DIRECTION('center_axis',(0.,-1.,-5.60383084497428E-34)) ;
#58424=DIRECTION('ref_axis',(-0.707106781186548,-3.96250679110365E-34,0.707106781186548)) ;
#58425=DIRECTION('center_axis',(0.,1.,0.)) ;
#58426=DIRECTION('ref_axis',(-1.,0.,0.)) ;
#58427=DIRECTION('',(0.,-1.,-5.60383084497428E-34)) ;
#58428=DIRECTION('center_axis',(-0.81649658092775,0.408248290463875,-0.408248290463804)) ;
#58429=DIRECTION('ref_axis',(-0.577350269189602,-0.577350269189744,0.577350269189531)) ;
#58430=DIRECTION('center_axis',(0.,0.,1.)) ;
#58431=DIRECTION('ref_axis',(-0.707106781186636,-0.707106781186459,0.)) ;
#58432=DIRECTION('center_axis',(-1.,0.,-1.51760508056877E-16)) ;
#58433=DIRECTION('ref_axis',(-1.07310884363347E-16,-0.707106781186459,0.707106781186636)) ;
#58434=DIRECTION('center_axis',(-1.,0.,-1.51760508056877E-16)) ;
#58435=DIRECTION('ref_axis',(1.07310884363343E-16,-0.707106781186485,-0.70710678118661)) ;
#58436=DIRECTION('',(-1.,0.,-1.51760508056877E-16)) ;
#58437=DIRECTION('center_axis',(1.,0.,0.)) ;
#58438=DIRECTION('ref_axis',(0.,-1.,0.)) ;
#58439=DIRECTION('center_axis',(0.,1.,0.)) ;
#58440=DIRECTION('ref_axis',(-1.,0.,-1.4923676700635E-16)) ;
#58441=DIRECTION('',(0.,0.,1.)) ;
#58442=DIRECTION('center_axis',(1.,0.,1.51760508056877E-16)) ;
#58443=DIRECTION('ref_axis',(-1.07310884363343E-16,-0.707106781186485,0.70710678118661)) ;
#58444=DIRECTION('',(1.,0.,1.51760508056877E-16)) ;
#58445=DIRECTION('center_axis',(-1.,0.,0.)) ;
#58446=DIRECTION('ref_axis',(0.,-1.,0.)) ;
#58447=DIRECTION('center_axis',(0.,0.,1.)) ;
#58448=DIRECTION('ref_axis',(-0.70710678118661,-0.707106781186485,0.)) ;
#58449=DIRECTION('',(0.,0.,-1.)) ;
#58450=DIRECTION('center_axis',(0.,0.,-1.)) ;
#58451=DIRECTION('ref_axis',(-0.707106781186636,-0.707106781186459,0.)) ;
#58452=DIRECTION('',(0.,0.,1.)) ;
#58453=DIRECTION('center_axis',(1.,0.,0.)) ;
#58454=DIRECTION('ref_axis',(0.,1.,0.)) ;
#58455=DIRECTION('',(0.,1.,5.60383084497428E-34)) ;
#58456=DIRECTION('center_axis',(1.,0.,0.)) ;
#58457=DIRECTION('ref_axis',(0.,0.,-1.)) ;
#58458=DIRECTION('center_axis',(0.,0.,1.)) ;
#58459=DIRECTION('ref_axis',(-1.,0.,0.)) ;
#58460=DIRECTION('center_axis',(-1.,0.,0.)) ;
#58461=DIRECTION('ref_axis',(0.,0.707106781186481,-0.707106781186614)) ;
#58462=DIRECTION('center_axis',(1.,0.,0.)) ;
#58463=DIRECTION('ref_axis',(0.,0.707106781186481,-0.707106781186614)) ;
#58464=DIRECTION('center_axis',(0.,0.,1.)) ;
#58465=DIRECTION('ref_axis',(-0.707106781186359,-0.707106781186736,0.)) ;
#58466=DIRECTION('center_axis',(0.,0.,1.)) ;
#58467=DIRECTION('ref_axis',(-1.,0.,0.)) ;
#58468=DIRECTION('',(0.,0.,-1.)) ;
#58469=DIRECTION('',(0.,0.,1.)) ;
#58470=DIRECTION('center_axis',(0.894427190999916,-0.447213595499958,0.)) ;
#58471=DIRECTION('ref_axis',(0.447213595499958,0.894427190999916,0.)) ;
#58472=DIRECTION('center_axis',(-0.447213595500021,0.894427190999884,0.)) ;
#58473=DIRECTION('ref_axis',(0.894427190999884,0.447213595500021,0.)) ;
#58474=DIRECTION('center_axis',(0.,1.,5.60383084497428E-34)) ;
#58475=DIRECTION('ref_axis',(0.707106781186548,-3.96250679110365E-34,0.707106781186548)) ;
#58476=DIRECTION('',(0.,1.,5.60383084497428E-34)) ;
#58477=DIRECTION('center_axis',(-0.70710678118661,-0.707106781186485,0.)) ;
#58478=DIRECTION('ref_axis',(0.707106781186485,-0.70710678118661,2.45326946669362E-16)) ;
#58479=DIRECTION('center_axis',(-1.,0.,0.)) ;
#58480=DIRECTION('ref_axis',(0.,-1.,0.)) ;
#58481=DIRECTION('',(0.,0.,1.)) ;
#58482=DIRECTION('center_axis',(0.,4.44089209850151E-14,-1.)) ;
#58483=DIRECTION('ref_axis',(-1.,0.,0.)) ;
#58484=DIRECTION('center_axis',(-0.447213595500021,-0.894427190999884,0.)) ;
#58485=DIRECTION('ref_axis',(0.894427190999884,-0.447213595500021,0.)) ;
#58486=DIRECTION('center_axis',(0.894427190999916,0.447213595499958,0.)) ;
#58487=DIRECTION('ref_axis',(0.447213595499958,-0.894427190999916,0.)) ;
#58488=DIRECTION('center_axis',(0.,0.,1.)) ;
#58489=DIRECTION('ref_axis',(-0.707106781186673,0.707106781186422,0.)) ;
#58490=DIRECTION('center_axis',(0.,0.,-1.)) ;
#58491=DIRECTION('ref_axis',(-1.,0.,0.)) ;
#58492=DIRECTION('',(0.,0.,1.)) ;
#58493=DIRECTION('',(0.,0.,-1.)) ;
#58494=DIRECTION('center_axis',(1.,0.,0.)) ;
#58495=DIRECTION('ref_axis',(0.,0.,-1.)) ;
#58496=DIRECTION('center_axis',(-1.,0.,0.)) ;
#58497=DIRECTION('ref_axis',(0.,-0.707106781186481,-0.707106781186614)) ;
#58498=DIRECTION('center_axis',(1.,0.,0.)) ;
#58499=DIRECTION('ref_axis',(0.,-0.707106781186481,-0.707106781186614)) ;
#58500=DIRECTION('center_axis',(-1.,0.,0.)) ;
#58501=DIRECTION('ref_axis',(0.,-1.,0.)) ;
#58502=DIRECTION('',(0.,1.,5.60383084497428E-34)) ;
#58503=DIRECTION('',(0.,0.,-1.)) ;
#58504=DIRECTION('center_axis',(0.,1.,5.60383084497428E-34)) ;
#58505=DIRECTION('ref_axis',(0.707106781186548,-3.96250679110365E-34,0.707106781186548)) ;
#58506=DIRECTION('center_axis',(-0.70710678118661,0.707106781186485,0.)) ;
#58507=DIRECTION('ref_axis',(0.707106781186485,0.70710678118661,1.83995210002018E-16)) ;
#58508=DIRECTION('center_axis',(1.,0.,1.51760508056877E-16)) ;
#58509=DIRECTION('ref_axis',(1.07310884363343E-16,0.707106781186485,-0.70710678118661)) ;
#58510=DIRECTION('center_axis',(-1.,0.,0.)) ;
#58511=DIRECTION('ref_axis',(0.,1.,0.)) ;
#58512=DIRECTION('center_axis',(-1.,0.,-2.01858731750028E-16)) ;
#58513=DIRECTION('ref_axis',(1.42735678062174E-16,0.707106781186485,-0.70710678118661)) ;
#58514=DIRECTION('',(1.,0.,1.51760508056877E-16)) ;
#58515=DIRECTION('center_axis',(1.51760508056877E-16,5.60383084497428E-34,
-1.)) ;
#58516=DIRECTION('ref_axis',(-1.,0.,0.)) ;
#58517=DIRECTION('center_axis',(-0.707106781186614,-0.707106781186481,0.)) ;
#58518=DIRECTION('ref_axis',(-0.707106781186481,0.707106781186614,0.)) ;
#58519=DIRECTION('center_axis',(-1.51760508056877E-16,-5.60383084497428E-34,
1.)) ;
#58520=DIRECTION('ref_axis',(0.382683432365032,-0.923879532511311,5.80762321206668E-17)) ;
#58521=DIRECTION('center_axis',(-0.707106781186555,-0.70710678118654,-1.07310884363335E-16)) ;
#58522=DIRECTION('ref_axis',(-0.499999999999977,0.499999999999988,-0.707106781186572)) ;
#58523=DIRECTION('center_axis',(-0.707106781186459,-0.707106781186636,0.)) ;
#58524=DIRECTION('ref_axis',(-0.707106781186636,0.707106781186459,0.)) ;
#58525=DIRECTION('',(0.707106781186555,0.70710678118654,1.07310884363335E-16)) ;
#58526=DIRECTION('center_axis',(1.51760508056877E-16,5.60383084497428E-34,
-1.)) ;
#58527=DIRECTION('ref_axis',(-1.,0.,0.)) ;
#58528=DIRECTION('center_axis',(0.,-1.,0.)) ;
#58529=DIRECTION('ref_axis',(-1.,0.,0.)) ;
#58530=DIRECTION('center_axis',(-1.51760508056877E-16,-5.60383084497428E-34,
1.)) ;
#58531=DIRECTION('ref_axis',(0.923879532511313,-0.382683432365025,1.40208427237267E-16)) ;
#58532=DIRECTION('center_axis',(-1.1311821873082E-49,1.,5.60383084497428E-34)) ;
#58533=DIRECTION('ref_axis',(-0.707106781186548,3.96250679110365E-34,-0.707106781186548)) ;
#58534=DIRECTION('center_axis',(0.,-1.,0.)) ;
#58535=DIRECTION('ref_axis',(-1.,0.,0.)) ;
#58536=DIRECTION('',(-1.1311821873082E-49,1.,5.60383084497428E-34)) ;
#58537=DIRECTION('center_axis',(1.51760508056877E-16,5.60383084497428E-34,
-1.)) ;
#58538=DIRECTION('ref_axis',(-1.,0.,0.)) ;
#58539=DIRECTION('center_axis',(-1.51760508056877E-16,-5.60383084497428E-34,
1.)) ;
#58540=DIRECTION('ref_axis',(0.923879532511313,0.382683432365025,1.40208427237267E-16)) ;
#58541=DIRECTION('center_axis',(1.1311821873082E-49,-1.,-5.60383084497428E-34)) ;
#58542=DIRECTION('ref_axis',(0.707106781186548,3.96250679110365E-34,-0.707106781186548)) ;
#58543=DIRECTION('center_axis',(0.,-1.,0.)) ;
#58544=DIRECTION('ref_axis',(0.707106781186548,0.,-0.707106781186548)) ;
#58545=DIRECTION('',(1.1311821873082E-49,-1.,-5.60383084497428E-34)) ;
#58546=DIRECTION('center_axis',(-1.,0.,-2.01858731750028E-16)) ;
#58547=DIRECTION('ref_axis',(0.,-1.,0.)) ;
#58548=DIRECTION('',(2.01858731750028E-16,0.,-1.)) ;
#58549=DIRECTION('',(-1.1311821873082E-49,1.,5.60383084497428E-34)) ;
#58550=DIRECTION('',(2.01858731750028E-16,0.,-1.)) ;
#58551=DIRECTION('center_axis',(-2.01858731750028E-16,0.,1.)) ;
#58552=DIRECTION('ref_axis',(-0.70710678118661,0.707106781186485,-1.42735678062174E-16)) ;
#58553=DIRECTION('',(-2.01858731750028E-16,0.,1.)) ;
#58554=DIRECTION('center_axis',(0.,0.,-1.)) ;
#58555=DIRECTION('ref_axis',(0.,1.,0.)) ;
#58556=DIRECTION('center_axis',(0.,1.,0.)) ;
#58557=DIRECTION('ref_axis',(-1.,0.,-1.4923676700635E-16)) ;
#58558=DIRECTION('',(2.01858731750028E-16,0.,-1.)) ;
#58559=DIRECTION('',(1.,0.,1.51760508056877E-16)) ;
#58560=DIRECTION('center_axis',(2.01858731750028E-16,0.,-1.)) ;
#58561=DIRECTION('ref_axis',(0.382683432365058,0.9238795325113,7.72479923189582E-17)) ;
#58562=DIRECTION('',(-2.01858731750028E-16,0.,1.)) ;
#58563=DIRECTION('center_axis',(0.,0.,-1.)) ;
#58564=DIRECTION('ref_axis',(0.707106781186481,0.707106781186614,0.)) ;
#58565=DIRECTION('center_axis',(-0.70710678118654,-0.707106781186555,-1.4273567806216E-16)) ;
#58566=DIRECTION('ref_axis',(-2.01858731750028E-16,-3.26018819696323E-31,
1.)) ;
#58567=DIRECTION('',(2.01858731750028E-16,-3.48630559684206E-32,-1.)) ;
#58568=DIRECTION('',(0.707106781186555,-0.70710678118654,1.07310884363335E-16)) ;
#58569=DIRECTION('center_axis',(-2.01858731750028E-16,3.48630559684206E-32,
1.)) ;
#58570=DIRECTION('ref_axis',(0.923879532511304,0.382683432365048,1.86493150722541E-16)) ;
#58571=DIRECTION('',(-2.01858731750028E-16,3.48630559684206E-32,1.)) ;
#58572=DIRECTION('center_axis',(0.,6.28036983473606E-14,-1.)) ;
#58573=DIRECTION('ref_axis',(1.,0.,0.)) ;
#58574=DIRECTION('center_axis',(1.,0.,2.01858731750028E-16)) ;
#58575=DIRECTION('ref_axis',(0.,1.,0.)) ;
#58576=DIRECTION('',(2.01858731750028E-16,3.48630559684206E-32,-1.)) ;
#58577=DIRECTION('',(1.1311821873082E-49,-1.,-5.60383084497428E-34)) ;
#58578=DIRECTION('center_axis',(2.01858731750028E-16,3.48630559684206E-32,
-1.)) ;
#58579=DIRECTION('ref_axis',(0.923879532511304,-0.382683432365048,1.86493150722541E-16)) ;
#58580=DIRECTION('',(-2.01858731750028E-16,-3.48630559684206E-32,1.)) ;
#58581=DIRECTION('center_axis',(0.,0.,-1.)) ;
#58582=DIRECTION('ref_axis',(0.707106781186592,-0.707106781186503,0.)) ;
#58583=DIRECTION('center_axis',(-0.70710678118654,0.707106781186555,-1.4273567806216E-16)) ;
#58584=DIRECTION('ref_axis',(-2.01858731750028E-16,3.26018819696323E-31,
1.)) ;
#58585=DIRECTION('',(2.01858731750028E-16,0.,-1.)) ;
#58586=DIRECTION('',(-0.707106781186555,-0.70710678118654,-1.07310884363335E-16)) ;
#58587=DIRECTION('center_axis',(-2.01858731750028E-16,0.,1.)) ;
#58588=DIRECTION('ref_axis',(0.382683432365017,-0.923879532511317,7.72479923189499E-17)) ;
#58589=DIRECTION('',(-2.01858731750028E-16,0.,1.)) ;
#58590=DIRECTION('center_axis',(0.,0.,-1.)) ;
#58591=DIRECTION('ref_axis',(0.,-1.,0.)) ;
#58592=DIRECTION('center_axis',(0.,-1.,0.)) ;
#58593=DIRECTION('ref_axis',(1.,0.,1.4923676700635E-16)) ;
#58594=DIRECTION('',(-2.01858731750028E-16,0.,1.)) ;
#58595=DIRECTION('',(-1.,0.,-1.51760508056877E-16)) ;
#58596=DIRECTION('center_axis',(-1.,0.,-1.51760508056877E-16)) ;
#58597=DIRECTION('ref_axis',(1.07310884363343E-16,-0.707106781186485,-0.70710678118661)) ;
#58598=DIRECTION('center_axis',(-1.,0.,0.)) ;
#58599=DIRECTION('ref_axis',(0.,0.,-1.)) ;
#58600=DIRECTION('',(-1.,0.,-1.51760508056877E-16)) ;
#58601=DIRECTION('center_axis',(1.,0.,0.)) ;
#58602=DIRECTION('ref_axis',(0.,-1.,4.44089209849993E-14)) ;
#58603=DIRECTION('center_axis',(1.51760508056877E-16,5.60383084497428E-34,
-1.)) ;
#58604=DIRECTION('ref_axis',(-1.,0.,0.)) ;
#58605=DIRECTION('center_axis',(0.,1.,0.)) ;
#58606=DIRECTION('ref_axis',(0.,0.,-1.)) ;
#58607=DIRECTION('center_axis',(-1.51760508056877E-16,-5.60383084497428E-34,
1.)) ;
#58608=DIRECTION('ref_axis',(0.707106781186592,0.707106781186503,1.0731088436334E-16)) ;
#58609=DIRECTION('center_axis',(0.,1.,5.60383084497428E-34)) ;
#58610=DIRECTION('ref_axis',(-0.707106781186579,3.96250679110348E-34,-0.707106781186516)) ;
#58611=DIRECTION('center_axis',(0.,1.,0.)) ;
#58612=DIRECTION('ref_axis',(0.,0.,-1.)) ;
#58613=DIRECTION('',(0.,1.,5.60383084497428E-34)) ;
#58614=DIRECTION('center_axis',(1.51760508056877E-16,5.60383084497428E-34,
-1.)) ;
#58615=DIRECTION('ref_axis',(-1.,0.,0.)) ;
#58616=DIRECTION('center_axis',(1.,0.,0.)) ;
#58617=DIRECTION('ref_axis',(0.,0.,-1.)) ;
#58618=DIRECTION('center_axis',(-1.51760508056877E-16,-5.60383084497428E-34,
1.)) ;
#58619=DIRECTION('ref_axis',(0.707106781186592,-0.707106781186503,1.0731088436334E-16)) ;
#58620=DIRECTION('center_axis',(1.,0.,1.51760508056877E-16)) ;
#58621=DIRECTION('ref_axis',(1.07310884363343E-16,0.707106781186485,-0.70710678118661)) ;
#58622=DIRECTION('center_axis',(1.,0.,0.)) ;
#58623=DIRECTION('ref_axis',(0.,0.,-1.)) ;
#58624=DIRECTION('',(1.,0.,1.51760508056877E-16)) ;
#58625=DIRECTION('center_axis',(1.51760508056877E-16,5.60383084497428E-34,
-1.)) ;
#58626=DIRECTION('ref_axis',(-1.,0.,0.)) ;
#58627=DIRECTION('center_axis',(0.,-1.,0.)) ;
#58628=DIRECTION('ref_axis',(0.,0.,-1.)) ;
#58629=DIRECTION('center_axis',(-1.51760508056877E-16,-5.60383084497428E-34,
1.)) ;
#58630=DIRECTION('ref_axis',(-0.707106781186592,-0.707106781186503,-1.0731088436334E-16)) ;
#58631=DIRECTION('center_axis',(0.,-1.,-5.60383084497428E-34)) ;
#58632=DIRECTION('ref_axis',(0.707106781186579,3.96250679110348E-34,-0.707106781186516)) ;
#58633=DIRECTION('center_axis',(0.,-1.,0.)) ;
#58634=DIRECTION('ref_axis',(0.,0.,-1.)) ;
#58635=DIRECTION('',(0.,-1.,-5.60383084497428E-34)) ;
#58636=DIRECTION('center_axis',(1.51760508056877E-16,5.60383084497428E-34,
-1.)) ;
#58637=DIRECTION('ref_axis',(-1.,0.,0.)) ;
#58638=DIRECTION('center_axis',(-1.,0.,0.)) ;
#58639=DIRECTION('ref_axis',(0.,0.,-1.)) ;
#58640=DIRECTION('center_axis',(-1.51760508056877E-16,-5.60383084497428E-34,
1.)) ;
#58641=DIRECTION('ref_axis',(-0.707106781186592,0.707106781186503,-1.0731088436334E-16)) ;
#58642=DIRECTION('center_axis',(-1.,0.,-1.51760508056877E-16)) ;
#58643=DIRECTION('ref_axis',(1.07310884363343E-16,-0.707106781186485,-0.70710678118661)) ;
#58644=DIRECTION('center_axis',(-1.,0.,0.)) ;
#58645=DIRECTION('ref_axis',(0.,0.,-1.)) ;
#58646=DIRECTION('',(-1.,0.,-1.51760508056877E-16)) ;
#58647=DIRECTION('center_axis',(0.,-1.,-5.60383084497428E-34)) ;
#58648=DIRECTION('ref_axis',(0.707106781186579,3.96250679110348E-34,-0.707106781186516)) ;
#58649=DIRECTION('center_axis',(0.,-1.,0.)) ;
#58650=DIRECTION('ref_axis',(0.,0.,-1.)) ;
#58651=DIRECTION('',(0.,-1.,-5.60383084497428E-34)) ;
#58652=DIRECTION('center_axis',(0.,1.,0.)) ;
#58653=DIRECTION('ref_axis',(1.,0.,0.)) ;
#58654=DIRECTION('center_axis',(1.51760508056877E-16,5.60383084497428E-34,
-1.)) ;
#58655=DIRECTION('ref_axis',(-1.,0.,0.)) ;
#58656=DIRECTION('center_axis',(-1.,0.,0.)) ;
#58657=DIRECTION('ref_axis',(0.,0.,-1.)) ;
#58658=DIRECTION('center_axis',(-1.51760508056877E-16,-5.60383084497428E-34,
1.)) ;
#58659=DIRECTION('ref_axis',(-0.707106781186592,0.707106781186503,-1.0731088436334E-16)) ;
#58660=DIRECTION('center_axis',(-1.,0.,-1.51760508056877E-16)) ;
#58661=DIRECTION('ref_axis',(1.07310884363343E-16,-0.707106781186485,-0.70710678118661)) ;
#58662=DIRECTION('center_axis',(-1.,0.,0.)) ;
#58663=DIRECTION('ref_axis',(0.,0.,-1.)) ;
#58664=DIRECTION('',(-1.,0.,-1.51760508056877E-16)) ;
#58665=DIRECTION('center_axis',(1.51760508056877E-16,5.60383084497428E-34,
-1.)) ;
#58666=DIRECTION('ref_axis',(-1.,0.,0.)) ;
#58667=DIRECTION('center_axis',(0.,1.,0.)) ;
#58668=DIRECTION('ref_axis',(0.,0.,-1.)) ;
#58669=DIRECTION('center_axis',(-1.51760508056877E-16,-5.60383084497428E-34,
1.)) ;
#58670=DIRECTION('ref_axis',(0.707106781186592,0.707106781186503,1.0731088436334E-16)) ;
#58671=DIRECTION('center_axis',(0.,1.,5.60383084497428E-34)) ;
#58672=DIRECTION('ref_axis',(-0.707106781186579,3.96250679110348E-34,-0.707106781186516)) ;
#58673=DIRECTION('center_axis',(0.,1.,0.)) ;
#58674=DIRECTION('ref_axis',(0.,0.,-1.)) ;
#58675=DIRECTION('',(0.,1.,5.60383084497428E-34)) ;
#58676=DIRECTION('center_axis',(-0.408248290463679,-0.816496580927927,0.408248290463644)) ;
#58677=DIRECTION('ref_axis',(0.577350269189721,-0.577350269189436,-0.577350269189721)) ;
#58678=DIRECTION('center_axis',(0.,0.,-1.)) ;
#58679=DIRECTION('ref_axis',(0.707106781186636,-0.707106781186459,0.)) ;
#58680=DIRECTION('center_axis',(-0.816496580927726,0.408248290463863,0.408248290463863)) ;
#58681=DIRECTION('ref_axis',(-0.577350269189614,-0.577350269189756,-0.577350269189507)) ;
#58682=DIRECTION('center_axis',(0.,0.,-1.)) ;
#58683=DIRECTION('ref_axis',(-0.707106781186681,-0.707106781186414,0.)) ;
#58684=DIRECTION('center_axis',(0.,0.,1.)) ;
#58685=DIRECTION('ref_axis',(0.70710678118661,-0.707106781186485,0.)) ;
#58686=DIRECTION('',(0.,0.,1.)) ;
#58687=DIRECTION('center_axis',(-4.44089209850072E-14,0.,-1.)) ;
#58688=DIRECTION('ref_axis',(0.,-1.,0.)) ;
#58689=DIRECTION('',(0.,0.,-1.)) ;
#58690=DIRECTION('center_axis',(0.,-1.,0.)) ;
#58691=DIRECTION('ref_axis',(1.,0.,1.4923676700635E-16)) ;
#58692=DIRECTION('',(0.,0.,-1.)) ;
#58693=DIRECTION('',(-1.,0.,-1.51760508056877E-16)) ;
#58694=DIRECTION('center_axis',(0.,0.,1.)) ;
#58695=DIRECTION('ref_axis',(-0.707106781186359,-0.707106781186736,0.)) ;
#58696=DIRECTION('',(0.,0.,1.)) ;
#58697=DIRECTION('center_axis',(0.,0.,-1.)) ;
#58698=DIRECTION('ref_axis',(-1.,0.,0.)) ;
#58699=DIRECTION('center_axis',(-1.,0.,0.)) ;
#58700=DIRECTION('ref_axis',(0.,-1.,0.)) ;
#58701=DIRECTION('',(0.,0.,-1.)) ;
#58702=DIRECTION('',(0.,1.,5.60383084497428E-34)) ;
#58703=DIRECTION('center_axis',(0.,0.,1.)) ;
#58704=DIRECTION('ref_axis',(-0.70710678118661,0.707106781186485,0.)) ;
#58705=DIRECTION('',(0.,0.,1.)) ;
#58706=DIRECTION('center_axis',(4.44089209850072E-14,0.,-1.)) ;
#58707=DIRECTION('ref_axis',(0.,1.,0.)) ;
#58708=DIRECTION('center_axis',(0.,1.,0.)) ;
#58709=DIRECTION('ref_axis',(-1.,0.,-1.4923676700635E-16)) ;
#58710=DIRECTION('',(0.,0.,-1.)) ;
#58711=DIRECTION('',(1.,0.,1.51760508056877E-16)) ;
#58712=DIRECTION('center_axis',(0.,0.,1.)) ;
#58713=DIRECTION('ref_axis',(0.70710678118661,-0.707106781186485,0.)) ;
#58714=DIRECTION('',(0.,0.,1.)) ;
#58715=DIRECTION('center_axis',(0.,0.,1.)) ;
#58716=DIRECTION('ref_axis',(1.,0.,0.)) ;
#58717=DIRECTION('center_axis',(-1.,0.,0.)) ;
#58718=DIRECTION('ref_axis',(0.,-1.,0.)) ;
#58719=DIRECTION('',(0.,0.,-1.)) ;
#58720=DIRECTION('',(0.,1.,5.60383084497428E-34)) ;
#58721=DIRECTION('center_axis',(0.,0.,-1.)) ;
#58722=DIRECTION('ref_axis',(-1.,0.,0.)) ;
#58723=DIRECTION('center_axis',(-1.,0.,0.)) ;
#58724=DIRECTION('ref_axis',(0.,1.,0.)) ;
#58725=DIRECTION('center_axis',(0.,4.44089209849993E-14,1.)) ;
#58726=DIRECTION('ref_axis',(1.,0.,0.)) ;
#58727=DIRECTION('center_axis',(0.,1.,0.)) ;
#58728=DIRECTION('ref_axis',(0.,0.,-1.)) ;
#58729=DIRECTION('center_axis',(0.,0.,1.)) ;
#58730=DIRECTION('ref_axis',(1.,0.,0.)) ;
#58731=DIRECTION('center_axis',(4.44089209850072E-14,0.,1.)) ;
#58732=DIRECTION('ref_axis',(0.,1.,0.)) ;
#58733=DIRECTION('center_axis',(-1.,0.,0.)) ;
#58734=DIRECTION('ref_axis',(0.,0.,-1.)) ;
#58735=DIRECTION('center_axis',(0.,-1.,0.)) ;
#58736=DIRECTION('ref_axis',(-1.,0.,0.)) ;
#58737=DIRECTION('center_axis',(-1.,0.,-1.51760508056877E-16)) ;
#58738=DIRECTION('ref_axis',(1.07310884363343E-16,-0.707106781186485,-0.70710678118661)) ;
#58739=DIRECTION('center_axis',(1.,0.,0.)) ;
#58740=DIRECTION('ref_axis',(0.,-1.,0.)) ;
#58741=DIRECTION('',(-1.,0.,-1.51760508056877E-16)) ;
#58742=DIRECTION('center_axis',(1.51760508056877E-16,5.60383084497428E-34,
-1.)) ;
#58743=DIRECTION('ref_axis',(-1.,0.,0.)) ;
#58744=DIRECTION('center_axis',(0.707106781186592,0.707106781186503,0.)) ;
#58745=DIRECTION('ref_axis',(0.707106781186503,-0.707106781186592,0.)) ;
#58746=DIRECTION('center_axis',(-1.51760508056877E-16,-5.60383084497428E-34,
1.)) ;
#58747=DIRECTION('ref_axis',(-0.38268343236507,0.923879532511295,-5.80762321206726E-17)) ;
#58748=DIRECTION('center_axis',(0.707106781186563,0.707106781186532,1.07310884363336E-16)) ;
#58749=DIRECTION('ref_axis',(0.499999999999956,-0.499999999999978,-0.707106781186594)) ;
#58750=DIRECTION('center_axis',(0.707106781186503,0.707106781186592,0.)) ;
#58751=DIRECTION('ref_axis',(0.707106781186592,-0.707106781186503,0.)) ;
#58752=DIRECTION('',(-0.707106781186563,-0.707106781186532,-1.07310884363336E-16)) ;
#58753=DIRECTION('center_axis',(1.51760508056877E-16,5.60383084497428E-34,
-1.)) ;
#58754=DIRECTION('ref_axis',(-1.,0.,0.)) ;
#58755=DIRECTION('center_axis',(0.,1.,0.)) ;
#58756=DIRECTION('ref_axis',(1.,0.,0.)) ;
#58757=DIRECTION('center_axis',(-1.51760508056877E-16,-5.60383084497428E-34,
1.)) ;
#58758=DIRECTION('ref_axis',(-0.923879532511313,0.382683432365025,-1.40208427237267E-16)) ;
#58759=DIRECTION('center_axis',(-3.73034936274055E-14,-1.,-5.66175752827605E-30)) ;
#58760=DIRECTION('ref_axis',(0.707106781186579,-2.63775533058888E-14,-0.707106781186516)) ;
#58761=DIRECTION('center_axis',(0.,1.,0.)) ;
#58762=DIRECTION('ref_axis',(1.,0.,0.)) ;
#58763=DIRECTION('',(-3.73034936274055E-14,-1.,-5.66175752827605E-30)) ;
#58764=DIRECTION('center_axis',(1.51760508056877E-16,5.60383084497428E-34,
-1.)) ;
#58765=DIRECTION('ref_axis',(-1.,0.,0.)) ;
#58766=DIRECTION('center_axis',(-0.707106781186636,0.707106781186459,0.)) ;
#58767=DIRECTION('ref_axis',(0.707106781186459,0.707106781186636,0.)) ;
#58768=DIRECTION('center_axis',(-1.51760508056877E-16,-5.60383084497428E-34,
1.)) ;
#58769=DIRECTION('ref_axis',(-0.923879532511313,-0.382683432365025,-1.40208427237267E-16)) ;
#58770=DIRECTION('center_axis',(-0.707106781186575,0.70710678118652,-1.07310884363338E-16)) ;
#58771=DIRECTION('ref_axis',(0.499999999999948,0.499999999999986,-0.707106781186594)) ;
#58772=DIRECTION('center_axis',(-0.707106781186503,0.707106781186592,0.)) ;
#58773=DIRECTION('ref_axis',(0.707106781186592,0.707106781186503,0.)) ;
#58774=DIRECTION('',(0.707106781186575,-0.70710678118652,1.07310884363338E-16)) ;
#58775=DIRECTION('center_axis',(1.51760508056877E-16,5.60383084497428E-34,
-1.)) ;
#58776=DIRECTION('ref_axis',(-1.,0.,0.)) ;
#58777=DIRECTION('center_axis',(-1.,0.,0.)) ;
#58778=DIRECTION('ref_axis',(0.,1.,0.)) ;
#58779=DIRECTION('center_axis',(-1.51760508056877E-16,-5.60383084497428E-34,
1.)) ;
#58780=DIRECTION('ref_axis',(-0.382683432364994,-0.923879532511326,-5.8076232120661E-17)) ;
#58781=DIRECTION('center_axis',(1.,-7.10542735760144E-15,1.51760508056877E-16)) ;
#58782=DIRECTION('ref_axis',(5.13160675215303E-15,0.707106781186736,-0.707106781186359)) ;
#58783=DIRECTION('',(1.,-7.10542735760144E-15,1.51760508056877E-16)) ;
#58784=DIRECTION('center_axis',(7.105427357601E-15,1.,1.07888364883526E-30)) ;
#58785=DIRECTION('ref_axis',(-0.707106781186516,5.02429586778786E-15,-0.707106781186579)) ;
#58786=DIRECTION('center_axis',(0.,-1.,0.)) ;
#58787=DIRECTION('ref_axis',(-0.707106781186516,0.,-0.707106781186579)) ;
#58788=DIRECTION('',(7.105427357601E-15,1.,1.07888364883526E-30)) ;
#58789=DIRECTION('center_axis',(0.,0.,1.)) ;
#58790=DIRECTION('ref_axis',(0.707106781186296,0.707106781186799,0.)) ;
#58791=DIRECTION('center_axis',(0.,-4.44089209849835E-14,1.)) ;
#58792=DIRECTION('ref_axis',(1.,0.,0.)) ;
#58793=DIRECTION('',(0.,0.,-1.)) ;
#58794=DIRECTION('',(0.,0.,1.)) ;
#58795=DIRECTION('center_axis',(-0.894427190999916,0.447213595499958,0.)) ;
#58796=DIRECTION('ref_axis',(-0.447213595499958,-0.894427190999916,0.)) ;
#58797=DIRECTION('center_axis',(0.447213595500021,-0.894427190999884,0.)) ;
#58798=DIRECTION('ref_axis',(-0.894427190999884,-0.447213595500021,0.)) ;
#58799=DIRECTION('center_axis',(0.,0.,1.)) ;
#58800=DIRECTION('ref_axis',(0.707106781186548,-0.707106781186548,0.)) ;
#58801=DIRECTION('center_axis',(4.44089209850072E-14,0.,1.)) ;
#58802=DIRECTION('ref_axis',(0.,-1.,0.)) ;
#58803=DIRECTION('',(0.,0.,-1.)) ;
#58804=DIRECTION('',(0.,0.,1.)) ;
#58805=DIRECTION('center_axis',(0.447213595500021,0.894427190999884,0.)) ;
#58806=DIRECTION('ref_axis',(-0.894427190999884,0.447213595500021,0.)) ;
#58807=DIRECTION('center_axis',(-0.894427190999916,-0.447213595499958,0.)) ;
#58808=DIRECTION('ref_axis',(-0.447213595499958,0.894427190999916,0.)) ;
#58809=DIRECTION('center_axis',(7.105427357601E-15,1.,1.07888364883526E-30)) ;
#58810=DIRECTION('ref_axis',(-0.707106781186516,5.02429586778786E-15,-0.707106781186579)) ;
#58811=DIRECTION('center_axis',(3.55271367880051E-14,1.,0.)) ;
#58812=DIRECTION('ref_axis',(-0.707106781186516,2.51214793389393E-14,-0.707106781186579)) ;
#58813=DIRECTION('',(7.105427357601E-15,1.,1.07888364883526E-30)) ;
#58814=DIRECTION('center_axis',(1.,-7.105427357601E-15,0.)) ;
#58815=DIRECTION('ref_axis',(7.105427357601E-15,1.,1.06039100704685E-30)) ;
#58816=DIRECTION('',(0.,0.,1.)) ;
#58817=DIRECTION('',(-7.105427357601E-15,-1.,-1.07888364883526E-30)) ;
#58818=DIRECTION('center_axis',(1.51760508056877E-16,5.60383084497428E-34,
-1.)) ;
#58819=DIRECTION('ref_axis',(-1.,0.,0.)) ;
#58820=DIRECTION('center_axis',(-1.,0.,0.)) ;
#58821=DIRECTION('ref_axis',(0.,0.,-1.)) ;
#58822=DIRECTION('center_axis',(0.,0.,1.)) ;
#58823=DIRECTION('ref_axis',(0.,1.,0.)) ;
#58824=DIRECTION('center_axis',(0.,1.,0.)) ;
#58825=DIRECTION('ref_axis',(0.707106781186548,0.,-0.707106781186548)) ;
#58826=DIRECTION('center_axis',(-1.,0.,-1.51760508056877E-16)) ;
#58827=DIRECTION('ref_axis',(1.07310884363343E-16,-0.707106781186485,-0.70710678118661)) ;
#58828=DIRECTION('center_axis',(-1.,0.,0.)) ;
#58829=DIRECTION('ref_axis',(0.,0.,-1.)) ;
#58830=DIRECTION('',(-1.,0.,-1.51760508056877E-16)) ;
#58831=DIRECTION('center_axis',(0.,-1.,-5.60383084497428E-34)) ;
#58832=DIRECTION('ref_axis',(0.707106781186548,3.96250679110365E-34,-0.707106781186548)) ;
#58833=DIRECTION('center_axis',(0.,-1.,0.)) ;
#58834=DIRECTION('ref_axis',(0.,0.,-1.)) ;
#58835=DIRECTION('',(0.,-1.,-5.60383084497428E-34)) ;
#58836=DIRECTION('center_axis',(0.,1.,0.)) ;
#58837=DIRECTION('ref_axis',(1.,0.,0.)) ;
#58838=DIRECTION('center_axis',(1.51760508056877E-16,5.60383084497428E-34,
-1.)) ;
#58839=DIRECTION('ref_axis',(-1.,0.,0.)) ;
#58840=DIRECTION('center_axis',(-1.,0.,0.)) ;
#58841=DIRECTION('ref_axis',(0.,0.,-1.)) ;
#58842=DIRECTION('center_axis',(-1.51760508056877E-16,-5.60383084497428E-34,
1.)) ;
#58843=DIRECTION('ref_axis',(-0.707106781186592,0.707106781186503,-1.0731088436334E-16)) ;
#58844=DIRECTION('center_axis',(-1.,0.,-1.51760508056877E-16)) ;
#58845=DIRECTION('ref_axis',(1.07310884363343E-16,-0.707106781186485,-0.70710678118661)) ;
#58846=DIRECTION('center_axis',(-1.,0.,0.)) ;
#58847=DIRECTION('ref_axis',(0.,0.,-1.)) ;
#58848=DIRECTION('',(-1.,0.,-1.51760508056877E-16)) ;
#58849=DIRECTION('center_axis',(1.51760508056877E-16,5.60383084497428E-34,
-1.)) ;
#58850=DIRECTION('ref_axis',(-1.,0.,0.)) ;
#58851=DIRECTION('center_axis',(0.,1.,0.)) ;
#58852=DIRECTION('ref_axis',(0.,0.,-1.)) ;
#58853=DIRECTION('center_axis',(-1.51760508056877E-16,-5.60383084497428E-34,
1.)) ;
#58854=DIRECTION('ref_axis',(0.707106781186592,0.707106781186503,1.0731088436334E-16)) ;
#58855=DIRECTION('center_axis',(0.,1.,5.60383084497428E-34)) ;
#58856=DIRECTION('ref_axis',(-0.707106781186548,3.96250679110365E-34,-0.707106781186548)) ;
#58857=DIRECTION('center_axis',(0.,1.,0.)) ;
#58858=DIRECTION('ref_axis',(0.,0.,-1.)) ;
#58859=DIRECTION('',(0.,1.,5.60383084497428E-34)) ;
#58860=DIRECTION('center_axis',(-0.408248290463679,-0.816496580927927,0.408248290463644)) ;
#58861=DIRECTION('ref_axis',(0.577350269189732,-0.577350269189448,-0.577350269189697)) ;
#58862=DIRECTION('center_axis',(0.,0.,-1.)) ;
#58863=DIRECTION('ref_axis',(0.707106781186636,-0.707106781186459,0.)) ;
#58864=DIRECTION('center_axis',(-1.,0.,-1.51760508056877E-16)) ;
#58865=DIRECTION('ref_axis',(1.07310884363343E-16,-0.707106781186485,-0.70710678118661)) ;
#58866=DIRECTION('center_axis',(-1.,0.,0.)) ;
#58867=DIRECTION('ref_axis',(0.,0.,-1.)) ;
#58868=DIRECTION('',(-1.,0.,-1.51760508056877E-16)) ;
#58869=DIRECTION('center_axis',(1.,0.,0.)) ;
#58870=DIRECTION('ref_axis',(0.,-1.,0.)) ;
#58871=DIRECTION('center_axis',(1.51760508056877E-16,5.60383084497428E-34,
-1.)) ;
#58872=DIRECTION('ref_axis',(-1.,0.,0.)) ;
#58873=DIRECTION('center_axis',(0.,1.,0.)) ;
#58874=DIRECTION('ref_axis',(-0.707106781186548,0.,-0.707106781186548)) ;
#58875=DIRECTION('center_axis',(0.,0.,-1.)) ;
#58876=DIRECTION('ref_axis',(0.,1.,0.)) ;
#58877=DIRECTION('center_axis',(-0.816496580927726,0.408248290463863,0.408248290463863)) ;
#58878=DIRECTION('ref_axis',(-0.577350269189614,-0.577350269189756,-0.577350269189507)) ;
#58879=DIRECTION('center_axis',(0.,0.,-1.)) ;
#58880=DIRECTION('ref_axis',(-0.707106781186681,-0.707106781186414,0.)) ;
#58881=DIRECTION('center_axis',(0.,1.,0.)) ;
#58882=DIRECTION('ref_axis',(-1.,0.,-1.4923676700635E-16)) ;
#58883=DIRECTION('',(0.,0.,-1.)) ;
#58884=DIRECTION('',(1.,0.,1.51760508056877E-16)) ;
#58885=DIRECTION('',(0.,0.,1.)) ;
#58886=DIRECTION('center_axis',(0.,0.,1.)) ;
#58887=DIRECTION('ref_axis',(0.70710678118661,-0.707106781186485,0.)) ;
#58888=DIRECTION('',(0.,0.,1.)) ;
#58889=DIRECTION('center_axis',(0.,0.,1.)) ;
#58890=DIRECTION('ref_axis',(1.,0.,0.)) ;
#58891=DIRECTION('center_axis',(-1.,0.,0.)) ;
#58892=DIRECTION('ref_axis',(0.,-1.,0.)) ;
#58893=DIRECTION('',(0.,0.,-1.)) ;
#58894=DIRECTION('',(0.,1.,5.60383084497428E-34)) ;
#58895=DIRECTION('center_axis',(0.,0.,1.)) ;
#58896=DIRECTION('ref_axis',(-0.70710678118661,0.707106781186485,0.)) ;
#58897=DIRECTION('',(0.,0.,1.)) ;
#58898=DIRECTION('center_axis',(0.,0.,-1.)) ;
#58899=DIRECTION('ref_axis',(0.,1.,0.)) ;
#58900=DIRECTION('center_axis',(0.,1.,0.)) ;
#58901=DIRECTION('ref_axis',(-1.,0.,-1.4923676700635E-16)) ;
#58902=DIRECTION('',(0.,0.,-1.)) ;
#58903=DIRECTION('',(1.,0.,1.51760508056877E-16)) ;
#58904=DIRECTION('center_axis',(0.,0.,1.)) ;
#58905=DIRECTION('ref_axis',(0.70710678118661,0.707106781186485,0.)) ;
#58906=DIRECTION('',(0.,0.,1.)) ;
#58907=DIRECTION('center_axis',(0.,0.,-1.)) ;
#58908=DIRECTION('ref_axis',(1.,0.,0.)) ;
#58909=DIRECTION('center_axis',(1.,0.,0.)) ;
#58910=DIRECTION('ref_axis',(0.,1.,0.)) ;
#58911=DIRECTION('',(0.,0.,-1.)) ;
#58912=DIRECTION('',(0.,-1.,-5.60383084497428E-34)) ;
#58913=DIRECTION('center_axis',(0.,0.,1.)) ;
#58914=DIRECTION('ref_axis',(-0.707106781186673,-0.707106781186422,0.)) ;
#58915=DIRECTION('',(0.,0.,1.)) ;
#58916=DIRECTION('center_axis',(0.,0.,1.)) ;
#58917=DIRECTION('ref_axis',(0.,-1.,0.)) ;
#58918=DIRECTION('center_axis',(0.,1.,0.)) ;
#58919=DIRECTION('ref_axis',(-1.,0.,-1.4923676700635E-16)) ;
#58920=DIRECTION('',(0.,0.,-1.)) ;
#58921=DIRECTION('',(1.,0.,1.51760508056877E-16)) ;
#58922=DIRECTION('center_axis',(1.51760508056877E-16,5.60383084497428E-34,
-1.)) ;
#58923=DIRECTION('ref_axis',(-1.,0.,0.)) ;
#58924=DIRECTION('center_axis',(-1.,0.,0.)) ;
#58925=DIRECTION('ref_axis',(0.,0.,-1.)) ;
#58926=DIRECTION('center_axis',(0.,0.,1.)) ;
#58927=DIRECTION('ref_axis',(0.,1.,0.)) ;
#58928=DIRECTION('center_axis',(0.,1.,0.)) ;
#58929=DIRECTION('ref_axis',(0.707106781186548,0.,-0.707106781186548)) ;
#58930=DIRECTION('center_axis',(-1.,0.,-1.51760508056877E-16)) ;
#58931=DIRECTION('ref_axis',(1.07310884363343E-16,-0.707106781186485,-0.70710678118661)) ;
#58932=DIRECTION('center_axis',(-1.,0.,0.)) ;
#58933=DIRECTION('ref_axis',(0.,0.,-1.)) ;
#58934=DIRECTION('',(-1.,0.,-1.51760508056877E-16)) ;
#58935=DIRECTION('center_axis',(0.,-1.,-5.60383084497428E-34)) ;
#58936=DIRECTION('ref_axis',(0.707106781186548,3.96250679110365E-34,-0.707106781186548)) ;
#58937=DIRECTION('center_axis',(0.,-1.,0.)) ;
#58938=DIRECTION('ref_axis',(0.,0.,-1.)) ;
#58939=DIRECTION('',(0.,-1.,-5.60383084497428E-34)) ;
#58940=DIRECTION('center_axis',(0.,1.,0.)) ;
#58941=DIRECTION('ref_axis',(1.,0.,0.)) ;
#58942=DIRECTION('center_axis',(1.51760508056877E-16,5.60383084497428E-34,
-1.)) ;
#58943=DIRECTION('ref_axis',(-1.,0.,0.)) ;
#58944=DIRECTION('center_axis',(-1.,0.,0.)) ;
#58945=DIRECTION('ref_axis',(0.,0.,-1.)) ;
#58946=DIRECTION('center_axis',(-1.51760508056877E-16,-5.60383084497428E-34,
1.)) ;
#58947=DIRECTION('ref_axis',(-0.707106781186636,0.707106781186459,-1.07310884363347E-16)) ;
#58948=DIRECTION('center_axis',(-1.,0.,-1.51760508056877E-16)) ;
#58949=DIRECTION('ref_axis',(1.07310884363343E-16,-0.707106781186485,-0.70710678118661)) ;
#58950=DIRECTION('center_axis',(-1.,0.,0.)) ;
#58951=DIRECTION('ref_axis',(0.,0.,-1.)) ;
#58952=DIRECTION('',(-1.,0.,-1.51760508056877E-16)) ;
#58953=DIRECTION('center_axis',(1.51760508056877E-16,5.60383084497428E-34,
-1.)) ;
#58954=DIRECTION('ref_axis',(-1.,0.,0.)) ;
#58955=DIRECTION('center_axis',(0.,1.,0.)) ;
#58956=DIRECTION('ref_axis',(0.,0.,-1.)) ;
#58957=DIRECTION('center_axis',(-1.51760508056877E-16,-5.60383084497428E-34,
1.)) ;
#58958=DIRECTION('ref_axis',(0.707106781186592,0.707106781186503,1.0731088436334E-16)) ;
#58959=DIRECTION('center_axis',(0.,1.,5.60383084497428E-34)) ;
#58960=DIRECTION('ref_axis',(-0.707106781186548,3.96250679110365E-34,-0.707106781186548)) ;
#58961=DIRECTION('center_axis',(0.,1.,0.)) ;
#58962=DIRECTION('ref_axis',(0.,0.,-1.)) ;
#58963=DIRECTION('',(0.,1.,5.60383084497428E-34)) ;
#58964=DIRECTION('center_axis',(-0.40824829046362,-0.816496580927951,0.408248290463656)) ;
#58965=DIRECTION('ref_axis',(0.577350269189721,-0.577350269189436,-0.577350269189721)) ;
#58966=DIRECTION('center_axis',(0.,0.,-1.)) ;
#58967=DIRECTION('ref_axis',(0.707106781186636,-0.707106781186459,0.)) ;
#58968=DIRECTION('center_axis',(-1.,0.,-1.51760508056877E-16)) ;
#58969=DIRECTION('ref_axis',(1.07310884363343E-16,-0.707106781186485,-0.70710678118661)) ;
#58970=DIRECTION('center_axis',(-1.,0.,0.)) ;
#58971=DIRECTION('ref_axis',(0.,0.,-1.)) ;
#58972=DIRECTION('',(-1.,0.,-1.51760508056877E-16)) ;
#58973=DIRECTION('center_axis',(1.,0.,0.)) ;
#58974=DIRECTION('ref_axis',(0.,-1.,0.)) ;
#58975=DIRECTION('center_axis',(1.51760508056877E-16,5.60383084497428E-34,
-1.)) ;
#58976=DIRECTION('ref_axis',(-1.,0.,0.)) ;
#58977=DIRECTION('center_axis',(0.,1.,0.)) ;
#58978=DIRECTION('ref_axis',(-0.707106781186548,0.,-0.707106781186548)) ;
#58979=DIRECTION('center_axis',(0.,0.,-1.)) ;
#58980=DIRECTION('ref_axis',(0.,1.,0.)) ;
#58981=DIRECTION('center_axis',(-0.81649658092775,0.408248290463875,0.408248290463804)) ;
#58982=DIRECTION('ref_axis',(-0.577350269189602,-0.577350269189744,-0.577350269189531)) ;
#58983=DIRECTION('center_axis',(0.,0.,-1.)) ;
#58984=DIRECTION('ref_axis',(-0.707106781186636,-0.707106781186459,0.)) ;
#58985=DIRECTION('center_axis',(0.,1.,0.)) ;
#58986=DIRECTION('ref_axis',(-1.,0.,-1.4923676700635E-16)) ;
#58987=DIRECTION('',(0.,0.,-1.)) ;
#58988=DIRECTION('',(1.,0.,1.51760508056877E-16)) ;
#58989=DIRECTION('',(0.,0.,1.)) ;
#58990=DIRECTION('center_axis',(0.,0.,1.)) ;
#58991=DIRECTION('ref_axis',(0.70710678118661,-0.707106781186485,0.)) ;
#58992=DIRECTION('',(0.,0.,1.)) ;
#58993=DIRECTION('center_axis',(0.,0.,1.)) ;
#58994=DIRECTION('ref_axis',(1.,0.,0.)) ;
#58995=DIRECTION('center_axis',(-1.,0.,0.)) ;
#58996=DIRECTION('ref_axis',(0.,-1.,0.)) ;
#58997=DIRECTION('',(0.,0.,-1.)) ;
#58998=DIRECTION('',(0.,1.,5.60383084497428E-34)) ;
#58999=DIRECTION('center_axis',(0.,0.,1.)) ;
#59000=DIRECTION('ref_axis',(-0.707106781186673,0.707106781186422,0.)) ;
#59001=DIRECTION('',(0.,0.,1.)) ;
#59002=DIRECTION('center_axis',(0.,0.,-1.)) ;
#59003=DIRECTION('ref_axis',(0.,1.,0.)) ;
#59004=DIRECTION('center_axis',(0.,1.,0.)) ;
#59005=DIRECTION('ref_axis',(-1.,0.,-1.4923676700635E-16)) ;
#59006=DIRECTION('',(0.,0.,-1.)) ;
#59007=DIRECTION('',(1.,0.,1.51760508056877E-16)) ;
#59008=DIRECTION('center_axis',(0.,0.,1.)) ;
#59009=DIRECTION('ref_axis',(0.70710678118661,0.707106781186485,0.)) ;
#59010=DIRECTION('',(0.,0.,1.)) ;
#59011=DIRECTION('center_axis',(0.,0.,-1.)) ;
#59012=DIRECTION('ref_axis',(1.,0.,0.)) ;
#59013=DIRECTION('center_axis',(1.,0.,0.)) ;
#59014=DIRECTION('ref_axis',(0.,1.,0.)) ;
#59015=DIRECTION('',(0.,0.,-1.)) ;
#59016=DIRECTION('',(0.,-1.,-5.60383084497428E-34)) ;
#59017=DIRECTION('center_axis',(0.,0.,1.)) ;
#59018=DIRECTION('ref_axis',(-0.70710678118661,-0.707106781186485,0.)) ;
#59019=DIRECTION('',(0.,0.,1.)) ;
#59020=DIRECTION('center_axis',(0.,0.,1.)) ;
#59021=DIRECTION('ref_axis',(0.,-1.,0.)) ;
#59022=DIRECTION('center_axis',(0.,1.,0.)) ;
#59023=DIRECTION('ref_axis',(-1.,0.,-1.4923676700635E-16)) ;
#59024=DIRECTION('',(0.,0.,-1.)) ;
#59025=DIRECTION('',(1.,0.,1.51760508056877E-16)) ;
#59026=DIRECTION('center_axis',(0.,1.,5.60383084497428E-34)) ;
#59027=DIRECTION('ref_axis',(-0.707106781186548,3.96250679110365E-34,-0.707106781186548)) ;
#59028=DIRECTION('center_axis',(0.,1.,0.)) ;
#59029=DIRECTION('ref_axis',(0.,0.,-1.)) ;
#59030=DIRECTION('center_axis',(-1.,0.,-1.51760508056877E-16)) ;
#59031=DIRECTION('ref_axis',(1.07310884363343E-16,-0.707106781186485,-0.70710678118661)) ;
#59032=DIRECTION('center_axis',(-1.,0.,0.)) ;
#59033=DIRECTION('ref_axis',(0.,0.,-1.)) ;
#59034=DIRECTION('',(-1.,0.,-1.51760508056877E-16)) ;
#59035=DIRECTION('center_axis',(1.,0.,0.)) ;
#59036=DIRECTION('ref_axis',(0.,-1.,0.)) ;
#59037=DIRECTION('center_axis',(1.51760508056877E-16,5.60383084497428E-34,
-1.)) ;
#59038=DIRECTION('ref_axis',(-1.,0.,0.)) ;
#59039=DIRECTION('center_axis',(0.,1.,0.)) ;
#59040=DIRECTION('ref_axis',(-0.707106781186548,0.,-0.707106781186548)) ;
#59041=DIRECTION('center_axis',(0.,0.,-1.)) ;
#59042=DIRECTION('ref_axis',(0.,1.,0.)) ;
#59043=DIRECTION('center_axis',(-0.816496580927773,0.408248290463851,0.40824829046378)) ;
#59044=DIRECTION('ref_axis',(-0.577350269189543,-0.577350269189756,-0.577350269189578)) ;
#59045=DIRECTION('center_axis',(0.,1.,0.)) ;
#59046=DIRECTION('ref_axis',(-1.,0.,-1.4923676700635E-16)) ;
#59047=DIRECTION('',(0.,0.,-1.)) ;
#59048=DIRECTION('center_axis',(0.,-1.,-5.60383084497428E-34)) ;
#59049=DIRECTION('ref_axis',(0.707106781186548,3.96250679110365E-34,-0.707106781186548)) ;
#59050=DIRECTION('',(0.,-1.,-5.60383084497428E-34)) ;
#59051=DIRECTION('center_axis',(1.51760508056877E-16,5.60383084497428E-34,
-1.)) ;
#59052=DIRECTION('ref_axis',(-1.,0.,0.)) ;
#59053=DIRECTION('center_axis',(0.,0.,1.)) ;
#59054=DIRECTION('ref_axis',(0.,1.,0.)) ;
#59055=DIRECTION('center_axis',(0.,1.,0.)) ;
#59056=DIRECTION('ref_axis',(0.707106781186548,0.,-0.707106781186548)) ;
#59057=DIRECTION('center_axis',(-1.,0.,0.)) ;
#59058=DIRECTION('ref_axis',(0.,-1.,0.)) ;
#59059=DIRECTION('center_axis',(1.,0.,1.51760508056877E-16)) ;
#59060=DIRECTION('ref_axis',(1.07310884363343E-16,0.707106781186485,-0.70710678118661)) ;
#59061=DIRECTION('',(1.,0.,1.51760508056877E-16)) ;
#59062=DIRECTION('center_axis',(-1.,0.,0.)) ;
#59063=DIRECTION('ref_axis',(0.,1.,0.)) ;
#59064=DIRECTION('center_axis',(1.51760508056877E-16,5.60383084497428E-34,
-1.)) ;
#59065=DIRECTION('ref_axis',(-1.,0.,0.)) ;
#59066=DIRECTION('center_axis',(-0.707106781186636,-0.707106781186459,0.)) ;
#59067=DIRECTION('ref_axis',(-0.707106781186459,0.707106781186636,0.)) ;
#59068=DIRECTION('center_axis',(-1.51760508056877E-16,-5.60383084497428E-34,
1.)) ;
#59069=DIRECTION('ref_axis',(0.382683432364994,-0.923879532511326,5.8076232120661E-17)) ;
#59070=DIRECTION('center_axis',(-0.707106781186555,-0.70710678118654,-1.07310884363335E-16)) ;
#59071=DIRECTION('ref_axis',(-0.499999999999931,0.499999999999941,-0.707106781186638)) ;
#59072=DIRECTION('center_axis',(-0.707106781186592,-0.707106781186503,0.)) ;
#59073=DIRECTION('ref_axis',(-0.707106781186503,0.707106781186592,0.)) ;
#59074=DIRECTION('',(0.707106781186555,0.70710678118654,1.07310884363335E-16)) ;
#59075=DIRECTION('center_axis',(1.51760508056877E-16,5.60383084497428E-34,
-1.)) ;
#59076=DIRECTION('ref_axis',(-1.,0.,0.)) ;
#59077=DIRECTION('center_axis',(0.,-1.,0.)) ;
#59078=DIRECTION('ref_axis',(-1.,0.,0.)) ;
#59079=DIRECTION('center_axis',(-1.51760508056877E-16,-5.60383084497428E-34,
1.)) ;
#59080=DIRECTION('ref_axis',(0.923879532511313,-0.382683432365025,1.40208427237267E-16)) ;
#59081=DIRECTION('center_axis',(0.,1.,5.60383084497428E-34)) ;
#59082=DIRECTION('ref_axis',(-0.707106781186548,3.96250679110365E-34,-0.707106781186548)) ;
#59083=DIRECTION('center_axis',(0.,-1.,0.)) ;
#59084=DIRECTION('ref_axis',(-1.,0.,0.)) ;
#59085=DIRECTION('',(0.,1.,5.60383084497428E-34)) ;
#59086=DIRECTION('center_axis',(1.51760508056877E-16,5.60383084497428E-34,
-1.)) ;
#59087=DIRECTION('ref_axis',(-1.,0.,0.)) ;
#59088=DIRECTION('center_axis',(0.707106781186459,-0.707106781186636,0.)) ;
#59089=DIRECTION('ref_axis',(-0.707106781186636,-0.707106781186459,0.)) ;
#59090=DIRECTION('center_axis',(-1.51760508056877E-16,-5.60383084497428E-34,
1.)) ;
#59091=DIRECTION('ref_axis',(0.923879532511313,0.382683432365025,1.40208427237267E-16)) ;
#59092=DIRECTION('center_axis',(0.707106781186555,-0.70710678118654,1.07310884363335E-16)) ;
#59093=DIRECTION('ref_axis',(-0.499999999999962,-0.499999999999972,-0.707106781186594)) ;
#59094=DIRECTION('center_axis',(0.707106781186503,-0.707106781186592,0.)) ;
#59095=DIRECTION('ref_axis',(-0.707106781186592,-0.707106781186503,0.)) ;
#59096=DIRECTION('',(-0.707106781186555,0.70710678118654,-1.07310884363335E-16)) ;
#59097=DIRECTION('center_axis',(1.51760508056877E-16,5.60383084497428E-34,
-1.)) ;
#59098=DIRECTION('ref_axis',(-1.,0.,0.)) ;
#59099=DIRECTION('center_axis',(1.,0.,0.)) ;
#59100=DIRECTION('ref_axis',(0.,-1.,0.)) ;
#59101=DIRECTION('center_axis',(-1.51760508056877E-16,-5.60383084497428E-34,
1.)) ;
#59102=DIRECTION('ref_axis',(0.382683432364994,0.923879532511326,5.8076232120661E-17)) ;
#59103=DIRECTION('center_axis',(-1.,0.,-1.51760508056877E-16)) ;
#59104=DIRECTION('ref_axis',(1.07310884363343E-16,-0.707106781186485,-0.70710678118661)) ;
#59105=DIRECTION('',(-1.,0.,-1.51760508056877E-16)) ;
#59106=DIRECTION('center_axis',(0.,1.,0.)) ;
#59107=DIRECTION('ref_axis',(-1.,0.,-1.4923676700635E-16)) ;
#59108=DIRECTION('',(0.,0.,-1.)) ;
#59109=DIRECTION('',(1.,0.,1.51760508056877E-16)) ;
#59110=DIRECTION('center_axis',(0.,0.,-1.)) ;
#59111=DIRECTION('ref_axis',(0.382683432365017,0.923879532511317,0.)) ;
#59112=DIRECTION('',(0.,0.,1.)) ;
#59113=DIRECTION('center_axis',(-4.44089209850105E-14,4.44089209849993E-14,
-1.)) ;
#59114=DIRECTION('ref_axis',(0.707106781186459,0.707106781186636,-6.25253024584262E-29)) ;
#59115=DIRECTION('center_axis',(-0.70710678118654,-0.707106781186555,0.)) ;
#59116=DIRECTION('ref_axis',(0.,0.,1.)) ;
#59117=DIRECTION('',(0.,0.,-1.)) ;
#59118=DIRECTION('',(0.707106781186555,-0.70710678118654,1.07310884363335E-16)) ;
#59119=DIRECTION('center_axis',(0.,0.,1.)) ;
#59120=DIRECTION('ref_axis',(0.923879532511311,0.382683432365031,0.)) ;
#59121=DIRECTION('',(0.,0.,1.)) ;
#59122=DIRECTION('center_axis',(0.,-6.28036983473606E-14,-1.)) ;
#59123=DIRECTION('ref_axis',(1.,0.,0.)) ;
#59124=DIRECTION('center_axis',(1.,0.,0.)) ;
#59125=DIRECTION('ref_axis',(0.,1.,0.)) ;
#59126=DIRECTION('',(0.,0.,-1.)) ;
#59127=DIRECTION('',(0.,-1.,-5.60383084497428E-34)) ;
#59128=DIRECTION('center_axis',(0.,0.,-1.)) ;
#59129=DIRECTION('ref_axis',(0.923879532511311,-0.382683432365031,0.)) ;
#59130=DIRECTION('',(0.,0.,1.)) ;
#59131=DIRECTION('center_axis',(4.44089209850072E-14,4.44089209850128E-14,
-1.)) ;
#59132=DIRECTION('ref_axis',(0.707106781186592,-0.707106781186503,-9.0726912223815E-30)) ;
#59133=DIRECTION('center_axis',(-0.70710678118654,0.707106781186555,0.)) ;
#59134=DIRECTION('ref_axis',(0.,0.,1.)) ;
#59135=DIRECTION('',(0.,0.,-1.)) ;
#59136=DIRECTION('',(-0.707106781186555,-0.70710678118654,-1.07310884363335E-16)) ;
#59137=DIRECTION('center_axis',(0.,0.,1.)) ;
#59138=DIRECTION('ref_axis',(0.382683432365017,-0.923879532511317,0.)) ;
#59139=DIRECTION('',(0.,0.,1.)) ;
#59140=DIRECTION('center_axis',(0.,0.,-1.)) ;
#59141=DIRECTION('ref_axis',(0.,-1.,0.)) ;
#59142=DIRECTION('center_axis',(0.,-1.,0.)) ;
#59143=DIRECTION('ref_axis',(1.,0.,1.4923676700635E-16)) ;
#59144=DIRECTION('',(-1.,0.,-1.51760508056877E-16)) ;
#59145=DIRECTION('center_axis',(0.,0.,1.)) ;
#59146=DIRECTION('ref_axis',(-0.707106781186673,0.707106781186422,0.)) ;
#59147=DIRECTION('',(0.,0.,-1.)) ;
#59148=DIRECTION('center_axis',(1.51760508056877E-16,5.60383084497428E-34,
-1.)) ;
#59149=DIRECTION('ref_axis',(-1.,0.,0.)) ;
#59150=DIRECTION('center_axis',(-1.,0.,0.)) ;
#59151=DIRECTION('ref_axis',(0.,1.,4.44089209849993E-14)) ;
#59152=DIRECTION('center_axis',(0.,0.,1.)) ;
#59153=DIRECTION('ref_axis',(0.,-1.,0.)) ;
#59154=DIRECTION('center_axis',(0.,-1.,0.)) ;
#59155=DIRECTION('ref_axis',(-0.707106781186548,0.,-0.707106781186548)) ;
#59156=DIRECTION('center_axis',(0.,-1.,0.)) ;
#59157=DIRECTION('ref_axis',(1.,0.,1.4923676700635E-16)) ;
#59158=DIRECTION('',(1.,0.,1.51760508056877E-16)) ;
#59159=DIRECTION('',(0.,0.,-1.)) ;
#59160=DIRECTION('',(-1.,0.,-1.51760508056877E-16)) ;
#59161=DIRECTION('',(0.,0.,1.)) ;
#59162=DIRECTION('center_axis',(0.,0.,1.)) ;
#59163=DIRECTION('ref_axis',(1.,0.,0.)) ;
#59164=DIRECTION('center_axis',(0.,0.,-1.)) ;
#59165=DIRECTION('ref_axis',(1.,0.,0.)) ;
#59166=DIRECTION('center_axis',(0.,-1.,0.)) ;
#59167=DIRECTION('ref_axis',(0.,0.,1.)) ;
#59168=DIRECTION('center_axis',(0.,0.,1.)) ;
#59169=DIRECTION('ref_axis',(0.707106781186359,0.707106781186736,0.)) ;
#59170=DIRECTION('',(0.,0.,1.)) ;
#59171=DIRECTION('center_axis',(0.,0.,1.)) ;
#59172=DIRECTION('ref_axis',(1.,0.,0.)) ;
#59173=DIRECTION('center_axis',(1.,0.,0.)) ;
#59174=DIRECTION('ref_axis',(0.,1.,0.)) ;
#59175=DIRECTION('center_axis',(0.,0.,-1.)) ;
#59176=DIRECTION('ref_axis',(-1.,0.,0.)) ;
#59177=DIRECTION('center_axis',(0.,1.,0.)) ;
#59178=DIRECTION('ref_axis',(0.,0.,1.)) ;
#59179=DIRECTION('center_axis',(0.,0.,1.)) ;
#59180=DIRECTION('ref_axis',(1.,0.,0.)) ;
#59181=DIRECTION('center_axis',(0.,1.,0.)) ;
#59182=DIRECTION('ref_axis',(-1.,0.,0.)) ;
#59183=DIRECTION('center_axis',(4.44089209850072E-14,0.,-1.)) ;
#59184=DIRECTION('ref_axis',(0.,-1.,0.)) ;
#59185=DIRECTION('center_axis',(-1.,0.,0.)) ;
#59186=DIRECTION('ref_axis',(0.,0.,1.)) ;
#59187=DIRECTION('center_axis',(0.,-1.,-5.60383084497428E-34)) ;
#59188=DIRECTION('ref_axis',(-0.707106781186548,-3.96250679110365E-34,0.707106781186548)) ;
#59189=DIRECTION('',(0.,-1.,-5.60383084497428E-34)) ;
#59190=DIRECTION('center_axis',(0.,0.,1.)) ;
#59191=DIRECTION('ref_axis',(0.70710678118661,-0.707106781186485,0.)) ;
#59192=DIRECTION('',(0.,0.,-1.)) ;
#59193=DIRECTION('center_axis',(-1.,0.,-1.51760508056877E-16)) ;
#59194=DIRECTION('ref_axis',(-1.07310884363343E-16,0.707106781186485,0.70710678118661)) ;
#59195=DIRECTION('center_axis',(0.,0.,1.)) ;
#59196=DIRECTION('ref_axis',(1.,0.,0.)) ;
#59197=DIRECTION('center_axis',(0.,0.,1.)) ;
#59198=DIRECTION('ref_axis',(0.,-1.,0.)) ;
#59199=DIRECTION('center_axis',(1.,0.,0.)) ;
#59200=DIRECTION('ref_axis',(0.,0.,-1.)) ;
#59201=DIRECTION('center_axis',(0.,1.,0.)) ;
#59202=DIRECTION('ref_axis',(1.,0.,0.)) ;
#59203=DIRECTION('center_axis',(1.,0.,1.51760508056877E-16)) ;
#59204=DIRECTION('ref_axis',(1.07310884363343E-16,0.707106781186485,-0.70710678118661)) ;
#59205=DIRECTION('center_axis',(0.,-1.,-5.60383084497428E-34)) ;
#59206=DIRECTION('ref_axis',(0.707106781186548,3.96250679110365E-34,-0.707106781186548)) ;
#59207=DIRECTION('',(0.,-1.,-5.60383084497428E-34)) ;
#59208=DIRECTION('center_axis',(0.,0.,1.)) ;
#59209=DIRECTION('ref_axis',(-0.707106781186359,-0.707106781186736,0.)) ;
#59210=DIRECTION('',(0.,0.,1.)) ;
#59211=DIRECTION('center_axis',(0.,1.,5.60383084497428E-34)) ;
#59212=DIRECTION('ref_axis',(0.707106781186548,-3.96250679110365E-34,0.707106781186548)) ;
#59213=DIRECTION('',(0.,1.,5.60383084497428E-34)) ;
#59214=DIRECTION('center_axis',(1.,0.,0.)) ;
#59215=DIRECTION('ref_axis',(0.,1.,0.)) ;
#59216=DIRECTION('',(0.,1.,5.60383084497428E-34)) ;
#59217=DIRECTION('center_axis',(0.,1.,5.60383084497428E-34)) ;
#59218=DIRECTION('ref_axis',(-0.707106781186548,3.96250679110365E-34,-0.707106781186548)) ;
#59219=DIRECTION('center_axis',(-1.51760508056877E-16,-5.60383084497428E-34,
1.)) ;
#59220=DIRECTION('ref_axis',(1.,0.,0.)) ;
#59221=DIRECTION('center_axis',(-1.,0.,0.)) ;
#59222=DIRECTION('ref_axis',(0.,1.,0.)) ;
#59223=DIRECTION('center_axis',(0.,-1.,0.)) ;
#59224=DIRECTION('ref_axis',(0.707106781186548,0.,-0.707106781186548)) ;
#59225=DIRECTION('center_axis',(0.,0.,-1.)) ;
#59226=DIRECTION('ref_axis',(0.,-1.,0.)) ;
#59227=DIRECTION('center_axis',(1.51760508056877E-16,5.60383084497428E-34,
-1.)) ;
#59228=DIRECTION('ref_axis',(-1.,0.,0.)) ;
#59229=DIRECTION('center_axis',(-1.,0.,0.)) ;
#59230=DIRECTION('ref_axis',(0.,1.,0.)) ;
#59231=DIRECTION('center_axis',(0.,0.,1.)) ;
#59232=DIRECTION('ref_axis',(0.,-1.,0.)) ;
#59233=DIRECTION('center_axis',(0.,-1.,0.)) ;
#59234=DIRECTION('ref_axis',(-0.707106781186548,0.,-0.707106781186548)) ;
#59235=DIRECTION('center_axis',(0.,-1.,0.)) ;
#59236=DIRECTION('ref_axis',(1.,0.,1.4923676700635E-16)) ;
#59237=DIRECTION('',(1.,0.,1.51760508056877E-16)) ;
#59238=DIRECTION('',(0.,0.,-1.)) ;
#59239=DIRECTION('',(-1.,0.,-1.51760508056877E-16)) ;
#59240=DIRECTION('',(0.,0.,1.)) ;
#59241=DIRECTION('center_axis',(0.,0.,-1.)) ;
#59242=DIRECTION('ref_axis',(-1.,0.,0.)) ;
#59243=DIRECTION('center_axis',(1.,0.,0.)) ;
#59244=DIRECTION('ref_axis',(0.,0.,1.)) ;
#59245=DIRECTION('center_axis',(0.,-1.,0.)) ;
#59246=DIRECTION('ref_axis',(1.,0.,0.)) ;
#59247=DIRECTION('center_axis',(0.,0.,1.)) ;
#59248=DIRECTION('ref_axis',(1.,0.,0.)) ;
#59249=DIRECTION('center_axis',(-1.,0.,0.)) ;
#59250=DIRECTION('ref_axis',(0.,-1.,0.)) ;
#59251=DIRECTION('center_axis',(0.,-1.,0.)) ;
#59252=DIRECTION('ref_axis',(0.,0.,1.)) ;
#59253=DIRECTION('center_axis',(1.,0.,1.51760508056877E-16)) ;
#59254=DIRECTION('ref_axis',(-1.07310884363343E-16,-0.707106781186485,0.70710678118661)) ;
#59255=DIRECTION('center_axis',(-0.816496580927844,-0.40824829046378,0.408248290463709)) ;
#59256=DIRECTION('ref_axis',(0.577350269189507,-0.577350269189934,0.577350269189436)) ;
#59257=DIRECTION('center_axis',(-3.55271367880058E-13,-1.,0.)) ;
#59258=DIRECTION('ref_axis',(0.,0.,1.)) ;
#59259=DIRECTION('center_axis',(1.,0.,0.)) ;
#59260=DIRECTION('ref_axis',(0.,-1.,0.)) ;
#59261=DIRECTION('center_axis',(-0.816496580927762,0.408248290463881,-0.408248290463774)) ;
#59262=DIRECTION('ref_axis',(-0.577350269189602,-0.577350269189744,0.577350269189531)) ;
#59263=DIRECTION('center_axis',(-1.,-8.88178419699986E-14,0.)) ;
#59264=DIRECTION('ref_axis',(0.,0.,1.)) ;
#59265=DIRECTION('center_axis',(0.,-1.,0.)) ;
#59266=DIRECTION('ref_axis',(-1.,0.,0.)) ;
#59267=DIRECTION('center_axis',(0.,-1.,-5.60383084497428E-34)) ;
#59268=DIRECTION('ref_axis',(-0.707106781186548,-3.96250679110365E-34,0.707106781186548)) ;
#59269=DIRECTION('center_axis',(0.,0.,1.)) ;
#59270=DIRECTION('ref_axis',(1.,0.,0.)) ;
#59271=DIRECTION('center_axis',(0.,-1.,0.)) ;
#59272=DIRECTION('ref_axis',(1.,0.,0.)) ;
#59273=DIRECTION('center_axis',(0.,0.,-1.)) ;
#59274=DIRECTION('ref_axis',(0.,1.,0.)) ;
#59275=DIRECTION('center_axis',(1.,0.,0.)) ;
#59276=DIRECTION('ref_axis',(0.,0.,1.)) ;
#59277=DIRECTION('center_axis',(0.,0.,1.)) ;
#59278=DIRECTION('ref_axis',(1.,0.,0.)) ;
#59279=DIRECTION('center_axis',(-1.,0.,0.)) ;
#59280=DIRECTION('ref_axis',(0.,-1.,0.)) ;
#59281=DIRECTION('center_axis',(0.,0.,-1.)) ;
#59282=DIRECTION('ref_axis',(1.,0.,0.)) ;
#59283=DIRECTION('center_axis',(0.,-1.,0.)) ;
#59284=DIRECTION('ref_axis',(0.,0.,1.)) ;
#59285=DIRECTION('center_axis',(1.,0.,1.51760508056877E-16)) ;
#59286=DIRECTION('ref_axis',(-1.07310884363343E-16,-0.707106781186485,0.70710678118661)) ;
#59287=DIRECTION('center_axis',(0.,0.,1.)) ;
#59288=DIRECTION('ref_axis',(0.707106781186359,0.707106781186736,0.)) ;
#59289=DIRECTION('',(0.,0.,1.)) ;
#59290=DIRECTION('center_axis',(0.,0.,1.)) ;
#59291=DIRECTION('ref_axis',(1.,0.,0.)) ;
#59292=DIRECTION('center_axis',(1.,0.,0.)) ;
#59293=DIRECTION('ref_axis',(0.,1.,0.)) ;
#59294=DIRECTION('center_axis',(0.,0.,-1.)) ;
#59295=DIRECTION('ref_axis',(-1.,0.,0.)) ;
#59296=DIRECTION('center_axis',(0.,1.,0.)) ;
#59297=DIRECTION('ref_axis',(0.,0.,1.)) ;
#59298=DIRECTION('center_axis',(0.,0.,1.)) ;
#59299=DIRECTION('ref_axis',(1.,0.,0.)) ;
#59300=DIRECTION('center_axis',(0.,1.,0.)) ;
#59301=DIRECTION('ref_axis',(-1.,0.,0.)) ;
#59302=DIRECTION('center_axis',(-4.44089209850072E-14,0.,-1.)) ;
#59303=DIRECTION('ref_axis',(0.,-1.,0.)) ;
#59304=DIRECTION('center_axis',(-1.,0.,0.)) ;
#59305=DIRECTION('ref_axis',(0.,0.,1.)) ;
#59306=DIRECTION('center_axis',(0.,-1.,-5.60383084497428E-34)) ;
#59307=DIRECTION('ref_axis',(-0.707106781186548,-3.96250679110365E-34,0.707106781186548)) ;
#59308=DIRECTION('',(0.,-1.,-5.60383084497428E-34)) ;
#59309=DIRECTION('center_axis',(0.,0.,1.)) ;
#59310=DIRECTION('ref_axis',(0.70710678118661,-0.707106781186485,0.)) ;
#59311=DIRECTION('',(0.,0.,-1.)) ;
#59312=DIRECTION('center_axis',(-1.,0.,-1.51760508056877E-16)) ;
#59313=DIRECTION('ref_axis',(-1.07310884363343E-16,0.707106781186485,0.70710678118661)) ;
#59314=DIRECTION('center_axis',(0.,0.,1.)) ;
#59315=DIRECTION('ref_axis',(-0.707106781186359,-0.707106781186736,0.)) ;
#59316=DIRECTION('',(0.,0.,1.)) ;
#59317=DIRECTION('center_axis',(0.,1.,5.60383084497428E-34)) ;
#59318=DIRECTION('ref_axis',(0.707106781186548,-3.96250679110365E-34,0.707106781186548)) ;
#59319=DIRECTION('',(0.,1.,5.60383084497428E-34)) ;
#59320=DIRECTION('center_axis',(0.,0.,1.)) ;
#59321=DIRECTION('ref_axis',(-0.707106781186673,0.707106781186422,0.)) ;
#59322=DIRECTION('',(0.,0.,-1.)) ;
#59323=DIRECTION('center_axis',(1.,0.,1.51760508056877E-16)) ;
#59324=DIRECTION('ref_axis',(-1.07310884363343E-16,-0.707106781186485,0.70710678118661)) ;
#59325=DIRECTION('center_axis',(0.,1.,5.60383084497428E-34)) ;
#59326=DIRECTION('ref_axis',(0.707106781186548,-3.96250679110365E-34,0.707106781186548)) ;
#59327=DIRECTION('center_axis',(1.,0.,1.51760508056877E-16)) ;
#59328=DIRECTION('ref_axis',(1.07310884363343E-16,0.707106781186485,-0.70710678118661)) ;
#59329=DIRECTION('center_axis',(1.,0.,0.)) ;
#59330=DIRECTION('ref_axis',(0.,1.,0.)) ;
#59331=DIRECTION('',(0.,1.,5.60383084497428E-34)) ;
#59332=DIRECTION('center_axis',(0.,1.,5.60383084497428E-34)) ;
#59333=DIRECTION('ref_axis',(-0.707106781186548,3.96250679110365E-34,-0.707106781186548)) ;
#59334=DIRECTION('center_axis',(-1.51760508056877E-16,-5.60383084497428E-34,
1.)) ;
#59335=DIRECTION('ref_axis',(1.,0.,0.)) ;
#59336=DIRECTION('center_axis',(-1.,0.,0.)) ;
#59337=DIRECTION('ref_axis',(0.,1.,0.)) ;
#59338=DIRECTION('center_axis',(0.,-1.,0.)) ;
#59339=DIRECTION('ref_axis',(0.707106781186548,0.,-0.707106781186548)) ;
#59340=DIRECTION('center_axis',(0.,0.,-1.)) ;
#59341=DIRECTION('ref_axis',(0.,-1.,0.)) ;
#59342=DIRECTION('center_axis',(1.51760508056877E-16,5.60383084497428E-34,
-1.)) ;
#59343=DIRECTION('ref_axis',(-1.,0.,0.)) ;
#59344=DIRECTION('center_axis',(-1.,0.,0.)) ;
#59345=DIRECTION('ref_axis',(0.,1.,0.)) ;
#59346=DIRECTION('center_axis',(0.,0.,1.)) ;
#59347=DIRECTION('ref_axis',(0.,-1.,0.)) ;
#59348=DIRECTION('center_axis',(0.,-1.,0.)) ;
#59349=DIRECTION('ref_axis',(-0.707106781186548,0.,-0.707106781186548)) ;
#59350=DIRECTION('center_axis',(0.,-1.,0.)) ;
#59351=DIRECTION('ref_axis',(1.,0.,1.4923676700635E-16)) ;
#59352=DIRECTION('',(1.,0.,1.51760508056877E-16)) ;
#59353=DIRECTION('',(0.,0.,-1.)) ;
#59354=DIRECTION('',(-1.,0.,-1.51760508056877E-16)) ;
#59355=DIRECTION('',(0.,0.,1.)) ;
#59356=DIRECTION('center_axis',(0.,0.,1.)) ;
#59357=DIRECTION('ref_axis',(1.,0.,0.)) ;
#59358=DIRECTION('center_axis',(0.,-1.,0.)) ;
#59359=DIRECTION('ref_axis',(1.,0.,0.)) ;
#59360=DIRECTION('center_axis',(1.,0.,0.)) ;
#59361=DIRECTION('ref_axis',(0.,0.,1.)) ;
#59362=DIRECTION('center_axis',(-0.816496580927809,-0.408248290463869,0.408248290463691)) ;
#59363=DIRECTION('ref_axis',(0.577350269189507,-0.577350269189792,0.577350269189578)) ;
#59364=DIRECTION('center_axis',(-3.55271367880058E-13,-1.,0.)) ;
#59365=DIRECTION('ref_axis',(0.,0.,1.)) ;
#59366=DIRECTION('center_axis',(1.,0.,0.)) ;
#59367=DIRECTION('ref_axis',(0.,-1.,0.)) ;
#59368=DIRECTION('center_axis',(0.,1.,5.60383084497428E-34)) ;
#59369=DIRECTION('ref_axis',(0.707106781186548,-3.96250679110365E-34,0.707106781186548)) ;
#59370=DIRECTION('center_axis',(0.,0.,1.)) ;
#59371=DIRECTION('ref_axis',(1.,0.,0.)) ;
#59372=DIRECTION('center_axis',(-1.,0.,0.)) ;
#59373=DIRECTION('ref_axis',(0.,-1.,0.)) ;
#59374=DIRECTION('center_axis',(0.,-1.,0.)) ;
#59375=DIRECTION('ref_axis',(0.,0.,1.)) ;
#59376=DIRECTION('center_axis',(1.,0.,1.51760508056877E-16)) ;
#59377=DIRECTION('ref_axis',(-1.07310884363343E-16,-0.707106781186485,0.70710678118661)) ;
#59378=DIRECTION('center_axis',(0.,0.,1.)) ;
#59379=DIRECTION('ref_axis',(1.,0.,0.)) ;
#59380=DIRECTION('center_axis',(0.,-1.,0.)) ;
#59381=DIRECTION('ref_axis',(1.,0.,0.)) ;
#59382=DIRECTION('center_axis',(0.,0.,-1.)) ;
#59383=DIRECTION('ref_axis',(0.,1.,0.)) ;
#59384=DIRECTION('center_axis',(1.,0.,0.)) ;
#59385=DIRECTION('ref_axis',(0.,0.,1.)) ;
#59386=DIRECTION('center_axis',(-0.81649658092775,0.408248290463875,-0.408248290463804)) ;
#59387=DIRECTION('ref_axis',(-0.577350269189555,-0.577350269189768,0.577350269189555)) ;
#59388=DIRECTION('center_axis',(-1.,0.,0.)) ;
#59389=DIRECTION('ref_axis',(0.,0.,1.)) ;
#59390=DIRECTION('center_axis',(0.,-1.,0.)) ;
#59391=DIRECTION('ref_axis',(-1.,0.,0.)) ;
#59392=DIRECTION('center_axis',(0.,-1.,-5.60383084497428E-34)) ;
#59393=DIRECTION('ref_axis',(-0.707106781186548,-3.96250679110365E-34,0.707106781186548)) ;
#59394=DIRECTION('center_axis',(0.,0.,1.)) ;
#59395=DIRECTION('ref_axis',(1.,0.,0.)) ;
#59396=DIRECTION('center_axis',(1.,0.,0.)) ;
#59397=DIRECTION('ref_axis',(0.,1.,0.)) ;
#59398=DIRECTION('center_axis',(0.,0.,-1.)) ;
#59399=DIRECTION('ref_axis',(-1.,0.,0.)) ;
#59400=DIRECTION('center_axis',(0.,1.,0.)) ;
#59401=DIRECTION('ref_axis',(0.,0.,1.)) ;
#59402=DIRECTION('center_axis',(0.,0.,1.)) ;
#59403=DIRECTION('ref_axis',(1.,0.,0.)) ;
#59404=DIRECTION('center_axis',(-1.,0.,0.)) ;
#59405=DIRECTION('ref_axis',(0.,-1.,0.)) ;
#59406=DIRECTION('center_axis',(0.,0.,-1.)) ;
#59407=DIRECTION('ref_axis',(1.,0.,0.)) ;
#59408=DIRECTION('center_axis',(0.,-1.,0.)) ;
#59409=DIRECTION('ref_axis',(0.,0.,1.)) ;
#59410=DIRECTION('center_axis',(1.,0.,1.51760508056877E-16)) ;
#59411=DIRECTION('ref_axis',(-1.07310884363343E-16,-0.707106781186485,0.70710678118661)) ;
#59412=DIRECTION('center_axis',(0.,0.,1.)) ;
#59413=DIRECTION('ref_axis',(0.707106781186359,0.707106781186736,0.)) ;
#59414=DIRECTION('',(0.,0.,1.)) ;
#59415=DIRECTION('center_axis',(0.,0.,1.)) ;
#59416=DIRECTION('ref_axis',(1.,0.,0.)) ;
#59417=DIRECTION('center_axis',(0.,1.,0.)) ;
#59418=DIRECTION('ref_axis',(-1.,0.,0.)) ;
#59419=DIRECTION('center_axis',(0.,0.,-1.)) ;
#59420=DIRECTION('ref_axis',(0.,-1.,0.)) ;
#59421=DIRECTION('center_axis',(-1.,0.,0.)) ;
#59422=DIRECTION('ref_axis',(0.,0.,1.)) ;
#59423=DIRECTION('center_axis',(0.,-1.,-5.60383084497428E-34)) ;
#59424=DIRECTION('ref_axis',(-0.707106781186548,-3.96250679110365E-34,0.707106781186548)) ;
#59425=DIRECTION('',(0.,-1.,-5.60383084497428E-34)) ;
#59426=DIRECTION('center_axis',(0.,0.,1.)) ;
#59427=DIRECTION('ref_axis',(0.707106781186548,-0.707106781186548,0.)) ;
#59428=DIRECTION('',(0.,0.,-1.)) ;
#59429=DIRECTION('center_axis',(-1.,0.,-1.51760508056877E-16)) ;
#59430=DIRECTION('ref_axis',(-1.07310884363343E-16,0.707106781186485,0.70710678118661)) ;
#59431=DIRECTION('center_axis',(0.,0.,1.)) ;
#59432=DIRECTION('ref_axis',(-0.707106781186359,-0.707106781186736,0.)) ;
#59433=DIRECTION('',(0.,0.,1.)) ;
#59434=DIRECTION('center_axis',(0.,1.,5.60383084497428E-34)) ;
#59435=DIRECTION('ref_axis',(0.707106781186548,-3.96250679110365E-34,0.707106781186548)) ;
#59436=DIRECTION('',(0.,1.,5.60383084497428E-34)) ;
#59437=DIRECTION('center_axis',(0.,0.,1.)) ;
#59438=DIRECTION('ref_axis',(-0.70710678118661,0.707106781186485,0.)) ;
#59439=DIRECTION('',(0.,0.,-1.)) ;
#59440=DIRECTION('center_axis',(1.,0.,1.51760508056877E-16)) ;
#59441=DIRECTION('ref_axis',(-1.07310884363343E-16,-0.707106781186485,0.70710678118661)) ;
#59442=DIRECTION('center_axis',(1.,0.,1.51760508056877E-16)) ;
#59443=DIRECTION('ref_axis',(1.07310884363343E-16,0.707106781186485,-0.70710678118661)) ;
#59444=DIRECTION('center_axis',(1.,0.,0.)) ;
#59445=DIRECTION('ref_axis',(0.,1.,0.)) ;
#59446=DIRECTION('',(0.,1.,5.60383084497428E-34)) ;
#59447=DIRECTION('center_axis',(0.,1.,5.60383084497428E-34)) ;
#59448=DIRECTION('ref_axis',(-0.707106781186548,3.96250679110365E-34,-0.707106781186548)) ;
#59449=DIRECTION('center_axis',(0.,0.,1.)) ;
#59450=DIRECTION('ref_axis',(1.,0.,0.)) ;
#59451=DIRECTION('center_axis',(-1.,0.,0.)) ;
#59452=DIRECTION('ref_axis',(0.,-1.,0.)) ;
#59453=DIRECTION('center_axis',(0.,0.,-1.)) ;
#59454=DIRECTION('ref_axis',(1.,0.,0.)) ;
#59455=DIRECTION('center_axis',(0.,-1.,0.)) ;
#59456=DIRECTION('ref_axis',(0.,0.,1.)) ;
#59457=DIRECTION('center_axis',(0.,0.,1.)) ;
#59458=DIRECTION('ref_axis',(1.,0.,0.)) ;
#59459=DIRECTION('center_axis',(0.,-1.,0.)) ;
#59460=DIRECTION('ref_axis',(1.,0.,0.)) ;
#59461=DIRECTION('center_axis',(-4.44089209850092E-14,0.,-1.)) ;
#59462=DIRECTION('ref_axis',(0.,1.,0.)) ;
#59463=DIRECTION('center_axis',(1.,0.,0.)) ;
#59464=DIRECTION('ref_axis',(0.,0.,1.)) ;
#59465=DIRECTION('center_axis',(0.,0.,1.)) ;
#59466=DIRECTION('ref_axis',(-0.707106781186359,0.707106781186736,0.)) ;
#59467=DIRECTION('center_axis',(0.,0.,1.)) ;
#59468=DIRECTION('ref_axis',(0.,1.,0.)) ;
#59469=DIRECTION('center_axis',(0.,0.,-1.)) ;
#59470=DIRECTION('ref_axis',(-1.,0.,0.)) ;
#59471=DIRECTION('center_axis',(1.,2.22044604925031E-16,0.)) ;
#59472=DIRECTION('ref_axis',(0.,0.,-1.)) ;
#59473=DIRECTION('center_axis',(0.,1.,0.)) ;
#59474=DIRECTION('ref_axis',(-1.,0.,0.)) ;
#59475=DIRECTION('center_axis',(-1.,-2.22044604925031E-16,0.)) ;
#59476=DIRECTION('ref_axis',(-1.57009245868375E-16,0.707106781186538,0.707106781186557)) ;
#59477=DIRECTION('center_axis',(2.22044604925031E-16,-1.,3.31372189702139E-32)) ;
#59478=DIRECTION('ref_axis',(-0.707106781186548,-1.57009245868377E-16,0.707106781186548)) ;
#59479=DIRECTION('center_axis',(0.,1.,0.)) ;
#59480=DIRECTION('ref_axis',(-1.,0.,0.)) ;
#59481=DIRECTION('center_axis',(1.51760508056877E-16,5.60383084497428E-34,
-1.)) ;
#59482=DIRECTION('ref_axis',(-1.,0.,0.)) ;
#59483=DIRECTION('center_axis',(-1.,0.,0.)) ;
#59484=DIRECTION('ref_axis',(0.,-1.,0.)) ;
#59485=DIRECTION('center_axis',(-1.51760508056877E-16,-5.60383084497428E-34,
1.)) ;
#59486=DIRECTION('ref_axis',(-0.70710678118657,-0.707106781186525,-1.07310884363337E-16)) ;
#59487=DIRECTION('center_axis',(1.,0.,1.51760508056877E-16)) ;
#59488=DIRECTION('ref_axis',(-1.07310884363343E-16,-0.707106781186485,0.70710678118661)) ;
#59489=DIRECTION('center_axis',(-1.,0.,0.)) ;
#59490=DIRECTION('ref_axis',(0.,-1.,0.)) ;
#59491=DIRECTION('',(1.,0.,1.51760508056877E-16)) ;
#59492=DIRECTION('center_axis',(1.51760508056877E-16,5.60383084497428E-34,
-1.)) ;
#59493=DIRECTION('ref_axis',(-1.,0.,0.)) ;
#59494=DIRECTION('center_axis',(0.,-1.,0.)) ;
#59495=DIRECTION('ref_axis',(1.,0.,0.)) ;
#59496=DIRECTION('center_axis',(-1.51760508056877E-16,-5.60383084497428E-34,
1.)) ;
#59497=DIRECTION('ref_axis',(0.707106781186574,-0.707106781186522,1.07310884363337E-16)) ;
#59498=DIRECTION('center_axis',(-2.33146835171284E-14,1.,-3.53768783266021E-30)) ;
#59499=DIRECTION('ref_axis',(0.707106781186579,1.64859708161805E-14,0.707106781186516)) ;
#59500=DIRECTION('',(-2.33146835171284E-14,1.,-3.53768783266021E-30)) ;
#59501=DIRECTION('center_axis',(0.,-1.,0.)) ;
#59502=DIRECTION('ref_axis',(0.,0.,-1.)) ;
#59503=DIRECTION('center_axis',(0.,-1.,0.)) ;
#59504=DIRECTION('ref_axis',(0.,0.,-1.)) ;
#59505=DIRECTION('center_axis',(0.,0.,-1.)) ;
#59506=DIRECTION('ref_axis',(0.,1.,0.)) ;
#59507=DIRECTION('center_axis',(0.,0.,1.)) ;
#59508=DIRECTION('ref_axis',(0.70710678118661,0.707106781186485,0.)) ;
#59509=DIRECTION('center_axis',(0.,0.,-1.)) ;
#59510=DIRECTION('ref_axis',(0.,1.,0.)) ;
#59511=DIRECTION('center_axis',(-1.,0.,0.)) ;
#59512=DIRECTION('ref_axis',(0.,0.,1.)) ;
#59513=DIRECTION('center_axis',(0.,1.,0.)) ;
#59514=DIRECTION('ref_axis',(0.,0.,1.)) ;
#59515=DIRECTION('center_axis',(1.,0.,0.)) ;
#59516=DIRECTION('ref_axis',(0.,0.707106781186538,0.707106781186557)) ;
#59517=DIRECTION('center_axis',(0.,1.,5.60383084497428E-34)) ;
#59518=DIRECTION('ref_axis',(0.707106781186516,-3.96250679110383E-34,0.707106781186579)) ;
#59519=DIRECTION('center_axis',(0.,1.,0.)) ;
#59520=DIRECTION('ref_axis',(0.,0.,1.)) ;
#59521=DIRECTION('center_axis',(-1.51760508056877E-16,-5.60383084497428E-34,
1.)) ;
#59522=DIRECTION('ref_axis',(1.,0.,0.)) ;
#59523=DIRECTION('center_axis',(-0.707106781186548,0.707106781186548,0.)) ;
#59524=DIRECTION('ref_axis',(0.,0.,1.)) ;
#59525=DIRECTION('center_axis',(1.51760508056877E-16,5.60383084497428E-34,
-1.)) ;
#59526=DIRECTION('ref_axis',(-0.923879532511263,-0.382683432365147,-1.40208427237259E-16)) ;
#59527=DIRECTION('center_axis',(-0.707106781186615,0.70710678118648,-1.07310884363344E-16)) ;
#59528=DIRECTION('ref_axis',(0.499999999999866,0.499999999999961,0.70710678118667)) ;
#59529=DIRECTION('center_axis',(-0.707106781186548,0.707106781186548,0.)) ;
#59530=DIRECTION('ref_axis',(0.,0.,1.)) ;
#59531=DIRECTION('',(-0.707106781186615,0.70710678118648,-1.07310884363344E-16)) ;
#59532=DIRECTION('center_axis',(1.51760508056877E-16,5.60383084497428E-34,
-1.)) ;
#59533=DIRECTION('ref_axis',(-1.,0.,0.)) ;
#59534=DIRECTION('center_axis',(0.,1.,0.)) ;
#59535=DIRECTION('ref_axis',(0.,0.,1.)) ;
#59536=DIRECTION('center_axis',(-1.51760508056877E-16,-5.60383084497428E-34,
1.)) ;
#59537=DIRECTION('ref_axis',(0.923879532511263,0.382683432365147,1.40208427237259E-16)) ;
#59538=DIRECTION('center_axis',(-6.83214169000096E-16,1.,-1.03124546314615E-31)) ;
#59539=DIRECTION('ref_axis',(0.707106781186453,4.83105371902635E-16,0.707106781186642)) ;
#59540=DIRECTION('center_axis',(0.,1.,0.)) ;
#59541=DIRECTION('ref_axis',(0.,0.,1.)) ;
#59542=DIRECTION('',(-6.83214169000096E-16,1.,-1.03124546314615E-31)) ;
#59543=DIRECTION('center_axis',(1.51760508056877E-16,5.60383084497428E-34,
-1.)) ;
#59544=DIRECTION('ref_axis',(-1.,0.,0.)) ;
#59545=DIRECTION('center_axis',(0.999479573214818,0.0322580645161017,0.)) ;
#59546=DIRECTION('ref_axis',(0.,0.,1.)) ;
#59547=DIRECTION('center_axis',(-1.51760508056877E-16,-5.60383084497428E-34,
1.)) ;
#59548=DIRECTION('ref_axis',(0.718421208107084,-0.695608343640269,1.09027967541166E-16)) ;
#59549=DIRECTION('center_axis',(1.51760508056877E-16,5.60383084497428E-34,
-1.)) ;
#59550=DIRECTION('ref_axis',(-1.,0.,0.)) ;
#59551=DIRECTION('center_axis',(0.,1.,0.)) ;
#59552=DIRECTION('ref_axis',(0.,0.,1.)) ;
#59553=DIRECTION('center_axis',(1.51760508056877E-16,5.60383084497428E-34,
-1.)) ;
#59554=DIRECTION('ref_axis',(-0.718421208107087,0.695608343640265,-1.09027967541167E-16)) ;
#59555=DIRECTION('center_axis',(0.,1.,5.60383084497428E-34)) ;
#59556=DIRECTION('ref_axis',(0.707106781186548,-3.96250679110365E-34,0.707106781186548)) ;
#59557=DIRECTION('center_axis',(0.,1.,0.)) ;
#59558=DIRECTION('ref_axis',(0.,0.,1.)) ;
#59559=DIRECTION('',(0.,1.,5.60383084497428E-34)) ;
#59560=DIRECTION('center_axis',(1.51760508056877E-16,5.60383084497428E-34,
-1.)) ;
#59561=DIRECTION('ref_axis',(-1.,0.,0.)) ;
#59562=DIRECTION('center_axis',(-0.999479573214819,0.0322580645160902,0.)) ;
#59563=DIRECTION('ref_axis',(0.,0.,1.)) ;
#59564=DIRECTION('center_axis',(1.51760508056877E-16,5.60383084497428E-34,
-1.)) ;
#59565=DIRECTION('ref_axis',(-0.718421208107092,-0.69560834364026,-1.09027967541168E-16)) ;
#59566=DIRECTION('center_axis',(1.51760508056877E-16,5.60383084497428E-34,
-1.)) ;
#59567=DIRECTION('ref_axis',(-1.,0.,0.)) ;
#59568=DIRECTION('center_axis',(0.,1.,0.)) ;
#59569=DIRECTION('ref_axis',(0.,0.,1.)) ;
#59570=DIRECTION('center_axis',(-1.51760508056877E-16,-5.60383084497428E-34,
1.)) ;
#59571=DIRECTION('ref_axis',(0.718421208107098,0.695608343640254,1.09027967541169E-16)) ;
#59572=DIRECTION('center_axis',(-6.83214169000096E-16,1.,-1.03124546314615E-31)) ;
#59573=DIRECTION('ref_axis',(0.707106781186579,4.83105371902721E-16,0.707106781186516)) ;
#59574=DIRECTION('center_axis',(0.,1.,0.)) ;
#59575=DIRECTION('ref_axis',(0.,0.,1.)) ;
#59576=DIRECTION('',(-6.83214169000096E-16,1.,-1.03124546314615E-31)) ;
#59577=DIRECTION('center_axis',(1.51760508056877E-16,5.60383084497428E-34,
-1.)) ;
#59578=DIRECTION('ref_axis',(-1.,0.,0.)) ;
#59579=DIRECTION('center_axis',(0.707106781186548,0.707106781186548,0.)) ;
#59580=DIRECTION('ref_axis',(0.,0.,1.)) ;
#59581=DIRECTION('center_axis',(-1.51760508056877E-16,-5.60383084497428E-34,
1.)) ;
#59582=DIRECTION('ref_axis',(0.923879532511288,-0.382683432365087,1.40208427237263E-16)) ;
#59583=DIRECTION('center_axis',(0.707106781186521,0.707106781186574,1.0731088436333E-16)) ;
#59584=DIRECTION('ref_axis',(0.499999999999964,-0.499999999999927,0.707106781186625)) ;
#59585=DIRECTION('center_axis',(0.707106781186548,0.707106781186548,0.)) ;
#59586=DIRECTION('ref_axis',(0.,0.,1.)) ;
#59587=DIRECTION('',(0.707106781186521,0.707106781186574,1.0731088436333E-16)) ;
#59588=DIRECTION('center_axis',(-1.51760508056877E-16,-5.60383084497428E-34,
1.)) ;
#59589=DIRECTION('ref_axis',(1.,0.,0.)) ;
#59590=DIRECTION('center_axis',(0.,1.,0.)) ;
#59591=DIRECTION('ref_axis',(0.,0.,1.)) ;
#59592=DIRECTION('center_axis',(1.51760508056877E-16,5.60383084497428E-34,
-1.)) ;
#59593=DIRECTION('ref_axis',(-0.923879532511313,0.382683432365025,-1.40208427237267E-16)) ;
#59594=DIRECTION('center_axis',(-5.23472275150178E-15,1.,-7.93863801220309E-31)) ;
#59595=DIRECTION('ref_axis',(0.707106781186516,3.70150795521825E-15,0.707106781186579)) ;
#59596=DIRECTION('center_axis',(0.,1.,0.)) ;
#59597=DIRECTION('ref_axis',(0.,0.,1.)) ;
#59598=DIRECTION('',(-5.23472275150178E-15,1.,-7.93863801220309E-31)) ;
#59599=DIRECTION('center_axis',(-1.51760508056877E-16,-5.60383084497428E-34,
1.)) ;
#59600=DIRECTION('ref_axis',(1.,0.,0.)) ;
#59601=DIRECTION('center_axis',(0.984807753012208,-0.173648177666931,0.)) ;
#59602=DIRECTION('ref_axis',(0.,0.,1.)) ;
#59603=DIRECTION('center_axis',(-1.51760508056877E-16,-5.60383084497428E-34,
1.)) ;
#59604=DIRECTION('ref_axis',(0.642787609686539,-0.766044443118978,9.75497742186947E-17)) ;
#59605=DIRECTION('center_axis',(0.984807753012209,-0.173648177666924,1.49454924935485E-16)) ;
#59606=DIRECTION('ref_axis',(-0.122787803968973,-0.696364240320047,0.70710678118652)) ;
#59607=DIRECTION('center_axis',(0.984807753012208,-0.173648177666931,0.)) ;
#59608=DIRECTION('ref_axis',(0.,0.,1.)) ;
#59609=DIRECTION('',(0.984807753012209,-0.173648177666924,1.49454924935485E-16)) ;
#59610=DIRECTION('center_axis',(1.51760508056877E-16,5.60383084497428E-34,
-1.)) ;
#59611=DIRECTION('ref_axis',(-1.,0.,0.)) ;
#59612=DIRECTION('center_axis',(0.573576436350949,-0.81915204428906,0.)) ;
#59613=DIRECTION('ref_axis',(0.,0.,1.)) ;
#59614=DIRECTION('center_axis',(-1.51760508056877E-16,-5.60383084497428E-34,
1.)) ;
#59615=DIRECTION('ref_axis',(-0.53729960834682,-0.843391445812888,-8.15408615414744E-17)) ;
#59616=DIRECTION('center_axis',(0.573576436351042,-0.819152044288994,8.70462513900874E-17)) ;
#59617=DIRECTION('ref_axis',(-0.579227965339658,-0.405579787672697,0.707106781186442)) ;
#59618=DIRECTION('center_axis',(0.573576436351033,-0.819152044289001,0.)) ;
#59619=DIRECTION('ref_axis',(0.,0.,1.)) ;
#59620=DIRECTION('',(0.573576436351042,-0.819152044288994,8.70462513900874E-17)) ;
#59621=DIRECTION('center_axis',(1.51760508056877E-16,5.60383084497428E-34,
-1.)) ;
#59622=DIRECTION('ref_axis',(-1.,0.,0.)) ;
#59623=DIRECTION('center_axis',(0.,-1.,0.)) ;
#59624=DIRECTION('ref_axis',(0.,0.,1.)) ;
#59625=DIRECTION('center_axis',(-1.51760508056877E-16,-5.60383084497428E-34,
1.)) ;
#59626=DIRECTION('ref_axis',(-0.953716950748229,-0.300705799504266,-1.44736568988007E-16)) ;
#59627=DIRECTION('center_axis',(-5.25359141716359E-35,-1.,-5.60383084497428E-34)) ;
#59628=DIRECTION('ref_axis',(-0.707106781186548,-3.59102177943767E-34,0.707106781186548)) ;
#59629=DIRECTION('center_axis',(0.,-1.,0.)) ;
#59630=DIRECTION('ref_axis',(0.,0.,1.)) ;
#59631=DIRECTION('',(-5.25359141716359E-35,-1.,-5.60383084497428E-34)) ;
#59632=DIRECTION('center_axis',(-1.51760508056877E-16,-5.60383084497428E-34,
1.)) ;
#59633=DIRECTION('ref_axis',(1.,0.,0.)) ;
#59634=DIRECTION('center_axis',(1.,0.,0.)) ;
#59635=DIRECTION('ref_axis',(0.,0.,1.)) ;
#59636=DIRECTION('center_axis',(1.51760508056877E-16,5.60383084497428E-34,
-1.)) ;
#59637=DIRECTION('ref_axis',(0.707106781186547,0.707106781186547,1.07310884363333E-16)) ;
#59638=DIRECTION('center_axis',(1.,0.,1.51760508056877E-16)) ;
#59639=DIRECTION('ref_axis',(-1.07310884363343E-16,-0.707106781186485,0.70710678118661)) ;
#59640=DIRECTION('center_axis',(1.,0.,0.)) ;
#59641=DIRECTION('ref_axis',(0.,0.,1.)) ;
#59642=DIRECTION('',(1.,0.,1.51760508056877E-16)) ;
#59643=DIRECTION('center_axis',(1.51760508056877E-16,5.60383084497428E-34,
-1.)) ;
#59644=DIRECTION('ref_axis',(-1.,0.,0.)) ;
#59645=DIRECTION('center_axis',(0.,-1.,0.)) ;
#59646=DIRECTION('ref_axis',(0.,0.,1.)) ;
#59647=DIRECTION('center_axis',(-1.51760508056877E-16,-5.60383084497428E-34,
1.)) ;
#59648=DIRECTION('ref_axis',(-0.707106781186547,-0.707106781186547,-1.07310884363333E-16)) ;
#59649=DIRECTION('center_axis',(-2.22044604925032E-15,-1.,-3.37536403631613E-31)) ;
#59650=DIRECTION('ref_axis',(-0.707106781186548,1.57009245868378E-15,0.707106781186548)) ;
#59651=DIRECTION('',(-2.22044604925032E-15,-1.,-3.37536403631613E-31)) ;
#59652=DIRECTION('center_axis',(0.,-1.,0.)) ;
#59653=DIRECTION('ref_axis',(0.,0.,-1.)) ;
#59654=DIRECTION('center_axis',(0.,0.,1.)) ;
#59655=DIRECTION('ref_axis',(0.,1.,0.)) ;
#59656=DIRECTION('center_axis',(0.,1.,0.)) ;
#59657=DIRECTION('ref_axis',(0.707106781186548,0.,-0.707106781186548)) ;
#59658=DIRECTION('center_axis',(0.,-1.,0.)) ;
#59659=DIRECTION('ref_axis',(0.707106781186548,0.,-0.707106781186548)) ;
#59660=DIRECTION('center_axis',(-2.01858731750028E-16,0.,1.)) ;
#59661=DIRECTION('ref_axis',(-0.707106781186579,0.707106781186516,-1.42735678062167E-16)) ;
#59662=DIRECTION('',(2.01858731750028E-16,0.,-1.)) ;
#59663=DIRECTION('',(-2.01858731750028E-16,0.,1.)) ;
#59664=DIRECTION('center_axis',(1.,0.,1.51760508056877E-16)) ;
#59665=DIRECTION('ref_axis',(-1.07310884363343E-16,-0.707106781186485,0.70710678118661)) ;
#59666=DIRECTION('',(1.,0.,1.51760508056877E-16)) ;
#59667=DIRECTION('center_axis',(-2.01858731750028E-16,0.,1.)) ;
#59668=DIRECTION('ref_axis',(0.70710678118661,0.707106781186485,1.42735678062174E-16)) ;
#59669=DIRECTION('center_axis',(0.,0.,-1.)) ;
#59670=DIRECTION('ref_axis',(0.,1.,0.)) ;
#59671=DIRECTION('',(-2.01858731750028E-16,0.,1.)) ;
#59672=DIRECTION('',(2.01858731750028E-16,0.,-1.)) ;
#59673=DIRECTION('center_axis',(0.,-1.,0.)) ;
#59674=DIRECTION('ref_axis',(0.,0.,-1.)) ;
#59675=DIRECTION('center_axis',(0.,1.,0.)) ;
#59676=DIRECTION('ref_axis',(-0.707106781186548,0.,-0.707106781186548)) ;
#59677=DIRECTION('center_axis',(0.,-1.,0.)) ;
#59678=DIRECTION('ref_axis',(-0.707106781186548,0.,-0.707106781186548)) ;
#59679=DIRECTION('center_axis',(-1.,0.,-1.51760508056877E-16)) ;
#59680=DIRECTION('ref_axis',(-1.07310884363335E-16,0.70710678118654,0.707106781186555)) ;
#59681=DIRECTION('center_axis',(-0.863778900898434,-0.503871025524085,0.)) ;
#59682=DIRECTION('ref_axis',(-0.503871025524085,0.863778900898434,0.)) ;
#59683=DIRECTION('center_axis',(-0.863778900898434,-0.503871025524085,0.)) ;
#59684=DIRECTION('ref_axis',(-0.503871025524085,0.863778900898434,0.)) ;
#59685=DIRECTION('center_axis',(0.70710678118648,0.707106781186615,0.)) ;
#59686=DIRECTION('ref_axis',(-0.707106781186615,0.70710678118648,-1.05526329952557E-16)) ;
#59687=DIRECTION('',(0.,0.,1.)) ;
#59688=DIRECTION('',(0.707106781186615,-0.70710678118648,1.07310884363344E-16)) ;
#59689=DIRECTION('',(0.,0.,-1.)) ;
#59690=DIRECTION('center_axis',(0.,0.,1.)) ;
#59691=DIRECTION('ref_axis',(0.923879532511284,0.382683432365097,0.)) ;
#59692=DIRECTION('',(0.,0.,-1.)) ;
#59693=DIRECTION('center_axis',(1.51760508056877E-16,5.60383084497428E-34,
-1.)) ;
#59694=DIRECTION('ref_axis',(0.923879532511263,0.382683432365147,1.40208427237259E-16)) ;
#59695=DIRECTION('center_axis',(1.,6.83214169000096E-16,0.)) ;
#59696=DIRECTION('ref_axis',(-6.83214169000096E-16,1.,-1.01960673754504E-31)) ;
#59697=DIRECTION('',(0.,0.,1.)) ;
#59698=DIRECTION('',(6.83214169000096E-16,-1.,1.03124546314615E-31)) ;
#59699=DIRECTION('center_axis',(0.,0.,-1.)) ;
#59700=DIRECTION('ref_axis',(-1.,0.,0.)) ;
#59701=DIRECTION('',(0.,0.,-1.)) ;
#59702=DIRECTION('center_axis',(1.51760508056877E-16,5.60383084497428E-34,
-1.)) ;
#59703=DIRECTION('ref_axis',(0.718421208107084,-0.695608343640269,1.09027967541166E-16)) ;
#59704=DIRECTION('center_axis',(0.,0.,1.)) ;
#59705=DIRECTION('ref_axis',(0.,1.,0.)) ;
#59706=DIRECTION('',(0.,0.,1.)) ;
#59707=DIRECTION('center_axis',(-1.51760508056877E-16,-5.60383084497428E-34,
1.)) ;
#59708=DIRECTION('ref_axis',(-0.718421208107087,0.695608343640265,-1.09027967541167E-16)) ;
#59709=DIRECTION('center_axis',(1.,0.,0.)) ;
#59710=DIRECTION('ref_axis',(0.,1.,0.)) ;
#59711=DIRECTION('',(0.,0.,1.)) ;
#59712=DIRECTION('',(0.,-1.,-5.60383084497428E-34)) ;
#59713=DIRECTION('center_axis',(0.,0.,1.)) ;
#59714=DIRECTION('ref_axis',(-1.,0.,0.)) ;
#59715=DIRECTION('',(0.,0.,1.)) ;
#59716=DIRECTION('center_axis',(-1.51760508056877E-16,-5.60383084497428E-34,
1.)) ;
#59717=DIRECTION('ref_axis',(-0.718421208107092,-0.69560834364026,-1.09027967541168E-16)) ;
#59718=DIRECTION('center_axis',(0.,0.,1.)) ;
#59719=DIRECTION('ref_axis',(-1.,0.,0.)) ;
#59720=DIRECTION('',(0.,0.,-1.)) ;
#59721=DIRECTION('center_axis',(1.51760508056877E-16,5.60383084497428E-34,
-1.)) ;
#59722=DIRECTION('ref_axis',(0.718421208107098,0.695608343640254,1.09027967541169E-16)) ;
#59723=DIRECTION('center_axis',(1.,6.83214169000096E-16,0.)) ;
#59724=DIRECTION('ref_axis',(-6.83214169000096E-16,1.,-1.01960673754504E-31)) ;
#59725=DIRECTION('',(0.,0.,1.)) ;
#59726=DIRECTION('',(6.83214169000096E-16,-1.,1.03124546314615E-31)) ;
#59727=DIRECTION('center_axis',(0.,0.,1.)) ;
#59728=DIRECTION('ref_axis',(0.923879532511284,-0.382683432365097,0.)) ;
#59729=DIRECTION('',(0.,0.,-1.)) ;
#59730=DIRECTION('center_axis',(1.51760508056877E-16,5.60383084497428E-34,
-1.)) ;
#59731=DIRECTION('ref_axis',(0.923879532511288,-0.382683432365087,1.40208427237263E-16)) ;
#59732=DIRECTION('center_axis',(0.707106781186574,-0.707106781186521,0.)) ;
#59733=DIRECTION('ref_axis',(0.707106781186521,0.707106781186574,1.05526329952543E-16)) ;
#59734=DIRECTION('',(0.,0.,1.)) ;
#59735=DIRECTION('',(-0.707106781186521,-0.707106781186574,-1.0731088436333E-16)) ;
#59736=DIRECTION('center_axis',(0.,0.,1.)) ;
#59737=DIRECTION('ref_axis',(-0.923879532511311,0.382683432365031,0.)) ;
#59738=DIRECTION('',(0.,0.,-1.)) ;
#59739=DIRECTION('center_axis',(-1.51760508056877E-16,-5.60383084497428E-34,
1.)) ;
#59740=DIRECTION('ref_axis',(-0.923879532511292,0.382683432365076,-1.40208427237264E-16)) ;
#59741=DIRECTION('center_axis',(1.,5.23472275150178E-15,0.)) ;
#59742=DIRECTION('ref_axis',(-5.23472275150178E-15,1.,-7.81213099608712E-31)) ;
#59743=DIRECTION('',(0.,0.,1.)) ;
#59744=DIRECTION('',(5.23472275150178E-15,-1.,7.93863801220309E-31)) ;
#59745=DIRECTION('center_axis',(0.,0.,1.)) ;
#59746=DIRECTION('ref_axis',(-0.17364817766693,-0.984807753012208,0.)) ;
#59747=DIRECTION('',(0.,0.,1.)) ;
#59748=DIRECTION('center_axis',(1.51760508056877E-16,5.60383084497428E-34,
-1.)) ;
#59749=DIRECTION('ref_axis',(0.642787609686539,-0.766044443118978,9.75497742186947E-17)) ;
#59750=DIRECTION('center_axis',(-0.173648177666924,-0.984807753012209,0.)) ;
#59751=DIRECTION('ref_axis',(0.984807753012209,-0.173648177666924,1.4696952518233E-16)) ;
#59752=DIRECTION('',(0.,0.,1.)) ;
#59753=DIRECTION('',(-0.984807753012209,0.173648177666924,-1.49454924935485E-16)) ;
#59754=DIRECTION('center_axis',(0.,0.,1.)) ;
#59755=DIRECTION('ref_axis',(-0.537299608346821,-0.843391445812888,0.)) ;
#59756=DIRECTION('',(0.,0.,-1.)) ;
#59757=DIRECTION('center_axis',(1.51760508056877E-16,5.60383084497428E-34,
-1.)) ;
#59758=DIRECTION('ref_axis',(-0.537299608346822,-0.843391445812887,-8.15408615414747E-17)) ;
#59759=DIRECTION('center_axis',(-0.819152044288994,-0.573576436351042,0.)) ;
#59760=DIRECTION('ref_axis',(0.573576436351042,-0.819152044288994,8.61198118612814E-17)) ;
#59761=DIRECTION('',(0.,0.,1.)) ;
#59762=DIRECTION('',(-0.573576436351042,0.819152044288994,-8.70462513900874E-17)) ;
#59763=DIRECTION('center_axis',(0.,0.,1.)) ;
#59764=DIRECTION('ref_axis',(-0.953716950748228,-0.300705799504269,0.)) ;
#59765=DIRECTION('',(0.,0.,-1.)) ;
#59766=DIRECTION('center_axis',(1.51760508056877E-16,5.60383084497428E-34,
-1.)) ;
#59767=DIRECTION('ref_axis',(-0.953716950748229,-0.300705799504266,-1.44736568988007E-16)) ;
#59768=DIRECTION('center_axis',(-1.,5.25359141716359E-35,0.)) ;
#59769=DIRECTION('ref_axis',(-5.25359141716359E-35,-1.,3.52030637124432E-19)) ;
#59770=DIRECTION('',(0.,0.,1.)) ;
#59771=DIRECTION('',(5.25359141716359E-35,1.,5.60383084497428E-34)) ;
#59772=DIRECTION('center_axis',(0.,0.,1.)) ;
#59773=DIRECTION('ref_axis',(0.707106781186537,0.707106781186558,0.)) ;
#59774=DIRECTION('',(0.,0.,-1.)) ;
#59775=DIRECTION('center_axis',(-1.51760508056877E-16,-5.60383084497428E-34,
1.)) ;
#59776=DIRECTION('ref_axis',(0.707106781186547,0.707106781186547,1.07310884363333E-16)) ;
#59777=DIRECTION('center_axis',(0.,-1.,0.)) ;
#59778=DIRECTION('ref_axis',(1.,0.,2.24978329294248E-16)) ;
#59779=DIRECTION('',(-2.01858731750028E-16,0.,1.)) ;
#59780=DIRECTION('',(-1.,0.,-1.51760508056877E-16)) ;
#59781=DIRECTION('center_axis',(2.01858731750028E-16,0.,-1.)) ;
#59782=DIRECTION('ref_axis',(-0.707106781186537,-0.707106781186558,-1.42735678062159E-16)) ;
#59783=DIRECTION('',(2.01858731750028E-16,0.,-1.)) ;
#59784=DIRECTION('center_axis',(1.51760508056877E-16,5.60383084497428E-34,
-1.)) ;
#59785=DIRECTION('ref_axis',(-0.707106781186547,-0.707106781186547,-1.07310884363333E-16)) ;
#59786=DIRECTION('center_axis',(1.,-2.22044604925032E-15,2.01858731750028E-16)) ;
#59787=DIRECTION('ref_axis',(2.22044604925032E-15,1.,1.18383464030937E-18)) ;
#59788=DIRECTION('',(2.22044604925032E-15,1.,3.37536403631613E-31)) ;
#59789=DIRECTION('center_axis',(2.22044604925032E-15,1.,3.37536403631613E-31)) ;
#59790=DIRECTION('ref_axis',(-0.707106781186548,1.57009245868378E-15,-0.707106781186548)) ;
#59791=DIRECTION('center_axis',(0.,-1.,0.)) ;
#59792=DIRECTION('ref_axis',(-1.,0.,0.)) ;
#59793=DIRECTION('center_axis',(0.,0.,1.)) ;
#59794=DIRECTION('ref_axis',(-0.707106781186359,0.707106781186736,0.)) ;
#59795=DIRECTION('center_axis',(-1.4923676700635E-16,0.,1.)) ;
#59796=DIRECTION('ref_axis',(-0.707106781186359,0.707106781186736,-1.05526329952519E-16)) ;
#59797=DIRECTION('',(0.,0.,1.)) ;
#59798=DIRECTION('center_axis',(0.,0.,-1.)) ;
#59799=DIRECTION('ref_axis',(-1.,0.,0.)) ;
#59800=DIRECTION('',(0.,0.,-1.)) ;
#59801=DIRECTION('center_axis',(0.,-1.,0.)) ;
#59802=DIRECTION('ref_axis',(0.,0.,-1.)) ;
#59803=DIRECTION('center_axis',(-1.,-9.23705556487986E-12,0.)) ;
#59804=DIRECTION('ref_axis',(0.,0.,1.)) ;
#59805=DIRECTION('center_axis',(0.,-1.,0.)) ;
#59806=DIRECTION('ref_axis',(-0.707106781186881,0.,0.707106781186214)) ;
#59807=DIRECTION('center_axis',(0.,1.,0.)) ;
#59808=DIRECTION('ref_axis',(-0.707106781186881,0.,0.707106781186215)) ;
#59809=DIRECTION('center_axis',(1.,0.,1.51760508056877E-16)) ;
#59810=DIRECTION('ref_axis',(-1.07310884363305E-16,0.707106781186736,0.707106781186359)) ;
#59811=DIRECTION('center_axis',(0.70710678118661,0.707106781186485,0.)) ;
#59812=DIRECTION('ref_axis',(-0.707106781186485,0.70710678118661,-2.45326946669362E-16)) ;
#59813=DIRECTION('center_axis',(3.17206578464329E-15,-1.,4.80833931982806E-31)) ;
#59814=DIRECTION('ref_axis',(-0.707106781186551,-2.24298922669111E-15,0.707106781186544)) ;
#59815=DIRECTION('',(3.17206578464329E-15,-1.,4.80833931982806E-31)) ;
#59816=DIRECTION('center_axis',(-3.55271367880051E-14,-1.,0.)) ;
#59817=DIRECTION('ref_axis',(-0.707106781186879,2.51214793389522E-14,0.707106781186216)) ;
#59818=DIRECTION('center_axis',(-1.,-3.17206578464329E-15,0.)) ;
#59819=DIRECTION('ref_axis',(3.17206578464329E-15,-1.,4.73388842431626E-31)) ;
#59820=DIRECTION('',(-3.17206578464329E-15,1.,-4.73388842431626E-31)) ;
#59821=DIRECTION('',(0.,0.,-1.)) ;
#59822=DIRECTION('center_axis',(-1.4923676700635E-16,0.,1.)) ;
#59823=DIRECTION('ref_axis',(1.,0.,1.4923676700635E-16)) ;
#59824=DIRECTION('',(1.,0.,1.4923676700635E-16)) ;
#59825=DIRECTION('',(-7.105427357601E-15,-1.,-1.06039100704685E-30)) ;
#59826=DIRECTION('',(-1.,3.55271367880051E-14,-1.4923676700635E-16)) ;
#59827=DIRECTION('center_axis',(-1.4923676700635E-16,0.,1.)) ;
#59828=DIRECTION('ref_axis',(-0.70710678118661,-0.707106781186485,-1.05526329952556E-16)) ;
#59829=DIRECTION('center_axis',(0.,0.,1.)) ;
#59830=DIRECTION('ref_axis',(-0.70710678118661,-0.707106781186485,0.)) ;
#59831=DIRECTION('',(0.,0.,1.)) ;
#59832=DIRECTION('center_axis',(0.,0.,-1.)) ;
#59833=DIRECTION('ref_axis',(0.,-1.,0.)) ;
#59834=DIRECTION('center_axis',(3.55271367880051E-14,1.,0.)) ;
#59835=DIRECTION('ref_axis',(0.,0.,1.)) ;
#59836=DIRECTION('center_axis',(-1.,4.25984888819251E-25,9.5923269327607E-12)) ;
#59837=DIRECTION('ref_axis',(-3.39809272400367E-40,-1.,4.44089209849993E-14)) ;
#59838=DIRECTION('center_axis',(3.55271367880051E-14,1.,0.)) ;
#59839=DIRECTION('ref_axis',(-0.707106781186879,2.51214793389522E-14,0.707106781186216)) ;
#59840=DIRECTION('center_axis',(-1.,3.55271367880051E-14,-1.51760508056877E-16)) ;
#59841=DIRECTION('ref_axis',(-2.52287902233105E-14,-0.707106781186736,0.707106781186359)) ;
#59842=DIRECTION('center_axis',(0.70710678118661,-0.707106781186485,0.)) ;
#59843=DIRECTION('ref_axis',(-0.707106781186485,-0.70710678118661,0.)) ;
#59844=DIRECTION('center_axis',(-3.55271367880051E-14,-1.,0.)) ;
#59845=DIRECTION('ref_axis',(1.,-3.55271367880051E-14,1.4923676700635E-16)) ;
#59846=DIRECTION('',(0.,0.,1.)) ;
#59847=DIRECTION('',(0.,0.,-1.)) ;
#59848=DIRECTION('center_axis',(0.,0.,1.)) ;
#59849=DIRECTION('ref_axis',(1.,0.,0.)) ;
#59850=DIRECTION('center_axis',(-1.,0.,0.)) ;
#59851=DIRECTION('ref_axis',(0.,-1.,0.)) ;
#59852=DIRECTION('center_axis',(0.,4.44089209849835E-14,-1.)) ;
#59853=DIRECTION('ref_axis',(1.,0.,0.)) ;
#59854=DIRECTION('center_axis',(0.,-1.,0.)) ;
#59855=DIRECTION('ref_axis',(0.,0.,1.)) ;
#59856=DIRECTION('center_axis',(0.,0.,-1.)) ;
#59857=DIRECTION('ref_axis',(-1.,0.,0.)) ;
#59858=DIRECTION('center_axis',(0.,0.,-1.)) ;
#59859=DIRECTION('ref_axis',(0.,1.,0.)) ;
#59860=DIRECTION('center_axis',(1.,0.,0.)) ;
#59861=DIRECTION('ref_axis',(0.,0.,1.)) ;
#59862=DIRECTION('center_axis',(-0.707106781186592,-0.707106781186503,0.)) ;
#59863=DIRECTION('ref_axis',(0.707106781186503,-0.707106781186592,0.)) ;
#59864=DIRECTION('center_axis',(1.,0.,1.51760508056877E-16)) ;
#59865=DIRECTION('ref_axis',(-1.07310884363343E-16,-0.707106781186485,0.70710678118661)) ;
#59866=DIRECTION('',(1.,0.,1.51760508056877E-16)) ;
#59867=DIRECTION('center_axis',(0.,0.,-1.)) ;
#59868=DIRECTION('ref_axis',(-1.,0.,0.)) ;
#59869=DIRECTION('center_axis',(4.44089209850072E-14,4.44089209850072E-14,
-1.)) ;
#59870=DIRECTION('ref_axis',(-0.707106781186547,0.707106781186547,-2.2709071609452E-30)) ;
#59871=DIRECTION('center_axis',(0.707106781186548,0.707106781186548,0.)) ;
#59872=DIRECTION('ref_axis',(0.,0.,1.)) ;
#59873=DIRECTION('center_axis',(0.,-1.,0.)) ;
#59874=DIRECTION('ref_axis',(1.,0.,0.)) ;
#59875=DIRECTION('center_axis',(-0.707106781186563,-0.707106781186532,-1.07310884363336E-16)) ;
#59876=DIRECTION('ref_axis',(0.499999999999956,-0.499999999999978,0.707106781186594)) ;
#59877=DIRECTION('',(0.707106781186563,0.707106781186532,1.07310884363336E-16)) ;
#59878=DIRECTION('center_axis',(0.,0.,-1.)) ;
#59879=DIRECTION('ref_axis',(-1.,0.,0.)) ;
#59880=DIRECTION('center_axis',(0.,-6.28036983473606E-14,-1.)) ;
#59881=DIRECTION('ref_axis',(-1.,0.,0.)) ;
#59882=DIRECTION('center_axis',(0.,1.,0.)) ;
#59883=DIRECTION('ref_axis',(0.,0.,1.)) ;
#59884=DIRECTION('center_axis',(0.707106781186548,-0.707106781186548,0.)) ;
#59885=DIRECTION('ref_axis',(0.707106781186547,0.707106781186547,0.)) ;
#59886=DIRECTION('center_axis',(3.73034936274055E-14,1.,5.66175752827605E-30)) ;
#59887=DIRECTION('ref_axis',(0.707106781186516,-2.63775533058864E-14,0.707106781186579)) ;
#59888=DIRECTION('',(3.73034936274055E-14,1.,5.66175752827605E-30)) ;
#59889=DIRECTION('center_axis',(0.,0.,-1.)) ;
#59890=DIRECTION('ref_axis',(-1.,0.,0.)) ;
#59891=DIRECTION('center_axis',(-4.44089209849937E-14,4.44089209849993E-14,
-1.)) ;
#59892=DIRECTION('ref_axis',(-0.707106781186592,-0.707106781186503,-5.90838107042161E-30)) ;
#59893=DIRECTION('center_axis',(-0.707106781186592,0.707106781186503,0.)) ;
#59894=DIRECTION('ref_axis',(0.,0.,1.)) ;
#59895=DIRECTION('center_axis',(1.,0.,0.)) ;
#59896=DIRECTION('ref_axis',(0.,1.,0.)) ;
#59897=DIRECTION('center_axis',(0.707106781186544,-0.707106781186551,1.07310884363333E-16)) ;
#59898=DIRECTION('ref_axis',(0.499999999999969,0.499999999999965,0.707106781186594)) ;
#59899=DIRECTION('',(-0.707106781186544,0.707106781186551,-1.07310884363333E-16)) ;
#59900=DIRECTION('center_axis',(0.,0.,1.)) ;
#59901=DIRECTION('ref_axis',(1.,0.,0.)) ;
#59902=DIRECTION('center_axis',(0.,1.,0.)) ;
#59903=DIRECTION('ref_axis',(-1.,0.,0.)) ;
#59904=DIRECTION('center_axis',(-4.44089209850072E-14,0.,-1.)) ;
#59905=DIRECTION('ref_axis',(0.,-1.,0.)) ;
#59906=DIRECTION('center_axis',(-1.,0.,0.)) ;
#59907=DIRECTION('ref_axis',(0.,0.,1.)) ;
#59908=DIRECTION('center_axis',(-7.105427357601E-15,-1.,-1.07888364883526E-30)) ;
#59909=DIRECTION('ref_axis',(-0.707106781186579,5.0242958677883E-15,0.707106781186516)) ;
#59910=DIRECTION('',(-7.105427357601E-15,-1.,-1.07888364883526E-30)) ;
#59911=DIRECTION('center_axis',(0.,0.,1.)) ;
#59912=DIRECTION('ref_axis',(0.707106781186548,-0.707106781186548,0.)) ;
#59913=DIRECTION('',(0.,0.,1.)) ;
#59914=DIRECTION('',(0.,0.,-1.)) ;
#59915=DIRECTION('center_axis',(-1.,7.10542735760144E-15,-1.51760508056877E-16)) ;
#59916=DIRECTION('ref_axis',(4.91698498342642E-15,0.707106781186736,0.707106781186359)) ;
#59917=DIRECTION('',(-1.,7.10542735760144E-15,-1.51760508056877E-16)) ;
#59918=DIRECTION('center_axis',(0.,0.,-1.)) ;
#59919=DIRECTION('ref_axis',(-0.382683432365045,-0.923879532511305,0.)) ;
#59920=DIRECTION('',(0.,0.,1.)) ;
#59921=DIRECTION('',(0.,0.,-1.)) ;
#59922=DIRECTION('center_axis',(0.,0.,1.)) ;
#59923=DIRECTION('ref_axis',(-0.923879532511297,-0.382683432365065,0.)) ;
#59924=DIRECTION('',(0.,0.,1.)) ;
#59925=DIRECTION('',(0.,0.,-1.)) ;
#59926=DIRECTION('center_axis',(0.,0.,-1.)) ;
#59927=DIRECTION('ref_axis',(-0.923879532511297,0.382683432365065,0.)) ;
#59928=DIRECTION('',(0.,0.,1.)) ;
#59929=DIRECTION('',(0.,0.,-1.)) ;
#59930=DIRECTION('center_axis',(0.,0.,1.)) ;
#59931=DIRECTION('ref_axis',(-0.382683432365099,0.923879532511283,0.)) ;
#59932=DIRECTION('',(0.,0.,1.)) ;
#59933=DIRECTION('',(0.,0.,-1.)) ;
#59934=DIRECTION('center_axis',(0.,0.,1.)) ;
#59935=DIRECTION('ref_axis',(0.707106781186296,0.707106781186799,0.)) ;
#59936=DIRECTION('',(0.,0.,1.)) ;
#59937=DIRECTION('',(0.,0.,-1.)) ;
#59938=DIRECTION('center_axis',(-7.105427357601E-15,-1.,-1.07888364883526E-30)) ;
#59939=DIRECTION('ref_axis',(-0.707106781186579,5.0242958677883E-15,0.707106781186516)) ;
#59940=DIRECTION('',(-7.105427357601E-15,-1.,-1.07888364883526E-30)) ;
#59941=DIRECTION('center_axis',(-7.10542735760144E-15,-1.,0.)) ;
#59942=DIRECTION('ref_axis',(1.,-7.10542735760144E-15,1.4923676700635E-16)) ;
#59943=DIRECTION('center_axis',(1.,-7.105427357601E-15,0.)) ;
#59944=DIRECTION('ref_axis',(7.105427357601E-15,1.,1.06039100704685E-30)) ;
#59945=DIRECTION('center_axis',(-0.81649658092775,0.408248290463875,-0.408248290463804)) ;
#59946=DIRECTION('ref_axis',(-0.577350269189602,-0.577350269189744,0.577350269189531)) ;
#59947=DIRECTION('center_axis',(-1.,-8.88178419699986E-14,0.)) ;
#59948=DIRECTION('ref_axis',(0.,0.,1.)) ;
#59949=DIRECTION('center_axis',(0.,-1.,0.)) ;
#59950=DIRECTION('ref_axis',(-1.,0.,0.)) ;
#59951=DIRECTION('center_axis',(-4.44089209850033E-14,0.,1.)) ;
#59952=DIRECTION('ref_axis',(0.,-1.,0.)) ;
#59953=DIRECTION('center_axis',(0.,0.,1.)) ;
#59954=DIRECTION('ref_axis',(1.,0.,0.)) ;
#59955=DIRECTION('center_axis',(-1.,0.,0.)) ;
#59956=DIRECTION('ref_axis',(0.,-1.,0.)) ;
#59957=DIRECTION('center_axis',(0.,0.,-1.)) ;
#59958=DIRECTION('ref_axis',(1.,0.,0.)) ;
#59959=DIRECTION('center_axis',(0.,-1.,0.)) ;
#59960=DIRECTION('ref_axis',(0.,0.,1.)) ;
#59961=DIRECTION('center_axis',(1.,0.,1.51760508056877E-16)) ;
#59962=DIRECTION('ref_axis',(-1.07310884363343E-16,-0.707106781186485,0.70710678118661)) ;
#59963=DIRECTION('',(1.,0.,1.51760508056877E-16)) ;
#59964=DIRECTION('center_axis',(0.,0.,1.)) ;
#59965=DIRECTION('ref_axis',(0.707106781186359,0.707106781186736,0.)) ;
#59966=DIRECTION('',(0.,0.,1.)) ;
#59967=DIRECTION('',(0.,0.,-1.)) ;
#59968=DIRECTION('center_axis',(0.,0.,1.)) ;
#59969=DIRECTION('ref_axis',(1.,0.,0.)) ;
#59970=DIRECTION('center_axis',(-1.,0.,0.)) ;
#59971=DIRECTION('ref_axis',(0.,-1.,0.)) ;
#59972=DIRECTION('center_axis',(0.,0.,-1.)) ;
#59973=DIRECTION('ref_axis',(1.,0.,0.)) ;
#59974=DIRECTION('center_axis',(0.,-1.,0.)) ;
#59975=DIRECTION('ref_axis',(0.,0.,1.)) ;
#59976=DIRECTION('center_axis',(0.,0.,1.)) ;
#59977=DIRECTION('ref_axis',(1.,0.,0.)) ;
#59978=DIRECTION('center_axis',(0.,1.,0.)) ;
#59979=DIRECTION('ref_axis',(-1.,0.,0.)) ;
#59980=DIRECTION('center_axis',(-1.,0.,0.)) ;
#59981=DIRECTION('ref_axis',(0.,0.,1.)) ;
#59982=DIRECTION('center_axis',(0.,-1.,-5.60383084497428E-34)) ;
#59983=DIRECTION('ref_axis',(-0.707106781186516,-3.96250679110383E-34,0.707106781186579)) ;
#59984=DIRECTION('',(0.,-1.,-5.60383084497428E-34)) ;
#59985=DIRECTION('center_axis',(0.,0.,-1.)) ;
#59986=DIRECTION('ref_axis',(-1.,0.,0.)) ;
#59987=DIRECTION('center_axis',(4.44089209850072E-14,0.,-1.)) ;
#59988=DIRECTION('ref_axis',(0.,1.,0.)) ;
#59989=DIRECTION('center_axis',(1.,0.,0.)) ;
#59990=DIRECTION('ref_axis',(0.,0.,1.)) ;
#59991=DIRECTION('center_axis',(0.,-1.,0.)) ;
#59992=DIRECTION('ref_axis',(1.,0.,0.)) ;
#59993=DIRECTION('center_axis',(1.,0.,1.51760508056877E-16)) ;
#59994=DIRECTION('ref_axis',(-1.07310884363343E-16,-0.707106781186485,0.70710678118661)) ;
#59995=DIRECTION('',(1.,0.,1.51760508056877E-16)) ;
#59996=DIRECTION('center_axis',(0.,0.,1.)) ;
#59997=DIRECTION('ref_axis',(1.,0.,0.)) ;
#59998=DIRECTION('center_axis',(1.,0.,0.)) ;
#59999=DIRECTION('ref_axis',(0.,1.,0.)) ;
#60000=DIRECTION('center_axis',(0.,1.,0.)) ;
#60001=DIRECTION('ref_axis',(0.,0.,1.)) ;
#60002=DIRECTION('center_axis',(-1.,0.,-1.51760508056877E-16)) ;
#60003=DIRECTION('ref_axis',(-1.07310884363343E-16,0.707106781186485,0.70710678118661)) ;
#60004=DIRECTION('center_axis',(-0.816496580927844,-0.40824829046378,0.408248290463709)) ;
#60005=DIRECTION('ref_axis',(0.577350269189507,-0.577350269189934,0.577350269189436)) ;
#60006=DIRECTION('center_axis',(-3.55271367880058E-13,-1.,0.)) ;
#60007=DIRECTION('ref_axis',(0.,0.,1.)) ;
#60008=DIRECTION('center_axis',(1.,0.,0.)) ;
#60009=DIRECTION('ref_axis',(0.,-1.,0.)) ;
#60010=DIRECTION('center_axis',(0.,0.,1.)) ;
#60011=DIRECTION('ref_axis',(1.,0.,0.)) ;
#60012=DIRECTION('center_axis',(0.,-1.,0.)) ;
#60013=DIRECTION('ref_axis',(1.,0.,0.)) ;
#60014=DIRECTION('center_axis',(1.,0.,0.)) ;
#60015=DIRECTION('ref_axis',(0.,0.,1.)) ;
#60016=DIRECTION('center_axis',(0.,1.,5.60383084497428E-34)) ;
#60017=DIRECTION('ref_axis',(0.707106781186516,-3.96250679110383E-34,0.707106781186579)) ;
#60018=DIRECTION('center_axis',(1.,0.,1.51760508056877E-16)) ;
#60019=DIRECTION('ref_axis',(-1.07310884363343E-16,-0.707106781186485,0.70710678118661)) ;
#60020=DIRECTION('center_axis',(0.,1.,5.60383084497428E-34)) ;
#60021=DIRECTION('ref_axis',(0.707106781186516,-3.96250679110383E-34,0.707106781186579)) ;
#60022=DIRECTION('center_axis',(0.,0.,1.)) ;
#60023=DIRECTION('ref_axis',(-0.70710678118661,0.707106781186485,0.)) ;
#60024=DIRECTION('',(0.,0.,1.)) ;
#60025=DIRECTION('center_axis',(0.,0.,1.)) ;
#60026=DIRECTION('ref_axis',(0.70710678118661,0.707106781186485,0.)) ;
#60027=DIRECTION('',(0.,0.,1.)) ;
#60028=DIRECTION('',(0.,0.,-1.)) ;
#60029=DIRECTION('center_axis',(0.,-1.,-5.60383084497428E-34)) ;
#60030=DIRECTION('ref_axis',(-0.707106781186516,-3.96250679110383E-34,0.707106781186579)) ;
#60031=DIRECTION('',(0.,-1.,-5.60383084497428E-34)) ;
#60032=DIRECTION('center_axis',(0.,0.,1.)) ;
#60033=DIRECTION('ref_axis',(-0.707106781186673,-0.707106781186422,0.)) ;
#60034=DIRECTION('',(0.,0.,1.)) ;
#60035=DIRECTION('',(0.,0.,-1.)) ;
#60036=DIRECTION('center_axis',(1.,0.,0.)) ;
#60037=DIRECTION('ref_axis',(0.,1.,0.)) ;
#60038=DIRECTION('center_axis',(0.,1.,0.)) ;
#60039=DIRECTION('ref_axis',(-1.,0.,-1.4923676700635E-16)) ;
#60040=DIRECTION('center_axis',(0.,0.,1.)) ;
#60041=DIRECTION('ref_axis',(0.70710678118661,0.707106781186485,0.)) ;
#60042=DIRECTION('center_axis',(-1.4923676700635E-16,0.,1.)) ;
#60043=DIRECTION('ref_axis',(0.70710678118661,0.707106781186485,1.05526329952556E-16)) ;
#60044=DIRECTION('',(0.,0.,1.)) ;
#60045=DIRECTION('center_axis',(0.,0.,-1.)) ;
#60046=DIRECTION('ref_axis',(0.,1.,0.)) ;
#60047=DIRECTION('',(0.,0.,-1.)) ;
#60048=DIRECTION('center_axis',(1.77635683940026E-14,-1.,0.)) ;
#60049=DIRECTION('ref_axis',(0.,0.,-1.)) ;
#60050=DIRECTION('center_axis',(1.,3.94430452610435E-27,-8.88178419700105E-14)) ;
#60051=DIRECTION('ref_axis',(9.19251792611137E-43,1.,4.44089209849993E-14)) ;
#60052=DIRECTION('center_axis',(-1.77635683940026E-14,1.,0.)) ;
#60053=DIRECTION('ref_axis',(0.707106781186549,1.25607396694703E-14,0.707106781186547)) ;
#60054=DIRECTION('center_axis',(1.77635683940026E-14,-1.,0.)) ;
#60055=DIRECTION('ref_axis',(0.707106781186548,1.25607396694703E-14,0.707106781186547)) ;
#60056=DIRECTION('center_axis',(1.,1.77635683940026E-14,1.51760508056877E-16)) ;
#60057=DIRECTION('ref_axis',(-1.26680505538369E-14,0.707106781186736,0.707106781186359)) ;
#60058=DIRECTION('center_axis',(-1.77635683940026E-14,1.,0.)) ;
#60059=DIRECTION('ref_axis',(-1.,-1.77635683940026E-14,-1.4923676700635E-16)) ;
#60060=DIRECTION('',(1.,1.77635683940026E-14,1.4923676700635E-16)) ;
#60061=DIRECTION('',(0.,0.,1.)) ;
#60062=DIRECTION('center_axis',(0.,0.,1.)) ;
#60063=DIRECTION('ref_axis',(0.707106781186359,-0.707106781186736,0.)) ;
#60064=DIRECTION('center_axis',(-1.4923676700635E-16,0.,1.)) ;
#60065=DIRECTION('ref_axis',(0.707106781186359,-0.707106781186736,1.05526329952519E-16)) ;
#60066=DIRECTION('',(0.,0.,1.)) ;
#60067=DIRECTION('center_axis',(0.,0.,-1.)) ;
#60068=DIRECTION('ref_axis',(1.,0.,0.)) ;
#60069=DIRECTION('',(0.,0.,-1.)) ;
#60070=DIRECTION('center_axis',(0.,1.,0.)) ;
#60071=DIRECTION('ref_axis',(0.,0.,1.)) ;
#60072=DIRECTION('center_axis',(1.,0.,0.)) ;
#60073=DIRECTION('ref_axis',(0.,0.,1.)) ;
#60074=DIRECTION('center_axis',(0.,1.,0.)) ;
#60075=DIRECTION('ref_axis',(0.707106781186547,0.,0.707106781186547)) ;
#60076=DIRECTION('center_axis',(0.,-1.,0.)) ;
#60077=DIRECTION('ref_axis',(0.707106781186548,0.,0.707106781186548)) ;
#60078=DIRECTION('center_axis',(-1.,0.,-1.51760508056877E-16)) ;
#60079=DIRECTION('ref_axis',(-1.07310884363343E-16,-0.707106781186485,0.70710678118661)) ;
#60080=DIRECTION('center_axis',(3.17206578464331E-15,1.,4.81954698151804E-31)) ;
#60081=DIRECTION('ref_axis',(0.707106781186548,-2.24298922669111E-15,0.707106781186548)) ;
#60082=DIRECTION('',(3.17206578464331E-15,1.,4.81954698151804E-31)) ;
#60083=DIRECTION('center_axis',(1.,-3.17206578464331E-15,0.)) ;
#60084=DIRECTION('ref_axis',(3.17206578464331E-15,1.,4.73388842431629E-31)) ;
#60085=DIRECTION('',(-3.17206578464331E-15,-1.,-4.73388842431629E-31)) ;
#60086=DIRECTION('center_axis',(0.,0.,-1.)) ;
#60087=DIRECTION('ref_axis',(-1.,0.,0.)) ;
#60088=DIRECTION('center_axis',(-1.,0.,0.)) ;
#60089=DIRECTION('ref_axis',(0.,0.,1.)) ;
#60090=DIRECTION('center_axis',(0.707106781186592,0.707106781186503,0.)) ;
#60091=DIRECTION('ref_axis',(-0.707106781186503,0.707106781186592,0.)) ;
#60092=DIRECTION('center_axis',(-1.,0.,-1.51760508056877E-16)) ;
#60093=DIRECTION('ref_axis',(-1.07310884363343E-16,0.707106781186485,0.70710678118661)) ;
#60094=DIRECTION('center_axis',(0.,0.,-1.)) ;
#60095=DIRECTION('ref_axis',(-1.,0.,0.)) ;
#60096=DIRECTION('center_axis',(-0.707106781186548,-0.707106781186548,0.)) ;
#60097=DIRECTION('ref_axis',(0.,0.,1.)) ;
#60098=DIRECTION('center_axis',(0.,1.,0.)) ;
#60099=DIRECTION('ref_axis',(-1.,0.,0.)) ;
#60100=DIRECTION('center_axis',(0.707106781186555,0.70710678118654,1.07310884363335E-16)) ;
#60101=DIRECTION('ref_axis',(-0.499999999999931,0.499999999999941,0.707106781186638)) ;
#60102=DIRECTION('center_axis',(0.,0.,-1.)) ;
#60103=DIRECTION('ref_axis',(-1.,0.,0.)) ;
#60104=DIRECTION('center_axis',(0.,-1.,0.)) ;
#60105=DIRECTION('ref_axis',(0.,0.,1.)) ;
#60106=DIRECTION('center_axis',(-0.707106781186503,0.707106781186592,0.)) ;
#60107=DIRECTION('ref_axis',(-0.707106781186592,-0.707106781186503,0.)) ;
#60108=DIRECTION('center_axis',(0.,-1.,-5.60383084497428E-34)) ;
#60109=DIRECTION('ref_axis',(-0.707106781186548,-3.96250679110365E-34,0.707106781186548)) ;
#60110=DIRECTION('center_axis',(0.,0.,-1.)) ;
#60111=DIRECTION('ref_axis',(-1.,0.,0.)) ;
#60112=DIRECTION('center_axis',(0.707106781186548,-0.707106781186548,0.)) ;
#60113=DIRECTION('ref_axis',(0.,0.,1.)) ;
#60114=DIRECTION('center_axis',(-1.,0.,0.)) ;
#60115=DIRECTION('ref_axis',(0.,-1.,0.)) ;
#60116=DIRECTION('center_axis',(-0.707106781186555,0.70710678118654,-1.07310884363335E-16)) ;
#60117=DIRECTION('ref_axis',(-0.499999999999962,-0.499999999999972,0.707106781186594)) ;
#60118=DIRECTION('center_axis',(1.,0.,1.51760508056877E-16)) ;
#60119=DIRECTION('ref_axis',(-1.07310884363343E-16,-0.707106781186485,0.70710678118661)) ;
#60120=DIRECTION('center_axis',(0.,0.,1.)) ;
#60121=DIRECTION('ref_axis',(-0.707106781186359,0.707106781186736,0.)) ;
#60122=DIRECTION('center_axis',(-1.4923676700635E-16,0.,1.)) ;
#60123=DIRECTION('ref_axis',(-0.707106781186359,0.707106781186736,-1.05526329952519E-16)) ;
#60124=DIRECTION('',(0.,0.,1.)) ;
#60125=DIRECTION('center_axis',(0.,0.,-1.)) ;
#60126=DIRECTION('ref_axis',(-1.,0.,0.)) ;
#60127=DIRECTION('',(0.,0.,-1.)) ;
#60128=DIRECTION('center_axis',(0.,-1.,0.)) ;
#60129=DIRECTION('ref_axis',(0.,0.,-1.)) ;
#60130=DIRECTION('center_axis',(-1.,-9.23705556487986E-12,0.)) ;
#60131=DIRECTION('ref_axis',(0.,0.,1.)) ;
#60132=DIRECTION('center_axis',(0.,-1.,0.)) ;
#60133=DIRECTION('ref_axis',(-0.707106781186543,0.,0.707106781186552)) ;
#60134=DIRECTION('center_axis',(0.,1.,0.)) ;
#60135=DIRECTION('ref_axis',(-0.707106781186543,0.,0.707106781186552)) ;
#60136=DIRECTION('center_axis',(1.,0.,1.51760508056877E-16)) ;
#60137=DIRECTION('ref_axis',(-1.07310884363343E-16,0.707106781186485,0.70710678118661)) ;
#60138=DIRECTION('center_axis',(0.70710678118661,0.707106781186485,0.)) ;
#60139=DIRECTION('ref_axis',(-0.707106781186485,0.70710678118661,-2.45326946669362E-16)) ;
#60140=DIRECTION('center_axis',(3.17206578464327E-15,-1.,4.80833931982803E-31)) ;
#60141=DIRECTION('ref_axis',(-0.707106781186551,-2.24298922669109E-15,0.707106781186544)) ;
#60142=DIRECTION('',(3.17206578464327E-15,-1.,4.80833931982803E-31)) ;
#60143=DIRECTION('center_axis',(-3.55271367880051E-14,-1.,0.)) ;
#60144=DIRECTION('ref_axis',(-0.707106781186548,2.51214793389405E-14,0.707106781186547)) ;
#60145=DIRECTION('center_axis',(-1.,-3.17206578464327E-15,0.)) ;
#60146=DIRECTION('ref_axis',(3.17206578464327E-15,-1.,4.73388842431623E-31)) ;
#60147=DIRECTION('',(-3.17206578464327E-15,1.,-4.73388842431623E-31)) ;
#60148=DIRECTION('',(0.,0.,-1.)) ;
#60149=DIRECTION('center_axis',(-1.4923676700635E-16,0.,1.)) ;
#60150=DIRECTION('ref_axis',(1.,0.,1.4923676700635E-16)) ;
#60151=DIRECTION('',(1.,0.,1.4923676700635E-16)) ;
#60152=DIRECTION('',(-3.17206578464323E-15,-1.,-4.73388842431617E-31)) ;
#60153=DIRECTION('',(-1.,3.55271367880051E-14,-1.4923676700635E-16)) ;
#60154=DIRECTION('center_axis',(-1.4923676700635E-16,0.,1.)) ;
#60155=DIRECTION('ref_axis',(-0.707106781186359,-0.707106781186736,-1.05526329952519E-16)) ;
#60156=DIRECTION('center_axis',(0.,0.,1.)) ;
#60157=DIRECTION('ref_axis',(-0.707106781186359,-0.707106781186736,0.)) ;
#60158=DIRECTION('',(0.,0.,1.)) ;
#60159=DIRECTION('center_axis',(0.,0.,-1.)) ;
#60160=DIRECTION('ref_axis',(0.,-1.,0.)) ;
#60161=DIRECTION('center_axis',(3.55271367880051E-14,1.,0.)) ;
#60162=DIRECTION('ref_axis',(0.,0.,1.)) ;
#60163=DIRECTION('center_axis',(-1.,4.25984888819251E-25,9.5923269327607E-12)) ;
#60164=DIRECTION('ref_axis',(-3.39809272400367E-40,-1.,4.44089209849993E-14)) ;
#60165=DIRECTION('center_axis',(3.55271367880051E-14,1.,0.)) ;
#60166=DIRECTION('ref_axis',(-0.707106781186548,2.51214793389405E-14,0.707106781186547)) ;
#60167=DIRECTION('center_axis',(-1.,3.55271367880051E-14,-1.51760508056877E-16)) ;
#60168=DIRECTION('ref_axis',(-2.52287902233016E-14,-0.707106781186485,0.70710678118661)) ;
#60169=DIRECTION('center_axis',(0.70710678118661,-0.707106781186485,0.)) ;
#60170=DIRECTION('ref_axis',(-0.707106781186485,-0.70710678118661,-1.22663473334685E-16)) ;
#60171=DIRECTION('center_axis',(-3.55271367880051E-14,-1.,0.)) ;
#60172=DIRECTION('ref_axis',(1.,-3.55271367880051E-14,1.4923676700635E-16)) ;
#60173=DIRECTION('',(0.,0.,1.)) ;
#60174=DIRECTION('',(0.,0.,-1.)) ;
#60175=DIRECTION('center_axis',(0.,0.,-1.)) ;
#60176=DIRECTION('ref_axis',(-1.,0.,0.)) ;
#60177=DIRECTION('center_axis',(-4.44089209849993E-14,4.44089209849993E-14,
-1.)) ;
#60178=DIRECTION('ref_axis',(-0.707106781186547,-0.707106781186547,-2.16129177030881E-30)) ;
#60179=DIRECTION('center_axis',(-0.707106781186503,0.707106781186592,0.)) ;
#60180=DIRECTION('ref_axis',(0.,0.,1.)) ;
#60181=DIRECTION('center_axis',(1.,0.,0.)) ;
#60182=DIRECTION('ref_axis',(0.,1.,0.)) ;
#60183=DIRECTION('center_axis',(-8.88178419700144E-14,0.,-1.)) ;
#60184=DIRECTION('ref_axis',(-1.,0.,8.28966525053497E-14)) ;
#60185=DIRECTION('center_axis',(0.,-6.28036983473606E-14,-1.)) ;
#60186=DIRECTION('ref_axis',(-1.,0.,0.)) ;
#60187=DIRECTION('center_axis',(0.,1.,0.)) ;
#60188=DIRECTION('ref_axis',(0.,0.,1.)) ;
#60189=DIRECTION('center_axis',(0.707106781186503,-0.707106781186592,-6.28036983473484E-14)) ;
#60190=DIRECTION('ref_axis',(0.707106781186592,0.707106781186503,2.27272335701132E-30)) ;
#60191=DIRECTION('center_axis',(0.,0.,-1.)) ;
#60192=DIRECTION('ref_axis',(-1.,0.,0.)) ;
#60193=DIRECTION('center_axis',(4.44089209850072E-14,4.44089209850072E-14,
-1.)) ;
#60194=DIRECTION('ref_axis',(-0.707106781186547,0.707106781186547,-2.2709071609452E-30)) ;
#60195=DIRECTION('center_axis',(0.707106781186548,0.707106781186548,0.)) ;
#60196=DIRECTION('ref_axis',(0.,0.,1.)) ;
#60197=DIRECTION('center_axis',(0.,-1.,0.)) ;
#60198=DIRECTION('ref_axis',(1.,0.,0.)) ;
#60199=DIRECTION('center_axis',(0.,0.,-1.)) ;
#60200=DIRECTION('ref_axis',(-1.,0.,0.)) ;
#60201=DIRECTION('center_axis',(0.,0.,-1.)) ;
#60202=DIRECTION('ref_axis',(0.,1.,0.)) ;
#60203=DIRECTION('center_axis',(1.,0.,0.)) ;
#60204=DIRECTION('ref_axis',(0.,0.,1.)) ;
#60205=DIRECTION('center_axis',(-0.707106781186548,-0.707106781186548,0.)) ;
#60206=DIRECTION('ref_axis',(0.707106781186547,-0.707106781186547,0.)) ;
#60207=DIRECTION('center_axis',(1.,0.,1.51760508056877E-16)) ;
#60208=DIRECTION('ref_axis',(-1.07310884363343E-16,-0.707106781186485,0.70710678118661)) ;
#60209=DIRECTION('',(1.,0.,1.51760508056877E-16)) ;
#60210=DIRECTION('center_axis',(-7.105427357601E-15,-1.,-1.07888364883526E-30)) ;
#60211=DIRECTION('ref_axis',(-0.707106781186453,5.02429586778741E-15,0.707106781186642)) ;
#60212=DIRECTION('center_axis',(-0.707106781186563,-0.707106781186532,-1.07310884363336E-16)) ;
#60213=DIRECTION('ref_axis',(0.499999999999956,-0.499999999999978,0.707106781186594)) ;
#60214=DIRECTION('',(0.707106781186563,0.707106781186532,1.07310884363336E-16)) ;
#60215=DIRECTION('center_axis',(0.,0.,1.)) ;
#60216=DIRECTION('ref_axis',(-0.382683432365099,0.923879532511283,0.)) ;
#60217=DIRECTION('',(0.,0.,1.)) ;
#60218=DIRECTION('',(0.,0.,-1.)) ;
#60219=DIRECTION('center_axis',(3.73034936274055E-14,1.,5.66175752827605E-30)) ;
#60220=DIRECTION('ref_axis',(0.707106781186516,-2.63775533058864E-14,0.707106781186579)) ;
#60221=DIRECTION('',(3.73034936274055E-14,1.,5.66175752827605E-30)) ;
#60222=DIRECTION('center_axis',(0.,0.,-1.)) ;
#60223=DIRECTION('ref_axis',(-0.923879532511297,0.382683432365065,0.)) ;
#60224=DIRECTION('',(0.,0.,1.)) ;
#60225=DIRECTION('',(0.,0.,-1.)) ;
#60226=DIRECTION('center_axis',(0.707106781186575,-0.70710678118652,1.07310884363338E-16)) ;
#60227=DIRECTION('ref_axis',(0.499999999999948,0.499999999999987,0.707106781186594)) ;
#60228=DIRECTION('',(-0.707106781186575,0.70710678118652,-1.07310884363338E-16)) ;
#60229=DIRECTION('center_axis',(0.,0.,1.)) ;
#60230=DIRECTION('ref_axis',(-0.923879532511297,-0.382683432365065,0.)) ;
#60231=DIRECTION('',(0.,0.,1.)) ;
#60232=DIRECTION('',(0.,0.,-1.)) ;
#60233=DIRECTION('center_axis',(-1.,7.10542735760144E-15,-1.51760508056877E-16)) ;
#60234=DIRECTION('ref_axis',(4.91698498342642E-15,0.707106781186736,0.707106781186359)) ;
#60235=DIRECTION('',(-1.,7.10542735760144E-15,-1.51760508056877E-16)) ;
#60236=DIRECTION('center_axis',(0.,0.,-1.)) ;
#60237=DIRECTION('ref_axis',(-0.382683432364963,-0.923879532511339,0.)) ;
#60238=DIRECTION('',(0.,0.,1.)) ;
#60239=DIRECTION('',(0.,0.,-1.)) ;
#60240=DIRECTION('center_axis',(-7.105427357601E-15,-1.,-1.07888364883526E-30)) ;
#60241=DIRECTION('ref_axis',(-0.707106781186453,5.02429586778741E-15,0.707106781186642)) ;
#60242=DIRECTION('',(-7.105427357601E-15,-1.,-1.07888364883526E-30)) ;
#60243=DIRECTION('center_axis',(0.707106781186532,-0.707106781186563,0.)) ;
#60244=DIRECTION('ref_axis',(0.,0.,-1.)) ;
#60245=DIRECTION('center_axis',(-1.,3.73034936274055E-14,0.)) ;
#60246=DIRECTION('ref_axis',(-3.73034936274055E-14,-1.,-5.56705278699598E-30)) ;
#60247=DIRECTION('center_axis',(0.70710678118652,0.707106781186575,0.)) ;
#60248=DIRECTION('ref_axis',(0.,0.,-1.)) ;
#60249=DIRECTION('center_axis',(-7.10542735760144E-15,-1.,0.)) ;
#60250=DIRECTION('ref_axis',(1.,-7.10542735760144E-15,1.4923676700635E-16)) ;
#60251=DIRECTION('center_axis',(1.,-7.105427357601E-15,0.)) ;
#60252=DIRECTION('ref_axis',(7.105427357601E-15,1.,1.06039100704685E-30)) ;
#60253=DIRECTION('center_axis',(0.,-1.,-5.60383084497428E-34)) ;
#60254=DIRECTION('ref_axis',(0.707106781186548,3.96250679110365E-34,-0.707106781186548)) ;
#60255=DIRECTION('',(0.,-1.,-5.60383084497428E-34)) ;
#60256=DIRECTION('center_axis',(-1.,0.,0.)) ;
#60257=DIRECTION('ref_axis',(0.,-1.,0.)) ;
#60258=DIRECTION('center_axis',(0.,-1.,-5.60383084497428E-34)) ;
#60259=DIRECTION('ref_axis',(0.707106781186548,3.96250679110365E-34,-0.707106781186548)) ;
#60260=DIRECTION('',(0.,-1.,-5.60383084497428E-34)) ;
#60261=DIRECTION('center_axis',(-1.,0.,0.)) ;
#60262=DIRECTION('ref_axis',(0.,-1.,0.)) ;
#60263=DIRECTION('center_axis',(0.,0.,1.)) ;
#60264=DIRECTION('ref_axis',(1.,0.,0.)) ;
#60265=DIRECTION('center_axis',(0.,1.,0.)) ;
#60266=DIRECTION('ref_axis',(-1.,0.,0.)) ;
#60267=DIRECTION('center_axis',(0.,0.,-1.)) ;
#60268=DIRECTION('ref_axis',(0.,-1.,0.)) ;
#60269=DIRECTION('center_axis',(-1.,0.,0.)) ;
#60270=DIRECTION('ref_axis',(0.,0.,1.)) ;
#60271=DIRECTION('center_axis',(0.,0.,1.)) ;
#60272=DIRECTION('ref_axis',(1.,0.,0.)) ;
#60273=DIRECTION('center_axis',(0.,0.,1.)) ;
#60274=DIRECTION('ref_axis',(1.,0.,0.)) ;
#60275=DIRECTION('center_axis',(0.,1.,0.)) ;
#60276=DIRECTION('ref_axis',(0.,0.,-1.)) ;
#60277=DIRECTION('center_axis',(-1.,0.,0.)) ;
#60278=DIRECTION('ref_axis',(0.,1.,0.)) ;
#60279=DIRECTION('center_axis',(0.,0.,1.)) ;
#60280=DIRECTION('ref_axis',(1.,0.,0.)) ;
#60281=DIRECTION('center_axis',(-1.,0.,0.)) ;
#60282=DIRECTION('ref_axis',(0.,-1.,0.)) ;
#60283=DIRECTION('center_axis',(0.,0.,-1.)) ;
#60284=DIRECTION('ref_axis',(1.,0.,0.)) ;
#60285=DIRECTION('center_axis',(0.,-1.,0.)) ;
#60286=DIRECTION('ref_axis',(0.,0.,1.)) ;
#60287=DIRECTION('center_axis',(0.,0.,-1.)) ;
#60288=DIRECTION('ref_axis',(-1.,0.,0.)) ;
#60289=DIRECTION('center_axis',(0.,0.,-1.)) ;
#60290=DIRECTION('ref_axis',(-1.,0.,0.)) ;
#60291=DIRECTION('center_axis',(0.,1.,0.)) ;
#60292=DIRECTION('ref_axis',(0.,0.,1.)) ;
#60293=DIRECTION('center_axis',(1.,0.,0.)) ;
#60294=DIRECTION('ref_axis',(0.,1.,0.)) ;
#60295=DIRECTION('center_axis',(0.,0.,-1.)) ;
#60296=DIRECTION('ref_axis',(-1.,0.,0.)) ;
#60297=DIRECTION('center_axis',(0.,1.,0.)) ;
#60298=DIRECTION('ref_axis',(1.,0.,0.)) ;
#60299=DIRECTION('center_axis',(0.,0.,1.)) ;
#60300=DIRECTION('ref_axis',(0.,-1.,0.)) ;
#60301=DIRECTION('center_axis',(1.,0.,0.)) ;
#60302=DIRECTION('ref_axis',(0.,0.,-1.)) ;
#60303=DIRECTION('center_axis',(0.,0.,1.)) ;
#60304=DIRECTION('ref_axis',(1.,0.,0.)) ;
#60305=DIRECTION('center_axis',(0.,0.,1.)) ;
#60306=DIRECTION('ref_axis',(0.,1.,0.)) ;
#60307=DIRECTION('center_axis',(-1.,0.,0.)) ;
#60308=DIRECTION('ref_axis',(0.,0.,-1.)) ;
#60309=DIRECTION('center_axis',(0.,-1.,0.)) ;
#60310=DIRECTION('ref_axis',(-1.,0.,0.)) ;
#60311=DIRECTION('center_axis',(0.,0.,1.)) ;
#60312=DIRECTION('ref_axis',(1.,0.,0.)) ;
#60313=DIRECTION('center_axis',(0.,-1.,0.)) ;
#60314=DIRECTION('ref_axis',(1.,0.,0.)) ;
#60315=DIRECTION('center_axis',(-4.44089209850092E-14,0.,-1.)) ;
#60316=DIRECTION('ref_axis',(0.,1.,0.)) ;
#60317=DIRECTION('center_axis',(1.,0.,0.)) ;
#60318=DIRECTION('ref_axis',(0.,0.,1.)) ;
#60319=DIRECTION('center_axis',(5.55111512312578E-16,1.,8.48043882212758E-32)) ;
#60320=DIRECTION('ref_axis',(0.707106781186579,-3.92523114670961E-16,0.707106781186516)) ;
#60321=DIRECTION('',(5.55111512312578E-16,1.,8.48043882212758E-32)) ;
#60322=DIRECTION('center_axis',(0.,0.,1.)) ;
#60323=DIRECTION('ref_axis',(1.,0.,0.)) ;
#60324=DIRECTION('center_axis',(0.,0.,1.)) ;
#60325=DIRECTION('ref_axis',(-1.,0.,0.)) ;
#60326=DIRECTION('center_axis',(0.,-1.,0.)) ;
#60327=DIRECTION('ref_axis',(0.,0.,-1.)) ;
#60328=DIRECTION('center_axis',(1.,0.,0.)) ;
#60329=DIRECTION('ref_axis',(0.,-1.,0.)) ;
#60330=DIRECTION('center_axis',(-5.55111512312578E-16,-1.,-8.48043882212758E-32)) ;
#60331=DIRECTION('ref_axis',(0.707106781186548,-3.92523114670943E-16,-0.707106781186548)) ;
#60332=DIRECTION('',(-5.55111512312578E-16,-1.,-8.48043882212758E-32)) ;
#60333=DIRECTION('center_axis',(-1.,0.,-1.51760508056877E-16)) ;
#60334=DIRECTION('ref_axis',(1.07310884363343E-16,-0.707106781186485,-0.70710678118661)) ;
#60335=DIRECTION('',(-1.,0.,-1.51760508056877E-16)) ;
#60336=DIRECTION('center_axis',(0.,0.,1.)) ;
#60337=DIRECTION('ref_axis',(-0.707106781186579,0.707106781186516,0.)) ;
#60338=DIRECTION('',(0.,0.,-1.)) ;
#60339=DIRECTION('',(0.,0.,1.)) ;
#60340=DIRECTION('center_axis',(1.,0.,1.51760508056877E-16)) ;
#60341=DIRECTION('ref_axis',(-1.07310884363343E-16,-0.707106781186485,0.70710678118661)) ;
#60342=DIRECTION('',(1.,0.,1.51760508056877E-16)) ;
#60343=DIRECTION('center_axis',(-1.11022302462516E-15,1.,-1.67927627189059E-31)) ;
#60344=DIRECTION('ref_axis',(-0.707106781186548,-7.8504622934189E-16,-0.707106781186548)) ;
#60345=DIRECTION('',(-1.11022302462516E-15,1.,-1.67927627189059E-31)) ;
#60346=DIRECTION('center_axis',(0.,0.,1.)) ;
#60347=DIRECTION('ref_axis',(0.70710678118661,0.707106781186485,0.)) ;
#60348=DIRECTION('',(0.,0.,-1.)) ;
#60349=DIRECTION('',(0.,0.,1.)) ;
#60350=DIRECTION('center_axis',(0.,0.,1.)) ;
#60351=DIRECTION('ref_axis',(-0.70710678118661,-0.707106781186485,0.)) ;
#60352=DIRECTION('',(0.,0.,-1.)) ;
#60353=DIRECTION('',(0.,0.,1.)) ;
#60354=DIRECTION('center_axis',(1.,0.,1.51760508056877E-16)) ;
#60355=DIRECTION('ref_axis',(1.07310884363343E-16,0.707106781186485,-0.70710678118661)) ;
#60356=DIRECTION('',(1.,0.,1.51760508056877E-16)) ;
#60357=DIRECTION('center_axis',(-1.,0.,-1.51760508056877E-16)) ;
#60358=DIRECTION('ref_axis',(-1.07310884363343E-16,0.707106781186485,0.70710678118661)) ;
#60359=DIRECTION('',(-1.,0.,-1.51760508056877E-16)) ;
#60360=DIRECTION('center_axis',(1.11022302462516E-15,-1.,1.67927627189059E-31)) ;
#60361=DIRECTION('ref_axis',(-0.707106781186548,-7.8504622934189E-16,0.707106781186548)) ;
#60362=DIRECTION('',(1.11022302462516E-15,-1.,1.67927627189059E-31)) ;
#60363=DIRECTION('center_axis',(0.,0.,1.)) ;
#60364=DIRECTION('ref_axis',(0.70710678118661,-0.707106781186485,0.)) ;
#60365=DIRECTION('',(0.,0.,-1.)) ;
#60366=DIRECTION('',(0.,0.,1.)) ;
#60367=DIRECTION('center_axis',(-1.,5.55111512312578E-16,0.)) ;
#60368=DIRECTION('ref_axis',(-5.55111512312578E-16,-1.,-8.28430474255348E-32)) ;
#60369=DIRECTION('center_axis',(0.,1.,0.)) ;
#60370=DIRECTION('ref_axis',(-1.,0.,-1.4923676700635E-16)) ;
#60371=DIRECTION('center_axis',(1.,1.11022302462516E-15,0.)) ;
#60372=DIRECTION('ref_axis',(-1.11022302462516E-15,1.,-1.6568609485107E-31)) ;
#60373=DIRECTION('center_axis',(0.,-1.,0.)) ;
#60374=DIRECTION('ref_axis',(1.,0.,1.4923676700635E-16)) ;
#60375=DIRECTION('center_axis',(-1.51760508056877E-16,-5.60383084497428E-34,
1.)) ;
#60376=DIRECTION('ref_axis',(1.,0.,0.)) ;
#60377=DIRECTION('center_axis',(0.,-1.,-5.60383084497428E-34)) ;
#60378=DIRECTION('ref_axis',(-1.,0.,0.)) ;
#60379=DIRECTION('center_axis',(-1.51760508056877E-16,-5.60383084497428E-34,
1.)) ;
#60380=DIRECTION('ref_axis',(1.,-2.24153233798967E-35,1.51760508056877E-16)) ;
#60381=DIRECTION('center_axis',(-2.01858731750028E-16,0.,1.)) ;
#60382=DIRECTION('ref_axis',(1.,0.,2.01858731750028E-16)) ;
#60383=DIRECTION('',(-2.01858731750028E-16,0.,1.)) ;
#60384=DIRECTION('center_axis',(1.51760508056877E-16,5.60383084497428E-34,
-1.)) ;
#60385=DIRECTION('ref_axis',(1.,2.24153233798966E-35,1.51760508056877E-16)) ;
#60386=DIRECTION('center_axis',(1.51760508056877E-16,5.60383084497428E-34,
-1.)) ;
#60387=DIRECTION('ref_axis',(1.,2.24153233798966E-35,1.51760508056877E-16)) ;
#60388=DIRECTION('center_axis',(1.51760508056877E-16,5.60383084497428E-34,
-1.)) ;
#60389=DIRECTION('ref_axis',(-1.,0.,0.)) ;
#60390=DIRECTION('center_axis',(0.,-1.,-5.60383084497428E-34)) ;
#60391=DIRECTION('ref_axis',(1.,0.,0.)) ;
#60392=DIRECTION('center_axis',(0.,0.,1.)) ;
#60393=DIRECTION('ref_axis',(0.70710678118661,0.707106781186485,0.)) ;
#60394=DIRECTION('center_axis',(-1.4923676700635E-16,0.,1.)) ;
#60395=DIRECTION('ref_axis',(0.70710678118661,0.707106781186485,1.05526329952556E-16)) ;
#60396=DIRECTION('',(0.,0.,1.)) ;
#60397=DIRECTION('center_axis',(0.,0.,-1.)) ;
#60398=DIRECTION('ref_axis',(0.,1.,0.)) ;
#60399=DIRECTION('',(0.,0.,-1.)) ;
#60400=DIRECTION('center_axis',(0.,-1.,0.)) ;
#60401=DIRECTION('ref_axis',(0.,0.,-1.)) ;
#60402=DIRECTION('center_axis',(1.,1.97215226305235E-27,4.44089209850092E-14)) ;
#60403=DIRECTION('ref_axis',(8.40779078574419E-43,1.,-4.44089209849993E-14)) ;
#60404=DIRECTION('center_axis',(0.,1.,0.)) ;
#60405=DIRECTION('ref_axis',(0.707106781186548,0.,0.707106781186548)) ;
#60406=DIRECTION('center_axis',(0.,-1.,0.)) ;
#60407=DIRECTION('ref_axis',(0.707106781186547,0.,0.707106781186547)) ;
#60408=DIRECTION('center_axis',(1.,0.,1.51760508056877E-16)) ;
#60409=DIRECTION('ref_axis',(-1.07310884363305E-16,0.707106781186736,0.707106781186359)) ;
#60410=DIRECTION('center_axis',(-0.70710678118661,0.707106781186485,0.)) ;
#60411=DIRECTION('ref_axis',(0.707106781186485,0.70710678118661,1.83995210002021E-16)) ;
#60412=DIRECTION('center_axis',(0.,1.,0.)) ;
#60413=DIRECTION('ref_axis',(-1.,0.,-1.4923676700635E-16)) ;
#60414=DIRECTION('',(1.,0.,1.4923676700635E-16)) ;
#60415=DIRECTION('',(0.,0.,1.)) ;
#60416=DIRECTION('center_axis',(-1.4923676700635E-16,0.,1.)) ;
#60417=DIRECTION('ref_axis',(1.,0.,1.4923676700635E-16)) ;
#60418=DIRECTION('',(0.,-1.,0.)) ;
#60419=DIRECTION('center_axis',(-1.4923676700635E-16,0.,1.)) ;
#60420=DIRECTION('ref_axis',(0.707106781186642,-0.707106781186453,1.05526329952561E-16)) ;
#60421=DIRECTION('',(-1.,-3.55271367880051E-14,-1.4923676700635E-16)) ;
#60422=DIRECTION('',(0.,1.,0.)) ;
#60423=DIRECTION('center_axis',(1.,0.,0.)) ;
#60424=DIRECTION('ref_axis',(0.,1.,0.)) ;
#60425=DIRECTION('',(0.,1.,5.60383084497428E-34)) ;
#60426=DIRECTION('',(0.,0.,1.)) ;
#60427=DIRECTION('center_axis',(0.,0.,1.)) ;
#60428=DIRECTION('ref_axis',(0.707106781186642,-0.707106781186453,0.)) ;
#60429=DIRECTION('center_axis',(0.,0.,-1.)) ;
#60430=DIRECTION('ref_axis',(1.,0.,0.)) ;
#60431=DIRECTION('',(0.,0.,-1.)) ;
#60432=DIRECTION('center_axis',(-3.55271367880051E-14,1.,0.)) ;
#60433=DIRECTION('ref_axis',(0.,0.,1.)) ;
#60434=DIRECTION('center_axis',(1.,4.44089209849835E-14,0.)) ;
#60435=DIRECTION('ref_axis',(0.,0.,1.)) ;
#60436=DIRECTION('center_axis',(-3.55271367880051E-14,1.,0.)) ;
#60437=DIRECTION('ref_axis',(0.707106781186546,2.51214793389404E-14,0.707106781186549)) ;
#60438=DIRECTION('center_axis',(3.55271367880051E-14,-1.,0.)) ;
#60439=DIRECTION('ref_axis',(0.707106781186546,2.51214793389404E-14,0.707106781186549)) ;
#60440=DIRECTION('center_axis',(-1.,-3.55271367880051E-14,-1.51760508056877E-16)) ;
#60441=DIRECTION('ref_axis',(2.50141684545749E-14,-0.707106781186485,0.70710678118661)) ;
#60442=DIRECTION('center_axis',(-0.70710678118661,-0.707106781186485,0.)) ;
#60443=DIRECTION('ref_axis',(0.707106781186485,-0.70710678118661,2.4532694666937E-16)) ;
#60444=DIRECTION('center_axis',(0.,1.,5.60383084497428E-34)) ;
#60445=DIRECTION('ref_axis',(0.707106781186548,-3.96250679110365E-34,0.707106781186548)) ;
#60446=DIRECTION('center_axis',(0.,0.,-1.)) ;
#60447=DIRECTION('ref_axis',(-1.,0.,0.)) ;
#60448=DIRECTION('center_axis',(-1.,0.,0.)) ;
#60449=DIRECTION('ref_axis',(0.,0.,1.)) ;
#60450=DIRECTION('center_axis',(0.707106781186503,0.707106781186592,0.)) ;
#60451=DIRECTION('ref_axis',(-0.707106781186592,0.707106781186503,0.)) ;
#60452=DIRECTION('center_axis',(-1.,0.,-1.51760508056877E-16)) ;
#60453=DIRECTION('ref_axis',(-1.07310884363343E-16,0.707106781186485,0.70710678118661)) ;
#60454=DIRECTION('center_axis',(0.70710678118661,-0.707106781186485,0.)) ;
#60455=DIRECTION('ref_axis',(0.707106781186485,0.70710678118661,2.14621768726686E-16)) ;
#60456=DIRECTION('center_axis',(0.,0.,-1.)) ;
#60457=DIRECTION('ref_axis',(-1.,0.,0.)) ;
#60458=DIRECTION('center_axis',(-0.707106781186481,-0.707106781186614,0.)) ;
#60459=DIRECTION('ref_axis',(0.,0.,1.)) ;
#60460=DIRECTION('center_axis',(0.,1.,0.)) ;
#60461=DIRECTION('ref_axis',(-1.,0.,0.)) ;
#60462=DIRECTION('center_axis',(0.707106781186555,0.70710678118654,1.07310884363335E-16)) ;
#60463=DIRECTION('ref_axis',(-0.499999999999977,0.499999999999988,0.707106781186572)) ;
#60464=DIRECTION('center_axis',(0.,0.,-1.)) ;
#60465=DIRECTION('ref_axis',(-1.,0.,0.)) ;
#60466=DIRECTION('center_axis',(0.,-1.,0.)) ;
#60467=DIRECTION('ref_axis',(0.,0.,1.)) ;
#60468=DIRECTION('center_axis',(-0.707106781186548,0.707106781186548,0.)) ;
#60469=DIRECTION('ref_axis',(-0.707106781186547,-0.707106781186547,0.)) ;
#60470=DIRECTION('center_axis',(1.1311821873082E-49,-1.,-5.60383084497428E-34)) ;
#60471=DIRECTION('ref_axis',(-0.707106781186548,-3.96250679110365E-34,0.707106781186548)) ;
#60472=DIRECTION('center_axis',(0.,0.,-1.)) ;
#60473=DIRECTION('ref_axis',(-1.,0.,0.)) ;
#60474=DIRECTION('center_axis',(0.70710678118657,-0.707106781186525,0.)) ;
#60475=DIRECTION('ref_axis',(0.,0.,1.)) ;
#60476=DIRECTION('center_axis',(-1.,0.,0.)) ;
#60477=DIRECTION('ref_axis',(0.,-1.,0.)) ;
#60478=DIRECTION('center_axis',(-0.707106781186555,0.70710678118654,-1.07310884363335E-16)) ;
#60479=DIRECTION('ref_axis',(-0.499999999999962,-0.499999999999972,0.707106781186594)) ;
#60480=DIRECTION('center_axis',(0.,0.,-1.)) ;
#60481=DIRECTION('ref_axis',(-1.,0.,0.)) ;
#60482=DIRECTION('center_axis',(1.,0.,0.)) ;
#60483=DIRECTION('ref_axis',(0.,0.,1.)) ;
#60484=DIRECTION('center_axis',(0.,-1.,0.)) ;
#60485=DIRECTION('ref_axis',(1.,0.,0.)) ;
#60486=DIRECTION('center_axis',(1.,0.,1.51760508056877E-16)) ;
#60487=DIRECTION('ref_axis',(-1.07310884363343E-16,-0.707106781186485,0.70710678118661)) ;
#60488=DIRECTION('center_axis',(-1.1311821873082E-49,1.,5.60383084497428E-34)) ;
#60489=DIRECTION('ref_axis',(0.707106781186548,-3.96250679110365E-34,0.707106781186548)) ;
#60490=DIRECTION('center_axis',(-1.1311821873082E-49,1.,5.60383084497428E-34)) ;
#60491=DIRECTION('ref_axis',(0.707106781186548,-3.96250679110365E-34,0.707106781186548)) ;
#60492=DIRECTION('',(-1.1311821873082E-49,1.,5.60383084497428E-34)) ;
#60493=DIRECTION('center_axis',(1.51760508056877E-16,5.60383084497428E-34,
-1.)) ;
#60494=DIRECTION('ref_axis',(-1.,0.,0.)) ;
#60495=DIRECTION('center_axis',(0.,-1.,-5.60383084497428E-34)) ;
#60496=DIRECTION('ref_axis',(1.,0.,0.)) ;
#60497=DIRECTION('center_axis',(1.51760508056877E-16,5.60383084497428E-34,
-1.)) ;
#60498=DIRECTION('ref_axis',(1.,2.24153233798966E-35,1.51760508056877E-16)) ;
#60499=DIRECTION('center_axis',(1.51760508056877E-16,5.60383084497428E-34,
-1.)) ;
#60500=DIRECTION('ref_axis',(1.,2.24153233798966E-35,1.51760508056877E-16)) ;
#60501=DIRECTION('center_axis',(0.,0.,1.)) ;
#60502=DIRECTION('ref_axis',(1.,0.,0.)) ;
#60503=DIRECTION('',(0.,0.,1.)) ;
#60504=DIRECTION('center_axis',(1.51760508056877E-16,5.60383084497428E-34,
-1.)) ;
#60505=DIRECTION('ref_axis',(-1.,0.,0.)) ;
#60506=DIRECTION('center_axis',(0.,-1.,-5.60383084497428E-34)) ;
#60507=DIRECTION('ref_axis',(1.,0.,0.)) ;
#60508=DIRECTION('center_axis',(1.51760508056877E-16,5.60383084497428E-34,
-1.)) ;
#60509=DIRECTION('ref_axis',(1.,2.80191542248707E-35,1.51760508056877E-16)) ;
#60510=DIRECTION('center_axis',(1.51760508056877E-16,5.60383084497428E-34,
-1.)) ;
#60511=DIRECTION('ref_axis',(1.,2.80191542248707E-35,1.51760508056877E-16)) ;
#60512=DIRECTION('center_axis',(0.,0.,1.)) ;
#60513=DIRECTION('ref_axis',(1.,0.,0.)) ;
#60514=DIRECTION('',(0.,0.,1.)) ;
#60515=DIRECTION('center_axis',(0.,1.,5.60383084497428E-34)) ;
#60516=DIRECTION('ref_axis',(0.707106781186548,3.96250679110365E-34,-0.707106781186548)) ;
#60517=DIRECTION('center_axis',(0.,1.,0.)) ;
#60518=DIRECTION('ref_axis',(1.,0.,0.)) ;
#60519=DIRECTION('center_axis',(1.51760508056877E-16,5.60383084497428E-34,
-1.)) ;
#60520=DIRECTION('ref_axis',(-1.,0.,0.)) ;
#60521=DIRECTION('center_axis',(-0.707106781186548,0.707106781186548,0.)) ;
#60522=DIRECTION('ref_axis',(0.707106781186547,0.707106781186547,0.)) ;
#60523=DIRECTION('center_axis',(-1.51760508056877E-16,-5.60383084497428E-34,
1.)) ;
#60524=DIRECTION('ref_axis',(-0.923879532511284,-0.382683432365097,-1.40208427237262E-16)) ;
#60525=DIRECTION('center_axis',(-0.707106781186615,0.70710678118648,-1.07310884363344E-16)) ;
#60526=DIRECTION('ref_axis',(0.499999999999888,0.499999999999984,-0.707106781186638)) ;
#60527=DIRECTION('center_axis',(-0.707106781186548,0.707106781186548,0.)) ;
#60528=DIRECTION('ref_axis',(0.707106781186547,0.707106781186547,0.)) ;
#60529=DIRECTION('center_axis',(-1.51760508056877E-16,-5.60383084497428E-34,
1.)) ;
#60530=DIRECTION('ref_axis',(1.,0.,0.)) ;
#60531=DIRECTION('center_axis',(0.,1.,0.)) ;
#60532=DIRECTION('ref_axis',(1.,0.,0.)) ;
#60533=DIRECTION('center_axis',(-6.83214169000096E-16,1.,-1.03124546314615E-31)) ;
#60534=DIRECTION('ref_axis',(0.707106781186485,4.83105371902657E-16,-0.70710678118661)) ;
#60535=DIRECTION('center_axis',(0.,1.,0.)) ;
#60536=DIRECTION('ref_axis',(1.,0.,0.)) ;
#60537=DIRECTION('center_axis',(-1.51760508056877E-16,-5.60383084497428E-34,
1.)) ;
#60538=DIRECTION('ref_axis',(1.,0.,0.)) ;
#60539=DIRECTION('center_axis',(0.999479573214818,0.0322580645161017,0.)) ;
#60540=DIRECTION('ref_axis',(0.0322580645161017,-0.999479573214818,0.)) ;
#60541=DIRECTION('center_axis',(1.51760508056877E-16,5.60383084497428E-34,
-1.)) ;
#60542=DIRECTION('ref_axis',(-1.,0.,0.)) ;
#60543=DIRECTION('center_axis',(0.,1.,0.)) ;
#60544=DIRECTION('ref_axis',(1.,0.,0.)) ;
#60545=DIRECTION('center_axis',(0.,1.,5.60383084497428E-34)) ;
#60546=DIRECTION('ref_axis',(0.707106781186485,3.962506791104E-34,-0.70710678118661)) ;
#60547=DIRECTION('center_axis',(0.,1.,0.)) ;
#60548=DIRECTION('ref_axis',(1.,0.,0.)) ;
#60549=DIRECTION('center_axis',(1.51760508056877E-16,5.60383084497428E-34,
-1.)) ;
#60550=DIRECTION('ref_axis',(-1.,0.,0.)) ;
#60551=DIRECTION('center_axis',(-0.999479573214819,0.0322580645160902,0.)) ;
#60552=DIRECTION('ref_axis',(0.0322580645160902,0.999479573214818,0.)) ;
#60553=DIRECTION('center_axis',(-1.51760508056877E-16,-5.60383084497428E-34,
1.)) ;
#60554=DIRECTION('ref_axis',(1.,0.,0.)) ;
#60555=DIRECTION('center_axis',(0.,1.,0.)) ;
#60556=DIRECTION('ref_axis',(1.,0.,0.)) ;
#60557=DIRECTION('center_axis',(-6.83214169000096E-16,1.,-1.03124546314615E-31)) ;
#60558=DIRECTION('ref_axis',(0.70710678118661,4.83105371902742E-16,-0.707106781186485)) ;
#60559=DIRECTION('center_axis',(0.,1.,0.)) ;
#60560=DIRECTION('ref_axis',(1.,0.,0.)) ;
#60561=DIRECTION('center_axis',(-1.51760508056877E-16,-5.60383084497428E-34,
1.)) ;
#60562=DIRECTION('ref_axis',(1.,0.,0.)) ;
#60563=DIRECTION('center_axis',(0.707106781186548,0.707106781186548,0.)) ;
#60564=DIRECTION('ref_axis',(0.707106781186547,-0.707106781186547,0.)) ;
#60565=DIRECTION('center_axis',(0.707106781186521,0.707106781186574,1.0731088436333E-16)) ;
#60566=DIRECTION('ref_axis',(0.499999999999986,-0.499999999999948,-0.707106781186594)) ;
#60567=DIRECTION('center_axis',(0.707106781186548,0.707106781186548,0.)) ;
#60568=DIRECTION('ref_axis',(0.707106781186547,-0.707106781186547,0.)) ;
#60569=DIRECTION('center_axis',(1.51760508056877E-16,5.60383084497428E-34,
-1.)) ;
#60570=DIRECTION('ref_axis',(-1.,0.,0.)) ;
#60571=DIRECTION('center_axis',(0.,1.,0.)) ;
#60572=DIRECTION('ref_axis',(1.,0.,0.)) ;
#60573=DIRECTION('center_axis',(-5.23472275150178E-15,1.,-7.93863801220309E-31)) ;
#60574=DIRECTION('ref_axis',(0.707106781186548,3.70150795521841E-15,-0.707106781186548)) ;
#60575=DIRECTION('center_axis',(0.,1.,0.)) ;
#60576=DIRECTION('ref_axis',(1.,0.,0.)) ;
#60577=DIRECTION('center_axis',(-1.51760508056877E-16,-5.60383084497428E-34,
1.)) ;
#60578=DIRECTION('ref_axis',(1.,0.,0.)) ;
#60579=DIRECTION('center_axis',(0.984807753012208,-0.173648177666931,0.)) ;
#60580=DIRECTION('ref_axis',(-0.173648177666931,-0.984807753012208,0.)) ;
#60581=DIRECTION('center_axis',(0.984807753012209,-0.173648177666924,1.49454924935485E-16)) ;
#60582=DIRECTION('ref_axis',(-0.122787803968973,-0.696364240320047,-0.70710678118652)) ;
#60583=DIRECTION('center_axis',(0.984807753012208,-0.173648177666931,0.)) ;
#60584=DIRECTION('ref_axis',(-0.173648177666931,-0.984807753012208,4.44089209850038E-14)) ;
#60585=DIRECTION('center_axis',(-1.51760508056877E-16,-5.60383084497428E-34,
1.)) ;
#60586=DIRECTION('ref_axis',(1.,0.,0.)) ;
#60587=DIRECTION('center_axis',(0.573576436350949,-0.81915204428906,0.)) ;
#60588=DIRECTION('ref_axis',(-0.81915204428906,-0.573576436350949,0.)) ;
#60589=DIRECTION('center_axis',(0.573576436351042,-0.819152044288994,8.70462513900874E-17)) ;
#60590=DIRECTION('ref_axis',(-0.579227965339616,-0.405579787672667,-0.707106781186493)) ;
#60591=DIRECTION('center_axis',(0.573576436351074,-0.819152044288972,0.)) ;
#60592=DIRECTION('ref_axis',(-0.819152044288972,-0.573576436351074,0.)) ;
#60593=DIRECTION('center_axis',(-1.51760508056877E-16,-5.60383084497428E-34,
1.)) ;
#60594=DIRECTION('ref_axis',(1.,0.,0.)) ;
#60595=DIRECTION('center_axis',(0.,-1.,0.)) ;
#60596=DIRECTION('ref_axis',(-1.,0.,0.)) ;
#60597=DIRECTION('center_axis',(-5.25359141716359E-35,-1.,-5.60383084497428E-34)) ;
#60598=DIRECTION('ref_axis',(-0.707106781186548,4.33399180276964E-34,-0.707106781186548)) ;
#60599=DIRECTION('center_axis',(0.,-1.,0.)) ;
#60600=DIRECTION('ref_axis',(-1.,0.,0.)) ;
#60601=DIRECTION('center_axis',(1.51760508056877E-16,5.60383084497428E-34,
-1.)) ;
#60602=DIRECTION('ref_axis',(-1.,0.,0.)) ;
#60603=DIRECTION('center_axis',(1.,0.,0.)) ;
#60604=DIRECTION('ref_axis',(0.,-1.,0.)) ;
#60605=DIRECTION('center_axis',(1.,0.,1.51760508056877E-16)) ;
#60606=DIRECTION('ref_axis',(1.07310884363343E-16,-0.707106781186485,-0.70710678118661)) ;
#60607=DIRECTION('center_axis',(1.,0.,0.)) ;
#60608=DIRECTION('ref_axis',(0.,-1.,0.)) ;
#60609=DIRECTION('center_axis',(-1.51760508056877E-16,-5.60383084497428E-34,
1.)) ;
#60610=DIRECTION('ref_axis',(1.,0.,0.)) ;
#60611=DIRECTION('center_axis',(0.,0.,1.)) ;
#60612=DIRECTION('ref_axis',(-0.923879532511279,-0.382683432365108,0.)) ;
#60613=DIRECTION('center_axis',(-1.51760508056877E-16,-5.60383084497428E-34,
1.)) ;
#60614=DIRECTION('ref_axis',(1.,0.,0.)) ;
#60615=DIRECTION('center_axis',(-1.,0.,0.)) ;
#60616=DIRECTION('ref_axis',(0.,0.,-1.)) ;
#60617=DIRECTION('center_axis',(1.51760508056877E-16,5.60383084497428E-34,
-1.)) ;
#60618=DIRECTION('ref_axis',(-0.70710678118657,-0.707106781186525,-1.07310884363337E-16)) ;
#60619=DIRECTION('center_axis',(1.,0.,1.51760508056877E-16)) ;
#60620=DIRECTION('ref_axis',(1.07310884363343E-16,-0.707106781186485,-0.70710678118661)) ;
#60621=DIRECTION('center_axis',(-1.,0.,0.)) ;
#60622=DIRECTION('ref_axis',(0.,0.,-1.)) ;
#60623=DIRECTION('',(-1.,0.,-1.51760508056877E-16)) ;
#60624=DIRECTION('center_axis',(-1.51760508056877E-16,-5.60383084497428E-34,
1.)) ;
#60625=DIRECTION('ref_axis',(1.,0.,0.)) ;
#60626=DIRECTION('center_axis',(0.,-1.,0.)) ;
#60627=DIRECTION('ref_axis',(0.,0.,-1.)) ;
#60628=DIRECTION('center_axis',(1.51760508056877E-16,5.60383084497428E-34,
-1.)) ;
#60629=DIRECTION('ref_axis',(0.707106781186544,-0.707106781186551,1.07310884363333E-16)) ;
#60630=DIRECTION('center_axis',(2.33146835171284E-14,-1.,3.53768783266021E-30)) ;
#60631=DIRECTION('ref_axis',(0.707106781186548,1.64859708161797E-14,-0.707106781186548)) ;
#60632=DIRECTION('',(2.33146835171284E-14,-1.,3.53768783266021E-30)) ;
#60633=DIRECTION('center_axis',(-1.4923676700635E-16,0.,1.)) ;
#60634=DIRECTION('ref_axis',(1.,0.,0.)) ;
#60635=DIRECTION('center_axis',(0.,-1.,0.)) ;
#60636=DIRECTION('ref_axis',(-1.,0.,0.)) ;
#60637=DIRECTION('center_axis',(-1.4923676700635E-16,0.,1.)) ;
#60638=DIRECTION('ref_axis',(1.,0.,1.4923676700635E-16)) ;
#60639=DIRECTION('center_axis',(-1.4923676700635E-16,0.,1.)) ;
#60640=DIRECTION('ref_axis',(1.,0.,1.4923676700635E-16)) ;
#60641=DIRECTION('center_axis',(1.4923676700635E-16,0.,-1.)) ;
#60642=DIRECTION('ref_axis',(1.,0.,1.4923676700635E-16)) ;
#60643=DIRECTION('center_axis',(1.4923676700635E-16,0.,-1.)) ;
#60644=DIRECTION('ref_axis',(-1.,0.,0.)) ;
#60645=DIRECTION('center_axis',(-1.4923676700635E-16,0.,1.)) ;
#60646=DIRECTION('ref_axis',(1.,0.,1.4923676700635E-16)) ;
#60647=DIRECTION('center_axis',(0.,1.,0.)) ;
#60648=DIRECTION('ref_axis',(1.,0.,0.)) ;
#60649=DIRECTION('center_axis',(-1.4923676700635E-16,0.,1.)) ;
#60650=DIRECTION('ref_axis',(1.,0.,1.4923676700635E-16)) ;
#60651=DIRECTION('center_axis',(0.,0.,-1.)) ;
#60652=DIRECTION('ref_axis',(1.,0.,0.)) ;
#60653=DIRECTION('center_axis',(0.,0.,-1.)) ;
#60654=DIRECTION('ref_axis',(1.,0.,0.)) ;
#60655=DIRECTION('',(0.,0.,-1.)) ;
#60656=DIRECTION('center_axis',(0.,0.,1.)) ;
#60657=DIRECTION('ref_axis',(1.,0.,0.)) ;
#60658=DIRECTION('center_axis',(0.,-1.,0.)) ;
#60659=DIRECTION('ref_axis',(-1.,0.,0.)) ;
#60660=DIRECTION('center_axis',(0.,0.,1.)) ;
#60661=DIRECTION('ref_axis',(1.,0.,0.)) ;
#60662=DIRECTION('center_axis',(0.,0.,1.)) ;
#60663=DIRECTION('ref_axis',(1.,0.,0.)) ;
#60664=DIRECTION('center_axis',(0.,0.,1.)) ;
#60665=DIRECTION('ref_axis',(1.,0.,0.)) ;
#60666=DIRECTION('center_axis',(0.,0.,-1.)) ;
#60667=DIRECTION('ref_axis',(1.,0.,0.)) ;
#60668=DIRECTION('center_axis',(0.,-1.,0.)) ;
#60669=DIRECTION('ref_axis',(-1.,0.,0.)) ;
#60670=DIRECTION('center_axis',(0.,0.,1.)) ;
#60671=DIRECTION('ref_axis',(1.,0.,0.)) ;
#60672=DIRECTION('center_axis',(0.,0.,1.)) ;
#60673=DIRECTION('ref_axis',(1.,0.,0.)) ;
#60674=DIRECTION('center_axis',(0.,0.,-1.)) ;
#60675=DIRECTION('ref_axis',(1.,0.,0.)) ;
#60676=DIRECTION('',(0.,0.,-1.)) ;
#60677=DIRECTION('center_axis',(-1.4923676700635E-16,0.,1.)) ;
#60678=DIRECTION('ref_axis',(1.,0.,1.4923676700635E-16)) ;
#60679=DIRECTION('center_axis',(-1.4923676700635E-16,0.,1.)) ;
#60680=DIRECTION('ref_axis',(1.,0.,1.4923676700635E-16)) ;
#60681=DIRECTION('center_axis',(1.4923676700635E-16,0.,-1.)) ;
#60682=DIRECTION('ref_axis',(-1.,0.,0.)) ;
#60683=DIRECTION('center_axis',(0.,1.,0.)) ;
#60684=DIRECTION('ref_axis',(1.,0.,0.)) ;
#60685=DIRECTION('center_axis',(1.4923676700635E-16,0.,-1.)) ;
#60686=DIRECTION('ref_axis',(1.,0.,1.4923676700635E-16)) ;
#60687=DIRECTION('center_axis',(-1.4923676700635E-16,0.,1.)) ;
#60688=DIRECTION('ref_axis',(1.,0.,1.4923676700635E-16)) ;
#60689=DIRECTION('center_axis',(-1.4923676700635E-16,0.,1.)) ;
#60690=DIRECTION('ref_axis',(1.,0.,1.4923676700635E-16)) ;
#60691=DIRECTION('center_axis',(-1.4923676700635E-16,0.,1.)) ;
#60692=DIRECTION('ref_axis',(1.,0.,0.)) ;
#60693=DIRECTION('center_axis',(1.4923676700635E-16,0.,-1.)) ;
#60694=DIRECTION('ref_axis',(1.,0.,1.4923676700635E-16)) ;
#60695=DIRECTION('center_axis',(0.,-1.,0.)) ;
#60696=DIRECTION('ref_axis',(-1.,0.,0.)) ;
#60697=DIRECTION('center_axis',(0.,0.,1.)) ;
#60698=DIRECTION('ref_axis',(1.,0.,0.)) ;
#60699=DIRECTION('center_axis',(-1.4923676700635E-16,0.,1.)) ;
#60700=DIRECTION('ref_axis',(1.,0.,1.4923676700635E-16)) ;
#60701=DIRECTION('',(0.,0.,1.)) ;
#60702=DIRECTION('center_axis',(0.,0.,1.)) ;
#60703=DIRECTION('ref_axis',(1.,0.,0.)) ;
#60704=DIRECTION('center_axis',(0.,0.,-1.)) ;
#60705=DIRECTION('ref_axis',(1.,0.,0.)) ;
#60706=DIRECTION('center_axis',(0.,-1.,0.)) ;
#60707=DIRECTION('ref_axis',(-1.,0.,0.)) ;
#60708=DIRECTION('center_axis',(0.,0.,1.)) ;
#60709=DIRECTION('ref_axis',(1.,0.,0.)) ;
#60710=DIRECTION('center_axis',(0.,0.,1.)) ;
#60711=DIRECTION('ref_axis',(1.,0.,0.)) ;
#60712=DIRECTION('center_axis',(0.,0.,-1.)) ;
#60713=DIRECTION('ref_axis',(1.,0.,0.)) ;
#60714=DIRECTION('',(0.,0.,-1.)) ;
#60715=DIRECTION('center_axis',(-1.4923676700635E-16,0.,1.)) ;
#60716=DIRECTION('ref_axis',(1.,0.,1.4923676700635E-16)) ;
#60717=DIRECTION('center_axis',(-1.4923676700635E-16,0.,1.)) ;
#60718=DIRECTION('ref_axis',(1.,0.,1.4923676700635E-16)) ;
#60719=DIRECTION('center_axis',(-1.4923676700635E-16,0.,1.)) ;
#60720=DIRECTION('ref_axis',(1.,0.,0.)) ;
#60721=DIRECTION('center_axis',(0.,-1.,0.)) ;
#60722=DIRECTION('ref_axis',(-1.,0.,0.)) ;
#60723=DIRECTION('center_axis',(-1.4923676700635E-16,0.,1.)) ;
#60724=DIRECTION('ref_axis',(1.,0.,1.4923676700635E-16)) ;
#60725=DIRECTION('center_axis',(-1.4923676700635E-16,0.,1.)) ;
#60726=DIRECTION('ref_axis',(1.,0.,1.4923676700635E-16)) ;
#60727=DIRECTION('center_axis',(1.4923676700635E-16,0.,-1.)) ;
#60728=DIRECTION('ref_axis',(1.,0.,1.4923676700635E-16)) ;
#60729=DIRECTION('center_axis',(1.4923676700635E-16,0.,-1.)) ;
#60730=DIRECTION('ref_axis',(-1.,0.,0.)) ;
#60731=DIRECTION('center_axis',(0.,1.,0.)) ;
#60732=DIRECTION('ref_axis',(1.,0.,0.)) ;
#60733=DIRECTION('center_axis',(-1.4923676700635E-16,0.,1.)) ;
#60734=DIRECTION('ref_axis',(-1.,0.,0.)) ;
#60735=DIRECTION('center_axis',(0.,1.,0.)) ;
#60736=DIRECTION('ref_axis',(1.,0.,0.)) ;
#60737=DIRECTION('center_axis',(-1.4923676700635E-16,0.,1.)) ;
#60738=DIRECTION('ref_axis',(-1.,0.,0.)) ;
#60739=DIRECTION('center_axis',(0.,1.,0.)) ;
#60740=DIRECTION('ref_axis',(1.,0.,0.)) ;
#60741=DIRECTION('center_axis',(-1.4923676700635E-16,0.,1.)) ;
#60742=DIRECTION('ref_axis',(-1.,0.,0.)) ;
#60743=DIRECTION('center_axis',(0.,1.,0.)) ;
#60744=DIRECTION('ref_axis',(1.,0.,0.)) ;
#60745=DIRECTION('center_axis',(-1.4923676700635E-16,0.,1.)) ;
#60746=DIRECTION('ref_axis',(1.,0.,1.4923676700635E-16)) ;
#60747=DIRECTION('center_axis',(-2.01858731750028E-16,0.,1.)) ;
#60748=DIRECTION('ref_axis',(0.707106781186579,-0.707106781186516,1.42735678062167E-16)) ;
#60749=DIRECTION('',(2.01858731750028E-16,0.,-1.)) ;
#60750=DIRECTION('',(-2.01858731750028E-16,0.,1.)) ;
#60751=DIRECTION('center_axis',(0.,-1.,0.)) ;
#60752=DIRECTION('ref_axis',(1.,0.,2.24978329294248E-16)) ;
#60753=DIRECTION('',(0.,0.,1.)) ;
#60754=DIRECTION('center_axis',(0.,0.,1.)) ;
#60755=DIRECTION('ref_axis',(-0.707106781186574,-0.707106781186521,0.)) ;
#60756=DIRECTION('center_axis',(0.707106781186551,0.707106781186544,0.)) ;
#60757=DIRECTION('ref_axis',(0.,0.,-1.)) ;
#60758=DIRECTION('center_axis',(-1.,3.73034936274055E-14,0.)) ;
#60759=DIRECTION('ref_axis',(-3.73034936274055E-14,-1.,-5.56705278699598E-30)) ;
#60760=DIRECTION('center_axis',(0.707106781186532,-0.707106781186563,0.)) ;
#60761=DIRECTION('ref_axis',(0.,0.,-1.)) ;
#60762=DIRECTION('center_axis',(0.,1.,0.)) ;
#60763=DIRECTION('ref_axis',(-1.,0.,-1.4923676700635E-16)) ;
#60764=DIRECTION('center_axis',(0.,1.,0.)) ;
#60765=DIRECTION('ref_axis',(-1.,0.,-1.4923676700635E-16)) ;
#60766=DIRECTION('center_axis',(0.863778900898434,-0.503871025524085,0.)) ;
#60767=DIRECTION('ref_axis',(0.503871025524085,0.863778900898434,0.)) ;
#60768=DIRECTION('center_axis',(-0.503871025524087,0.863778900898433,0.)) ;
#60769=DIRECTION('ref_axis',(0.863778900898433,0.503871025524087,0.)) ;
#60770=DIRECTION('center_axis',(0.,0.,1.)) ;
#60771=DIRECTION('ref_axis',(1.,0.,0.)) ;
#60772=DIRECTION('center_axis',(0.503871025524087,0.863778900898433,0.)) ;
#60773=DIRECTION('ref_axis',(-0.863778900898433,0.503871025524087,0.)) ;
#60774=DIRECTION('center_axis',(0.503871025524087,0.863778900898433,0.)) ;
#60775=DIRECTION('ref_axis',(-0.863778900898433,0.503871025524087,0.)) ;
#60776=DIRECTION('center_axis',(-0.863778900898434,-0.503871025524085,0.)) ;
#60777=DIRECTION('ref_axis',(-0.503871025524085,0.863778900898434,0.)) ;
#60778=DIRECTION('center_axis',(-0.863778900898434,-0.503871025524085,0.)) ;
#60779=DIRECTION('ref_axis',(-0.503871025524085,0.863778900898434,0.)) ;
#60780=DIRECTION('center_axis',(-8.88178419700128E-15,8.88178419700113E-15,
1.)) ;
#60781=DIRECTION('ref_axis',(0.,1.,-8.88178419700113E-15)) ;
#60782=DIRECTION('center_axis',(0.863778900898434,-0.503871025524085,0.)) ;
#60783=DIRECTION('ref_axis',(0.503871025524085,0.863778900898434,0.)) ;
#60784=DIRECTION('center_axis',(0.863778900898434,-0.503871025524085,0.)) ;
#60785=DIRECTION('ref_axis',(0.503871025524085,0.863778900898434,0.)) ;
#60786=DIRECTION('center_axis',(-0.503871025524087,0.863778900898433,0.)) ;
#60787=DIRECTION('ref_axis',(0.863778900898433,0.503871025524087,0.)) ;
#60788=DIRECTION('center_axis',(-0.503871025524087,0.863778900898433,0.)) ;
#60789=DIRECTION('ref_axis',(0.863778900898433,0.503871025524087,0.)) ;
#60790=DIRECTION('center_axis',(0.,0.,1.)) ;
#60791=DIRECTION('ref_axis',(1.,0.,0.)) ;
#60792=DIRECTION('center_axis',(0.503871025524087,0.863778900898433,0.)) ;
#60793=DIRECTION('ref_axis',(-0.863778900898433,0.503871025524087,0.)) ;
#60794=DIRECTION('center_axis',(0.503871025524087,0.863778900898433,0.)) ;
#60795=DIRECTION('ref_axis',(-0.863778900898433,0.503871025524087,0.)) ;
#60796=DIRECTION('center_axis',(0.,-8.88178419700113E-15,1.)) ;
#60797=DIRECTION('ref_axis',(0.,1.,8.88178419700113E-15)) ;
#60798=DIRECTION('center_axis',(0.,-1.,-5.60383084497428E-34)) ;
#60799=DIRECTION('ref_axis',(-0.707106781186545,-3.96250679110367E-34,0.70710678118655)) ;
#60800=DIRECTION('',(0.,-1.,-5.60383084497428E-34)) ;
#60801=DIRECTION('center_axis',(0.,1.,0.)) ;
#60802=DIRECTION('ref_axis',(-1.,0.,0.)) ;
#60803=DIRECTION('center_axis',(1.,0.,0.)) ;
#60804=DIRECTION('ref_axis',(0.,0.97854978498675,0.206010481049835)) ;
#60805=DIRECTION('center_axis',(0.,-0.402044149173841,-0.915620282712808)) ;
#60806=DIRECTION('ref_axis',(0.,-0.915620282712808,0.402044149173841)) ;
#60807=DIRECTION('center_axis',(-1.,3.19495806435525E-17,-1.51760508056877E-16)) ;
#60808=DIRECTION('ref_axis',(-9.77165742124407E-17,0.630075201444312,0.77653412064436)) ;
#60809=DIRECTION('center_axis',(1.,0.,0.)) ;
#60810=DIRECTION('ref_axis',(0.,0.97854978498675,0.206010481049835)) ;
#60811=DIRECTION('center_axis',(0.,-1.,0.)) ;
#60812=DIRECTION('ref_axis',(1.,0.,7.40148683083442E-15)) ;
#60813=DIRECTION('center_axis',(0.,-0.402044149173841,-0.915620282712808)) ;
#60814=DIRECTION('ref_axis',(0.,-0.915620282712808,0.402044149173841)) ;
#60815=DIRECTION('center_axis',(0.,1.,5.60383084497428E-34)) ;
#60816=DIRECTION('ref_axis',(0.707106781186545,-3.96250679110367E-34,0.70710678118655)) ;
#60817=DIRECTION('',(0.,1.,5.60383084497428E-34)) ;
#60818=DIRECTION('center_axis',(-1.,0.,-1.51760508056877E-16)) ;
#60819=DIRECTION('ref_axis',(-1.07310884363335E-16,0.70710678118654,0.707106781186555)) ;
#60820=DIRECTION('center_axis',(0.,-1.,-5.60383084497428E-34)) ;
#60821=DIRECTION('ref_axis',(-0.70710678118655,-3.96250679110364E-34,0.707106781186545)) ;
#60822=DIRECTION('',(0.,-1.,-5.60383084497428E-34)) ;
#60823=DIRECTION('center_axis',(0.,1.,0.)) ;
#60824=DIRECTION('ref_axis',(-1.,0.,0.)) ;
#60825=DIRECTION('center_axis',(1.,0.,0.)) ;
#60826=DIRECTION('ref_axis',(0.,0.978549784986751,0.206010481049832)) ;
#60827=DIRECTION('center_axis',(0.,-0.402044149173841,-0.915620282712808)) ;
#60828=DIRECTION('ref_axis',(0.,-0.915620282712808,0.402044149173841)) ;
#60829=DIRECTION('center_axis',(-1.,3.19495806435525E-17,-1.51760508056877E-16)) ;
#60830=DIRECTION('ref_axis',(-9.7716574212441E-17,0.63007520144431,0.776534120644362)) ;
#60831=DIRECTION('center_axis',(1.,0.,0.)) ;
#60832=DIRECTION('ref_axis',(0.,0.978549784986751,0.206010481049832)) ;
#60833=DIRECTION('center_axis',(0.,-1.,0.)) ;
#60834=DIRECTION('ref_axis',(1.,0.,3.70074341541719E-15)) ;
#60835=DIRECTION('center_axis',(0.,-0.402044149173847,-0.915620282712805)) ;
#60836=DIRECTION('ref_axis',(0.,-0.915620282712805,0.402044149173847)) ;
#60837=DIRECTION('center_axis',(0.,1.,5.60383084497428E-34)) ;
#60838=DIRECTION('ref_axis',(0.707106781186547,-3.96250679110365E-34,0.707106781186547)) ;
#60839=DIRECTION('',(0.,1.,5.60383084497428E-34)) ;
#60840=DIRECTION('center_axis',(-1.,0.,-1.51760508056877E-16)) ;
#60841=DIRECTION('ref_axis',(-1.07310884363335E-16,0.70710678118654,0.707106781186555)) ;
#60842=DIRECTION('center_axis',(0.,0.206010481049838,-0.97854978498675)) ;
#60843=DIRECTION('ref_axis',(-0.707106781186557,-0.691939188692759,-0.145671408145841)) ;
#60844=DIRECTION('center_axis',(0.,0.206010481049834,-0.978549784986751)) ;
#60845=DIRECTION('ref_axis',(0.,-0.978549784986751,-0.206010481049834)) ;
#60846=DIRECTION('',(0.,-0.206010481049838,0.97854978498675)) ;
#60847=DIRECTION('center_axis',(0.,-0.206010481049838,0.97854978498675)) ;
#60848=DIRECTION('ref_axis',(0.707106781186556,-0.691939188692761,-0.145671408145841)) ;
#60849=DIRECTION('',(0.,0.206010481049838,-0.97854978498675)) ;
#60850=DIRECTION('center_axis',(0.,0.206010481049843,-0.978549784986749)) ;
#60851=DIRECTION('ref_axis',(1.,0.,0.)) ;
#60852=DIRECTION('center_axis',(-1.,0.,0.)) ;
#60853=DIRECTION('ref_axis',(0.,-1.,0.)) ;
#60854=DIRECTION('',(0.,0.,1.)) ;
#60855=DIRECTION('center_axis',(0.,0.,1.)) ;
#60856=DIRECTION('ref_axis',(-0.707106781186523,0.707106781186573,0.)) ;
#60857=DIRECTION('center_axis',(0.,-0.994505452921406,-0.104684784518042)) ;
#60858=DIRECTION('ref_axis',(0.,0.104684784518042,-0.994505452921406)) ;
#60859=DIRECTION('center_axis',(0.,0.,1.)) ;
#60860=DIRECTION('ref_axis',(0.707106781186523,0.707106781186573,0.)) ;
#60861=DIRECTION('',(0.,0.,-1.)) ;
#60862=DIRECTION('center_axis',(0.,-0.994505452921406,-0.104684784518042)) ;
#60863=DIRECTION('ref_axis',(0.,0.104684784518042,-0.994505452921406)) ;
#60864=DIRECTION('center_axis',(1.,0.,0.)) ;
#60865=DIRECTION('ref_axis',(0.,1.,0.)) ;
#60866=DIRECTION('',(0.,-0.206010481049838,0.97854978498675)) ;
#60867=DIRECTION('center_axis',(0.,0.206010481049838,-0.97854978498675)) ;
#60868=DIRECTION('ref_axis',(-0.707106781186556,-0.691939188692761,-0.145671408145841)) ;
#60869=DIRECTION('center_axis',(0.,0.206010481049834,-0.978549784986751)) ;
#60870=DIRECTION('ref_axis',(0.,-0.978549784986751,-0.206010481049834)) ;
#60871=DIRECTION('center_axis',(0.,-0.206010481049838,0.97854978498675)) ;
#60872=DIRECTION('ref_axis',(0.707106781186543,-0.691939188692773,-0.145671408145844)) ;
#60873=DIRECTION('',(0.,0.206010481049838,-0.97854978498675)) ;
#60874=DIRECTION('center_axis',(0.,0.206010481049843,-0.978549784986749)) ;
#60875=DIRECTION('ref_axis',(1.,0.,0.)) ;
#60876=DIRECTION('center_axis',(-1.,0.,0.)) ;
#60877=DIRECTION('ref_axis',(0.,-1.,0.)) ;
#60878=DIRECTION('',(0.,0.,1.)) ;
#60879=DIRECTION('center_axis',(0.,0.,1.)) ;
#60880=DIRECTION('ref_axis',(-0.70710678118651,0.707106781186585,0.)) ;
#60881=DIRECTION('center_axis',(0.,-0.994505452921406,-0.104684784518042)) ;
#60882=DIRECTION('ref_axis',(0.,0.104684784518042,-0.994505452921406)) ;
#60883=DIRECTION('center_axis',(0.,-1.,0.)) ;
#60884=DIRECTION('ref_axis',(1.,0.,1.4923676700635E-16)) ;
#60885=DIRECTION('',(0.,0.,1.)) ;
#60886=DIRECTION('',(-1.,0.,-1.4923676700635E-16)) ;
#60887=DIRECTION('center_axis',(-1.,0.,0.)) ;
#60888=DIRECTION('ref_axis',(0.,-1.,0.)) ;
#60889=DIRECTION('',(0.,1.,0.)) ;
#60890=DIRECTION('center_axis',(-1.4923676700635E-16,0.,1.)) ;
#60891=DIRECTION('ref_axis',(1.,0.,1.4923676700635E-16)) ;
#60892=DIRECTION('center_axis',(3.55271367880051E-14,-1.,0.)) ;
#60893=DIRECTION('ref_axis',(1.,3.55271367880051E-14,1.4923676700635E-16)) ;
#60894=DIRECTION('',(-2.01858731750028E-16,-7.1714627747365E-30,1.)) ;
#60895=DIRECTION('',(0.,0.,1.)) ;
#60896=DIRECTION('center_axis',(-1.,0.,0.)) ;
#60897=DIRECTION('ref_axis',(0.,-1.,0.)) ;
#60898=DIRECTION('center_axis',(-1.,0.,-2.01858731750028E-16)) ;
#60899=DIRECTION('ref_axis',(0.,-1.,0.)) ;
#60900=DIRECTION('center_axis',(0.,1.,0.)) ;
#60901=DIRECTION('ref_axis',(-1.,0.,-1.4923676700635E-16)) ;
#60902=DIRECTION('',(0.,0.,1.)) ;
#60903=DIRECTION('',(0.,0.,1.)) ;
#60904=DIRECTION('center_axis',(1.,-7.105427357601E-15,0.)) ;
#60905=DIRECTION('ref_axis',(7.105427357601E-15,1.,1.06039100704685E-30)) ;
#60906=DIRECTION('center_axis',(1.,-7.105427357601E-15,0.)) ;
#60907=DIRECTION('ref_axis',(7.105427357601E-15,1.,1.06039100704685E-30)) ;
#60908=DIRECTION('center_axis',(0.,1.,0.)) ;
#60909=DIRECTION('ref_axis',(-1.,0.,-1.4923676700635E-16)) ;
#60910=DIRECTION('',(0.,0.,1.)) ;
#60911=DIRECTION('center_axis',(1.,-3.17206578464323E-15,0.)) ;
#60912=DIRECTION('ref_axis',(3.17206578464323E-15,1.,4.73388842431617E-31)) ;
#60913=DIRECTION('center_axis',(0.,1.,0.)) ;
#60914=DIRECTION('ref_axis',(-1.,0.,-1.4923676700635E-16)) ;
#60915=DIRECTION('center_axis',(-1.,0.,0.)) ;
#60916=DIRECTION('ref_axis',(0.,-1.,0.)) ;
#60917=DIRECTION('center_axis',(1.,0.,0.)) ;
#60918=DIRECTION('ref_axis',(0.,1.,0.)) ;
#60919=DIRECTION('center_axis',(0.,1.,0.)) ;
#60920=DIRECTION('ref_axis',(-1.,0.,-1.4923676700635E-16)) ;
#60921=DIRECTION('center_axis',(0.,1.,0.)) ;
#60922=DIRECTION('ref_axis',(-1.,0.,-1.4923676700635E-16)) ;
#60923=DIRECTION('center_axis',(-1.,-2.33146835171284E-14,-2.01858731750028E-16)) ;
#60924=DIRECTION('ref_axis',(2.33146835171284E-14,-1.,3.47940799187248E-30)) ;
#60925=DIRECTION('center_axis',(0.,0.206010481049838,-0.97854978498675)) ;
#60926=DIRECTION('ref_axis',(-0.707106781186557,-0.691939188692759,-0.145671408145841)) ;
#60927=DIRECTION('center_axis',(0.,0.206010481049838,-0.97854978498675)) ;
#60928=DIRECTION('ref_axis',(-0.707106781186556,-0.691939188692761,-0.145671408145841)) ;
#60929=DIRECTION('',(0.,-0.206010481049838,0.97854978498675)) ;
#60930=DIRECTION('center_axis',(0.,-0.206010481049838,0.97854978498675)) ;
#60931=DIRECTION('ref_axis',(0.707106781186556,-0.691939188692761,-0.145671408145841)) ;
#60932=DIRECTION('',(0.,0.206010481049838,-0.97854978498675)) ;
#60933=DIRECTION('center_axis',(1.,0.,0.)) ;
#60934=DIRECTION('ref_axis',(0.,1.,0.)) ;
#60935=DIRECTION('center_axis',(-1.,0.,0.)) ;
#60936=DIRECTION('ref_axis',(0.,-1.,0.)) ;
#60937=DIRECTION('center_axis',(0.,-0.994505452921406,-0.104684784518042)) ;
#60938=DIRECTION('ref_axis',(0.,0.104684784518042,-0.994505452921406)) ;
#60939=DIRECTION('center_axis',(0.,0.,1.)) ;
#60940=DIRECTION('ref_axis',(0.707106781186523,0.707106781186573,0.)) ;
#60941=DIRECTION('',(0.,0.,-1.)) ;
#60942=DIRECTION('center_axis',(1.,0.,0.)) ;
#60943=DIRECTION('ref_axis',(0.,1.,0.)) ;
#79197=CARTESIAN_POINT('',(0.,0.,0.)) ;
#79198=CARTESIAN_POINT('Ctrl Pts',(49.8966187896629,247.701952531225,31.7413203435596)) ;
#79199=CARTESIAN_POINT('Ctrl Pts',(49.8969225423282,247.6986843043,31.7413203435596)) ;
#79200=CARTESIAN_POINT('Ctrl Pts',(49.8972304579647,247.69541527565,31.7413203435597)) ;
#79201=CARTESIAN_POINT('Ctrl Pts',(49.9067236558174,247.591181597776,31.7413203435597)) ;
#79202=CARTESIAN_POINT('Ctrl Pts',(49.9177374288024,247.504008411497,31.7413203435597)) ;
#79203=CARTESIAN_POINT('Ctrl Pts',(49.9804256035652,247.364244651485,31.7413203435597)) ;
#79204=CARTESIAN_POINT('Ctrl Pts',(50.0370077354619,247.298814470324,31.7413203435597)) ;
#79205=CARTESIAN_POINT('Ctrl Pts',(50.1086106021864,247.221561922593,31.7413203435597)) ;
#79206=CARTESIAN_POINT('Ctrl Pts',(50.1123189230203,247.217536513008,31.7413203435596)) ;
#79207=CARTESIAN_POINT('Ctrl Pts',(50.1160311831359,247.213516656002,31.7413203435596)) ;
#79208=CARTESIAN_POINT('Ctrl Pts',(49.8966187896629,247.701952531225,31.7054164275186)) ;
#79209=CARTESIAN_POINT('Ctrl Pts',(49.8969225423282,247.6986843043,31.7054164275186)) ;
#79210=CARTESIAN_POINT('Ctrl Pts',(49.8972304579647,247.69541527565,31.7054164275186)) ;
#79211=CARTESIAN_POINT('Ctrl Pts',(49.9067236558174,247.591181597776,31.7054164275186)) ;
#79212=CARTESIAN_POINT('Ctrl Pts',(49.9177374288024,247.504008411497,31.7054164275186)) ;
#79213=CARTESIAN_POINT('Ctrl Pts',(49.9804256035652,247.364244651485,31.7054164275186)) ;
#79214=CARTESIAN_POINT('Ctrl Pts',(50.0370077354619,247.298814470324,31.7054164275186)) ;
#79215=CARTESIAN_POINT('Ctrl Pts',(50.1086106021864,247.221561922593,31.7054164275186)) ;
#79216=CARTESIAN_POINT('Ctrl Pts',(50.1123189230203,247.217536513008,31.7054164275186)) ;
#79217=CARTESIAN_POINT('Ctrl Pts',(50.1160311831359,247.213516656002,31.7054164275186)) ;
#79218=CARTESIAN_POINT('Ctrl Pts',(49.8665894217931,247.699161568194,31.6432842907294)) ;
#79219=CARTESIAN_POINT('Ctrl Pts',(49.8668865433394,247.69588922041,31.6432842907294)) ;
#79220=CARTESIAN_POINT('Ctrl Pts',(49.8672076246043,247.692627717528,31.6432842907294)) ;
#79221=CARTESIAN_POINT('Ctrl Pts',(49.876579092001,247.588366078285,31.6432842907294)) ;
#79222=CARTESIAN_POINT('Ctrl Pts',(49.8877086829376,247.497236411322,31.6432842907294)) ;
#79223=CARTESIAN_POINT('Ctrl Pts',(49.9553609719887,247.346407965604,31.6432842907294)) ;
#79224=CARTESIAN_POINT('Ctrl Pts',(50.0147608319875,247.278282429423,31.6432842907294)) ;
#79225=CARTESIAN_POINT('Ctrl Pts',(50.0864627823533,247.201105202407,31.6432842907294)) ;
#79226=CARTESIAN_POINT('Ctrl Pts',(50.0901533731766,247.197072101885,31.6432842907294)) ;
#79227=CARTESIAN_POINT('Ctrl Pts',(50.0938748615201,247.193055721962,31.6432842907294)) ;
#79228=CARTESIAN_POINT('Ctrl Pts',(49.8039461216876,247.693339429828,31.6213203435596)) ;
#79229=CARTESIAN_POINT('Ctrl Pts',(49.8042459616924,247.69006877141,31.6213203435596)) ;
#79230=CARTESIAN_POINT('Ctrl Pts',(49.8045604603195,247.686803113285,31.6213203435596)) ;
#79231=CARTESIAN_POINT('Ctrl Pts',(49.8140384370984,247.582601988406,31.6213203435596)) ;
#79232=CARTESIAN_POINT('Ctrl Pts',(49.8250164956597,247.48333041954,31.6213203435596)) ;
#79233=CARTESIAN_POINT('Ctrl Pts',(49.903198192551,247.309016626601,31.6213203435597)) ;
#79234=CARTESIAN_POINT('Ctrl Pts',(49.9686480743411,247.235639578897,31.6213203435596)) ;
#79235=CARTESIAN_POINT('Ctrl Pts',(50.0402371297429,247.158420268992,31.6213203435597)) ;
#79236=CARTESIAN_POINT('Ctrl Pts',(50.0439375652229,247.154390629808,31.6213203435596)) ;
#79237=CARTESIAN_POINT('Ctrl Pts',(50.0476552704109,247.15037282444,31.6213203435596)) ;
#79238=CARTESIAN_POINT('Ctrl Pts',(49.777133739023,247.690847456999,31.6213203435596)) ;
#79239=CARTESIAN_POINT('Ctrl Pts',(49.7774374916883,247.687579230074,31.6213203435596)) ;
#79240=CARTESIAN_POINT('Ctrl Pts',(49.7777435177816,247.684308495694,31.6213203435596)) ;
#79241=CARTESIAN_POINT('Ctrl Pts',(49.7873269510022,247.580153011363,31.6213203435596)) ;
#79242=CARTESIAN_POINT('Ctrl Pts',(49.7981748530167,247.477415105803,31.6213203435596)) ;
#79243=CARTESIAN_POINT('Ctrl Pts',(49.8808922016941,247.292982144188,31.6213203435597)) ;
#79244=CARTESIAN_POINT('Ctrl Pts',(49.9489601708937,247.21741901313,31.6213203435596)) ;
#79245=CARTESIAN_POINT('Ctrl Pts',(50.0204478229115,247.14014860368,31.6213203435597)) ;
#79246=CARTESIAN_POINT('Ctrl Pts',(50.0241602504257,247.136123685724,31.6213203435596)) ;
#79247=CARTESIAN_POINT('Ctrl Pts',(50.0278725105414,247.132103828718,31.6213203435596)) ;
#79248=CARTESIAN_POINT('',(49.777133739023,247.690847456999,31.6213203435596)) ;
#79249=CARTESIAN_POINT('',(50.0278725105413,247.132103828718,31.6213203435596)) ;
#79250=CARTESIAN_POINT('Ctrl Pts',(49.777133739023,247.690847456999,31.6213203435596)) ;
#79251=CARTESIAN_POINT('Ctrl Pts',(49.7774374916883,247.687579230074,31.6213203435596)) ;
#79252=CARTESIAN_POINT('Ctrl Pts',(49.7777435177816,247.684308495694,31.6213203435596)) ;
#79253=CARTESIAN_POINT('Ctrl Pts',(49.7873269510022,247.580153011363,31.6213203435596)) ;
#79254=CARTESIAN_POINT('Ctrl Pts',(49.7981748530167,247.477415105803,31.6213203435596)) ;
#79255=CARTESIAN_POINT('Ctrl Pts',(49.8808922016941,247.292982144188,31.6213203435597)) ;
#79256=CARTESIAN_POINT('Ctrl Pts',(49.9489601708937,247.21741901313,31.6213203435596)) ;
#79257=CARTESIAN_POINT('Ctrl Pts',(50.0204478229115,247.14014860368,31.6213203435597)) ;
#79258=CARTESIAN_POINT('Ctrl Pts',(50.0241602504257,247.136123685724,31.6213203435596)) ;
#79259=CARTESIAN_POINT('Ctrl Pts',(50.0278725105414,247.132103828718,31.6213203435596)) ;
#79260=CARTESIAN_POINT('',(50.1048949947523,247.225574360848,31.7413203435596)) ;
#79261=CARTESIAN_POINT('Ctrl Pts',(50.0278725105414,247.132103828718,31.6213203435596)) ;
#79262=CARTESIAN_POINT('Ctrl Pts',(50.0280595512392,247.132330804138,31.6213203435596)) ;
#79263=CARTESIAN_POINT('Ctrl Pts',(50.0282465911107,247.132557779856,31.6213214458748)) ;
#79264=CARTESIAN_POINT('Ctrl Pts',(50.038504940272,247.145006504587,31.6214422185109)) ;
#79265=CARTESIAN_POINT('Ctrl Pts',(50.0485724477496,247.15722379173,31.6247500298547)) ;
#79266=CARTESIAN_POINT('Ctrl Pts',(50.0656603915231,247.177955014042,31.6359582847072)) ;
#79267=CARTESIAN_POINT('Ctrl Pts',(50.0742393969475,247.18836221985,31.6438392648492)) ;
#79268=CARTESIAN_POINT('Ctrl Pts',(50.0891026914623,247.206401264955,31.6671840249628)) ;
#79269=CARTESIAN_POINT('Ctrl Pts',(50.0946683323572,247.213159727899,31.6801574547695)) ;
#79270=CARTESIAN_POINT('Ctrl Pts',(50.1006035968679,247.220368116857,31.7016634476284)) ;
#79271=CARTESIAN_POINT('Ctrl Pts',(50.1021875059769,247.22229201451,31.7093904709062)) ;
#79272=CARTESIAN_POINT('Ctrl Pts',(50.1043315944804,247.224896338963,31.7251872827606)) ;
#79273=CARTESIAN_POINT('Ctrl Pts',(50.1048906386302,247.225575402442,31.7332454904375)) ;
#79274=CARTESIAN_POINT('Ctrl Pts',(50.1048906386303,247.225575402442,31.7413203435596)) ;
#79275=CARTESIAN_POINT('',(49.8975295575751,247.692147713814,31.7413203435596)) ;
#79276=CARTESIAN_POINT('Ctrl Pts',(50.1048956053956,247.225574924765,31.7413203435597)) ;
#79277=CARTESIAN_POINT('Ctrl Pts',(50.092755916046,247.23872050556,31.7413203435597)) ;
#79278=CARTESIAN_POINT('Ctrl Pts',(50.0808929246769,247.251573001433,31.7413203435597)) ;
#79279=CARTESIAN_POINT('Ctrl Pts',(50.0694690210685,247.264236937633,31.7413203435597)) ;
#79280=CARTESIAN_POINT('Ctrl Pts',(50.0573611518781,247.277659081954,31.7413203435597)) ;
#79281=CARTESIAN_POINT('Ctrl Pts',(50.0457460902749,247.290869219247,31.7413203435597)) ;
#79282=CARTESIAN_POINT('Ctrl Pts',(50.0347633830109,247.303967779101,31.7413203435597)) ;
#79283=CARTESIAN_POINT('Ctrl Pts',(50.0225934949892,247.318482233765,31.7413203435597)) ;
#79284=CARTESIAN_POINT('Ctrl Pts',(50.0111997909391,247.332859565364,31.7413203435597)) ;
#79285=CARTESIAN_POINT('Ctrl Pts',(50.0007131697972,247.347210090936,31.7413203435597)) ;
#79286=CARTESIAN_POINT('Ctrl Pts',(49.9892528408923,247.362893097005,31.7413203435597)) ;
#79287=CARTESIAN_POINT('Ctrl Pts',(49.9788750866055,247.378543740406,31.7413203435597)) ;
#79288=CARTESIAN_POINT('Ctrl Pts',(49.9696925368555,247.39428001492,31.7413203435597)) ;
#79289=CARTESIAN_POINT('Ctrl Pts',(49.962085283186,247.407316680693,31.7413203435597)) ;
#79290=CARTESIAN_POINT('Ctrl Pts',(49.9552968604527,247.420411462331,31.7413203435597)) ;
#79291=CARTESIAN_POINT('Ctrl Pts',(49.9493716598566,247.433622676736,31.7413203435597)) ;
#79292=CARTESIAN_POINT('Ctrl Pts',(49.9485345864462,247.435489070306,31.7413203435597)) ;
#79293=CARTESIAN_POINT('Ctrl Pts',(49.947710735811,247.437366665178,31.7413203435597)) ;
#79294=CARTESIAN_POINT('Ctrl Pts',(49.9468999191231,247.439255484219,31.7413203435597)) ;
#79295=CARTESIAN_POINT('Ctrl Pts',(49.9394567849731,247.456594463195,31.7413203435597)) ;
#79296=CARTESIAN_POINT('Ctrl Pts',(49.9331153249188,247.474880671756,31.7413203435597)) ;
#79297=CARTESIAN_POINT('Ctrl Pts',(49.9277105050193,247.494120607347,31.7413203435597)) ;
#79298=CARTESIAN_POINT('Ctrl Pts',(49.9230312826354,247.510777580003,31.7413203435597)) ;
#79299=CARTESIAN_POINT('Ctrl Pts',(49.9190545065783,247.528149577348,31.7413203435597)) ;
#79300=CARTESIAN_POINT('Ctrl Pts',(49.9156386352171,247.546225434154,31.7413203435597)) ;
#79301=CARTESIAN_POINT('Ctrl Pts',(49.9124482520327,247.563108069212,31.7413203435597)) ;
#79302=CARTESIAN_POINT('Ctrl Pts',(49.9097477074761,247.580604946861,31.7413203435597)) ;
#79303=CARTESIAN_POINT('Ctrl Pts',(49.9073825196643,247.598689486076,31.7413203435597)) ;
#79304=CARTESIAN_POINT('Ctrl Pts',(49.9052155686072,247.615258280814,31.7413203435597)) ;
#79305=CARTESIAN_POINT('Ctrl Pts',(49.9033303248592,247.632320450204,31.7413203435597)) ;
#79306=CARTESIAN_POINT('Ctrl Pts',(49.9015691997015,247.649838235728,31.7413203435597)) ;
#79307=CARTESIAN_POINT('Ctrl Pts',(49.9001789372978,247.66366707606,31.7413203435597)) ;
#79308=CARTESIAN_POINT('Ctrl Pts',(49.8988654497563,247.677779591041,31.7413203435597)) ;
#79309=CARTESIAN_POINT('Ctrl Pts',(49.897530056052,247.692147760143,31.7413203435597)) ;
#79310=CARTESIAN_POINT('Ctrl Pts',(49.777133739023,247.690847456999,31.6213203435596)) ;
#79311=CARTESIAN_POINT('Ctrl Pts',(49.7774262573671,247.690850619957,31.6213203435596)) ;
#79312=CARTESIAN_POINT('Ctrl Pts',(49.7777187754276,247.690853779499,31.6213214470556)) ;
#79313=CARTESIAN_POINT('Ctrl Pts',(49.7938052827997,247.691027362574,31.6214426730848)) ;
#79314=CARTESIAN_POINT('Ctrl Pts',(49.8095865790889,247.691194286689,31.6247713732388)) ;
#79315=CARTESIAN_POINT('Ctrl Pts',(49.8363324427948,247.691489707221,31.6360317764872)) ;
#79316=CARTESIAN_POINT('Ctrl Pts',(49.8497322009203,247.691640499545,31.6439353156995)) ;
#79317=CARTESIAN_POINT('Ctrl Pts',(49.8729530816466,247.691892838565,31.6673317964462)) ;
#79318=CARTESIAN_POINT('Ctrl Pts',(49.8816380976473,247.69198301369,31.6803265126481)) ;
#79319=CARTESIAN_POINT('Ctrl Pts',(49.8908743054425,247.69207751469,31.7018134432135)) ;
#79320=CARTESIAN_POINT('Ctrl Pts',(49.8933328310453,247.692102380517,31.7095135527032)) ;
#79321=CARTESIAN_POINT('Ctrl Pts',(49.8966608708735,247.692136012753,31.7252506528064)) ;
#79322=CARTESIAN_POINT('Ctrl Pts',(49.8975283263115,247.692144732519,31.7332777489016)) ;
#79323=CARTESIAN_POINT('Ctrl Pts',(49.8975283263115,247.692144732519,31.7413203435596)) ;
#79324=CARTESIAN_POINT('Ctrl Pts',(50.8831605335109,248.366098818484,31.7413203435596)) ;
#79325=CARTESIAN_POINT('Ctrl Pts',(50.7693177137058,248.364889140804,31.7413203435596)) ;
#79326=CARTESIAN_POINT('Ctrl Pts',(50.6611870949586,248.363142107183,31.7413203435596)) ;
#79327=CARTESIAN_POINT('Ctrl Pts',(50.48051672475,248.335752825127,31.7413203435596)) ;
#79328=CARTESIAN_POINT('Ctrl Pts',(50.3998763353304,248.314886646393,31.7413203435596)) ;
#79329=CARTESIAN_POINT('Ctrl Pts',(50.31189617328,248.291603218974,31.7413203435597)) ;
#79330=CARTESIAN_POINT('Ctrl Pts',(50.3087987422526,248.29078568304,31.7413203435596)) ;
#79331=CARTESIAN_POINT('Ctrl Pts',(50.3057018899657,248.289967396769,31.7413203435596)) ;
#79332=CARTESIAN_POINT('Ctrl Pts',(50.8831605335109,248.366098818484,31.7054164275186)) ;
#79333=CARTESIAN_POINT('Ctrl Pts',(50.7693177137058,248.364889140804,31.7054164275186)) ;
#79334=CARTESIAN_POINT('Ctrl Pts',(50.6611870949586,248.363142107183,31.7054164275186)) ;
#79335=CARTESIAN_POINT('Ctrl Pts',(50.48051672475,248.335752825127,31.7054164275186)) ;
#79336=CARTESIAN_POINT('Ctrl Pts',(50.3998763353304,248.314886646393,31.7054164275185)) ;
#79337=CARTESIAN_POINT('Ctrl Pts',(50.31189617328,248.291603218974,31.7054164275186)) ;
#79338=CARTESIAN_POINT('Ctrl Pts',(50.3087987422526,248.29078568304,31.7054164275186)) ;
#79339=CARTESIAN_POINT('Ctrl Pts',(50.3057018899657,248.289967396769,31.7054164275186)) ;
#79340=CARTESIAN_POINT('Ctrl Pts',(50.8828400884159,248.396255920492,31.6432843121591)) ;
#79341=CARTESIAN_POINT('Ctrl Pts',(50.7689838795759,248.395080367539,31.6432843121591)) ;
#79342=CARTESIAN_POINT('Ctrl Pts',(50.6593409446893,248.393370604139,31.6432843121591)) ;
#79343=CARTESIAN_POINT('Ctrl Pts',(50.4739365108437,248.365260768839,31.6432843121591)) ;
#79344=CARTESIAN_POINT('Ctrl Pts',(50.3921658146156,248.344058969898,31.6432843121591)) ;
#79345=CARTESIAN_POINT('Ctrl Pts',(50.3041921025262,248.32076002337,31.6432843121591)) ;
#79346=CARTESIAN_POINT('Ctrl Pts',(50.3010938281301,248.319945161113,31.6432843121591)) ;
#79347=CARTESIAN_POINT('Ctrl Pts',(50.297997400334,248.319125488718,31.6432843121591)) ;
#79348=CARTESIAN_POINT('Ctrl Pts',(50.882171618778,248.459165627568,31.6213203435596)) ;
#79349=CARTESIAN_POINT('Ctrl Pts',(50.7683209006786,248.457976080325,31.6213203435596)) ;
#79350=CARTESIAN_POINT('Ctrl Pts',(50.6555070294052,248.456412411503,31.6213203435597)) ;
#79351=CARTESIAN_POINT('Ctrl Pts',(50.4602045792046,248.426813697693,31.6213203435596)) ;
#79352=CARTESIAN_POINT('Ctrl Pts',(50.3760989166878,248.404868583297,31.6213203435597)) ;
#79353=CARTESIAN_POINT('Ctrl Pts',(50.2881197869039,248.381586520614,31.6213203435596)) ;
#79354=CARTESIAN_POINT('Ctrl Pts',(50.2850219278525,248.380770298768,31.6213203435596)) ;
#79355=CARTESIAN_POINT('Ctrl Pts',(50.2819253259759,248.379951194812,31.6213203435596)) ;
#79356=CARTESIAN_POINT('Ctrl Pts',(50.8818855024848,248.486092044526,31.6213203435596)) ;
#79357=CARTESIAN_POINT('Ctrl Pts',(50.7680426826797,248.484882366845,31.6213203435596)) ;
#79358=CARTESIAN_POINT('Ctrl Pts',(50.6538689168924,248.483392574996,31.6213203435597)) ;
#79359=CARTESIAN_POINT('Ctrl Pts',(50.4543262221993,248.453158960515,31.6213203435596)) ;
#79360=CARTESIAN_POINT('Ctrl Pts',(50.3692249609673,248.430888524762,31.6213203435597)) ;
#79361=CARTESIAN_POINT('Ctrl Pts',(50.2812403793008,248.407621865807,31.6213203435596)) ;
#79362=CARTESIAN_POINT('Ctrl Pts',(50.2781430590352,248.406803910429,31.6213203435596)) ;
#79363=CARTESIAN_POINT('Ctrl Pts',(50.2750462067483,248.405985624158,31.6213203435596)) ;
#79364=CARTESIAN_POINT('',(50.3149897315107,248.29242201045,31.7413203435596)) ;
#79365=CARTESIAN_POINT('',(50.8825230540255,248.366092043133,31.7413203435596)) ;
#79366=CARTESIAN_POINT('Ctrl Pts',(50.3149921209254,248.292422543133,31.7413203435596)) ;
#79367=CARTESIAN_POINT('Ctrl Pts',(50.3998764650291,248.314886679953,31.7413203435596)) ;
#79368=CARTESIAN_POINT('Ctrl Pts',(50.4805167880214,248.335752834719,31.7413203435596)) ;
#79369=CARTESIAN_POINT('Ctrl Pts',(50.6609967037988,248.363113244248,31.7413203435596)) ;
#79370=CARTESIAN_POINT('Ctrl Pts',(50.7689140351779,248.364882570555,31.7413203435596)) ;
#79371=CARTESIAN_POINT('Ctrl Pts',(50.8825230540528,248.36609203838,31.7413203435597)) ;
#79372=CARTESIAN_POINT('',(50.8818855024848,248.486092044526,31.6213203435596)) ;
#79373=CARTESIAN_POINT('Ctrl Pts',(50.8825230540529,248.366092044717,31.7413203435596)) ;
#79374=CARTESIAN_POINT('Ctrl Pts',(50.8825534101719,248.366092044717,31.7323443646095)) ;
#79375=CARTESIAN_POINT('Ctrl Pts',(50.8825723197285,248.367103672931,31.7233637724199)) ;
#79376=CARTESIAN_POINT('Ctrl Pts',(50.8825808693696,248.369103069156,31.7146074328755)) ;
#79377=CARTESIAN_POINT('Ctrl Pts',(50.8825893303654,248.371081735008,31.7059418818336)) ;
#79378=CARTESIAN_POINT('Ctrl Pts',(50.8825876451619,248.374027516586,31.6974967825055)) ;
#79379=CARTESIAN_POINT('Ctrl Pts',(50.882576866955,248.37786615277,31.6894825551018)) ;
#79380=CARTESIAN_POINT('Ctrl Pts',(50.8825659193641,248.381765114724,31.6813423807673)) ;
#79381=CARTESIAN_POINT('Ctrl Pts',(50.8825455907234,248.386584929551,31.6736475899965)) ;
#79382=CARTESIAN_POINT('Ctrl Pts',(50.8825169846678,248.392198656087,31.6665939655429)) ;
#79383=CARTESIAN_POINT('Ctrl Pts',(50.8824883786122,248.397812382623,31.6595403410893)) ;
#79384=CARTESIAN_POINT('Ctrl Pts',(50.8824514951415,248.40421940593,31.6531285618175)) ;
#79385=CARTESIAN_POINT('Ctrl Pts',(50.8824074378906,248.411251057174,31.6475182829018)) ;
#79386=CARTESIAN_POINT('Ctrl Pts',(50.8823652042211,248.417991660111,31.642140220023)) ;
#79387=CARTESIAN_POINT('Ctrl Pts',(50.8823163775403,248.425329993554,31.6374798978438)) ;
#79388=CARTESIAN_POINT('Ctrl Pts',(50.882263087073,248.433092826769,31.6336584519873)) ;
#79389=CARTESIAN_POINT('Ctrl Pts',(50.8822098779665,248.440843808143,31.6298428404918)) ;
#79390=CARTESIAN_POINT('Ctrl Pts',(50.8821522186931,248.449017181676,31.6268640064795)) ;
#79391=CARTESIAN_POINT('Ctrl Pts',(50.8820922287401,248.457415213738,31.6247972155335)) ;
#79392=CARTESIAN_POINT('Ctrl Pts',(50.8820322287777,248.465814647027,31.6227300797397)) ;
#79393=CARTESIAN_POINT('Ctrl Pts',(50.8819698973578,248.474437905681,31.6215755144355)) ;
#79394=CARTESIAN_POINT('Ctrl Pts',(50.8819073550288,248.483074795671,31.6213582820227)) ;
#79395=CARTESIAN_POINT('Ctrl Pts',(50.8819000725911,248.48408047637,31.6213329874496)) ;
#79396=CARTESIAN_POINT('Ctrl Pts',(50.8818927872939,248.485086337244,31.6213203435612)) ;
#79397=CARTESIAN_POINT('Ctrl Pts',(50.8818855024848,248.486092044526,31.6213203435596)) ;
#79398=CARTESIAN_POINT('',(50.2750462067483,248.405985624158,31.6213203435596)) ;
#79399=CARTESIAN_POINT('Ctrl Pts',(50.8818855024848,248.486092044526,31.6213203435596)) ;
#79400=CARTESIAN_POINT('Ctrl Pts',(50.7680426826797,248.484882366845,31.6213203435596)) ;
#79401=CARTESIAN_POINT('Ctrl Pts',(50.6538689168924,248.483392574996,31.6213203435597)) ;
#79402=CARTESIAN_POINT('Ctrl Pts',(50.4543262221993,248.453158960515,31.6213203435596)) ;
#79403=CARTESIAN_POINT('Ctrl Pts',(50.3692249609673,248.430888524762,31.6213203435597)) ;
#79404=CARTESIAN_POINT('Ctrl Pts',(50.2812403793008,248.407621865807,31.6213203435596)) ;
#79405=CARTESIAN_POINT('Ctrl Pts',(50.2781430590352,248.406803910429,31.6213203435596)) ;
#79406=CARTESIAN_POINT('Ctrl Pts',(50.2750462067483,248.405985624158,31.6213203435596)) ;
#79407=CARTESIAN_POINT('Ctrl Pts',(50.2750462067483,248.405985624158,31.6213203435597)) ;
#79408=CARTESIAN_POINT('Ctrl Pts',(50.2751432418492,248.405709761836,31.6213203435597)) ;
#79409=CARTESIAN_POINT('Ctrl Pts',(50.2752402756055,248.405433899341,31.6213214466179)) ;
#79410=CARTESIAN_POINT('Ctrl Pts',(50.2805774980751,248.390260268583,31.6214426485925)) ;
#79411=CARTESIAN_POINT('Ctrl Pts',(50.2858131262488,248.37537442858,31.6247712032253)) ;
#79412=CARTESIAN_POINT('Ctrl Pts',(50.2946911962445,248.350147654523,31.636032021281)) ;
#79413=CARTESIAN_POINT('Ctrl Pts',(50.2991400709367,248.337508840197,31.6439361481532)) ;
#79414=CARTESIAN_POINT('Ctrl Pts',(50.306843750394,248.315602834959,31.667336609376)) ;
#79415=CARTESIAN_POINT('Ctrl Pts',(50.3097222277476,248.307408665322,31.6803338949418)) ;
#79416=CARTESIAN_POINT('Ctrl Pts',(50.3127818601181,248.298696206946,31.7018216584692)) ;
#79417=CARTESIAN_POINT('Ctrl Pts',(50.313595920062,248.296377561573,31.7095201461793)) ;
#79418=CARTESIAN_POINT('Ctrl Pts',(50.314697907942,248.29323881435,31.7252539715263)) ;
#79419=CARTESIAN_POINT('Ctrl Pts',(50.3149851263684,248.292420692069,31.7332794168424)) ;
#79420=CARTESIAN_POINT('Ctrl Pts',(50.3149851263684,248.292420692069,31.7413203435596)) ;
#79421=CARTESIAN_POINT('Ctrl Pts',(50.090934083219,247.234198089337,31.7413203435596)) ;
#79422=CARTESIAN_POINT('Ctrl Pts',(50.0955897177682,247.231322397455,31.7413203435596)) ;
#79423=CARTESIAN_POINT('Ctrl Pts',(50.1002475219359,247.228449453589,31.7413203435596)) ;
#79424=CARTESIAN_POINT('Ctrl Pts',(50.1974027007021,247.168311194945,31.7413203435596)) ;
#79425=CARTESIAN_POINT('Ctrl Pts',(50.2828817770592,247.117341800874,31.7413203435594)) ;
#79426=CARTESIAN_POINT('Ctrl Pts',(50.48239795585,247.050779599937,31.7413203435595)) ;
#79427=CARTESIAN_POINT('Ctrl Pts',(50.61275116216,247.045540729033,31.7413203435581)) ;
#79428=CARTESIAN_POINT('Ctrl Pts',(50.754699340979,247.042754795613,31.7413203435597)) ;
#79429=CARTESIAN_POINT('Ctrl Pts',(50.7551163582219,247.042745762277,31.7413203435596)) ;
#79430=CARTESIAN_POINT('Ctrl Pts',(50.7555331333966,247.042737076062,31.7413203435596)) ;
#79431=CARTESIAN_POINT('Ctrl Pts',(50.090934083219,247.234198089337,31.7054164275186)) ;
#79432=CARTESIAN_POINT('Ctrl Pts',(50.0955897177682,247.231322397455,31.7054164275186)) ;
#79433=CARTESIAN_POINT('Ctrl Pts',(50.1002475219359,247.228449453589,31.7054164275186)) ;
#79434=CARTESIAN_POINT('Ctrl Pts',(50.1974027007021,247.168311194945,31.7054164275186)) ;
#79435=CARTESIAN_POINT('Ctrl Pts',(50.2828817770592,247.117341800874,31.7054164275184)) ;
#79436=CARTESIAN_POINT('Ctrl Pts',(50.48239795585,247.050779599937,31.7054164275185)) ;
#79437=CARTESIAN_POINT('Ctrl Pts',(50.61275116216,247.045540729033,31.7054164275171)) ;
#79438=CARTESIAN_POINT('Ctrl Pts',(50.754699340979,247.042754795613,31.7054164275186)) ;
#79439=CARTESIAN_POINT('Ctrl Pts',(50.7551163582219,247.042745762277,31.7054164275186)) ;
#79440=CARTESIAN_POINT('Ctrl Pts',(50.7555331333966,247.042737076062,31.7054164275186)) ;
#79441=CARTESIAN_POINT('Ctrl Pts',(50.0750852444689,247.208539428997,31.643284293333)) ;
#79442=CARTESIAN_POINT('Ctrl Pts',(50.079737436052,247.205657852922,31.643284293333)) ;
#79443=CARTESIAN_POINT('Ctrl Pts',(50.084402484806,247.202796447652,31.643284293333)) ;
#79444=CARTESIAN_POINT('Ctrl Pts',(50.181499622757,247.142586958144,31.6432842933329)) ;
#79445=CARTESIAN_POINT('Ctrl Pts',(50.2691603574096,247.090132541043,31.6432842933329)) ;
#79446=CARTESIAN_POINT('Ctrl Pts',(50.4783018806032,247.020329393151,31.6432842933329)) ;
#79447=CARTESIAN_POINT('Ctrl Pts',(50.612092332105,247.015290900225,31.6432842933323)) ;
#79448=CARTESIAN_POINT('Ctrl Pts',(50.7540735388923,247.012605482336,31.6432842933329)) ;
#79449=CARTESIAN_POINT('Ctrl Pts',(50.7544850390502,247.012590329561,31.6432842933329)) ;
#79450=CARTESIAN_POINT('Ctrl Pts',(50.7549047158396,247.012584835157,31.643284293333)) ;
#79451=CARTESIAN_POINT('Ctrl Pts',(50.0420234943591,247.155013727228,31.6213203435596)) ;
#79452=CARTESIAN_POINT('Ctrl Pts',(50.0466770974599,247.152134563504,31.6213203435596)) ;
#79453=CARTESIAN_POINT('Ctrl Pts',(50.0513388387582,247.14926712736,31.6213203435596)) ;
#79454=CARTESIAN_POINT('Ctrl Pts',(50.1484713080158,247.089126522815,31.6213203435596)) ;
#79455=CARTESIAN_POINT('Ctrl Pts',(50.2404085533977,247.033396611465,31.6213203435596)) ;
#79456=CARTESIAN_POINT('Ctrl Pts',(50.4699588786217,246.956838370791,31.6213203435596)) ;
#79457=CARTESIAN_POINT('Ctrl Pts',(50.6108414563099,246.952489795875,31.6213203435594)) ;
#79458=CARTESIAN_POINT('Ctrl Pts',(50.7527614502915,246.949704550992,31.6213203435596)) ;
#79459=CARTESIAN_POINT('Ctrl Pts',(50.7531753070812,246.949692023209,31.6213203435596)) ;
#79460=CARTESIAN_POINT('Ctrl Pts',(50.7535937942914,246.949685220255,31.6213203435596)) ;
#79461=CARTESIAN_POINT('Ctrl Pts',(50.0278725105413,247.132103828718,31.6213203435596)) ;
#79462=CARTESIAN_POINT('Ctrl Pts',(50.0325281450905,247.129228136836,31.6213203435596)) ;
#79463=CARTESIAN_POINT('Ctrl Pts',(50.0371854114367,247.126353120034,31.6213203435596)) ;
#79464=CARTESIAN_POINT('Ctrl Pts',(50.1343589801246,247.066278119072,31.6213203435596)) ;
#79465=CARTESIAN_POINT('Ctrl Pts',(50.2280810409672,247.009116738647,31.6213203435596)) ;
#79466=CARTESIAN_POINT('Ctrl Pts',(50.4664214310973,246.92966815855,31.6213203435596)) ;
#79467=CARTESIAN_POINT('Ctrl Pts',(50.6103265699945,246.925660041206,31.6213203435594)) ;
#79468=CARTESIAN_POINT('Ctrl Pts',(50.752198754358,246.922780663952,31.6213203435596)) ;
#79469=CARTESIAN_POINT('Ctrl Pts',(50.7526159226971,246.922771815846,31.6213203435596)) ;
#79470=CARTESIAN_POINT('Ctrl Pts',(50.7530326978718,246.922763129631,31.6213203435596)) ;
#79471=CARTESIAN_POINT('',(50.7530325637488,246.922763132443,31.6213203435596)) ;
#79472=CARTESIAN_POINT('Ctrl Pts',(50.0278725105413,247.132103828718,31.6213203435596)) ;
#79473=CARTESIAN_POINT('Ctrl Pts',(50.0325281450905,247.129228136836,31.6213203435596)) ;
#79474=CARTESIAN_POINT('Ctrl Pts',(50.0371854114367,247.126353120034,31.6213203435596)) ;
#79475=CARTESIAN_POINT('Ctrl Pts',(50.1343589801246,247.066278119072,31.6213203435596)) ;
#79476=CARTESIAN_POINT('Ctrl Pts',(50.2280810409672,247.009116738647,31.6213203435596)) ;
#79477=CARTESIAN_POINT('Ctrl Pts',(50.4664214310973,246.92966815855,31.6213203435596)) ;
#79478=CARTESIAN_POINT('Ctrl Pts',(50.6103265699945,246.925660041206,31.6213203435594)) ;
#79479=CARTESIAN_POINT('Ctrl Pts',(50.752198709726,246.922780664858,31.6213203435596)) ;
#79480=CARTESIAN_POINT('Ctrl Pts',(50.7526158331972,246.922771817744,31.6213203435596)) ;
#79481=CARTESIAN_POINT('Ctrl Pts',(50.7530325637484,246.922763132426,31.6213203435596)) ;
#79482=CARTESIAN_POINT('',(50.7542787411678,247.0427631542,31.7413203435596)) ;
#79483=CARTESIAN_POINT('Ctrl Pts',(50.7530325621815,246.922763132459,31.6213203435596)) ;
#79484=CARTESIAN_POINT('Ctrl Pts',(50.7527646460474,246.923064784013,31.6213203435596)) ;
#79485=CARTESIAN_POINT('Ctrl Pts',(50.7525399567633,246.923325470576,31.6213212662913)) ;
#79486=CARTESIAN_POINT('Ctrl Pts',(50.7496325890277,246.926757551588,31.6213461545782)) ;
#79487=CARTESIAN_POINT('Ctrl Pts',(50.7470175666196,246.930311340193,31.6214748940474)) ;
#79488=CARTESIAN_POINT('Ctrl Pts',(50.7435785332281,246.938306579103,31.6222776096934)) ;
#79489=CARTESIAN_POINT('Ctrl Pts',(50.7426974857717,246.941965162815,31.6228030626945)) ;
#79490=CARTESIAN_POINT('Ctrl Pts',(50.742015015904,246.951808512294,31.6247263169256)) ;
#79491=CARTESIAN_POINT('Ctrl Pts',(50.7431812437154,246.957639467861,31.6263476325659)) ;
#79492=CARTESIAN_POINT('Ctrl Pts',(50.74716434657,246.970554975215,31.630972221387)) ;
#79493=CARTESIAN_POINT('Ctrl Pts',(50.750429117442,246.977541017359,31.6342831692237)) ;
#79494=CARTESIAN_POINT('Ctrl Pts',(50.7527478979496,246.985568780879,31.6390534647648)) ;
#79495=CARTESIAN_POINT('Ctrl Pts',(50.7540558850527,246.99020320561,31.6418509510241)) ;
#79496=CARTESIAN_POINT('Ctrl Pts',(50.7533210295252,246.999864991888,31.6491953852256)) ;
#79497=CARTESIAN_POINT('Ctrl Pts',(50.751086767988,247.003933060654,31.6527832509983)) ;
#79498=CARTESIAN_POINT('Ctrl Pts',(50.7460406591654,247.012784207256,31.6616377388116)) ;
#79499=CARTESIAN_POINT('Ctrl Pts',(50.7421051714273,247.018704860938,31.6684626416789)) ;
#79500=CARTESIAN_POINT('Ctrl Pts',(50.7399004608286,247.028197434459,31.6835662597949)) ;
#79501=CARTESIAN_POINT('Ctrl Pts',(50.7403530673341,247.031356765315,31.6897667463312)) ;
#79502=CARTESIAN_POINT('Ctrl Pts',(50.7435531726753,247.037095265575,31.7039618703478)) ;
#79503=CARTESIAN_POINT('Ctrl Pts',(50.7464670059396,247.039184790426,31.7113680720848)) ;
#79504=CARTESIAN_POINT('Ctrl Pts',(50.7517448065935,247.042040603547,31.7260362201993)) ;
#79505=CARTESIAN_POINT('Ctrl Pts',(50.7542745642648,247.042763132459,31.7337592180439)) ;
#79506=CARTESIAN_POINT('Ctrl Pts',(50.7542745642651,247.042763132459,31.7413203435596)) ;
#79507=CARTESIAN_POINT('Ctrl Pts',(50.7542787425273,247.042763219434,31.7413203435596)) ;
#79508=CARTESIAN_POINT('Ctrl Pts',(50.7271094895703,247.043329467085,31.7413203435593)) ;
#79509=CARTESIAN_POINT('Ctrl Pts',(50.7003265960474,247.043892035075,31.7413203435591)) ;
#79510=CARTESIAN_POINT('Ctrl Pts',(50.6740010884586,247.044750914502,31.741320343559)) ;
#79511=CARTESIAN_POINT('Ctrl Pts',(50.6460147492917,247.045663979173,31.7413203435589)) ;
#79512=CARTESIAN_POINT('Ctrl Pts',(50.618545300155,247.046911831848,31.7413203435589)) ;
#79513=CARTESIAN_POINT('Ctrl Pts',(50.59166023966,247.048796849032,31.7413203435589)) ;
#79514=CARTESIAN_POINT('Ctrl Pts',(50.5637291844762,247.050755205011,31.7413203435589)) ;
#79515=CARTESIAN_POINT('Ctrl Pts',(50.536428756022,247.053400881479,31.741320343559)) ;
#79516=CARTESIAN_POINT('Ctrl Pts',(50.5098172256807,247.057016257844,31.7413203435591)) ;
#79517=CARTESIAN_POINT('Ctrl Pts',(50.4812755613452,247.060893857416,31.7413203435592)) ;
#79518=CARTESIAN_POINT('Ctrl Pts',(50.4535262834992,247.065886704076,31.7413203435593)) ;
#79519=CARTESIAN_POINT('Ctrl Pts',(50.4266229919826,247.072283650437,31.7413203435594)) ;
#79520=CARTESIAN_POINT('Ctrl Pts',(50.407159438196,247.076911608673,31.7413203435594)) ;
#79521=CARTESIAN_POINT('Ctrl Pts',(50.3881382694205,247.082273157551,31.7413203435595)) ;
#79522=CARTESIAN_POINT('Ctrl Pts',(50.369574863394,247.088461667103,31.7413203435594)) ;
#79523=CARTESIAN_POINT('Ctrl Pts',(50.3695707922032,247.088463024321,31.7413203435594)) ;
#79524=CARTESIAN_POINT('Ctrl Pts',(50.3695667210145,247.088464381587,31.7413203435594)) ;
#79525=CARTESIAN_POINT('Ctrl Pts',(50.3695626498277,247.088465738898,31.7413203435594)) ;
#79526=CARTESIAN_POINT('Ctrl Pts',(50.346746489969,247.096072522687,31.7413203435594)) ;
#79527=CARTESIAN_POINT('Ctrl Pts',(50.3239939476063,247.105139848513,31.7413203435594)) ;
#79528=CARTESIAN_POINT('Ctrl Pts',(50.3011789250779,247.115462173694,31.7413203435595)) ;
#79529=CARTESIAN_POINT('Ctrl Pts',(50.280021321461,247.12503462379,31.7413203435595)) ;
#79530=CARTESIAN_POINT('Ctrl Pts',(50.2588101814923,247.135686992053,31.7413203435595)) ;
#79531=CARTESIAN_POINT('Ctrl Pts',(50.2374330483465,247.147216651365,31.7413203435595)) ;
#79532=CARTESIAN_POINT('Ctrl Pts',(50.2173075360903,247.158071254656,31.7413203435595)) ;
#79533=CARTESIAN_POINT('Ctrl Pts',(50.19703505635,247.169703937684,31.7413203435596)) ;
#79534=CARTESIAN_POINT('Ctrl Pts',(50.1765083716673,247.181902012136,31.7413203435596)) ;
#79535=CARTESIAN_POINT('Ctrl Pts',(50.1573661728375,247.19327734966,31.7413203435596)) ;
#79536=CARTESIAN_POINT('Ctrl Pts',(50.1380029859063,247.205144648437,31.7413203435596)) ;
#79537=CARTESIAN_POINT('Ctrl Pts',(50.11831824308,247.217287162085,31.7413203435596)) ;
#79538=CARTESIAN_POINT('Ctrl Pts',(50.1138614227384,247.220036347192,31.7413203435596)) ;
#79539=CARTESIAN_POINT('Ctrl Pts',(50.1093880575593,247.222799440314,31.7413203435596)) ;
#79540=CARTESIAN_POINT('Ctrl Pts',(50.1048968673761,247.225573558217,31.7413203435596)) ;
#79541=CARTESIAN_POINT('Origin',(50.7706539553668,246.922763132459,31.7413203435596)) ;
#79542=CARTESIAN_POINT('',(52.1403128398474,246.922763132459,31.6213203435596)) ;
#79543=CARTESIAN_POINT('',(50.7706539553668,246.922763132459,31.6213203435596)) ;
#79544=CARTESIAN_POINT('',(52.0203128398474,247.042763132459,31.7413203435596)) ;
#79545=CARTESIAN_POINT('Origin',(52.1403128398474,246.922763132459,31.7413203435596)) ;
#79546=CARTESIAN_POINT('',(50.7706539553668,247.042763132459,31.7413203435596)) ;
#79547=CARTESIAN_POINT('Origin',(52.1403128398474,247.821753594881,31.7413203435596)) ;
#79548=CARTESIAN_POINT('',(52.0203128398474,248.366092044717,31.7413203435596)) ;
#79549=CARTESIAN_POINT('',(52.0203128398474,247.821753594881,31.7413203435596)) ;
#79550=CARTESIAN_POINT('',(52.1403128398474,248.486092044717,31.6213203435596)) ;
#79551=CARTESIAN_POINT('',(52.1403128398474,247.821753594881,31.6213203435596)) ;
#79552=CARTESIAN_POINT('Origin',(52.1403128398474,248.486092044717,31.7413203435596)) ;
#79553=CARTESIAN_POINT('Origin',(51.4036689174439,248.486092044717,31.7413203435596)) ;
#79554=CARTESIAN_POINT('',(51.4036689174439,248.366092044717,31.7413203435596)) ;
#79555=CARTESIAN_POINT('',(51.4036689174439,248.486092044717,31.6213203435596)) ;
#79556=CARTESIAN_POINT('Ctrl Pts',(50.3237735145971,248.296324101873,31.7413203435596)) ;
#79557=CARTESIAN_POINT('Ctrl Pts',(50.3208460868592,248.295023320436,31.7413203435596)) ;
#79558=CARTESIAN_POINT('Ctrl Pts',(50.3179187784833,248.293719247106,31.7413203435596)) ;
#79559=CARTESIAN_POINT('Ctrl Pts',(50.2432348124463,248.260661053439,31.7413203435597)) ;
#79560=CARTESIAN_POINT('Ctrl Pts',(50.1823953545993,248.2316465172,31.7413203435596)) ;
#79561=CARTESIAN_POINT('Ctrl Pts',(50.0901995406341,248.158990991578,31.7413203435596)) ;
#79562=CARTESIAN_POINT('Ctrl Pts',(50.0496571268392,248.110309168465,31.7413203435596)) ;
#79563=CARTESIAN_POINT('Ctrl Pts',(50.0018795748302,248.049699199696,31.7413203435596)) ;
#79564=CARTESIAN_POINT('Ctrl Pts',(49.9998104000328,248.04708637804,31.7413203435596)) ;
#79565=CARTESIAN_POINT('Ctrl Pts',(49.9977443179459,248.04447261808,31.7413203435596)) ;
#79566=CARTESIAN_POINT('Ctrl Pts',(50.3237735145971,248.296324101873,31.7054164275186)) ;
#79567=CARTESIAN_POINT('Ctrl Pts',(50.3208460868592,248.295023320436,31.7054164275186)) ;
#79568=CARTESIAN_POINT('Ctrl Pts',(50.3179187784833,248.293719247106,31.7054164275186)) ;
#79569=CARTESIAN_POINT('Ctrl Pts',(50.2432348124463,248.260661053439,31.7054164275186)) ;
#79570=CARTESIAN_POINT('Ctrl Pts',(50.1823953545993,248.2316465172,31.7054164275186)) ;
#79571=CARTESIAN_POINT('Ctrl Pts',(50.0901995406341,248.158990991578,31.7054164275186)) ;
#79572=CARTESIAN_POINT('Ctrl Pts',(50.0496571268392,248.110309168465,31.7054164275186)) ;
#79573=CARTESIAN_POINT('Ctrl Pts',(50.0018795748302,248.049699199696,31.7054164275186)) ;
#79574=CARTESIAN_POINT('Ctrl Pts',(49.9998104000328,248.04708637804,31.7054164275186)) ;
#79575=CARTESIAN_POINT('Ctrl Pts',(49.9977443179459,248.04447261808,31.7054164275186)) ;
#79576=CARTESIAN_POINT('Ctrl Pts',(50.3115272061083,248.323884599068,31.6432843040156)) ;
#79577=CARTESIAN_POINT('Ctrl Pts',(50.3085977460324,248.322586591314,31.6432843040155)) ;
#79578=CARTESIAN_POINT('Ctrl Pts',(50.3056742108328,248.321276920664,31.6432843040155)) ;
#79579=CARTESIAN_POINT('Ctrl Pts',(50.2309743184436,248.288272310817,31.6432843040156)) ;
#79580=CARTESIAN_POINT('Ctrl Pts',(50.1673000436637,248.258157776563,31.6432843040156)) ;
#79581=CARTESIAN_POINT('Ctrl Pts',(50.068167766932,248.180033272884,31.6432843040156)) ;
#79582=CARTESIAN_POINT('Ctrl Pts',(50.0259496726954,248.129031375463,31.6432843040156)) ;
#79583=CARTESIAN_POINT('Ctrl Pts',(49.9782226660684,248.06839939147,31.6432843040155)) ;
#79584=CARTESIAN_POINT('Ctrl Pts',(49.976147980735,248.065790714156,31.6432843040156)) ;
#79585=CARTESIAN_POINT('Ctrl Pts',(49.9740845925537,248.063174769602,31.6432843040155)) ;
#79586=CARTESIAN_POINT('Ctrl Pts',(50.2859805890603,248.381377636101,31.6213203435597)) ;
#79587=CARTESIAN_POINT('Ctrl Pts',(50.2830519623244,248.380078491027,31.6213203435596)) ;
#79588=CARTESIAN_POINT('Ctrl Pts',(50.2801263647861,248.378771734628,31.6213203435596)) ;
#79589=CARTESIAN_POINT('Ctrl Pts',(50.2054515729317,248.34572107069,31.6213203435597)) ;
#79590=CARTESIAN_POINT('Ctrl Pts',(50.1358824073971,248.313488625072,31.6213203435596)) ;
#79591=CARTESIAN_POINT('Ctrl Pts',(50.0221638717514,248.223877898007,31.6213203435597)) ;
#79592=CARTESIAN_POINT('Ctrl Pts',(49.9766326160923,248.16801950669,31.6213203435597)) ;
#79593=CARTESIAN_POINT('Ctrl Pts',(49.9288651949389,248.107414681377,31.6213203435596)) ;
#79594=CARTESIAN_POINT('Ctrl Pts',(49.926793318698,248.104803754981,31.6213203435596)) ;
#79595=CARTESIAN_POINT('Ctrl Pts',(49.9247288259075,248.102188706199,31.6213203435596)) ;
#79596=CARTESIAN_POINT('Ctrl Pts',(50.2750462067483,248.405985624158,31.6213203435597)) ;
#79597=CARTESIAN_POINT('Ctrl Pts',(50.2721187790104,248.40468484272,31.6213203435597)) ;
#79598=CARTESIAN_POINT('Ctrl Pts',(50.2691906493995,248.403381756314,31.6213203435596)) ;
#79599=CARTESIAN_POINT('Ctrl Pts',(50.1945362851629,248.370285173624,31.6213203435597)) ;
#79600=CARTESIAN_POINT('Ctrl Pts',(50.1224471164977,248.337175575328,31.6213203435596)) ;
#79601=CARTESIAN_POINT('Ctrl Pts',(50.0024661001059,248.242635671415,31.6213203435597)) ;
#79602=CARTESIAN_POINT('Ctrl Pts',(49.9555470447246,248.184695852018,31.6213203435597)) ;
#79603=CARTESIAN_POINT('Ctrl Pts',(49.9077381074784,248.124114785998,31.6213203435596)) ;
#79604=CARTESIAN_POINT('Ctrl Pts',(49.9056698086987,248.121501088032,31.6213203435596)) ;
#79605=CARTESIAN_POINT('Ctrl Pts',(49.9036037266118,248.118887328072,31.6213203435596)) ;
#79606=CARTESIAN_POINT('',(50.0039413950685,248.052313607497,31.7413203435596)) ;
#79607=CARTESIAN_POINT('Ctrl Pts',(50.0039408165155,248.052314063558,31.7413203435596)) ;
#79608=CARTESIAN_POINT('Ctrl Pts',(50.0496575583587,248.110309686617,31.7413203435596)) ;
#79609=CARTESIAN_POINT('Ctrl Pts',(50.0901997785078,248.158991179037,31.7413203435596)) ;
#79610=CARTESIAN_POINT('Ctrl Pts',(50.1823947037638,248.231646004304,31.7413203435596)) ;
#79611=CARTESIAN_POINT('Ctrl Pts',(50.2432331451607,248.260660258303,31.7413203435597)) ;
#79612=CARTESIAN_POINT('Ctrl Pts',(50.3149894650065,248.292422612535,31.7413203435596)) ;
#79613=CARTESIAN_POINT('',(49.9036037266118,248.118887328072,31.6213203435596)) ;
#79614=CARTESIAN_POINT('Ctrl Pts',(50.2750462067483,248.405985624158,31.6213203435597)) ;
#79615=CARTESIAN_POINT('Ctrl Pts',(50.2721187790104,248.40468484272,31.6213203435597)) ;
#79616=CARTESIAN_POINT('Ctrl Pts',(50.2691906493995,248.403381756314,31.6213203435596)) ;
#79617=CARTESIAN_POINT('Ctrl Pts',(50.1945362851629,248.370285173624,31.6213203435597)) ;
#79618=CARTESIAN_POINT('Ctrl Pts',(50.1224471164977,248.337175575328,31.6213203435596)) ;
#79619=CARTESIAN_POINT('Ctrl Pts',(50.0024661001059,248.242635671415,31.6213203435597)) ;
#79620=CARTESIAN_POINT('Ctrl Pts',(49.9555470447246,248.184695852018,31.6213203435597)) ;
#79621=CARTESIAN_POINT('Ctrl Pts',(49.9077381074784,248.124114785998,31.6213203435596)) ;
#79622=CARTESIAN_POINT('Ctrl Pts',(49.9056698086987,248.121501088032,31.6213203435596)) ;
#79623=CARTESIAN_POINT('Ctrl Pts',(49.9036037266118,248.118887328072,31.6213203435596)) ;
#79624=CARTESIAN_POINT('Ctrl Pts',(49.9036037266118,248.118887328072,31.6213203435596)) ;
#79625=CARTESIAN_POINT('Ctrl Pts',(49.9038474528801,248.118725615821,31.6213203435596)) ;
#79626=CARTESIAN_POINT('Ctrl Pts',(49.9040911791549,248.118563904141,31.6213214465272)) ;
#79627=CARTESIAN_POINT('Ctrl Pts',(49.9174965285971,248.109669521949,31.6214426327676)) ;
#79628=CARTESIAN_POINT('Ctrl Pts',(49.9306479955595,248.100944075181,31.6247706510038)) ;
#79629=CARTESIAN_POINT('Ctrl Pts',(49.9529368794178,248.086154166638,31.6360300282615)) ;
#79630=CARTESIAN_POINT('Ctrl Pts',(49.9641037850844,248.078743851301,31.6439332011361)) ;
#79631=CARTESIAN_POINT('Ctrl Pts',(49.9834573384472,248.065902717465,31.6673300848568)) ;
#79632=CARTESIAN_POINT('Ctrl Pts',(49.9906968210535,248.061100122706,31.6803259746533)) ;
#79633=CARTESIAN_POINT('Ctrl Pts',(49.9983952806611,248.055993282155,31.7018142049946)) ;
#79634=CARTESIAN_POINT('Ctrl Pts',(50.0004443425674,248.054634068328,31.7095140383626)) ;
#79635=CARTESIAN_POINT('Ctrl Pts',(50.0032181564329,248.052794101758,31.725250816951)) ;
#79636=CARTESIAN_POINT('Ctrl Pts',(50.0039411676504,248.052314509003,31.7332778179758)) ;
#79637=CARTESIAN_POINT('Ctrl Pts',(50.0039411676504,248.052314509003,31.7413203435596)) ;
#79638=CARTESIAN_POINT('Ctrl Pts',(50.0087569650634,248.061070406301,31.7413203435596)) ;
#79639=CARTESIAN_POINT('Ctrl Pts',(50.0071517479483,248.058150953433,31.7413203435596)) ;
#79640=CARTESIAN_POINT('Ctrl Pts',(50.0055483551771,248.055229229945,31.7413203435596)) ;
#79641=CARTESIAN_POINT('Ctrl Pts',(49.9690056264369,247.988957027741,31.7413203435597)) ;
#79642=CARTESIAN_POINT('Ctrl Pts',(49.9400850019578,247.933416217127,31.7413203435596)) ;
#79643=CARTESIAN_POINT('Ctrl Pts',(49.908310637077,247.825263262329,31.7413203435596)) ;
#79644=CARTESIAN_POINT('Ctrl Pts',(49.9025264824017,247.763574370657,31.7413203435596)) ;
#79645=CARTESIAN_POINT('Ctrl Pts',(49.8972996831157,247.688877147303,31.7413203435596)) ;
#79646=CARTESIAN_POINT('Ctrl Pts',(49.8970639748427,247.685602333175,31.7413203435596)) ;
#79647=CARTESIAN_POINT('Ctrl Pts',(49.8968309655685,247.682328422,31.7413203435596)) ;
#79648=CARTESIAN_POINT('Ctrl Pts',(50.0087569650634,248.061070406301,31.7054164275186)) ;
#79649=CARTESIAN_POINT('Ctrl Pts',(50.0071517479483,248.058150953433,31.7054164275186)) ;
#79650=CARTESIAN_POINT('Ctrl Pts',(50.0055483551771,248.055229229945,31.7054164275186)) ;
#79651=CARTESIAN_POINT('Ctrl Pts',(49.9690056264369,247.988957027741,31.7054164275186)) ;
#79652=CARTESIAN_POINT('Ctrl Pts',(49.9400850019578,247.933416217127,31.7054164275186)) ;
#79653=CARTESIAN_POINT('Ctrl Pts',(49.908310637077,247.825263262329,31.7054164275186)) ;
#79654=CARTESIAN_POINT('Ctrl Pts',(49.9025264824017,247.763574370657,31.7054164275186)) ;
#79655=CARTESIAN_POINT('Ctrl Pts',(49.8972996831157,247.688877147303,31.7054164275186)) ;
#79656=CARTESIAN_POINT('Ctrl Pts',(49.8970639748427,247.685602333175,31.7054164275186)) ;
#79657=CARTESIAN_POINT('Ctrl Pts',(49.8968309655685,247.682328422,31.7054164275186)) ;
#79658=CARTESIAN_POINT('Ctrl Pts',(49.9823295099218,248.075601143813,31.6432842968685)) ;
#79659=CARTESIAN_POINT('Ctrl Pts',(49.9807217753671,248.072682998912,31.6432842968685)) ;
#79660=CARTESIAN_POINT('Ctrl Pts',(49.97912328038,248.069758521438,31.6432842968685)) ;
#79661=CARTESIAN_POINT('Ctrl Pts',(49.9425479159984,248.003516731425,31.6432842968685)) ;
#79662=CARTESIAN_POINT('Ctrl Pts',(49.9122630644889,247.945726734908,31.6432842968685)) ;
#79663=CARTESIAN_POINT('Ctrl Pts',(49.8782632727103,247.829997860369,31.6432842968685)) ;
#79664=CARTESIAN_POINT('Ctrl Pts',(49.8724029099475,247.765706746907,31.6432842968685)) ;
#79665=CARTESIAN_POINT('Ctrl Pts',(49.867219756094,247.691018175729,31.6432842968685)) ;
#79666=CARTESIAN_POINT('Ctrl Pts',(49.866978468971,247.687743550218,31.6432842968685)) ;
#79667=CARTESIAN_POINT('Ctrl Pts',(49.8667482678629,247.684469453685,31.6432842968685)) ;
#79668=CARTESIAN_POINT('Ctrl Pts',(49.9272000581419,248.105913241166,31.6213203435596)) ;
#79669=CARTESIAN_POINT('Ctrl Pts',(49.9255933557227,248.102994560006,31.6213203435596)) ;
#79670=CARTESIAN_POINT('Ctrl Pts',(49.9239922395177,248.100071502154,31.6213203435596)) ;
#79671=CARTESIAN_POINT('Ctrl Pts',(49.8874505962389,248.033806555933,31.6213203435596)) ;
#79672=CARTESIAN_POINT('Ctrl Pts',(49.854252009404,247.971446824694,31.6213203435596)) ;
#79673=CARTESIAN_POINT('Ctrl Pts',(49.8155828998778,247.839827717225,31.6213203435596)) ;
#79674=CARTESIAN_POINT('Ctrl Pts',(49.8096869765514,247.770175268382,31.6213203435597)) ;
#79675=CARTESIAN_POINT('Ctrl Pts',(49.8044634272261,247.695484582515,31.6213203435596)) ;
#79676=CARTESIAN_POINT('Ctrl Pts',(49.8042250862893,247.692209810553,31.6213203435596)) ;
#79677=CARTESIAN_POINT('Ctrl Pts',(49.8039937338495,247.688935790016,31.6213203435596)) ;
#79678=CARTESIAN_POINT('Ctrl Pts',(49.9036037266118,248.118887328072,31.6213203435596)) ;
#79679=CARTESIAN_POINT('Ctrl Pts',(49.9019985094967,248.115967875204,31.6213203435596)) ;
#79680=CARTESIAN_POINT('Ctrl Pts',(49.900394139303,248.113046614805,31.6213203435596)) ;
#79681=CARTESIAN_POINT('Ctrl Pts',(49.8638838353781,248.046757375974,31.6213203435596)) ;
#79682=CARTESIAN_POINT('Ctrl Pts',(49.8294268503797,247.982462018373,31.6213203435596)) ;
#79683=CARTESIAN_POINT('Ctrl Pts',(49.7887547225882,247.844027283432,31.6213203435596)) ;
#79684=CARTESIAN_POINT('Ctrl Pts',(49.782864074239,247.772091232065,31.6213203435597)) ;
#79685=CARTESIAN_POINT('Ctrl Pts',(49.7776014062417,247.697396292484,31.6213203435596)) ;
#79686=CARTESIAN_POINT('Ctrl Pts',(49.7773667482972,247.694121368174,31.6213203435596)) ;
#79687=CARTESIAN_POINT('Ctrl Pts',(49.777133739023,247.690847456999,31.6213203435596)) ;
#79688=CARTESIAN_POINT('Ctrl Pts',(49.8975299240168,247.692149180776,31.7413203435596)) ;
#79689=CARTESIAN_POINT('Ctrl Pts',(49.8986150818286,247.707396257523,31.7413203435596)) ;
#79690=CARTESIAN_POINT('Ctrl Pts',(49.8996743511139,247.7222161151,31.7413203435596)) ;
#79691=CARTESIAN_POINT('Ctrl Pts',(49.9008630958013,247.736607865466,31.7413203435596)) ;
#79692=CARTESIAN_POINT('Ctrl Pts',(49.9022047500129,247.75285084236,31.7413203435596)) ;
#79693=CARTESIAN_POINT('Ctrl Pts',(49.9037110345681,247.768548580157,31.7413203435596)) ;
#79694=CARTESIAN_POINT('Ctrl Pts',(49.9055395786114,247.783719168488,31.7413203435596)) ;
#79695=CARTESIAN_POINT('Ctrl Pts',(49.907561373165,247.800493067359,31.7413203435596)) ;
#79696=CARTESIAN_POINT('Ctrl Pts',(49.9099760964081,247.816622813088,31.7413203435596)) ;
#79697=CARTESIAN_POINT('Ctrl Pts',(49.9129324761923,247.832151816603,31.7413203435596)) ;
#79698=CARTESIAN_POINT('Ctrl Pts',(49.9160302485486,247.848423514193,31.7413203435596)) ;
#79699=CARTESIAN_POINT('Ctrl Pts',(49.9197208568293,247.864036184029,31.7413203435596)) ;
#79700=CARTESIAN_POINT('Ctrl Pts',(49.9241326690729,247.879052359467,31.7413203435596)) ;
#79701=CARTESIAN_POINT('Ctrl Pts',(49.9246589347965,247.880843573145,31.7413203435596)) ;
#79702=CARTESIAN_POINT('Ctrl Pts',(49.9251983743351,247.882636314972,31.7413203435596)) ;
#79703=CARTESIAN_POINT('Ctrl Pts',(49.9257508799616,247.884430785863,31.7413203435596)) ;
#79704=CARTESIAN_POINT('Ctrl Pts',(49.9305613985087,247.900054763414,31.7413203435596)) ;
#79705=CARTESIAN_POINT('Ctrl Pts',(49.9363650702522,247.915808958345,31.7413203435596)) ;
#79706=CARTESIAN_POINT('Ctrl Pts',(49.9430749294362,247.931828632111,31.7413203435596)) ;
#79707=CARTESIAN_POINT('Ctrl Pts',(49.9489705758089,247.945904386748,31.7413203435596)) ;
#79708=CARTESIAN_POINT('Ctrl Pts',(49.955566837351,247.960184802822,31.7413203435596)) ;
#79709=CARTESIAN_POINT('Ctrl Pts',(49.9627697116877,247.974771949686,31.7413203435596)) ;
#79710=CARTESIAN_POINT('Ctrl Pts',(49.9690514229702,247.987493571743,31.7413203435597)) ;
#79711=CARTESIAN_POINT('Ctrl Pts',(49.9757948143974,248.000448397417,31.7413203435597)) ;
#79712=CARTESIAN_POINT('Ctrl Pts',(49.9829015268903,248.013714738828,31.7413203435596)) ;
#79713=CARTESIAN_POINT('Ctrl Pts',(49.9896302636225,248.026275500058,31.7413203435596)) ;
#79714=CARTESIAN_POINT('Ctrl Pts',(49.9966853053433,248.039115344112,31.7413203435596)) ;
#79715=CARTESIAN_POINT('Ctrl Pts',(50.003941798311,248.05231292904,31.7413203435596)) ;
#79716=CARTESIAN_POINT('Ctrl Pts',(49.9036037266118,248.118887328072,31.6213203435596)) ;
#79717=CARTESIAN_POINT('Ctrl Pts',(49.9019985094967,248.115967875204,31.6213203435596)) ;
#79718=CARTESIAN_POINT('Ctrl Pts',(49.900394139303,248.113046614805,31.6213203435596)) ;
#79719=CARTESIAN_POINT('Ctrl Pts',(49.8638838353781,248.046757375974,31.6213203435596)) ;
#79720=CARTESIAN_POINT('Ctrl Pts',(49.8294268503797,247.982462018373,31.6213203435596)) ;
#79721=CARTESIAN_POINT('Ctrl Pts',(49.7887547225882,247.844027283432,31.6213203435596)) ;
#79722=CARTESIAN_POINT('Ctrl Pts',(49.782864074239,247.772091232065,31.6213203435597)) ;
#79723=CARTESIAN_POINT('Ctrl Pts',(49.7776014062417,247.697396292484,31.6213203435596)) ;
#79724=CARTESIAN_POINT('Ctrl Pts',(49.7773667482972,247.694121368174,31.6213203435596)) ;
#79725=CARTESIAN_POINT('Ctrl Pts',(49.777133739023,247.690847456999,31.6213203435596)) ;
#79726=CARTESIAN_POINT('Origin',(50.7542829156931,247.042763132459,31.9213203435596)) ;
#79727=CARTESIAN_POINT('',(52.0203128398474,247.042763132459,31.8013203435596)) ;
#79728=CARTESIAN_POINT('',(52.0203128398474,247.042763132459,31.9213203435596)) ;
#79729=CARTESIAN_POINT('',(50.7542829156931,247.042763132459,31.8013203435596)) ;
#79730=CARTESIAN_POINT('',(52.2271414578465,247.042763132459,31.8013203435596)) ;
#79731=CARTESIAN_POINT('',(50.7542829156931,247.042763132459,31.9213203435596)) ;
#79732=CARTESIAN_POINT('Origin',(52.0203128398474,247.042763132459,31.9213203435596)) ;
#79733=CARTESIAN_POINT('',(52.0203128398474,248.366092044717,31.8013203435596)) ;
#79734=CARTESIAN_POINT('',(52.0203128398474,248.366092044717,31.9213203435596)) ;
#79735=CARTESIAN_POINT('',(52.0203128398474,243.213135158824,31.8013203435596)) ;
#79736=CARTESIAN_POINT('Origin',(52.0203128398474,248.366092044717,31.9213203435596)) ;
#79737=CARTESIAN_POINT('',(50.8825230539854,248.366092044717,31.8013203435596)) ;
#79738=CARTESIAN_POINT('',(50.8825230539854,248.366092044717,31.9213203435596)) ;
#79739=CARTESIAN_POINT('',(52.8601564199237,248.366092044717,31.8013203435596)) ;
#79740=CARTESIAN_POINT('Ctrl Pts',(50.8825230539854,248.366092044717,31.9213203435596)) ;
#79741=CARTESIAN_POINT('Ctrl Pts',(50.8825230539854,248.366092044717,31.5613203435596)) ;
#79742=CARTESIAN_POINT('Ctrl Pts',(50.7740455687365,248.364939378322,31.9213203435596)) ;
#79743=CARTESIAN_POINT('Ctrl Pts',(50.7740455687365,248.364939378322,31.5613203435596)) ;
#79744=CARTESIAN_POINT('Ctrl Pts',(50.5817028363738,248.362895571688,31.9213203435596)) ;
#79745=CARTESIAN_POINT('Ctrl Pts',(50.5817028363738,248.362895571688,31.5613203435596)) ;
#79746=CARTESIAN_POINT('Ctrl Pts',(50.3959737706177,248.313820081291,31.9213203435596)) ;
#79747=CARTESIAN_POINT('Ctrl Pts',(50.3959737706177,248.313820081291,31.5613203435596)) ;
#79748=CARTESIAN_POINT('Ctrl Pts',(50.3149922133501,248.292422193891,31.9213203435596)) ;
#79749=CARTESIAN_POINT('Ctrl Pts',(50.3149922133501,248.292422193891,31.5613203435596)) ;
#79750=CARTESIAN_POINT('',(50.3149922133501,248.292422193891,31.8013203435596)) ;
#79751=CARTESIAN_POINT('',(50.3149922133501,248.292422193891,31.9213203435596)) ;
#79752=CARTESIAN_POINT('Ctrl Pts',(50.8825230530914,248.366092044866,31.8013203435596)) ;
#79753=CARTESIAN_POINT('Ctrl Pts',(50.780063617307,248.365003768851,31.8013203435596)) ;
#79754=CARTESIAN_POINT('Ctrl Pts',(50.6723937595897,248.364790853518,31.8013203435596)) ;
#79755=CARTESIAN_POINT('Ctrl Pts',(50.471719498392,248.334437936584,31.8013203435596)) ;
#79756=CARTESIAN_POINT('Ctrl Pts',(50.3915513141507,248.312651528491,31.8013203435596)) ;
#79757=CARTESIAN_POINT('Ctrl Pts',(50.31499221335,248.292422193891,31.8013203435596)) ;
#79758=CARTESIAN_POINT('Origin',(50.7870249950405,248.600744057303,31.6213203435596)) ;
#79759=CARTESIAN_POINT('',(51.4064264123735,248.704482161408,31.6213203435596)) ;
#79760=CARTESIAN_POINT('',(52.1403128398474,248.704482161408,31.6213203435596)) ;
#79761=CARTESIAN_POINT('',(51.0967112553384,248.704482161408,31.6213203435596)) ;
#79762=CARTESIAN_POINT('',(51.086156364446,248.725988135576,31.6213203435596)) ;
#79763=CARTESIAN_POINT('Ctrl Pts',(51.086156364446,248.725988135576,31.6213203435596)) ;
#79764=CARTESIAN_POINT('Ctrl Pts',(51.0891401619064,248.72557110151,31.6213203435596)) ;
#79765=CARTESIAN_POINT('Ctrl Pts',(51.0921240529548,248.725154332015,31.6213203435596)) ;
#79766=CARTESIAN_POINT('Ctrl Pts',(51.1368100661075,248.718902921604,31.6213203435596)) ;
#79767=CARTESIAN_POINT('Ctrl Pts',(51.1785415671225,248.713138013086,31.6213203435596)) ;
#79768=CARTESIAN_POINT('Ctrl Pts',(51.2823351634085,248.704548527333,31.6213203435596)) ;
#79769=CARTESIAN_POINT('Ctrl Pts',(51.3444132215067,248.704452338598,31.6213203435597)) ;
#79770=CARTESIAN_POINT('Ctrl Pts',(51.4064264123667,248.70448216142,31.6213203435597)) ;
#79771=CARTESIAN_POINT('',(50.803890188879,248.850701676295,31.6213203435596)) ;
#79772=CARTESIAN_POINT('Ctrl Pts',(50.803890188879,248.850701676295,31.6213203435596)) ;
#79773=CARTESIAN_POINT('Ctrl Pts',(50.8057995745649,248.849549687667,31.6213203435596)) ;
#79774=CARTESIAN_POINT('Ctrl Pts',(50.807709533127,248.848398088001,31.6213203435596)) ;
#79775=CARTESIAN_POINT('Ctrl Pts',(50.8526791620758,248.821240949726,31.6213203435597)) ;
#79776=CARTESIAN_POINT('Ctrl Pts',(50.8960447320484,248.795457119086,31.6213203435597)) ;
#79777=CARTESIAN_POINT('Ctrl Pts',(50.9859328579063,248.756098193207,31.6213203435597)) ;
#79778=CARTESIAN_POINT('Ctrl Pts',(51.0317272198324,248.742164050894,31.6213203435597)) ;
#79779=CARTESIAN_POINT('Ctrl Pts',(51.0803807937155,248.727707582416,31.6213203435597)) ;
#79780=CARTESIAN_POINT('Ctrl Pts',(51.0832686016586,248.726847429988,31.6213203435597)) ;
#79781=CARTESIAN_POINT('Ctrl Pts',(51.086156364446,248.725988135576,31.6213203435597)) ;
#79782=CARTESIAN_POINT('',(50.5065284460866,249.143989702353,31.6213203435597)) ;
#79783=CARTESIAN_POINT('Ctrl Pts',(50.5065286369161,249.143989458401,31.6213203435597)) ;
#79784=CARTESIAN_POINT('Ctrl Pts',(50.5069608349978,249.14344985097,31.6213203435597)) ;
#79785=CARTESIAN_POINT('Ctrl Pts',(50.5073932243977,249.142910226211,31.6213203435597)) ;
#79786=CARTESIAN_POINT('Ctrl Pts',(50.556272300514,249.081846646474,31.62132034356)) ;
#79787=CARTESIAN_POINT('Ctrl Pts',(50.6051720569295,249.021342538492,31.6213203435597)) ;
#79788=CARTESIAN_POINT('Ctrl Pts',(50.7045314789452,248.927144579668,31.6213203435597)) ;
#79789=CARTESIAN_POINT('Ctrl Pts',(50.7515320882953,248.890838723369,31.6213203435597)) ;
#79790=CARTESIAN_POINT('Ctrl Pts',(50.8003512733757,248.853416193082,31.6213203435596)) ;
#79791=CARTESIAN_POINT('Ctrl Pts',(50.8021206938697,248.852058742774,31.6213203435597)) ;
#79792=CARTESIAN_POINT('Ctrl Pts',(50.803890188879,248.850701676295,31.6213203435597)) ;
#79793=CARTESIAN_POINT('',(50.1184962383157,249.703743076409,31.6213203435596)) ;
#79794=CARTESIAN_POINT('Ctrl Pts',(50.1184962401253,249.703743073639,31.6213203435596)) ;
#79795=CARTESIAN_POINT('Ctrl Pts',(50.1885559277244,249.595500406139,31.6213203435596)) ;
#79796=CARTESIAN_POINT('Ctrl Pts',(50.2586477088752,249.487244711046,31.6213203435595)) ;
#79797=CARTESIAN_POINT('Ctrl Pts',(50.3887608735185,249.301944161957,31.6213203435596)) ;
#79798=CARTESIAN_POINT('Ctrl Pts',(50.4470208542166,249.223788058288,31.6213203435592)) ;
#79799=CARTESIAN_POINT('Ctrl Pts',(50.5057014968488,249.145098643882,31.6213203435596)) ;
#79800=CARTESIAN_POINT('Ctrl Pts',(50.5061149650076,249.144544163959,31.6213203435596)) ;
#79801=CARTESIAN_POINT('Ctrl Pts',(50.5065284346353,249.143989693814,31.6213203435596)) ;
#79802=CARTESIAN_POINT('',(49.6242728881931,250.480744087106,31.6213203435596)) ;
#79803=CARTESIAN_POINT('',(50.1997327628534,249.576025797013,31.6213203435596)) ;
#79804=CARTESIAN_POINT('',(49.2435109302601,250.480744087106,31.6213203435596)) ;
#79805=CARTESIAN_POINT('',(49.9057153088118,250.480744087106,31.6213203435596)) ;
#79806=CARTESIAN_POINT('',(49.8203579156189,249.578148362944,31.6213203435596)) ;
#79807=CARTESIAN_POINT('',(50.182743804609,249.011121144029,31.6213203435596)) ;
#79808=CARTESIAN_POINT('',(50.2391705625565,249.070003642667,31.6213203435604)) ;
#79809=CARTESIAN_POINT('Ctrl Pts',(50.2391707426563,249.070004176103,31.6213203435596)) ;
#79810=CARTESIAN_POINT('Ctrl Pts',(50.1657687234013,249.143332160444,31.6213203435596)) ;
#79811=CARTESIAN_POINT('Ctrl Pts',(50.0923185561359,249.216754385207,31.6213203435596)) ;
#79812=CARTESIAN_POINT('Ctrl Pts',(49.9511520237043,249.385651900106,31.6213203435596)) ;
#79813=CARTESIAN_POINT('Ctrl Pts',(49.885777159574,249.482014947007,31.6213203435596)) ;
#79814=CARTESIAN_POINT('Ctrl Pts',(49.8203580221144,249.578148200324,31.6213203435596)) ;
#79815=CARTESIAN_POINT('',(50.8634509060979,248.724567452152,31.6213203435596)) ;
#79816=CARTESIAN_POINT('Ctrl Pts',(50.8634509060979,248.724567452152,31.6213203435597)) ;
#79817=CARTESIAN_POINT('Ctrl Pts',(50.752878376055,248.779202490392,31.6213203435597)) ;
#79818=CARTESIAN_POINT('Ctrl Pts',(50.6422811339546,248.833795616323,31.6213203435596)) ;
#79819=CARTESIAN_POINT('Ctrl Pts',(50.4731253324676,248.917460196317,31.6213203435596)) ;
#79820=CARTESIAN_POINT('Ctrl Pts',(50.4140730966128,248.946294536072,31.6213203435596)) ;
#79821=CARTESIAN_POINT('Ctrl Pts',(50.3173047320902,249.008815217813,31.6213203435596)) ;
#79822=CARTESIAN_POINT('Ctrl Pts',(50.2782046295083,249.039403431305,31.6213203435596)) ;
#79823=CARTESIAN_POINT('Ctrl Pts',(50.239170406004,249.070003442965,31.6213203435596)) ;
#79824=CARTESIAN_POINT('',(49.7134657448932,248.324869300773,31.6213203435596)) ;
#79825=CARTESIAN_POINT('Ctrl Pts',(49.7134669918129,248.324871302986,31.6213203435596)) ;
#79826=CARTESIAN_POINT('Ctrl Pts',(49.8135354254198,248.404517214071,31.6213203435596)) ;
#79827=CARTESIAN_POINT('Ctrl Pts',(49.9140472672828,248.485001685424,31.6213203435596)) ;
#79828=CARTESIAN_POINT('Ctrl Pts',(50.1766164005556,248.610148341557,31.6213203435597)) ;
#79829=CARTESIAN_POINT('Ctrl Pts',(50.339328262466,248.63513713406,31.6213203435596)) ;
#79830=CARTESIAN_POINT('Ctrl Pts',(50.6193644682054,248.68318651908,31.6213203435596)) ;
#79831=CARTESIAN_POINT('Ctrl Pts',(50.7413810446874,248.703796823408,31.6213203435596)) ;
#79832=CARTESIAN_POINT('Ctrl Pts',(50.863450906098,248.724567452152,31.6213203435596)) ;
#79833=CARTESIAN_POINT('',(49.4721211893692,247.691149925186,31.6213203435611)) ;
#79834=CARTESIAN_POINT('Ctrl Pts',(49.472122022277,247.691150967144,31.6213203435596)) ;
#79835=CARTESIAN_POINT('Ctrl Pts',(49.4776322982804,247.761009018444,31.6213203435596)) ;
#79836=CARTESIAN_POINT('Ctrl Pts',(49.4868918774019,247.879515131177,31.6213203435596)) ;
#79837=CARTESIAN_POINT('Ctrl Pts',(49.5146718619417,247.995378904774,31.6213203435596)) ;
#79838=CARTESIAN_POINT('Ctrl Pts',(49.549547538703,248.084463228595,31.6213203435596)) ;
#79839=CARTESIAN_POINT('Ctrl Pts',(49.6044221987356,248.183416394021,31.6213203435596)) ;
#79840=CARTESIAN_POINT('Ctrl Pts',(49.6732807190579,248.272880146134,31.6213203435596)) ;
#79841=CARTESIAN_POINT('Ctrl Pts',(49.7134670322841,248.324868305633,31.6213203435596)) ;
#79842=CARTESIAN_POINT('',(49.6210141597778,247.151691936914,31.6213203435596)) ;
#79843=CARTESIAN_POINT('Ctrl Pts',(49.6210131682005,247.151692804282,31.6213203435596)) ;
#79844=CARTESIAN_POINT('Ctrl Pts',(49.5779432602701,247.234817978226,31.6213203435596)) ;
#79845=CARTESIAN_POINT('Ctrl Pts',(49.5342097952782,247.318188901882,31.6213203435596)) ;
#79846=CARTESIAN_POINT('Ctrl Pts',(49.4834370857315,247.500442371379,31.6213203435596)) ;
#79847=CARTESIAN_POINT('Ctrl Pts',(49.478005366162,247.596089312949,31.6213203435596)) ;
#79848=CARTESIAN_POINT('Ctrl Pts',(49.4721207423776,247.691149897516,31.6213203435596)) ;
#79849=CARTESIAN_POINT('',(50.0058124410862,246.822526614227,31.6213203435597)) ;
#79850=CARTESIAN_POINT('Ctrl Pts',(50.005809812189,246.822528105688,31.6213203435597)) ;
#79851=CARTESIAN_POINT('Ctrl Pts',(49.9776833689163,246.836265985231,31.6213203435597)) ;
#79852=CARTESIAN_POINT('Ctrl Pts',(49.9026192503807,246.873207876842,31.6213203435597)) ;
#79853=CARTESIAN_POINT('Ctrl Pts',(49.8301799972564,246.915958463683,31.6213203435596)) ;
#79854=CARTESIAN_POINT('Ctrl Pts',(49.7621487599861,246.973100389465,31.6213203435596)) ;
#79855=CARTESIAN_POINT('Ctrl Pts',(49.701845797924,247.037610514595,31.6213203435597)) ;
#79856=CARTESIAN_POINT('Ctrl Pts',(49.6508881669957,247.109484107848,31.6213203435596)) ;
#79857=CARTESIAN_POINT('Ctrl Pts',(49.6210149532587,247.151692498505,31.6213203435596)) ;
#79858=CARTESIAN_POINT('',(50.7765817870421,246.720744026659,31.6213203435596)) ;
#79859=CARTESIAN_POINT('Ctrl Pts',(50.7765817856215,246.720744025627,31.6213203435596)) ;
#79860=CARTESIAN_POINT('Ctrl Pts',(50.625471196441,246.721928462813,31.6213203435596)) ;
#79861=CARTESIAN_POINT('Ctrl Pts',(50.4737979877614,246.722566749351,31.6213203435597)) ;
#79862=CARTESIAN_POINT('Ctrl Pts',(50.2164851948485,246.763827191512,31.6213203435597)) ;
#79863=CARTESIAN_POINT('Ctrl Pts',(50.1110650243439,246.793152996729,31.6213203435597)) ;
#79864=CARTESIAN_POINT('Ctrl Pts',(50.005812342985,246.822526262703,31.6213203435597)) ;
#79865=CARTESIAN_POINT('',(52.4296443674977,246.720744027501,31.6213203435596)) ;
#79866=CARTESIAN_POINT('',(51.6683346812691,246.720744027501,31.6213203435596)) ;
#79867=CARTESIAN_POINT('',(52.4296443674977,250.480744087106,31.6213203435596)) ;
#79868=CARTESIAN_POINT('',(52.4296443674977,249.600744072205,31.6213203435596)) ;
#79869=CARTESIAN_POINT('',(52.1403128398474,250.480744087106,31.6213203435596)) ;
#79870=CARTESIAN_POINT('',(51.4036689174439,250.480744087106,31.6213203435596)) ;
#79871=CARTESIAN_POINT('',(52.1403128398474,248.712613109356,31.6213203435596)) ;
#79872=CARTESIAN_POINT('Origin',(50.182743804609,249.011121144029,31.7413203435596)) ;
#79873=CARTESIAN_POINT('',(49.0244056225832,250.600744087106,31.7413203435596)) ;
#79874=CARTESIAN_POINT('Origin',(49.2435109302601,250.480744087106,31.7413203435596)) ;
#79875=CARTESIAN_POINT('',(49.7201766015108,249.512067336446,31.7413203435596)) ;
#79876=CARTESIAN_POINT('',(50.0816298410385,248.946499426541,31.7413203435596)) ;
#79877=CARTESIAN_POINT('Ctrl Pts',(49.8203578030133,249.578148522292,31.6213203435596)) ;
#79878=CARTESIAN_POINT('Ctrl Pts',(49.8201143316048,249.57798792436,31.6213203435596)) ;
#79879=CARTESIAN_POINT('Ctrl Pts',(49.8198708575707,249.57782732467,31.6213214476887)) ;
#79880=CARTESIAN_POINT('Ctrl Pts',(49.8120344278958,249.572658275908,31.6213924401153)) ;
#79881=CARTESIAN_POINT('Ctrl Pts',(49.804486837198,249.567679673608,31.6225275324167)) ;
#79882=CARTESIAN_POINT('Ctrl Pts',(49.791651457411,249.559212971364,31.6262185924614)) ;
#79883=CARTESIAN_POINT('Ctrl Pts',(49.786279037641,249.555669070629,31.6283381657329)) ;
#79884=CARTESIAN_POINT('Ctrl Pts',(49.7740832540178,249.547624217164,31.6345403110037)) ;
#79885=CARTESIAN_POINT('Ctrl Pts',(49.767470915909,249.54326245926,31.6390055724476)) ;
#79886=CARTESIAN_POINT('Ctrl Pts',(49.7601937918778,249.538462793976,31.6453557245753)) ;
#79887=CARTESIAN_POINT('Ctrl Pts',(49.7590266040823,249.537692991468,31.646424002123)) ;
#79888=CARTESIAN_POINT('Ctrl Pts',(49.7547988343126,249.534904730099,31.6504832283805)) ;
#79889=CARTESIAN_POINT('Ctrl Pts',(49.7518693497122,249.532972909003,31.6536742656277)) ;
#79890=CARTESIAN_POINT('Ctrl Pts',(49.7437891211446,249.527644641772,31.663605970272)) ;
#79891=CARTESIAN_POINT('Ctrl Pts',(49.7391293356128,249.524572046805,31.6708380022079)) ;
#79892=CARTESIAN_POINT('Ctrl Pts',(49.7323690685834,249.520113636147,31.6841034424277)) ;
#79893=CARTESIAN_POINT('Ctrl Pts',(49.7299190041598,249.518497551385,31.6898732056734)) ;
#79894=CARTESIAN_POINT('Ctrl Pts',(49.7249579883231,249.515224496342,31.7042366795402)) ;
#79895=CARTESIAN_POINT('Ctrl Pts',(49.7228443575224,249.513829279031,31.712944490313)) ;
#79896=CARTESIAN_POINT('Ctrl Pts',(49.720654622348,249.512383268816,31.7282514461642)) ;
#79897=CARTESIAN_POINT('Ctrl Pts',(49.7201766015108,249.512067336446,31.7347662286955)) ;
#79898=CARTESIAN_POINT('Ctrl Pts',(49.7201766015108,249.512067336446,31.7413203435596)) ;
#79899=CARTESIAN_POINT('Origin',(49.9057153088118,250.480744087106,31.7413203435596)) ;
#79900=CARTESIAN_POINT('',(49.6901629806574,250.600744087106,31.7413203435596)) ;
#79901=CARTESIAN_POINT('Origin',(49.6242728881931,250.480744087106,31.7413203435596)) ;
#79902=CARTESIAN_POINT('',(49.9057153088118,250.600744087106,31.7413203435596)) ;
#79903=CARTESIAN_POINT('Origin',(50.1997327628534,249.576025797013,31.7413203435596)) ;
#79904=CARTESIAN_POINT('',(50.2194942457775,249.76854761595,31.7413203435596)) ;
#79905=CARTESIAN_POINT('Ctrl Pts',(50.1184962360783,249.703743079888,31.6213203435596)) ;
#79906=CARTESIAN_POINT('Ctrl Pts',(50.1187416948551,249.703900576469,31.6213203435596)) ;
#79907=CARTESIAN_POINT('Ctrl Pts',(50.1189871559203,249.704058075343,31.6213214476896)) ;
#79908=CARTESIAN_POINT('Ctrl Pts',(50.1268875814148,249.709127312317,31.6213924404081)) ;
#79909=CARTESIAN_POINT('Ctrl Pts',(50.134496779585,249.714009714011,31.6225275410102)) ;
#79910=CARTESIAN_POINT('Ctrl Pts',(50.1474348105249,249.722311369703,31.6262179993372)) ;
#79911=CARTESIAN_POINT('Ctrl Pts',(50.1528490540415,249.725785419901,31.6283365564217)) ;
#79912=CARTESIAN_POINT('Ctrl Pts',(50.1651429552605,249.733673783677,31.634536887502)) ;
#79913=CARTESIAN_POINT('Ctrl Pts',(50.1718096792711,249.73795147265,31.6390018254195)) ;
#79914=CARTESIAN_POINT('Ctrl Pts',(50.1791479853649,249.742659914759,31.6453529319083)) ;
#79915=CARTESIAN_POINT('Ctrl Pts',(50.1803262224953,249.743415895318,31.6464225668027)) ;
#79916=CARTESIAN_POINT('Ctrl Pts',(50.1845881438841,249.746150400814,31.6504816500711)) ;
#79917=CARTESIAN_POINT('Ctrl Pts',(50.1875398130984,249.748044174978,31.6536708439172)) ;
#79918=CARTESIAN_POINT('Ctrl Pts',(50.195684363488,249.753269627988,31.6636000631244)) ;
#79919=CARTESIAN_POINT('Ctrl Pts',(50.2003820835136,249.756283589114,31.6708316856961)) ;
#79920=CARTESIAN_POINT('Ctrl Pts',(50.2071983400128,249.760656974874,31.684097470937)) ;
#79921=CARTESIAN_POINT('Ctrl Pts',(50.2096690460319,249.762242278695,31.689868116927)) ;
#79922=CARTESIAN_POINT('Ctrl Pts',(50.2146716460624,249.765452344316,31.7042327086333)) ;
#79923=CARTESIAN_POINT('Ctrl Pts',(50.2168031754755,249.766820304159,31.7129407270407)) ;
#79924=CARTESIAN_POINT('Ctrl Pts',(50.219011933072,249.768237978459,31.7282490558558)) ;
#79925=CARTESIAN_POINT('Ctrl Pts',(50.2194942440176,249.76854761887,31.7347650345167)) ;
#79926=CARTESIAN_POINT('Ctrl Pts',(50.2194942440175,249.76854761887,31.7413203435596)) ;
#79927=CARTESIAN_POINT('',(50.3009858231264,249.640429351149,31.7413203435596)) ;
#79928=CARTESIAN_POINT('Ctrl Pts',(50.2192360308921,249.768946559407,31.7413203435596)) ;
#79929=CARTESIAN_POINT('Ctrl Pts',(50.2892957198384,249.660703889824,31.7413203435596)) ;
#79930=CARTESIAN_POINT('Ctrl Pts',(50.3585729066663,249.55375538464,31.7413203435595)) ;
#79931=CARTESIAN_POINT('Ctrl Pts',(50.4856696244485,249.372752864996,31.7413203435596)) ;
#79932=CARTESIAN_POINT('Ctrl Pts',(50.543217787302,249.295522367444,31.7413203435593)) ;
#79933=CARTESIAN_POINT('Ctrl Pts',(50.6018996488782,249.216833692745,31.7413203435597)) ;
#79934=CARTESIAN_POINT('Ctrl Pts',(50.6023131730112,249.216279125981,31.7413203435596)) ;
#79935=CARTESIAN_POINT('Ctrl Pts',(50.6027267043398,249.215724573099,31.7413203435596)) ;
#79936=CARTESIAN_POINT('Ctrl Pts',(50.2192360308921,249.768946559407,31.7054164275186)) ;
#79937=CARTESIAN_POINT('Ctrl Pts',(50.2892957198384,249.660703889824,31.7054164275186)) ;
#79938=CARTESIAN_POINT('Ctrl Pts',(50.3585729066663,249.55375538464,31.7054164275185)) ;
#79939=CARTESIAN_POINT('Ctrl Pts',(50.4856696244485,249.372752864996,31.7054164275186)) ;
#79940=CARTESIAN_POINT('Ctrl Pts',(50.543217787302,249.295522367444,31.7054164275182)) ;
#79941=CARTESIAN_POINT('Ctrl Pts',(50.6018996488782,249.216833692745,31.7054164275186)) ;
#79942=CARTESIAN_POINT('Ctrl Pts',(50.6023131730112,249.216279125981,31.7054164275186)) ;
#79943=CARTESIAN_POINT('Ctrl Pts',(50.6027267043398,249.215724573099,31.7054164275186)) ;
#79944=CARTESIAN_POINT('Ctrl Pts',(50.1939177594495,249.752559396851,31.6432843216851)) ;
#79945=CARTESIAN_POINT('Ctrl Pts',(50.2639758267822,249.644313855627,31.6432843216851)) ;
#79946=CARTESIAN_POINT('Ctrl Pts',(50.3334588863795,249.537039133955,31.643284321685)) ;
#79947=CARTESIAN_POINT('Ctrl Pts',(50.4613142664604,249.354956858061,31.6432843216851)) ;
#79948=CARTESIAN_POINT('Ctrl Pts',(50.5190399474795,249.277492812335,31.6432843216847)) ;
#79949=CARTESIAN_POINT('Ctrl Pts',(50.5777228825355,249.198805024834,31.6432843216851)) ;
#79950=CARTESIAN_POINT('Ctrl Pts',(50.5781362671757,249.198250352243,31.6432843216851)) ;
#79951=CARTESIAN_POINT('Ctrl Pts',(50.5785498711154,249.197695854323,31.6432843216851)) ;
#79952=CARTESIAN_POINT('Ctrl Pts',(50.1411021931731,249.718374706478,31.6213203435596)) ;
#79953=CARTESIAN_POINT('Ctrl Pts',(50.2111609256163,249.610130343067,31.6213203435596)) ;
#79954=CARTESIAN_POINT('Ctrl Pts',(50.2810705890642,249.502169342483,31.6213203435595)) ;
#79955=CARTESIAN_POINT('Ctrl Pts',(50.4105071949428,249.31783352678,31.6213203435596)) ;
#79956=CARTESIAN_POINT('Ctrl Pts',(50.4686066310802,249.239884584998,31.6213203435592)) ;
#79957=CARTESIAN_POINT('Ctrl Pts',(50.5272883998386,249.161195917641,31.6213203435596)) ;
#79958=CARTESIAN_POINT('Ctrl Pts',(50.5277018452843,249.160641291024,31.6213203435596)) ;
#79959=CARTESIAN_POINT('Ctrl Pts',(50.5281154194423,249.160086770561,31.6213203435596)) ;
#79960=CARTESIAN_POINT('Ctrl Pts',(50.1184962360798,249.703743079889,31.6213203435596)) ;
#79961=CARTESIAN_POINT('Ctrl Pts',(50.1885559250262,249.595500410306,31.6213203435596)) ;
#79962=CARTESIAN_POINT('Ctrl Pts',(50.258647707449,249.487244713078,31.6213203435595)) ;
#79963=CARTESIAN_POINT('Ctrl Pts',(50.3887608735185,249.301944161957,31.6213203435596)) ;
#79964=CARTESIAN_POINT('Ctrl Pts',(50.4470208542166,249.223788058288,31.6213203435592)) ;
#79965=CARTESIAN_POINT('Ctrl Pts',(50.5057015585495,249.145098561143,31.6213203435596)) ;
#79966=CARTESIAN_POINT('Ctrl Pts',(50.506115088408,249.144543998473,31.6213203435596)) ;
#79967=CARTESIAN_POINT('Ctrl Pts',(50.5065286197366,249.14398944559,31.6213203435596)) ;
#79968=CARTESIAN_POINT('',(50.6014860873806,249.217388210622,31.7413203435596)) ;
#79969=CARTESIAN_POINT('Ctrl Pts',(50.5065282662,249.143989955527,31.6213203435597)) ;
#79970=CARTESIAN_POINT('Ctrl Pts',(50.5067587814614,249.144168655837,31.6213203436138)) ;
#79971=CARTESIAN_POINT('Ctrl Pts',(50.5069898102017,249.144346708618,31.6213214476891)) ;
#79972=CARTESIAN_POINT('Ctrl Pts',(50.507220589837,249.144525091037,31.6213236533711)) ;
#79973=CARTESIAN_POINT('Ctrl Pts',(50.5144175329847,249.150088008785,31.6213924383321)) ;
#79974=CARTESIAN_POINT('Ctrl Pts',(50.5215715307724,249.155617632913,31.6225274810686)) ;
#79975=CARTESIAN_POINT('Ctrl Pts',(50.5285466406673,249.161008894249,31.6246435392332)) ;
#79976=CARTESIAN_POINT('Ctrl Pts',(50.5337389459037,249.165022175028,31.6262187430729)) ;
#79977=CARTESIAN_POINT('Ctrl Pts',(50.5388325053053,249.168959069177,31.628338843696)) ;
#79978=CARTESIAN_POINT('Ctrl Pts',(50.5437677752371,249.172773650262,31.6309868527295)) ;
#79979=CARTESIAN_POINT('Ctrl Pts',(50.5503934802315,249.177894806612,31.634541861254)) ;
#79980=CARTESIAN_POINT('Ctrl Pts',(50.5566609773773,249.182739119391,31.6390071822895)) ;
#79981=CARTESIAN_POINT('Ctrl Pts',(50.5624328792937,249.187201020017,31.6443215166813)) ;
#79982=CARTESIAN_POINT('Ctrl Pts',(50.5635573448131,249.18807027481,31.6453568401965)) ;
#79983=CARTESIAN_POINT('Ctrl Pts',(50.5646629450614,249.188924974179,31.6464245294253)) ;
#79984=CARTESIAN_POINT('Ctrl Pts',(50.5657485650742,249.189764263626,31.6475243300193)) ;
#79985=CARTESIAN_POINT('Ctrl Pts',(50.5686699459928,249.192022774103,31.6504838705877)) ;
#79986=CARTESIAN_POINT('Ctrl Pts',(50.5714468197053,249.194169827638,31.6536757758731)) ;
#79987=CARTESIAN_POINT('Ctrl Pts',(50.5740702737092,249.196198328858,31.6570786924021)) ;
#79988=CARTESIAN_POINT('Ctrl Pts',(50.5791044212708,249.200090821145,31.6636085511004)) ;
#79989=CARTESIAN_POINT('Ctrl Pts',(50.5835198746397,249.203505131949,31.670840665461)) ;
#79990=CARTESIAN_POINT('Ctrl Pts',(50.5872694481144,249.206403957949,31.6786045970734)) ;
#79991=CARTESIAN_POINT('Ctrl Pts',(50.5899263174098,249.208458005388,31.684105956535)) ;
#79992=CARTESIAN_POINT('Ctrl Pts',(50.5922483559534,249.210252861051,31.6898754635384)) ;
#79993=CARTESIAN_POINT('Ctrl Pts',(50.5942080262981,249.211767237315,31.6958607981639)) ;
#79994=CARTESIAN_POINT('Ctrl Pts',(50.5969510272122,249.213886948668,31.7042386247684)) ;
#79995=CARTESIAN_POINT('Ctrl Pts',(50.5989553811672,249.215434921791,31.7129463762652)) ;
#79996=CARTESIAN_POINT('Ctrl Pts',(50.6001611416934,249.216365729467,31.7218322584633)) ;
#79997=CARTESIAN_POINT('Ctrl Pts',(50.6009919855187,249.217007113716,31.7279551827062)) ;
#79998=CARTESIAN_POINT('Ctrl Pts',(50.601442996467,249.217354970191,31.7341633653977)) ;
#79999=CARTESIAN_POINT('Ctrl Pts',(50.6014830955948,249.217385899284,31.7404096300915)) ;
#80000=CARTESIAN_POINT('Ctrl Pts',(50.6014850438655,249.217387402016,31.7407131133612)) ;
#80001=CARTESIAN_POINT('Ctrl Pts',(50.6014860200994,249.217388154977,31.7410166863487)) ;
#80002=CARTESIAN_POINT('Ctrl Pts',(50.6014860200994,249.217388154977,31.7413203435596)) ;
#80003=CARTESIAN_POINT('Ctrl Pts',(50.6014861078465,249.217388225182,31.7413203435596)) ;
#80004=CARTESIAN_POINT('Ctrl Pts',(50.543217787302,249.295522367444,31.7413203435593)) ;
#80005=CARTESIAN_POINT('Ctrl Pts',(50.4856696244485,249.372752864996,31.7413203435596)) ;
#80006=CARTESIAN_POINT('Ctrl Pts',(50.3586618302853,249.553628745657,31.7413203435595)) ;
#80007=CARTESIAN_POINT('Ctrl Pts',(50.2894659462689,249.660441111302,31.7413203435596)) ;
#80008=CARTESIAN_POINT('Ctrl Pts',(50.2194942440175,249.76854761887,31.7413203435596)) ;
#80009=CARTESIAN_POINT('Ctrl Pts',(50.6001891375754,249.219007527002,31.7413203435596)) ;
#80010=CARTESIAN_POINT('Ctrl Pts',(50.6006214646902,249.218467758338,31.7413203435596)) ;
#80011=CARTESIAN_POINT('Ctrl Pts',(50.6010540649099,249.217928043864,31.7413203435596)) ;
#80012=CARTESIAN_POINT('Ctrl Pts',(50.6499195763086,249.156852387871,31.7413203435601)) ;
#80013=CARTESIAN_POINT('Ctrl Pts',(50.695202994675,249.10133535881,31.7413203435597)) ;
#80014=CARTESIAN_POINT('Ctrl Pts',(50.7813866081462,249.019639600231,31.7413203435597)) ;
#80015=CARTESIAN_POINT('Ctrl Pts',(50.8245550336637,248.986049007095,31.7413203435597)) ;
#80016=CARTESIAN_POINT('Ctrl Pts',(50.8733785425078,248.948637433444,31.7413203435596)) ;
#80017=CARTESIAN_POINT('Ctrl Pts',(50.8751478527577,248.947279717694,31.7413203435596)) ;
#80018=CARTESIAN_POINT('Ctrl Pts',(50.876917347767,248.945922651215,31.7413203435596)) ;
#80019=CARTESIAN_POINT('Ctrl Pts',(50.6001891375754,249.219007527002,31.7054164275186)) ;
#80020=CARTESIAN_POINT('Ctrl Pts',(50.6006214646902,249.218467758338,31.7054164275186)) ;
#80021=CARTESIAN_POINT('Ctrl Pts',(50.6010540649099,249.217928043864,31.7054164275186)) ;
#80022=CARTESIAN_POINT('Ctrl Pts',(50.6499195763086,249.156852387871,31.7054164275191)) ;
#80023=CARTESIAN_POINT('Ctrl Pts',(50.695202994675,249.10133535881,31.7054164275187)) ;
#80024=CARTESIAN_POINT('Ctrl Pts',(50.7813866081462,249.019639600231,31.7054164275187)) ;
#80025=CARTESIAN_POINT('Ctrl Pts',(50.8245550336637,248.986049007095,31.7054164275187)) ;
#80026=CARTESIAN_POINT('Ctrl Pts',(50.8733785425078,248.948637433444,31.7054164275186)) ;
#80027=CARTESIAN_POINT('Ctrl Pts',(50.8751478527577,248.947279717694,31.7054164275186)) ;
#80028=CARTESIAN_POINT('Ctrl Pts',(50.876917347767,248.945922651215,31.7054164275186)) ;
#80029=CARTESIAN_POINT('Ctrl Pts',(50.5766499626794,249.200153850869,31.6432843195571)) ;
#80030=CARTESIAN_POINT('Ctrl Pts',(50.5770818425322,249.19961354785,31.6432843195571)) ;
#80031=CARTESIAN_POINT('Ctrl Pts',(50.5775153094751,249.199074856023,31.6432843195571)) ;
#80032=CARTESIAN_POINT('Ctrl Pts',(50.6263655239759,249.13798899133,31.6432843195575)) ;
#80033=CARTESIAN_POINT('Ctrl Pts',(50.6725751704915,249.081223960805,31.6432843195572)) ;
#80034=CARTESIAN_POINT('Ctrl Pts',(50.7620696300964,248.996395824763,31.6432843195572)) ;
#80035=CARTESIAN_POINT('Ctrl Pts',(50.8061966649443,248.962103736337,31.6432843195572)) ;
#80036=CARTESIAN_POINT('Ctrl Pts',(50.8550255073703,248.924707064648,31.6432843195571)) ;
#80037=CARTESIAN_POINT('Ctrl Pts',(50.8567939979677,248.9233475544,31.6432843195571)) ;
#80038=CARTESIAN_POINT('Ctrl Pts',(50.8585639123037,248.921991389961,31.6432843195571)) ;
#80039=CARTESIAN_POINT('Ctrl Pts',(50.5275457036156,249.16082384881,31.6213203435597)) ;
#80040=CARTESIAN_POINT('Ctrl Pts',(50.5279777669084,249.160283764952,31.6213203435597)) ;
#80041=CARTESIAN_POINT('Ctrl Pts',(50.5284108272628,249.15974460881,31.6213203435597)) ;
#80042=CARTESIAN_POINT('Ctrl Pts',(50.5772759064884,249.098670406059,31.62132034356)) ;
#80043=CARTESIAN_POINT('Ctrl Pts',(50.6253743971568,249.039288562501,31.6213203435597)) ;
#80044=CARTESIAN_POINT('Ctrl Pts',(50.721776854263,248.947901823281,31.6213203435597)) ;
#80045=CARTESIAN_POINT('Ctrl Pts',(50.7679148643503,248.912194012504,31.6213203435597)) ;
#80046=CARTESIAN_POINT('Ctrl Pts',(50.8167388067278,248.874784355228,31.6213203435596)) ;
#80047=CARTESIAN_POINT('Ctrl Pts',(50.8185077026595,248.873425747502,31.6213203435597)) ;
#80048=CARTESIAN_POINT('Ctrl Pts',(50.8202774450129,248.8720692131,31.6213203435597)) ;
#80049=CARTESIAN_POINT('Ctrl Pts',(50.5065282494735,249.14398994213,31.6213203435597)) ;
#80050=CARTESIAN_POINT('Ctrl Pts',(50.5069605765884,249.143450173467,31.6213203435597)) ;
#80051=CARTESIAN_POINT('Ctrl Pts',(50.5073930953378,249.142910387443,31.6213203435597)) ;
#80052=CARTESIAN_POINT('Ctrl Pts',(50.556272300514,249.081846646474,31.62132034356)) ;
#80053=CARTESIAN_POINT('Ctrl Pts',(50.6051720569295,249.021342538492,31.6213203435597)) ;
#80054=CARTESIAN_POINT('Ctrl Pts',(50.7045314789452,248.927144579668,31.6213203435597)) ;
#80055=CARTESIAN_POINT('Ctrl Pts',(50.7515320882953,248.890838723369,31.6213203435597)) ;
#80056=CARTESIAN_POINT('Ctrl Pts',(50.8003512733757,248.853416193082,31.6213203435596)) ;
#80057=CARTESIAN_POINT('Ctrl Pts',(50.8021206938697,248.852058742774,31.6213203435597)) ;
#80058=CARTESIAN_POINT('Ctrl Pts',(50.803890188879,248.850701676295,31.6213203435597)) ;
#80059=CARTESIAN_POINT('',(50.8716089055848,248.949993517828,31.7413203435596)) ;
#80060=CARTESIAN_POINT('Ctrl Pts',(50.803890188879,248.850701676295,31.6213203435596)) ;
#80061=CARTESIAN_POINT('Ctrl Pts',(50.8040547677524,248.850942988537,31.6213203435596)) ;
#80062=CARTESIAN_POINT('Ctrl Pts',(50.8042193485049,248.85118430314,31.6213214476844)) ;
#80063=CARTESIAN_POINT('Ctrl Pts',(50.8043839279318,248.851425615335,31.6213236533551)) ;
#80064=CARTESIAN_POINT('Ctrl Pts',(50.8095148172735,248.858948707318,31.6213924168237)) ;
#80065=CARTESIAN_POINT('Ctrl Pts',(50.8146154558497,248.866426990874,31.622526772514)) ;
#80066=CARTESIAN_POINT('Ctrl Pts',(50.8195890325768,248.873718590005,31.6246418150554)) ;
#80067=CARTESIAN_POINT('Ctrl Pts',(50.8233140073649,248.87917965443,31.6262258823324)) ;
#80068=CARTESIAN_POINT('Ctrl Pts',(50.8269680033362,248.884536381477,31.6283613268649)) ;
#80069=CARTESIAN_POINT('Ctrl Pts',(50.8305075891557,248.889725537149,31.6310310265338)) ;
#80070=CARTESIAN_POINT('Ctrl Pts',(50.8352281370105,248.896646024156,31.634591455829)) ;
#80071=CARTESIAN_POINT('Ctrl Pts',(50.8396936131263,248.903192690413,31.6390611416434)) ;
#80072=CARTESIAN_POINT('Ctrl Pts',(50.8438048542172,248.909222926106,31.6443797592907)) ;
#80073=CARTESIAN_POINT('Ctrl Pts',(50.8445910533297,248.910376097581,31.6453968469247)) ;
#80074=CARTESIAN_POINT('Ctrl Pts',(50.8453642565382,248.911510329011,31.6464451166949)) ;
#80075=CARTESIAN_POINT('Ctrl Pts',(50.8461236980812,248.912624528739,31.6475243338418)) ;
#80076=CARTESIAN_POINT('Ctrl Pts',(50.8482225676657,248.915703843982,31.6505069676805)) ;
#80077=CARTESIAN_POINT('Ctrl Pts',(50.8502164642029,248.918630336928,31.6537258079622)) ;
#80078=CARTESIAN_POINT('Ctrl Pts',(50.8520991972097,248.921393981,31.6571590528307)) ;
#80079=CARTESIAN_POINT('Ctrl Pts',(50.8556826308346,248.926654065705,31.6636935986531)) ;
#80080=CARTESIAN_POINT('Ctrl Pts',(50.8588251896843,248.931267858224,31.6709300524943)) ;
#80081=CARTESIAN_POINT('Ctrl Pts',(50.861494385594,248.935184014523,31.6786985561853)) ;
#80082=CARTESIAN_POINT('Ctrl Pts',(50.8633811693728,248.937952241521,31.6841899053575)) ;
#80083=CARTESIAN_POINT('Ctrl Pts',(50.8650310448257,248.940371382877,31.6899482287076)) ;
#80084=CARTESIAN_POINT('Ctrl Pts',(50.8664243752224,248.942412655009,31.695921743135)) ;
#80085=CARTESIAN_POINT('Ctrl Pts',(50.868377896629,248.9452746243,31.7042969198579)) ;
#80086=CARTESIAN_POINT('Ctrl Pts',(50.8698066535716,248.947363601716,31.7130016467406)) ;
#80087=CARTESIAN_POINT('Ctrl Pts',(50.8706661025465,248.948618375692,31.7218846188127)) ;
#80088=CARTESIAN_POINT('Ctrl Pts',(50.871243897259,248.9494619415,31.7278565082957)) ;
#80089=CARTESIAN_POINT('Ctrl Pts',(50.8715638860115,248.949927796603,31.73390960257)) ;
#80090=CARTESIAN_POINT('Ctrl Pts',(50.871604452196,248.949986859998,31.7400001290171)) ;
#80091=CARTESIAN_POINT('Ctrl Pts',(50.8716073820482,248.949991125793,31.7404400112056)) ;
#80092=CARTESIAN_POINT('Ctrl Pts',(50.8716088516813,248.949993265221,31.7408800883011)) ;
#80093=CARTESIAN_POINT('Ctrl Pts',(50.8716088516813,248.949993265221,31.7413203435596)) ;
#80094=CARTESIAN_POINT('Ctrl Pts',(50.8716089964922,248.949993748075,31.7413203435596)) ;
#80095=CARTESIAN_POINT('Ctrl Pts',(50.8566479182176,248.961467743602,31.7413203435596)) ;
#80096=CARTESIAN_POINT('Ctrl Pts',(50.8420547949466,248.972665709568,31.7413203435597)) ;
#80097=CARTESIAN_POINT('Ctrl Pts',(50.8279269473814,248.983761457176,31.7413203435597)) ;
#80098=CARTESIAN_POINT('Ctrl Pts',(50.8119753337364,248.996289556601,31.7413203435597)) ;
#80099=CARTESIAN_POINT('Ctrl Pts',(50.7966166422762,249.008687104005,31.7413203435597)) ;
#80100=CARTESIAN_POINT('Ctrl Pts',(50.7819399930112,249.021151679859,31.7413203435597)) ;
#80101=CARTESIAN_POINT('Ctrl Pts',(50.7687471099837,249.032356123616,31.7413203435597)) ;
#80102=CARTESIAN_POINT('Ctrl Pts',(50.7561040600851,249.043613412057,31.7413203435597)) ;
#80103=CARTESIAN_POINT('Ctrl Pts',(50.7440508843477,249.055041570073,31.7413203435597)) ;
#80104=CARTESIAN_POINT('Ctrl Pts',(50.7440503228543,249.05504210245,31.7413203435597)) ;
#80105=CARTESIAN_POINT('Ctrl Pts',(50.7440497613621,249.055042634828,31.7413203435597)) ;
#80106=CARTESIAN_POINT('Ctrl Pts',(50.7440491998712,249.055043167206,31.7413203435597)) ;
#80107=CARTESIAN_POINT('Ctrl Pts',(50.728296029037,249.06997954555,31.7413203435597)) ;
#80108=CARTESIAN_POINT('Ctrl Pts',(50.7128815963623,249.085842182003,31.7413203435597)) ;
#80109=CARTESIAN_POINT('Ctrl Pts',(50.6976247786594,249.102536202228,31.7413203435598)) ;
#80110=CARTESIAN_POINT('Ctrl Pts',(50.6834654512365,249.118029347848,31.7413203435598)) ;
#80111=CARTESIAN_POINT('Ctrl Pts',(50.6694423288583,249.134239033941,31.7413203435599)) ;
#80112=CARTESIAN_POINT('Ctrl Pts',(50.6553801487296,249.151057959041,31.7413203435599)) ;
#80113=CARTESIAN_POINT('Ctrl Pts',(50.6424648114365,249.166505214629,31.7413203435599)) ;
#80114=CARTESIAN_POINT('Ctrl Pts',(50.6295167370137,249.182466604728,31.7413203435598)) ;
#80115=CARTESIAN_POINT('Ctrl Pts',(50.6163691801403,249.198827039825,31.7413203435597)) ;
#80116=CARTESIAN_POINT('Ctrl Pts',(50.6114399261129,249.204960859315,31.7413203435597)) ;
#80117=CARTESIAN_POINT('Ctrl Pts',(50.6064822852617,249.21115041187,31.7413203435597)) ;
#80118=CARTESIAN_POINT('Ctrl Pts',(50.6014861116635,249.217388230071,31.7413203435596)) ;
#80119=CARTESIAN_POINT('Ctrl Pts',(50.7761110306795,246.600744027501,31.7413203435596)) ;
#80120=CARTESIAN_POINT('Ctrl Pts',(50.6248447035851,246.601930855739,31.7413203435596)) ;
#80121=CARTESIAN_POINT('Ctrl Pts',(50.4675419277232,246.602054016768,31.7413203435596)) ;
#80122=CARTESIAN_POINT('Ctrl Pts',(50.1844609819171,246.647423619666,31.7413203435596)) ;
#80123=CARTESIAN_POINT('Ctrl Pts',(50.0717748712232,246.679540434335,31.7413203435596)) ;
#80124=CARTESIAN_POINT('Ctrl Pts',(49.963014268976,246.709884602433,31.7413203435596)) ;
#80125=CARTESIAN_POINT('Ctrl Pts',(50.7761110306795,246.600744027501,31.7054164275186)) ;
#80126=CARTESIAN_POINT('Ctrl Pts',(50.6248447035851,246.601930855739,31.7054164275186)) ;
#80127=CARTESIAN_POINT('Ctrl Pts',(50.4675419277232,246.602054016768,31.7054164275186)) ;
#80128=CARTESIAN_POINT('Ctrl Pts',(50.1844609819171,246.647423619666,31.7054164275186)) ;
#80129=CARTESIAN_POINT('Ctrl Pts',(50.0717748712232,246.679540434335,31.7054164275186)) ;
#80130=CARTESIAN_POINT('Ctrl Pts',(49.963014268976,246.709884602433,31.7054164275186)) ;
#80131=CARTESIAN_POINT('Ctrl Pts',(50.7763476477493,246.630901883472,31.6432842878474)) ;
#80132=CARTESIAN_POINT('Ctrl Pts',(50.6250864771979,246.632151520329,31.6432842878474)) ;
#80133=CARTESIAN_POINT('Ctrl Pts',(50.4691644240128,246.632354151178,31.6432842878474)) ;
#80134=CARTESIAN_POINT('Ctrl Pts',(50.1915979820207,246.67682460216,31.6432842878474)) ;
#80135=CARTESIAN_POINT('Ctrl Pts',(50.0798957973197,246.708634083591,31.6432842878474)) ;
#80136=CARTESIAN_POINT('Ctrl Pts',(49.9711190288638,246.738933959252,31.6432842878474)) ;
#80137=CARTESIAN_POINT('Ctrl Pts',(50.7768412470791,246.693813225893,31.6213203435596)) ;
#80138=CARTESIAN_POINT('Ctrl Pts',(50.6255779626741,246.695037115223,31.6213203435596)) ;
#80139=CARTESIAN_POINT('Ctrl Pts',(50.4725210286059,246.695515526414,31.6213203435597)) ;
#80140=CARTESIAN_POINT('Ctrl Pts',(50.2064980096239,246.738155380204,31.6213203435597)) ;
#80141=CARTESIAN_POINT('Ctrl Pts',(50.0967962515652,246.769214864176,31.6213203435597)) ;
#80142=CARTESIAN_POINT('Ctrl Pts',(49.9880261102236,246.799532896911,31.6213203435597)) ;
#80143=CARTESIAN_POINT('Ctrl Pts',(50.7770525158595,246.720740334135,31.6213203435596)) ;
#80144=CARTESIAN_POINT('Ctrl Pts',(50.625786188765,246.721927162373,31.6213203435596)) ;
#80145=CARTESIAN_POINT('Ctrl Pts',(50.4739530550717,246.722541884105,31.6213203435597)) ;
#80146=CARTESIAN_POINT('Ctrl Pts',(50.2128774242644,246.764405702234,31.6213203435597)) ;
#80147=CARTESIAN_POINT('Ctrl Pts',(50.1040232264648,246.795126089086,31.6213203435597)) ;
#80148=CARTESIAN_POINT('Ctrl Pts',(49.9952626242177,246.825470257184,31.6213203435597)) ;
#80149=CARTESIAN_POINT('',(49.963014268976,246.709884602433,31.7413203435596)) ;
#80150=CARTESIAN_POINT('',(50.7761110306795,246.600744027501,31.7413203435596)) ;
#80151=CARTESIAN_POINT('Ctrl Pts',(49.963014268976,246.709884602433,31.7413203435596)) ;
#80152=CARTESIAN_POINT('Ctrl Pts',(50.0717748712232,246.679540434335,31.7413203435596)) ;
#80153=CARTESIAN_POINT('Ctrl Pts',(50.1844609819171,246.647423619666,31.7413203435596)) ;
#80154=CARTESIAN_POINT('Ctrl Pts',(50.4675419277232,246.602054016768,31.7413203435596)) ;
#80155=CARTESIAN_POINT('Ctrl Pts',(50.6248447035851,246.601930855739,31.7413203435596)) ;
#80156=CARTESIAN_POINT('Ctrl Pts',(50.7761110306795,246.600744027501,31.7413203435596)) ;
#80157=CARTESIAN_POINT('Origin',(50.776816088154,246.720741444438,31.7413196030361)) ;
#80158=CARTESIAN_POINT('Ctrl Pts',(50.0058152416557,246.822525453759,31.6213203435597)) ;
#80159=CARTESIAN_POINT('Ctrl Pts',(50.0057108572187,246.822251975345,31.6213203435597)) ;
#80160=CARTESIAN_POINT('Ctrl Pts',(50.0056064783735,246.821978495101,31.6213214466101)) ;
#80161=CARTESIAN_POINT('Ctrl Pts',(49.9998694926128,246.806946276468,31.6214425632436)) ;
#80162=CARTESIAN_POINT('Ctrl Pts',(49.9942568463425,246.792192381567,31.6247663677073)) ;
#80163=CARTESIAN_POINT('Ctrl Pts',(49.9847524089911,246.767174852646,31.6360173172129)) ;
#80164=CARTESIAN_POINT('Ctrl Pts',(49.9799936655788,246.754633080418,31.6439181882807)) ;
#80165=CARTESIAN_POINT('Ctrl Pts',(49.9717481869224,246.732896031175,31.6673134404803)) ;
#80166=CARTESIAN_POINT('Ctrl Pts',(49.9686632968791,246.724764023479,31.6803089503134)) ;
#80167=CARTESIAN_POINT('Ctrl Pts',(49.96538060094,246.716115506741,31.7018008541679)) ;
#80168=CARTESIAN_POINT('Ctrl Pts',(49.9645064199671,246.713813311183,31.7095030704103)) ;
#80169=CARTESIAN_POINT('Ctrl Pts',(49.9633228773224,246.710696906288,31.7252452258737)) ;
#80170=CARTESIAN_POINT('Ctrl Pts',(49.963014268976,246.709884602433,31.7332749378809)) ;
#80171=CARTESIAN_POINT('Ctrl Pts',(49.963014268976,246.709884602433,31.7413203435596)) ;
#80172=CARTESIAN_POINT('Ctrl Pts',(50.8658810352972,248.953449595789,31.7413203435596)) ;
#80173=CARTESIAN_POINT('Ctrl Pts',(50.8677904209831,248.952297607161,31.7413203435596)) ;
#80174=CARTESIAN_POINT('Ctrl Pts',(50.8697007917982,248.95114620239,31.7413203435596)) ;
#80175=CARTESIAN_POINT('Ctrl Pts',(50.9146555099304,248.923982502807,31.7413203435597)) ;
#80176=CARTESIAN_POINT('Ctrl Pts',(50.9528763911288,248.901570300818,31.7413203435596)) ;
#80177=CARTESIAN_POINT('Ctrl Pts',(51.0258112433797,248.869636083941,31.7413203435597)) ;
#80178=CARTESIAN_POINT('Ctrl Pts',(51.0659577418149,248.857165972989,31.7413203435597)) ;
#80179=CARTESIAN_POINT('Ctrl Pts',(51.1146051981685,248.842724136288,31.7413203435596)) ;
#80180=CARTESIAN_POINT('Ctrl Pts',(51.1174932228874,248.841863408451,31.7413203435596)) ;
#80181=CARTESIAN_POINT('Ctrl Pts',(51.1203809856748,248.841004114039,31.7413203435596)) ;
#80182=CARTESIAN_POINT('Ctrl Pts',(50.8658810352972,248.953449595789,31.7054164275186)) ;
#80183=CARTESIAN_POINT('Ctrl Pts',(50.8677904209831,248.952297607161,31.7054164275186)) ;
#80184=CARTESIAN_POINT('Ctrl Pts',(50.8697007917982,248.95114620239,31.7054164275186)) ;
#80185=CARTESIAN_POINT('Ctrl Pts',(50.9146555099304,248.923982502807,31.7054164275187)) ;
#80186=CARTESIAN_POINT('Ctrl Pts',(50.9528763911288,248.901570300818,31.7054164275186)) ;
#80187=CARTESIAN_POINT('Ctrl Pts',(51.0258112433797,248.869636083941,31.7054164275186)) ;
#80188=CARTESIAN_POINT('Ctrl Pts',(51.0659577418149,248.857165972989,31.7054164275186)) ;
#80189=CARTESIAN_POINT('Ctrl Pts',(51.1146051981685,248.842724136288,31.7054164275186)) ;
#80190=CARTESIAN_POINT('Ctrl Pts',(51.1174932228874,248.841863408451,31.7054164275186)) ;
#80191=CARTESIAN_POINT('Ctrl Pts',(51.1203809856748,248.841004114039,31.7054164275186)) ;
#80192=CARTESIAN_POINT('Ctrl Pts',(50.8503012828812,248.927626635796,31.6432843213404)) ;
#80193=CARTESIAN_POINT('Ctrl Pts',(50.8522098095963,248.926474052239,31.6432843213404)) ;
#80194=CARTESIAN_POINT('Ctrl Pts',(50.8541218808106,248.92532381438,31.6432843213404)) ;
#80195=CARTESIAN_POINT('Ctrl Pts',(50.8990610907504,248.898152284773,31.6432843213404)) ;
#80196=CARTESIAN_POINT('Ctrl Pts',(50.9385926468991,248.874899245215,31.6432843213404)) ;
#80197=CARTESIAN_POINT('Ctrl Pts',(51.0157881375332,248.841100025522,31.6432843213404)) ;
#80198=CARTESIAN_POINT('Ctrl Pts',(51.0573613312886,248.828244720669,31.6432843213404)) ;
#80199=CARTESIAN_POINT('Ctrl Pts',(51.1060034495555,248.813819167932,31.6432843213404)) ;
#80200=CARTESIAN_POINT('Ctrl Pts',(51.108892071156,248.81295593694,31.6432843213404)) ;
#80201=CARTESIAN_POINT('Ctrl Pts',(51.1117795363305,248.812097903334,31.6432843213404)) ;
#80202=CARTESIAN_POINT('Ctrl Pts',(50.817800902286,248.873758255513,31.6213203435596)) ;
#80203=CARTESIAN_POINT('Ctrl Pts',(50.8197097813091,248.872605915967,31.6213203435596)) ;
#80204=CARTESIAN_POINT('Ctrl Pts',(50.8216208964723,248.871455077228,31.6213203435596)) ;
#80205=CARTESIAN_POINT('Ctrl Pts',(50.866575821533,248.844290875403,31.6213203435597)) ;
#80206=CARTESIAN_POINT('Ctrl Pts',(50.9087973628861,248.819267489191,31.6213203435597)) ;
#80207=CARTESIAN_POINT('Ctrl Pts',(50.9948811142887,248.781575254289,31.6213203435597)) ;
#80208=CARTESIAN_POINT('Ctrl Pts',(51.0394123778877,248.767959465833,31.6213203435597)) ;
#80209=CARTESIAN_POINT('Ctrl Pts',(51.088060523457,248.753518054849,31.6213203435597)) ;
#80210=CARTESIAN_POINT('Ctrl Pts',(51.0909487642498,248.752656211516,31.6213203435597)) ;
#80211=CARTESIAN_POINT('Ctrl Pts',(51.0938363514906,248.751797660789,31.6213203435597)) ;
#80212=CARTESIAN_POINT('Ctrl Pts',(50.803890188879,248.850701676295,31.6213203435596)) ;
#80213=CARTESIAN_POINT('Ctrl Pts',(50.8057995745649,248.849549687667,31.6213203435596)) ;
#80214=CARTESIAN_POINT('Ctrl Pts',(50.807709533127,248.848398088001,31.6213203435596)) ;
#80215=CARTESIAN_POINT('Ctrl Pts',(50.8526791620758,248.821240949726,31.6213203435597)) ;
#80216=CARTESIAN_POINT('Ctrl Pts',(50.8960447320484,248.795457119086,31.6213203435597)) ;
#80217=CARTESIAN_POINT('Ctrl Pts',(50.9859328579063,248.756098193207,31.6213203435597)) ;
#80218=CARTESIAN_POINT('Ctrl Pts',(51.0317272198324,248.742164050894,31.6213203435597)) ;
#80219=CARTESIAN_POINT('Ctrl Pts',(51.0803807937155,248.727707582416,31.6213203435597)) ;
#80220=CARTESIAN_POINT('Ctrl Pts',(51.0832686016586,248.726847429988,31.6213203435597)) ;
#80221=CARTESIAN_POINT('Ctrl Pts',(51.086156364446,248.725988135576,31.6213203435597)) ;
#80222=CARTESIAN_POINT('',(51.1117180549604,248.843581675164,31.7413203435596)) ;
#80223=CARTESIAN_POINT('Ctrl Pts',(51.086156364446,248.725988135576,31.6213203435596)) ;
#80224=CARTESIAN_POINT('Ctrl Pts',(51.0862184877469,248.726273926329,31.6213203435596)) ;
#80225=CARTESIAN_POINT('Ctrl Pts',(51.0862806119271,248.726559719963,31.6213214476805)) ;
#80226=CARTESIAN_POINT('Ctrl Pts',(51.0863427360275,248.726845510821,31.6213236533421)) ;
#80227=CARTESIAN_POINT('Ctrl Pts',(51.0882792485619,248.735754091775,31.6213924075178)) ;
#80228=CARTESIAN_POINT('Ctrl Pts',(51.0902047015119,248.744610062794,31.6225264675735)) ;
#80229=CARTESIAN_POINT('Ctrl Pts',(51.0920824713405,248.753245454865,31.6246412173916)) ;
#80230=CARTESIAN_POINT('Ctrl Pts',(51.0934961261605,248.759746498517,31.6262332795432)) ;
#80231=CARTESIAN_POINT('Ctrl Pts',(51.0948829023365,248.76612299147,31.6283824423936)) ;
#80232=CARTESIAN_POINT('Ctrl Pts',(51.0962258862543,248.772298724066,31.6310714658467)) ;
#80233=CARTESIAN_POINT('Ctrl Pts',(51.0980065041998,248.780486923596,31.6346367530796)) ;
#80234=CARTESIAN_POINT('Ctrl Pts',(51.0996908773251,248.788233065203,31.6391102795551)) ;
#80235=CARTESIAN_POINT('Ctrl Pts',(51.1012400129114,248.795367565278,31.6444325796703)) ;
#80236=CARTESIAN_POINT('Ctrl Pts',(51.1015312478744,248.796708839653,31.6454331634095)) ;
#80237=CARTESIAN_POINT('Ctrl Pts',(51.1018176837993,248.798028431586,31.6464638781034)) ;
#80238=CARTESIAN_POINT('Ctrl Pts',(51.1020990289973,248.799325104428,31.6475245056918)) ;
#80239=CARTESIAN_POINT('Ctrl Pts',(51.102895783385,248.802997211799,31.6505281456707)) ;
#80240=CARTESIAN_POINT('Ctrl Pts',(51.1036517788236,248.806485735886,31.6537715081556)) ;
#80241=CARTESIAN_POINT('Ctrl Pts',(51.1043651577471,248.809778676875,31.6572323814361)) ;
#80242=CARTESIAN_POINT('Ctrl Pts',(51.1057129105313,248.81599987327,31.6637708443012)) ;
#80243=CARTESIAN_POINT('Ctrl Pts',(51.106894374542,248.82145637452,31.6710108132204)) ;
#80244=CARTESIAN_POINT('Ctrl Pts',(51.1078992539062,248.82608772059,31.6787830171431)) ;
#80245=CARTESIAN_POINT('Ctrl Pts',(51.1086080932376,248.829354660253,31.6842655098964)) ;
#80246=CARTESIAN_POINT('Ctrl Pts',(51.1092288843809,248.832210410807,31.6900139551922)) ;
#80247=CARTESIAN_POINT('Ctrl Pts',(51.1097541934407,248.834620869011,31.6959770540884)) ;
#80248=CARTESIAN_POINT('Ctrl Pts',(51.1104917883012,248.838005431963,31.7043499367117)) ;
#80249=CARTESIAN_POINT('Ctrl Pts',(51.111033494853,248.840476230148,31.7130520747481)) ;
#80250=CARTESIAN_POINT('Ctrl Pts',(51.1113601040974,248.841959524176,31.7219325936276)) ;
#80251=CARTESIAN_POINT('Ctrl Pts',(51.1115813979812,248.842964529093,31.7279495834929)) ;
#80252=CARTESIAN_POINT('Ctrl Pts',(51.1117037272201,248.843515379474,31.7340491166042)) ;
#80253=CARTESIAN_POINT('Ctrl Pts',(51.111717190373,248.843576024758,31.7401863974346)) ;
#80254=CARTESIAN_POINT('Ctrl Pts',(51.1117180192344,248.843579758396,31.7405642402226)) ;
#80255=CARTESIAN_POINT('Ctrl Pts',(51.1117184349279,248.843581630191,31.7409422258038)) ;
#80256=CARTESIAN_POINT('Ctrl Pts',(51.1117184349279,248.843581630191,31.7413203435596)) ;
#80257=CARTESIAN_POINT('Ctrl Pts',(51.1117179332896,248.843581270679,31.7413203435596)) ;
#80258=CARTESIAN_POINT('Ctrl Pts',(51.065957488389,248.857166051707,31.7413203435597)) ;
#80259=CARTESIAN_POINT('Ctrl Pts',(51.0258111312861,248.869636133021,31.7413203435597)) ;
#80260=CARTESIAN_POINT('Ctrl Pts',(50.9528764837856,248.901570260249,31.7413203435596)) ;
#80261=CARTESIAN_POINT('Ctrl Pts',(50.914655699209,248.923982391817,31.7413203435597)) ;
#80262=CARTESIAN_POINT('Ctrl Pts',(50.8716087793554,248.949993308924,31.7413203435596)) ;
#80263=CARTESIAN_POINT('Origin',(51.0967112553384,248.704482161408,31.7413203435596)) ;
#80264=CARTESIAN_POINT('',(52.0203128398474,248.824482161408,31.7413203435596)) ;
#80265=CARTESIAN_POINT('',(51.4063975156363,248.824482161408,31.7413203435596)) ;
#80266=CARTESIAN_POINT('',(51.0967112553384,248.824482161408,31.7413203435596)) ;
#80267=CARTESIAN_POINT('Origin',(51.4064119640033,248.704480196061,31.7413223089067)) ;
#80268=CARTESIAN_POINT('Origin',(52.1403128398474,248.704482161408,31.7413203435596)) ;
#80269=CARTESIAN_POINT('Ctrl Pts',(51.1027668548594,248.844832957121,31.7413203435596)) ;
#80270=CARTESIAN_POINT('Ctrl Pts',(51.1057506523197,248.844415923056,31.7413203435596)) ;
#80271=CARTESIAN_POINT('Ctrl Pts',(51.108734666895,248.843999359902,31.7413203435596)) ;
#80272=CARTESIAN_POINT('Ctrl Pts',(51.1534179425839,248.837743668557,31.7413203435596)) ;
#80273=CARTESIAN_POINT('Ctrl Pts',(51.1927045698,248.832377914482,31.7413203435596)) ;
#80274=CARTESIAN_POINT('Ctrl Pts',(51.2859410141499,248.824656420132,31.7413203435596)) ;
#80275=CARTESIAN_POINT('Ctrl Pts',(51.3443769229423,248.824452291525,31.7413203435596)) ;
#80276=CARTESIAN_POINT('Ctrl Pts',(51.4064008275487,248.824482163003,31.7413203435596)) ;
#80277=CARTESIAN_POINT('Ctrl Pts',(51.1027668548594,248.844832957121,31.7054164275186)) ;
#80278=CARTESIAN_POINT('Ctrl Pts',(51.1057506523197,248.844415923056,31.7054164275186)) ;
#80279=CARTESIAN_POINT('Ctrl Pts',(51.108734666895,248.843999359902,31.7054164275186)) ;
#80280=CARTESIAN_POINT('Ctrl Pts',(51.1534179425839,248.837743668557,31.7054164275186)) ;
#80281=CARTESIAN_POINT('Ctrl Pts',(51.1927045698,248.832377914482,31.7054164275186)) ;
#80282=CARTESIAN_POINT('Ctrl Pts',(51.2859410141499,248.824656420132,31.7054164275186)) ;
#80283=CARTESIAN_POINT('Ctrl Pts',(51.3443769229423,248.824452291525,31.7054164275186)) ;
#80284=CARTESIAN_POINT('Ctrl Pts',(51.4064008275487,248.824482163003,31.7054164275186)) ;
#80285=CARTESIAN_POINT('Ctrl Pts',(51.0985922489639,248.814964465564,31.643284324805)) ;
#80286=CARTESIAN_POINT('Ctrl Pts',(51.1015758214971,248.814546944233,31.643284324805)) ;
#80287=CARTESIAN_POINT('Ctrl Pts',(51.104560266249,248.81413132837,31.643284324805)) ;
#80288=CARTESIAN_POINT('Ctrl Pts',(51.1492415021694,248.80787131815,31.643284324805)) ;
#80289=CARTESIAN_POINT('Ctrl Pts',(51.1891454007169,248.802410297526,31.643284324805)) ;
#80290=CARTESIAN_POINT('Ctrl Pts',(51.2850366354972,248.794467602977,31.643284324805)) ;
#80291=CARTESIAN_POINT('Ctrl Pts',(51.3443931112797,248.794282641714,31.643284324805)) ;
#80292=CARTESIAN_POINT('Ctrl Pts',(51.4064153524046,248.794323351499,31.643284324805)) ;
#80293=CARTESIAN_POINT('Ctrl Pts',(51.0898837497786,248.752656851168,31.6213203435596)) ;
#80294=CARTESIAN_POINT('Ctrl Pts',(51.0928674145709,248.7522395297,31.6213203435596)) ;
#80295=CARTESIAN_POINT('Ctrl Pts',(51.0958516053795,248.751823395832,31.6213203435596)) ;
#80296=CARTESIAN_POINT('Ctrl Pts',(51.1405353953433,248.745567842801,31.6213203435596)) ;
#80297=CARTESIAN_POINT('Ctrl Pts',(51.1817199296158,248.739895483147,31.6213203435596)) ;
#80298=CARTESIAN_POINT('Ctrl Pts',(51.2831521234115,248.731498417485,31.6213203435596)) ;
#80299=CARTESIAN_POINT('Ctrl Pts',(51.3444227287569,248.73137384663,31.6213203435596)) ;
#80300=CARTESIAN_POINT('Ctrl Pts',(51.4064456521979,248.731410110828,31.6213203435597)) ;
#80301=CARTESIAN_POINT('Ctrl Pts',(51.086156364446,248.725988135576,31.6213203435596)) ;
#80302=CARTESIAN_POINT('Ctrl Pts',(51.0891401619064,248.72557110151,31.6213203435596)) ;
#80303=CARTESIAN_POINT('Ctrl Pts',(51.0921240529548,248.725154332015,31.6213203435596)) ;
#80304=CARTESIAN_POINT('Ctrl Pts',(51.1368100661075,248.718902921604,31.6213203435596)) ;
#80305=CARTESIAN_POINT('Ctrl Pts',(51.1785415671225,248.713138013086,31.6213203435596)) ;
#80306=CARTESIAN_POINT('Ctrl Pts',(51.2823458655609,248.704547641672,31.6213203435596)) ;
#80307=CARTESIAN_POINT('Ctrl Pts',(51.3444347164168,248.704452305443,31.6213203435597)) ;
#80308=CARTESIAN_POINT('Ctrl Pts',(51.4064586210232,248.704482176921,31.6213203435597)) ;
#80309=CARTESIAN_POINT('Ctrl Pts',(51.4063975156363,248.824482161408,31.7413203435596)) ;
#80310=CARTESIAN_POINT('Ctrl Pts',(51.3843454600747,248.824471540866,31.7413203435596)) ;
#80311=CARTESIAN_POINT('Ctrl Pts',(51.3627451413246,248.82446585171,31.7413203435596)) ;
#80312=CARTESIAN_POINT('Ctrl Pts',(51.3415687668468,248.824692574776,31.7413203435596)) ;
#80313=CARTESIAN_POINT('Ctrl Pts',(51.3183068802966,248.824941626201,31.7413203435596)) ;
#80314=CARTESIAN_POINT('Ctrl Pts',(51.2955565276338,248.825470785683,31.7413203435596)) ;
#80315=CARTESIAN_POINT('Ctrl Pts',(51.2732760199652,248.826515819019,31.7413203435596)) ;
#80316=CARTESIAN_POINT('Ctrl Pts',(51.2587924657089,248.827195148109,31.7413203435596)) ;
#80317=CARTESIAN_POINT('Ctrl Pts',(51.2445073560321,248.828091135254,31.7413203435596)) ;
#80318=CARTESIAN_POINT('Ctrl Pts',(51.2304083944376,248.829257089501,31.7413203435596)) ;
#80319=CARTESIAN_POINT('Ctrl Pts',(51.2282454160114,248.829435963234,31.7413203435596)) ;
#80320=CARTESIAN_POINT('Ctrl Pts',(51.2260772117856,248.829621971491,31.7413203435596)) ;
#80321=CARTESIAN_POINT('Ctrl Pts',(51.223903630718,248.829814863711,31.7413203435596)) ;
#80322=CARTESIAN_POINT('Ctrl Pts',(51.2060460327205,248.831399617905,31.7413203435596)) ;
#80323=CARTESIAN_POINT('Ctrl Pts',(51.1878257913053,248.833452870398,31.7413203435596)) ;
#80324=CARTESIAN_POINT('Ctrl Pts',(51.1691574004514,248.835811237207,31.7413203435596)) ;
#80325=CARTESIAN_POINT('Ctrl Pts',(51.1521435087056,248.83796059212,31.7413203435596)) ;
#80326=CARTESIAN_POINT('Ctrl Pts',(51.1347574231604,248.840363925417,31.7413203435596)) ;
#80327=CARTESIAN_POINT('Ctrl Pts',(51.1169311642445,248.842853457903,31.7413203435596)) ;
#80328=CARTESIAN_POINT('Ctrl Pts',(51.115197667293,248.843095550032,31.7413203435596)) ;
#80329=CARTESIAN_POINT('Ctrl Pts',(51.113460004846,248.843338416063,31.7413203435596)) ;
#80330=CARTESIAN_POINT('Ctrl Pts',(51.1117181123312,248.84358187378,31.7413203435596)) ;
#80331=CARTESIAN_POINT('Origin',(52.1403128398474,248.712613109356,31.7413203435596)) ;
#80332=CARTESIAN_POINT('',(52.0203128398474,250.600744087106,31.7413203435596)) ;
#80333=CARTESIAN_POINT('Origin',(52.1403128398474,250.480744087106,31.7413203435596)) ;
#80334=CARTESIAN_POINT('',(52.0203128398474,248.712613109356,31.7413203435596)) ;
#80335=CARTESIAN_POINT('Origin',(51.4036689174439,250.480744087106,31.7413203435596)) ;
#80336=CARTESIAN_POINT('',(52.5496443674977,250.600744087106,31.7413203435596)) ;
#80337=CARTESIAN_POINT('',(51.4036689174439,250.600744087106,31.7413203435596)) ;
#80338=CARTESIAN_POINT('Origin',(52.4296443674977,250.480744087106,31.7413203435596)) ;
#80339=CARTESIAN_POINT('Origin',(52.4296443674977,249.600744072205,31.7413203435596)) ;
#80340=CARTESIAN_POINT('',(52.5496443674977,246.600744027501,31.7413203435596)) ;
#80341=CARTESIAN_POINT('',(52.5496443674977,249.600744072205,31.7413203435596)) ;
#80342=CARTESIAN_POINT('Origin',(52.4296443674977,246.720744027501,31.7413203435596)) ;
#80343=CARTESIAN_POINT('Origin',(51.6683346812691,246.720744027501,31.7413203435596)) ;
#80344=CARTESIAN_POINT('',(51.6683346812691,246.600744027501,31.7413203435596)) ;
#80345=CARTESIAN_POINT('Ctrl Pts',(49.963014268976,246.709884602433,31.7413203435596)) ;
#80346=CARTESIAN_POINT('Ctrl Pts',(49.931599450876,246.725215026983,31.7413203435596)) ;
#80347=CARTESIAN_POINT('Ctrl Pts',(49.8506223616046,246.764832992921,31.7413203435596)) ;
#80348=CARTESIAN_POINT('Ctrl Pts',(49.7636581126107,246.815285524649,31.7413203435596)) ;
#80349=CARTESIAN_POINT('Ctrl Pts',(49.6774660851055,246.887582047699,31.7413203435596)) ;
#80350=CARTESIAN_POINT('Ctrl Pts',(49.6042085555324,246.966699774459,31.7413203435596)) ;
#80351=CARTESIAN_POINT('Ctrl Pts',(49.5497454158327,247.044683872908,31.7413203435596)) ;
#80352=CARTESIAN_POINT('Ctrl Pts',(49.5182664633806,247.089148063069,31.7413203435596)) ;
#80353=CARTESIAN_POINT('Ctrl Pts',(49.963014268976,246.709884602433,31.7054164275186)) ;
#80354=CARTESIAN_POINT('Ctrl Pts',(49.931599450876,246.725215026983,31.7054164275186)) ;
#80355=CARTESIAN_POINT('Ctrl Pts',(49.8506223616046,246.764832992921,31.7054164275186)) ;
#80356=CARTESIAN_POINT('Ctrl Pts',(49.7636581126107,246.815285524649,31.7054164275186)) ;
#80357=CARTESIAN_POINT('Ctrl Pts',(49.6774660851055,246.887582047699,31.7054164275186)) ;
#80358=CARTESIAN_POINT('Ctrl Pts',(49.6042085555324,246.966699774459,31.7054164275186)) ;
#80359=CARTESIAN_POINT('Ctrl Pts',(49.5497454158327,247.044683872908,31.7054164275186)) ;
#80360=CARTESIAN_POINT('Ctrl Pts',(49.5182664633806,247.089148063069,31.7054164275186)) ;
#80361=CARTESIAN_POINT('Ctrl Pts',(49.9762408566705,246.736988277557,31.6432842791516)) ;
#80362=CARTESIAN_POINT('Ctrl Pts',(49.944806126295,246.752294468368,31.6432842791516)) ;
#80363=CARTESIAN_POINT('Ctrl Pts',(49.86448943937,246.791620886194,31.6432842791516)) ;
#80364=CARTESIAN_POINT('Ctrl Pts',(49.7803936532232,246.840563126454,31.6432842791516)) ;
#80365=CARTESIAN_POINT('Ctrl Pts',(49.6987354791454,246.909056370919,31.6432842791516)) ;
#80366=CARTESIAN_POINT('Ctrl Pts',(49.6282809757044,246.985040051368,31.6432842791516)) ;
#80367=CARTESIAN_POINT('Ctrl Pts',(49.5743922695998,247.06208594874,31.6432842791516)) ;
#80368=CARTESIAN_POINT('Ctrl Pts',(49.5428810753553,247.106574270477,31.6432842791516)) ;
#80369=CARTESIAN_POINT('Ctrl Pts',(50.0038324296295,246.793528410729,31.6213203435597)) ;
#80370=CARTESIAN_POINT('Ctrl Pts',(49.9724058609042,246.808844534472,31.6213203435597)) ;
#80371=CARTESIAN_POINT('Ctrl Pts',(49.8934018962093,246.847455485118,31.6213203435597)) ;
#80372=CARTESIAN_POINT('Ctrl Pts',(49.8152625837333,246.893353442029,31.6213203435596)) ;
#80373=CARTESIAN_POINT('Ctrl Pts',(49.7431381507101,246.953899251354,31.6213203435596)) ;
#80374=CARTESIAN_POINT('Ctrl Pts',(49.6784688486474,247.023279651295,31.6213203435597)) ;
#80375=CARTESIAN_POINT('Ctrl Pts',(49.6257268303213,247.098448108743,31.6213203435596)) ;
#80376=CARTESIAN_POINT('Ctrl Pts',(49.5942288513534,247.142926539422,31.6213203435596)) ;
#80377=CARTESIAN_POINT('Ctrl Pts',(50.0156420836194,246.817728531914,31.6213203435597)) ;
#80378=CARTESIAN_POINT('Ctrl Pts',(49.9842272655194,246.833058956463,31.6213203435597)) ;
#80379=CARTESIAN_POINT('Ctrl Pts',(49.9057743814449,246.871345851783,31.6213203435597)) ;
#80380=CARTESIAN_POINT('Ctrl Pts',(49.8301799972564,246.915958463683,31.6213203435596)) ;
#80381=CARTESIAN_POINT('Ctrl Pts',(49.7621487599861,246.973100389465,31.6213203435596)) ;
#80382=CARTESIAN_POINT('Ctrl Pts',(49.6999453025556,247.039643602022,31.6213203435597)) ;
#80383=CARTESIAN_POINT('Ctrl Pts',(49.6476855094111,247.114021727431,31.6213203435596)) ;
#80384=CARTESIAN_POINT('Ctrl Pts',(49.616206556959,247.158485917592,31.6213203435596)) ;
#80385=CARTESIAN_POINT('',(49.5182664633806,247.089148063069,31.7413203435596)) ;
#80386=CARTESIAN_POINT('Ctrl Pts',(49.5182664633806,247.089148063069,31.7413203435596)) ;
#80387=CARTESIAN_POINT('Ctrl Pts',(49.5497454158327,247.044683872908,31.7413203435596)) ;
#80388=CARTESIAN_POINT('Ctrl Pts',(49.6042085555324,246.966699774459,31.7413203435596)) ;
#80389=CARTESIAN_POINT('Ctrl Pts',(49.6774660851055,246.887582047699,31.7413203435596)) ;
#80390=CARTESIAN_POINT('Ctrl Pts',(49.7636581126107,246.815285524649,31.7413203435596)) ;
#80391=CARTESIAN_POINT('Ctrl Pts',(49.8506223616046,246.764832992921,31.7413203435596)) ;
#80392=CARTESIAN_POINT('Ctrl Pts',(49.931599450876,246.725215026983,31.7413203435596)) ;
#80393=CARTESIAN_POINT('Ctrl Pts',(49.963014268976,246.709884602433,31.7413203435596)) ;
#80394=CARTESIAN_POINT('Ctrl Pts',(49.6210143583557,247.151690507276,31.6213203435596)) ;
#80395=CARTESIAN_POINT('Ctrl Pts',(49.6207661365521,247.151539246675,31.6213203435596)) ;
#80396=CARTESIAN_POINT('Ctrl Pts',(49.6205164447654,247.151387225589,31.6213214399498)) ;
#80397=CARTESIAN_POINT('Ctrl Pts',(49.6202667549629,247.151235205894,31.6213236426165)) ;
#80398=CARTESIAN_POINT('Ctrl Pts',(49.6124809300875,247.146494929318,31.6213923261465)) ;
#80399=CARTESIAN_POINT('Ctrl Pts',(49.6047409010513,247.141782670592,31.6225275482499)) ;
#80400=CARTESIAN_POINT('Ctrl Pts',(49.5971939561122,247.13718789474,31.6246439453278)) ;
#80401=CARTESIAN_POINT('Ctrl Pts',(49.5915259656661,247.133737075124,31.6262334253776)) ;
#80402=CARTESIAN_POINT('Ctrl Pts',(49.585966463366,247.130352225227,31.6283776256885)) ;
#80403=CARTESIAN_POINT('Ctrl Pts',(49.5805814724203,247.127073844614,31.6310592826868)) ;
#80404=CARTESIAN_POINT('Ctrl Pts',(49.5734257007315,247.122717413301,31.6346227659724)) ;
#80405=CARTESIAN_POINT('Ctrl Pts',(49.5666561311895,247.118596395527,31.6390944397671)) ;
#80406=CARTESIAN_POINT('Ctrl Pts',(49.5604201950558,247.114802652923,31.6444146524314)) ;
#80407=CARTESIAN_POINT('Ctrl Pts',(49.5592408348075,247.11408516815,31.6454208281193)) ;
#80408=CARTESIAN_POINT('Ctrl Pts',(49.558080617175,247.113379429088,31.6464574885456)) ;
#80409=CARTESIAN_POINT('Ctrl Pts',(49.556940634716,247.112686124991,31.6475244112343)) ;
#80410=CARTESIAN_POINT('Ctrl Pts',(49.556940190168,247.11268585463,31.6475248272918)) ;
#80411=CARTESIAN_POINT('Ctrl Pts',(49.5569397456231,247.112685584271,31.647525243354)) ;
#80412=CARTESIAN_POINT('Ctrl Pts',(49.5569393010813,247.112685313913,31.6475256594207)) ;
#80413=CARTESIAN_POINT('Ctrl Pts',(49.5537377487577,247.110738223408,31.6505221368304)) ;
#80414=CARTESIAN_POINT('Ctrl Pts',(49.5506956091687,247.108889076253,31.6537571310734)) ;
#80415=CARTESIAN_POINT('Ctrl Pts',(49.5478235026766,247.107143545382,31.6572085979443)) ;
#80416=CARTESIAN_POINT('Ctrl Pts',(49.5423838363783,247.103837572752,31.6637455519426)) ;
#80417=CARTESIAN_POINT('Ctrl Pts',(49.5376124175149,247.10093844266,31.6709841927054)) ;
#80418=CARTESIAN_POINT('Ctrl Pts',(49.533562965559,247.09847574875,31.678755099518)) ;
#80419=CARTESIAN_POINT('Ctrl Pts',(49.5307045400923,247.096737383394,31.6842404239951)) ;
#80420=CARTESIAN_POINT('Ctrl Pts',(49.5282063572055,247.095216848345,31.6899920749716)) ;
#80421=CARTESIAN_POINT('Ctrl Pts',(49.5260982265622,247.093932318721,31.6959585760797)) ;
#80422=CARTESIAN_POINT('Ctrl Pts',(49.5231392608972,247.092129356904,31.7043331386219)) ;
#80423=CARTESIAN_POINT('Ctrl Pts',(49.5209800806778,247.090810247108,31.7130371660676)) ;
#80424=CARTESIAN_POINT('Ctrl Pts',(49.519684064817,247.090016978543,31.7219195434862)) ;
#80425=CARTESIAN_POINT('Ctrl Pts',(49.5187514549454,247.089446144406,31.7283112807438)) ;
#80426=CARTESIAN_POINT('Ctrl Pts',(49.5182664633807,247.089148063069,31.7347961218212)) ;
#80427=CARTESIAN_POINT('Ctrl Pts',(49.5182664633807,247.089148063069,31.7413203435596)) ;
#80428=CARTESIAN_POINT('Ctrl Pts',(49.5182664633807,247.089148063069,31.7413203435596)) ;
#80429=CARTESIAN_POINT('Ctrl Pts',(49.4739778031524,247.174728266885,31.7413203435596)) ;
#80430=CARTESIAN_POINT('Ctrl Pts',(49.4243564080963,247.265450319237,31.7413203435596)) ;
#80431=CARTESIAN_POINT('Ctrl Pts',(49.3620432342539,247.48914516309,31.7413203435596)) ;
#80432=CARTESIAN_POINT('Ctrl Pts',(49.3579333223532,247.594303447023,31.7413203435596)) ;
#80433=CARTESIAN_POINT('Ctrl Pts',(49.3518273473795,247.692149180776,31.7413203435596)) ;
#80434=CARTESIAN_POINT('Ctrl Pts',(49.5182664633807,247.089148063069,31.7054164275186)) ;
#80435=CARTESIAN_POINT('Ctrl Pts',(49.4739778031524,247.174728266885,31.7054164275186)) ;
#80436=CARTESIAN_POINT('Ctrl Pts',(49.4243564080963,247.265450319237,31.7054164275186)) ;
#80437=CARTESIAN_POINT('Ctrl Pts',(49.3620432342539,247.48914516309,31.7054164275186)) ;
#80438=CARTESIAN_POINT('Ctrl Pts',(49.3579333223532,247.594303447023,31.7054164275186)) ;
#80439=CARTESIAN_POINT('Ctrl Pts',(49.3518273473795,247.692149180776,31.7054164275186)) ;
#80440=CARTESIAN_POINT('Ctrl Pts',(49.5450510815804,247.103009386154,31.6432842835775)) ;
#80441=CARTESIAN_POINT('Ctrl Pts',(49.5009087357332,247.188686189581,31.6432842835775)) ;
#80442=CARTESIAN_POINT('Ctrl Pts',(49.4521809274138,247.278024774281,31.6432842835775)) ;
#80443=CARTESIAN_POINT('Ctrl Pts',(49.3923857677425,247.492693277404,31.6432842835775)) ;
#80444=CARTESIAN_POINT('Ctrl Pts',(49.38821128267,247.596175793791,31.6432842835775)) ;
#80445=CARTESIAN_POINT('Ctrl Pts',(49.3819275757361,247.694027558442,31.6432842835775)) ;
#80446=CARTESIAN_POINT('Ctrl Pts',(49.6009256299209,247.131925055626,31.6213203435596)) ;
#80447=CARTESIAN_POINT('Ctrl Pts',(49.5567233085258,247.217562262025,31.6213203435596)) ;
#80448=CARTESIAN_POINT('Ctrl Pts',(49.5101540874739,247.304273277684,31.6213203435596)) ;
#80449=CARTESIAN_POINT('Ctrl Pts',(49.4556207812252,247.500038912409,31.6213203435596)) ;
#80450=CARTESIAN_POINT('Ctrl Pts',(49.4509295670317,247.600096690393,31.6213203435596)) ;
#80451=CARTESIAN_POINT('Ctrl Pts',(49.4447187139868,247.697945982926,31.6213203435596)) ;
#80452=CARTESIAN_POINT('Ctrl Pts',(49.6248408710857,247.144301445761,31.6213203435596)) ;
#80453=CARTESIAN_POINT('Ctrl Pts',(49.5805522108574,247.229881649577,31.6213203435596)) ;
#80454=CARTESIAN_POINT('Ctrl Pts',(49.5349558256602,247.315510954877,31.6213203435596)) ;
#80455=CARTESIAN_POINT('Ctrl Pts',(49.4826761929734,247.503173668296,31.6213203435596)) ;
#80456=CARTESIAN_POINT('Ctrl Pts',(49.4777003462836,247.601777400386,31.6213203435596)) ;
#80457=CARTESIAN_POINT('Ctrl Pts',(49.4715943713098,247.699623134138,31.6213203435596)) ;
#80458=CARTESIAN_POINT('',(49.3518273473795,247.692149180776,31.7413203435596)) ;
#80459=CARTESIAN_POINT('Ctrl Pts',(49.3518273473795,247.692149180776,31.7413203435596)) ;
#80460=CARTESIAN_POINT('Ctrl Pts',(49.3532388697544,247.669530116159,31.7413203435596)) ;
#80461=CARTESIAN_POINT('Ctrl Pts',(49.3546686212915,247.646555189823,31.7413203435596)) ;
#80462=CARTESIAN_POINT('Ctrl Pts',(49.3563472260032,247.623183539353,31.7413203435596)) ;
#80463=CARTESIAN_POINT('Ctrl Pts',(49.3578189696063,247.602692069958,31.7413203435596)) ;
#80464=CARTESIAN_POINT('Ctrl Pts',(49.3594818314035,247.581895581421,31.7413203435596)) ;
#80465=CARTESIAN_POINT('Ctrl Pts',(49.3615296529984,247.560777183086,31.7413203435596)) ;
#80466=CARTESIAN_POINT('Ctrl Pts',(49.3634663892828,247.540804364933,31.7413203435596)) ;
#80467=CARTESIAN_POINT('Ctrl Pts',(49.3657469823047,247.520543483475,31.7413203435596)) ;
#80468=CARTESIAN_POINT('Ctrl Pts',(49.3685771465373,247.499991824908,31.7413203435596)) ;
#80469=CARTESIAN_POINT('Ctrl Pts',(49.3713415064495,247.479918014202,31.7413203435596)) ;
#80470=CARTESIAN_POINT('Ctrl Pts',(49.3746294947228,247.459566601333,31.7413203435596)) ;
#80471=CARTESIAN_POINT('Ctrl Pts',(49.3786823865536,247.438948806417,31.7413203435596)) ;
#80472=CARTESIAN_POINT('Ctrl Pts',(49.3807088324691,247.428639908959,31.7413203435596)) ;
#80473=CARTESIAN_POINT('Ctrl Pts',(49.3829273491322,247.418264650282,31.7413203435596)) ;
#80474=CARTESIAN_POINT('Ctrl Pts',(49.3853737884668,247.407826011524,31.7413203435596)) ;
#80475=CARTESIAN_POINT('Ctrl Pts',(49.386597008134,247.402606692145,31.7413203435596)) ;
#80476=CARTESIAN_POINT('Ctrl Pts',(49.3878772728497,247.3973715456,31.7413203435596)) ;
#80477=CARTESIAN_POINT('Ctrl Pts',(49.3892194719798,247.392121057641,31.7413203435596)) ;
#80478=CARTESIAN_POINT('Ctrl Pts',(49.3900313620237,247.388945061766,31.7413203435596)) ;
#80479=CARTESIAN_POINT('Ctrl Pts',(49.3908659191905,247.385763453995,31.7413203435596)) ;
#80480=CARTESIAN_POINT('Ctrl Pts',(49.3917242773753,247.382576356185,31.7413203435596)) ;
#80481=CARTESIAN_POINT('Ctrl Pts',(49.3922849384499,247.380494612556,31.7413203435596)) ;
#80482=CARTESIAN_POINT('Ctrl Pts',(49.3928557558029,247.378410523425,31.7413203435596)) ;
#80483=CARTESIAN_POINT('Ctrl Pts',(49.393437051874,247.376324135667,31.7413203435596)) ;
#80484=CARTESIAN_POINT('Ctrl Pts',(49.3988416175673,247.35692606941,31.7413203435596)) ;
#80485=CARTESIAN_POINT('Ctrl Pts',(49.4049126636213,247.338171165244,31.7413203435596)) ;
#80486=CARTESIAN_POINT('Ctrl Pts',(49.4114315368304,247.319954022923,31.7413203435596)) ;
#80487=CARTESIAN_POINT('Ctrl Pts',(49.4182839819689,247.300804706111,31.7413203435596)) ;
#80488=CARTESIAN_POINT('Ctrl Pts',(49.4256316444079,247.282249701211,31.7413203435596)) ;
#80489=CARTESIAN_POINT('Ctrl Pts',(49.433276546524,247.264182112204,31.7413203435596)) ;
#80490=CARTESIAN_POINT('Ctrl Pts',(49.4415958507146,247.244520674208,31.7413203435596)) ;
#80491=CARTESIAN_POINT('Ctrl Pts',(49.4502673598285,247.225436498998,31.7413203435596)) ;
#80492=CARTESIAN_POINT('Ctrl Pts',(49.4590962100918,247.206808544484,31.7413203435596)) ;
#80493=CARTESIAN_POINT('Ctrl Pts',(49.4689135927178,247.186094889642,31.7413203435596)) ;
#80494=CARTESIAN_POINT('Ctrl Pts',(49.4789257823363,247.165945409405,31.7413203435596)) ;
#80495=CARTESIAN_POINT('Ctrl Pts',(49.4889328468167,247.146212535825,31.7413203435596)) ;
#80496=CARTESIAN_POINT('Ctrl Pts',(49.498761731518,247.126831013938,31.7413203435596)) ;
#80497=CARTESIAN_POINT('Ctrl Pts',(49.5085870880952,247.107851787803,31.7413203435596)) ;
#80498=CARTESIAN_POINT('Ctrl Pts',(49.5182664633806,247.089148063069,31.7413203435596)) ;
#80499=CARTESIAN_POINT('Ctrl Pts',(49.4721208157112,247.69114871288,31.6213203435642)) ;
#80500=CARTESIAN_POINT('Ctrl Pts',(49.4718285538257,247.691151145633,31.6213203461521)) ;
#80501=CARTESIAN_POINT('Ctrl Pts',(49.4715362875381,247.691153578127,31.6213214522989)) ;
#80502=CARTESIAN_POINT('Ctrl Pts',(49.4712440226149,247.691156010318,31.6213236594508)) ;
#80503=CARTESIAN_POINT('Ctrl Pts',(49.4621299528602,247.691231856448,31.6213924878829)) ;
#80504=CARTESIAN_POINT('Ctrl Pts',(49.453068413761,247.691306946542,31.6225270006307)) ;
#80505=CARTESIAN_POINT('Ctrl Pts',(49.4442320358178,247.691379867774,31.6246429710497)) ;
#80506=CARTESIAN_POINT('Ctrl Pts',(49.4375943456525,247.691434644577,31.6262324408676)) ;
#80507=CARTESIAN_POINT('Ctrl Pts',(49.4310832231964,247.691488164056,31.6283769854049)) ;
#80508=CARTESIAN_POINT('Ctrl Pts',(49.4247764592481,247.691540106816,31.6310595117001)) ;
#80509=CARTESIAN_POINT('Ctrl Pts',(49.416396458367,247.691609124838,31.6346238709977)) ;
#80510=CARTESIAN_POINT('Ctrl Pts',(49.408468612876,247.691674511449,31.639097198746)) ;
#80511=CARTESIAN_POINT('Ctrl Pts',(49.4011672799356,247.69173678212,31.6444197570069)) ;
#80512=CARTESIAN_POINT('Ctrl Pts',(49.3997898445836,247.691748529814,31.6454238859751)) ;
#80513=CARTESIAN_POINT('Ctrl Pts',(49.398434774684,247.691760171008,31.6464583727284)) ;
#80514=CARTESIAN_POINT('Ctrl Pts',(49.3971033555651,247.691771716554,31.6475229947526)) ;
#80515=CARTESIAN_POINT('Ctrl Pts',(49.3971027624604,247.691771721697,31.6475234690077)) ;
#80516=CARTESIAN_POINT('Ctrl Pts',(49.3971021693603,247.69177172684,31.6475239432689)) ;
#80517=CARTESIAN_POINT('Ctrl Pts',(49.397101576265,247.691771731983,31.647524417536)) ;
#80518=CARTESIAN_POINT('Ctrl Pts',(49.3933525775546,247.691804242096,31.6505222943044)) ;
#80519=CARTESIAN_POINT('Ctrl Pts',(49.3897908797355,247.691835977459,31.6537589339136)) ;
#80520=CARTESIAN_POINT('Ctrl Pts',(49.3864285291373,247.691866160815,31.6572122154329)) ;
#80521=CARTESIAN_POINT('Ctrl Pts',(49.3800593805917,247.69192333578,31.6637536103066)) ;
#80522=CARTESIAN_POINT('Ctrl Pts',(49.374473703726,247.691974088573,31.67099741896)) ;
#80523=CARTESIAN_POINT('Ctrl Pts',(49.3697327311707,247.69201525315,31.6787738331248)) ;
#80524=CARTESIAN_POINT('Ctrl Pts',(49.366391190525,247.69204426684,31.6842548190841)) ;
#80525=CARTESIAN_POINT('Ctrl Pts',(49.3634699029181,247.69206856051,31.6900015151129)) ;
#80526=CARTESIAN_POINT('Ctrl Pts',(49.3610036578803,247.692087865578,31.6959626248072)) ;
#80527=CARTESIAN_POINT('Ctrl Pts',(49.3575396024612,247.692114981224,31.704335521265)) ;
#80528=CARTESIAN_POINT('Ctrl Pts',(49.355009880036,247.692131795729,31.7130376254696)) ;
#80529=CARTESIAN_POINT('Ctrl Pts',(49.3534904620416,247.692140603079,31.7219180382076)) ;
#80530=CARTESIAN_POINT('Ctrl Pts',(49.3523967698609,247.692146942697,31.7283102475993)) ;
#80531=CARTESIAN_POINT('Ctrl Pts',(49.3518273473795,247.692149180776,31.7347955926502)) ;
#80532=CARTESIAN_POINT('Ctrl Pts',(49.3518273473795,247.692149180776,31.7413203435596)) ;
#80533=CARTESIAN_POINT('Ctrl Pts',(49.3518273473795,247.692149180776,31.7413203435596)) ;
#80534=CARTESIAN_POINT('Ctrl Pts',(49.3575747933183,247.764817090958,31.7413203435596)) ;
#80535=CARTESIAN_POINT('Ctrl Pts',(49.3665625013471,247.891107509426,31.7413203435596)) ;
#80536=CARTESIAN_POINT('Ctrl Pts',(49.3988727594182,248.028724139293,31.7413203435597)) ;
#80537=CARTESIAN_POINT('Ctrl Pts',(49.4417511608872,248.138252930567,31.7413203435597)) ;
#80538=CARTESIAN_POINT('Ctrl Pts',(49.5086086325514,248.25752820517,31.7413203435597)) ;
#80539=CARTESIAN_POINT('Ctrl Pts',(49.5842744886713,248.353930549759,31.7413203435597)) ;
#80540=CARTESIAN_POINT('Ctrl Pts',(49.6274070383129,248.40974827469,31.7413203435597)) ;
#80541=CARTESIAN_POINT('Ctrl Pts',(49.3518273473795,247.692149180776,31.7054164275186)) ;
#80542=CARTESIAN_POINT('Ctrl Pts',(49.3575747933183,247.764817090958,31.7054164275186)) ;
#80543=CARTESIAN_POINT('Ctrl Pts',(49.3665625013471,247.891107509426,31.7054164275186)) ;
#80544=CARTESIAN_POINT('Ctrl Pts',(49.3988727594182,248.028724139293,31.7054164275186)) ;
#80545=CARTESIAN_POINT('Ctrl Pts',(49.4417511608872,248.138252930567,31.7054164275186)) ;
#80546=CARTESIAN_POINT('Ctrl Pts',(49.5086086325514,248.25752820517,31.7054164275186)) ;
#80547=CARTESIAN_POINT('Ctrl Pts',(49.5842744886713,248.353930549759,31.7054164275186)) ;
#80548=CARTESIAN_POINT('Ctrl Pts',(49.6274070383129,248.40974827469,31.7054164275186)) ;
#80549=CARTESIAN_POINT('Ctrl Pts',(49.3818922493259,247.689771289377,31.6432842964434)) ;
#80550=CARTESIAN_POINT('Ctrl Pts',(49.3876703792343,247.762477814527,31.6432842964434)) ;
#80551=CARTESIAN_POINT('Ctrl Pts',(49.3966525635991,247.887497453901,31.6432842964434)) ;
#80552=CARTESIAN_POINT('Ctrl Pts',(49.4279714952411,248.020314617985,31.6432842964434)) ;
#80553=CARTESIAN_POINT('Ctrl Pts',(49.468857501104,248.124759718921,31.6432842964434)) ;
#80554=CARTESIAN_POINT('Ctrl Pts',(49.5332946362515,248.239961500277,31.6432842964434)) ;
#80555=CARTESIAN_POINT('Ctrl Pts',(49.6081351537844,248.335445899508,31.6432842964434)) ;
#80556=CARTESIAN_POINT('Ctrl Pts',(49.6512710987205,248.391307577376,31.6432842964434)) ;
#80557=CARTESIAN_POINT('Ctrl Pts',(49.4446096612768,247.68481084764,31.6213203435596)) ;
#80558=CARTESIAN_POINT('Ctrl Pts',(49.450375211021,247.757501540984,31.6213203435596)) ;
#80559=CARTESIAN_POINT('Ctrl Pts',(49.4593850671176,247.879972198323,31.6213203435596)) ;
#80560=CARTESIAN_POINT('Ctrl Pts',(49.4886840834143,248.002844395605,31.6213203435596)) ;
#80561=CARTESIAN_POINT('Ctrl Pts',(49.5253667039704,248.096548590802,31.6213203435596)) ;
#80562=CARTESIAN_POINT('Ctrl Pts',(49.5847592850748,248.203341158271,31.6213203435596)) ;
#80563=CARTESIAN_POINT('Ctrl Pts',(49.6579185843663,248.296995382265,31.6213203435596)) ;
#80564=CARTESIAN_POINT('Ctrl Pts',(49.7010531372608,248.352839039806,31.6213203435596)) ;
#80565=CARTESIAN_POINT('Ctrl Pts',(49.4714537670856,247.682687695253,31.6213203435596)) ;
#80566=CARTESIAN_POINT('Ctrl Pts',(49.4772012130244,247.755355605436,31.6213203435596)) ;
#80567=CARTESIAN_POINT('Ctrl Pts',(49.4862294221888,247.876752186485,31.6213203435596)) ;
#80568=CARTESIAN_POINT('Ctrl Pts',(49.5146718619417,247.995378904774,31.6213203435596)) ;
#80569=CARTESIAN_POINT('Ctrl Pts',(49.549547538703,248.084463228595,31.6213203435596)) ;
#80570=CARTESIAN_POINT('Ctrl Pts',(49.6067817018178,248.187671186647,31.6213203435596)) ;
#80571=CARTESIAN_POINT('Ctrl Pts',(49.6792281363268,248.280556134621,31.6213203435596)) ;
#80572=CARTESIAN_POINT('Ctrl Pts',(49.7223606859683,248.336373859551,31.6213203435596)) ;
#80573=CARTESIAN_POINT('',(49.6274070383127,248.40974827469,31.7413203435596)) ;
#80574=CARTESIAN_POINT('Ctrl Pts',(49.6274070383129,248.40974827469,31.7413203435597)) ;
#80575=CARTESIAN_POINT('Ctrl Pts',(49.5842744886713,248.353930549759,31.7413203435597)) ;
#80576=CARTESIAN_POINT('Ctrl Pts',(49.5086086325514,248.25752820517,31.7413203435597)) ;
#80577=CARTESIAN_POINT('Ctrl Pts',(49.4417511608872,248.138252930567,31.7413203435597)) ;
#80578=CARTESIAN_POINT('Ctrl Pts',(49.3988727594182,248.028724139293,31.7413203435597)) ;
#80579=CARTESIAN_POINT('Ctrl Pts',(49.3665625013471,247.891107509426,31.7413203435596)) ;
#80580=CARTESIAN_POINT('Ctrl Pts',(49.3575747933183,247.764817090958,31.7413203435596)) ;
#80581=CARTESIAN_POINT('Ctrl Pts',(49.3518273473795,247.692149180776,31.7413203435596)) ;
#80582=CARTESIAN_POINT('Ctrl Pts',(49.7134632100808,248.324868293052,31.6213203435596)) ;
#80583=CARTESIAN_POINT('Ctrl Pts',(49.7132559890637,248.325072106525,31.6213203435596)) ;
#80584=CARTESIAN_POINT('Ctrl Pts',(49.7130468330129,248.325278354732,31.621321434825)) ;
#80585=CARTESIAN_POINT('Ctrl Pts',(49.712837678588,248.325484601394,31.6213236383315)) ;
#80586=CARTESIAN_POINT('Ctrl Pts',(49.7063180337272,248.331913607096,31.6213923248027)) ;
#80587=CARTESIAN_POINT('Ctrl Pts',(49.6998357440119,248.338305723809,31.6225297303056)) ;
#80588=CARTESIAN_POINT('Ctrl Pts',(49.6935146400323,248.344538332334,31.6246496199846)) ;
#80589=CARTESIAN_POINT('Ctrl Pts',(49.6886750426664,248.349310175338,31.6262726612349)) ;
#80590=CARTESIAN_POINT('Ctrl Pts',(49.6839295209328,248.353988818993,31.628472662309)) ;
#80591=CARTESIAN_POINT('Ctrl Pts',(49.6793363545858,248.358517816042,31.6312289392204)) ;
#80592=CARTESIAN_POINT('Ctrl Pts',(49.6733673312916,248.364403448488,31.6348108432593)) ;
#80593=CARTESIAN_POINT('Ctrl Pts',(49.6677194483372,248.36997314875,31.6392916211414)) ;
#80594=CARTESIAN_POINT('Ctrl Pts',(49.6625123775627,248.375115188156,31.6446092618829)) ;
#80595=CARTESIAN_POINT('Ctrl Pts',(49.6615906227216,248.376025431155,31.6455505898019)) ;
#80596=CARTESIAN_POINT('Ctrl Pts',(49.6606827178263,248.376922252148,31.6465182725826)) ;
#80597=CARTESIAN_POINT('Ctrl Pts',(49.6597893874932,248.377804993748,31.647512135677)) ;
#80598=CARTESIAN_POINT('Ctrl Pts',(49.6597891089285,248.377805269011,31.6475124455905)) ;
#80599=CARTESIAN_POINT('Ctrl Pts',(49.6597888303653,248.377805544272,31.6475127555065)) ;
#80600=CARTESIAN_POINT('Ctrl Pts',(49.6597885518034,248.377805819532,31.6475130654251)) ;
#80601=CARTESIAN_POINT('Ctrl Pts',(49.657032152052,248.380529548023,31.6505797438691)) ;
#80602=CARTESIAN_POINT('Ctrl Pts',(49.6544141961377,248.383119520525,31.6538954477906)) ;
#80603=CARTESIAN_POINT('Ctrl Pts',(49.6519440230935,248.385564616432,31.6574398704136)) ;
#80604=CARTESIAN_POINT('Ctrl Pts',(49.647394880906,248.390067575838,31.6639673817243)) ;
#80605=CARTESIAN_POINT('Ctrl Pts',(49.6433948408339,248.39403132537,31.6711969715355)) ;
#80606=CARTESIAN_POINT('Ctrl Pts',(49.6400004957735,248.397389763697,31.6789765359587)) ;
#80607=CARTESIAN_POINT('Ctrl Pts',(49.6376234961975,248.399741618425,31.6844244267906)) ;
#80608=CARTESIAN_POINT('Ctrl Pts',(49.6355443643873,248.401795839926,31.6901429783145)) ;
#80609=CARTESIAN_POINT('Ctrl Pts',(49.633795270634,248.403518871082,31.6960817822648)) ;
#80610=CARTESIAN_POINT('Ctrl Pts',(49.6320218954418,248.405265821869,31.7021030304553)) ;
#80611=CARTESIAN_POINT('Ctrl Pts',(49.630602327527,248.406657503578,31.7083012694437)) ;
#80612=CARTESIAN_POINT('Ctrl Pts',(49.6295626123056,248.407669693824,31.7146126499384)) ;
#80613=CARTESIAN_POINT('Ctrl Pts',(49.6291545699323,248.408066933859,31.7170895884534)) ;
#80614=CARTESIAN_POINT('Ctrl Pts',(49.6288050733612,248.408405673376,31.7195840029885)) ;
#80615=CARTESIAN_POINT('Ctrl Pts',(49.6285134696779,248.408687250091,31.7220909516336)) ;
#80616=CARTESIAN_POINT('Ctrl Pts',(49.6277755257932,248.409399819331,31.7284351356344)) ;
#80617=CARTESIAN_POINT('Ctrl Pts',(49.6274070383132,248.40974827469,31.7348594076613)) ;
#80618=CARTESIAN_POINT('Ctrl Pts',(49.6274070383132,248.40974827469,31.7413203435596)) ;
#80619=CARTESIAN_POINT('Ctrl Pts',(49.6274070383123,248.409748274689,31.7413203435596)) ;
#80620=CARTESIAN_POINT('Ctrl Pts',(49.7312574008403,248.49230944133,31.7413203435596)) ;
#80621=CARTESIAN_POINT('Ctrl Pts',(49.8396524076077,248.582427489684,31.7413203435597)) ;
#80622=CARTESIAN_POINT('Ctrl Pts',(50.1474076999394,248.729045342162,31.7413203435597)) ;
#80623=CARTESIAN_POINT('Ctrl Pts',(50.3192350498477,248.753191697813,31.7413203435597)) ;
#80624=CARTESIAN_POINT('Ctrl Pts',(50.5991697276986,248.801611100965,31.7413203435596)) ;
#80625=CARTESIAN_POINT('Ctrl Pts',(50.7212519229577,248.822096521034,31.7413203435596)) ;
#80626=CARTESIAN_POINT('Ctrl Pts',(50.8433217843682,248.842867149778,31.7413203435596)) ;
#80627=CARTESIAN_POINT('Ctrl Pts',(49.6274070383123,248.409748274689,31.7323443645494)) ;
#80628=CARTESIAN_POINT('Ctrl Pts',(49.7312574008403,248.49230944133,31.7323443645494)) ;
#80629=CARTESIAN_POINT('Ctrl Pts',(49.8396524076077,248.582427489684,31.7323443645494)) ;
#80630=CARTESIAN_POINT('Ctrl Pts',(50.1474076999394,248.729045342162,31.7323443645494)) ;
#80631=CARTESIAN_POINT('Ctrl Pts',(50.3192350498477,248.753191697813,31.7323443645494)) ;
#80632=CARTESIAN_POINT('Ctrl Pts',(50.5991697276986,248.801611100965,31.7323443645494)) ;
#80633=CARTESIAN_POINT('Ctrl Pts',(50.7212519229577,248.822096521034,31.7323443645494)) ;
#80634=CARTESIAN_POINT('Ctrl Pts',(50.8433217843682,248.842867149778,31.7323443645494)) ;
#80635=CARTESIAN_POINT('Ctrl Pts',(49.6298309197071,248.406699372017,31.6964046663919)) ;
#80636=CARTESIAN_POINT('Ctrl Pts',(49.7337722606661,248.489158151831,31.6964046663919)) ;
#80637=CARTESIAN_POINT('Ctrl Pts',(49.8419061460976,248.579207835096,31.6964046663919)) ;
#80638=CARTESIAN_POINT('Ctrl Pts',(50.1484057708637,248.72514366954,31.6964046663919)) ;
#80639=CARTESIAN_POINT('Ctrl Pts',(50.3199044061097,248.749301688654,31.6964046663919)) ;
#80640=CARTESIAN_POINT('Ctrl Pts',(50.599825132755,248.797797189828,31.6964046663919)) ;
#80641=CARTESIAN_POINT('Ctrl Pts',(50.7219148934239,248.818219204104,31.6964046663919)) ;
#80642=CARTESIAN_POINT('Ctrl Pts',(50.8439751417561,248.839027340845,31.6964046663919)) ;
#80643=CARTESIAN_POINT('Ctrl Pts',(49.6518601569296,248.378989682767,31.6401779597124)) ;
#80644=CARTESIAN_POINT('Ctrl Pts',(49.7557604408709,248.461494668013,31.6401779597124)) ;
#80645=CARTESIAN_POINT('Ctrl Pts',(49.8625658822425,248.549845910284,31.6401779597124)) ;
#80646=CARTESIAN_POINT('Ctrl Pts',(50.1569996132661,248.690088864524,31.6401779597124)) ;
#80647=CARTESIAN_POINT('Ctrl Pts',(50.3258240494323,248.714502474362,31.6401779597124)) ;
#80648=CARTESIAN_POINT('Ctrl Pts',(50.6057825093676,248.762849060457,31.6401779597124)) ;
#80649=CARTESIAN_POINT('Ctrl Pts',(50.7278485375342,248.783338358162,31.6401779597124)) ;
#80650=CARTESIAN_POINT('Ctrl Pts',(50.8499131240851,248.804129568182,31.6401779597124)) ;
#80651=CARTESIAN_POINT('Ctrl Pts',(49.6853263616349,248.336893893275,31.6213203435596)) ;
#80652=CARTESIAN_POINT('Ctrl Pts',(49.7892736755946,248.419345951094,31.6213203435596)) ;
#80653=CARTESIAN_POINT('Ctrl Pts',(49.8939292891865,248.505252742644,31.6213203435596)) ;
#80654=CARTESIAN_POINT('Ctrl Pts',(50.1701152721836,248.636783501172,31.6213203435597)) ;
#80655=CARTESIAN_POINT('Ctrl Pts',(50.3348376474163,248.661566541191,31.6213203435596)) ;
#80656=CARTESIAN_POINT('Ctrl Pts',(50.6148326914291,248.709792850834,31.6213203435596)) ;
#80657=CARTESIAN_POINT('Ctrl Pts',(50.736874324539,248.730303242972,31.6213203435596)) ;
#80658=CARTESIAN_POINT('Ctrl Pts',(50.8589339417444,248.751113842222,31.6213203435596)) ;
#80659=CARTESIAN_POINT('Ctrl Pts',(49.7020837842334,248.315815407073,31.6213203435596)) ;
#80660=CARTESIAN_POINT('Ctrl Pts',(49.8059341467614,248.398376573714,31.6213203435596)) ;
#80661=CARTESIAN_POINT('Ctrl Pts',(49.9096583356794,248.482909816866,31.6213203435596)) ;
#80662=CARTESIAN_POINT('Ctrl Pts',(50.1766164005556,248.610148341557,31.6213203435597)) ;
#80663=CARTESIAN_POINT('Ctrl Pts',(50.339328262466,248.63513713406,31.6213203435596)) ;
#80664=CARTESIAN_POINT('Ctrl Pts',(50.6193644682054,248.68318651908,31.6213203435596)) ;
#80665=CARTESIAN_POINT('Ctrl Pts',(50.7413810446874,248.703796823408,31.6213203435596)) ;
#80666=CARTESIAN_POINT('Ctrl Pts',(50.863450906098,248.724567452152,31.6213203435596)) ;
#80667=CARTESIAN_POINT('',(50.4787115899697,248.780775843391,31.7413203435597)) ;
#80668=CARTESIAN_POINT('Ctrl Pts',(50.4787115899697,248.780775843391,31.7413203435597)) ;
#80669=CARTESIAN_POINT('Ctrl Pts',(50.3192144841703,248.75318880758,31.7413203435597)) ;
#80670=CARTESIAN_POINT('Ctrl Pts',(50.1473975700188,248.729040516162,31.7413203435597)) ;
#80671=CARTESIAN_POINT('Ctrl Pts',(49.8396524076077,248.582427489684,31.7413203435597)) ;
#80672=CARTESIAN_POINT('Ctrl Pts',(49.7312574008403,248.49230944133,31.7413203435596)) ;
#80673=CARTESIAN_POINT('Ctrl Pts',(49.6274070383123,248.409748274689,31.7413203435596)) ;
#80674=CARTESIAN_POINT('Ctrl Pts',(50.8634509060979,248.724567452152,31.6213203435596)) ;
#80675=CARTESIAN_POINT('Ctrl Pts',(50.8626007665065,248.724691643753,31.6213203435596)) ;
#80676=CARTESIAN_POINT('Ctrl Pts',(50.8617506188712,248.724815832774,31.6213212569625)) ;
#80677=CARTESIAN_POINT('Ctrl Pts',(50.7857444298763,248.735918471341,31.6214844105417)) ;
#80678=CARTESIAN_POINT('Ctrl Pts',(50.7110413428426,248.746835358112,31.6287307234378)) ;
#80679=CARTESIAN_POINT('Ctrl Pts',(50.5933441727746,248.764125424106,31.6532575437195)) ;
#80680=CARTESIAN_POINT('Ctrl Pts',(50.5540600843127,248.769941046334,31.6679370990345)) ;
#80681=CARTESIAN_POINT('Ctrl Pts',(50.5153142312762,248.775614320839,31.6899900308231)) ;
#80682=CARTESIAN_POINT('Ctrl Pts',(50.5011451295166,248.777681686943,31.6993930061635)) ;
#80683=CARTESIAN_POINT('Ctrl Pts',(50.4874117295432,248.77962254954,31.7157669263666)) ;
#80684=CARTESIAN_POINT('Ctrl Pts',(50.4841511122824,248.780071069011,31.7207255508811)) ;
#80685=CARTESIAN_POINT('Ctrl Pts',(50.4799059585844,248.780643053467,31.7309912272279)) ;
#80686=CARTESIAN_POINT('Ctrl Pts',(50.4787822579947,248.780788066527,31.7360662774667)) ;
#80687=CARTESIAN_POINT('Ctrl Pts',(50.4787822579947,248.780788066527,31.7413203435596)) ;
#80688=CARTESIAN_POINT('Ctrl Pts',(50.8102927712973,248.61698393713,31.7413203435596)) ;
#80689=CARTESIAN_POINT('Ctrl Pts',(50.6997202412544,248.67161897537,31.7413203435596)) ;
#80690=CARTESIAN_POINT('Ctrl Pts',(50.5890955276099,248.726159041176,31.7413203435596)) ;
#80691=CARTESIAN_POINT('Ctrl Pts',(50.4199680949566,248.80991384992,31.7413203435596)) ;
#80692=CARTESIAN_POINT('Ctrl Pts',(50.3572873056676,248.840130404076,31.7413203435596)) ;
#80693=CARTESIAN_POINT('Ctrl Pts',(50.2435365148802,248.91361297365,31.7413203435596)) ;
#80694=CARTESIAN_POINT('Ctrl Pts',(50.200394038611,248.947930936924,31.7413203435596)) ;
#80695=CARTESIAN_POINT('Ctrl Pts',(50.1594670058306,248.980007368928,31.7413203435596)) ;
#80696=CARTESIAN_POINT('Ctrl Pts',(50.8102927712973,248.61698393713,31.7054164275186)) ;
#80697=CARTESIAN_POINT('Ctrl Pts',(50.6997202412544,248.67161897537,31.7054164275186)) ;
#80698=CARTESIAN_POINT('Ctrl Pts',(50.5890955276099,248.726159041176,31.7054164275186)) ;
#80699=CARTESIAN_POINT('Ctrl Pts',(50.4199680949566,248.80991384992,31.7054164275186)) ;
#80700=CARTESIAN_POINT('Ctrl Pts',(50.3572873056676,248.840130404076,31.7054164275186)) ;
#80701=CARTESIAN_POINT('Ctrl Pts',(50.2435365148802,248.91361297365,31.7054164275186)) ;
#80702=CARTESIAN_POINT('Ctrl Pts',(50.200394038611,248.947930936924,31.7054164275186)) ;
#80703=CARTESIAN_POINT('Ctrl Pts',(50.1594670058306,248.980007368928,31.7054164275186)) ;
#80704=CARTESIAN_POINT('Ctrl Pts',(50.8236526539486,248.644022190848,31.6432843149836)) ;
#80705=CARTESIAN_POINT('Ctrl Pts',(50.7130834685387,248.698667433839,31.6432843149836)) ;
#80706=CARTESIAN_POINT('Ctrl Pts',(50.6024674717828,248.753214385732,31.6432843149835)) ;
#80707=CARTESIAN_POINT('Ctrl Pts',(50.4333332648237,248.836947603607,31.6432843149835)) ;
#80708=CARTESIAN_POINT('Ctrl Pts',(50.3715718870589,248.866830519993,31.6432843149835)) ;
#80709=CARTESIAN_POINT('Ctrl Pts',(50.2615666635795,248.937859766662,31.6432843149835)) ;
#80710=CARTESIAN_POINT('Ctrl Pts',(50.2190256737229,248.97169349187,31.6432843149835)) ;
#80711=CARTESIAN_POINT('Ctrl Pts',(50.1780708772915,249.003744462163,31.6432843149835)) ;
#80712=CARTESIAN_POINT('Ctrl Pts',(50.8515222485431,248.700425767835,31.6213203435597)) ;
#80713=CARTESIAN_POINT('Ctrl Pts',(50.7409516914641,248.755066825751,31.6213203435597)) ;
#80714=CARTESIAN_POINT('Ctrl Pts',(50.6303493540251,248.809644240723,31.6213203435596)) ;
#80715=CARTESIAN_POINT('Ctrl Pts',(50.4612001281632,248.89332970846,31.6213203435596)) ;
#80716=CARTESIAN_POINT('Ctrl Pts',(50.401338053989,248.922482324456,31.6213203435596)) ;
#80717=CARTESIAN_POINT('Ctrl Pts',(50.2991824066269,248.988460164396,31.6213203435596)) ;
#80718=CARTESIAN_POINT('Ctrl Pts',(50.2578231879838,249.021200188683,31.6213203435596)) ;
#80719=CARTESIAN_POINT('Ctrl Pts',(50.2168797777163,249.053261601091,31.6213203435596)) ;
#80720=CARTESIAN_POINT('Ctrl Pts',(50.8634509060979,248.724567452152,31.6213203435597)) ;
#80721=CARTESIAN_POINT('Ctrl Pts',(50.752878376055,248.779202490392,31.6213203435597)) ;
#80722=CARTESIAN_POINT('Ctrl Pts',(50.6422811339546,248.833795616323,31.6213203435596)) ;
#80723=CARTESIAN_POINT('Ctrl Pts',(50.4731253324676,248.917460196317,31.6213203435596)) ;
#80724=CARTESIAN_POINT('Ctrl Pts',(50.4140730966128,248.946294536072,31.6213203435596)) ;
#80725=CARTESIAN_POINT('Ctrl Pts',(50.3152831890075,249.010121308417,31.6213203435596)) ;
#80726=CARTESIAN_POINT('Ctrl Pts',(50.2744176758496,249.042379341516,31.6213203435596)) ;
#80727=CARTESIAN_POINT('Ctrl Pts',(50.2334906430692,249.07445577352,31.6213203435596)) ;
#80728=CARTESIAN_POINT('',(50.1594670058306,248.980007368928,31.7413203435597)) ;
#80729=CARTESIAN_POINT('Ctrl Pts',(50.1594670058306,248.980007368928,31.7413203435596)) ;
#80730=CARTESIAN_POINT('Ctrl Pts',(50.200394038611,248.947930936924,31.7413203435596)) ;
#80731=CARTESIAN_POINT('Ctrl Pts',(50.2435365148802,248.91361297365,31.7413203435596)) ;
#80732=CARTESIAN_POINT('Ctrl Pts',(50.3572882948742,248.840129765052,31.7413203435596)) ;
#80733=CARTESIAN_POINT('Ctrl Pts',(50.4199700498958,248.809912907504,31.7413203435596)) ;
#80734=CARTESIAN_POINT('Ctrl Pts',(50.4787034919505,248.780827072781,31.7413203435596)) ;
#80735=CARTESIAN_POINT('Ctrl Pts',(50.2391706755516,249.070003231659,31.6213203435618)) ;
#80736=CARTESIAN_POINT('Ctrl Pts',(50.2389769980947,249.069784524285,31.6213203453679)) ;
#80737=CARTESIAN_POINT('Ctrl Pts',(50.2387833183675,249.069565814233,31.6213214511405)) ;
#80738=CARTESIAN_POINT('Ctrl Pts',(50.238589640211,249.0693471058,31.6213236583075)) ;
#80739=CARTESIAN_POINT('Ctrl Pts',(50.2325500741904,249.062527007738,31.6213924855366)) ;
#80740=CARTESIAN_POINT('Ctrl Pts',(50.2265461170565,249.055746946487,31.6225272947468)) ;
#80741=CARTESIAN_POINT('Ctrl Pts',(50.2206919611659,249.049135822006,31.6246433236309)) ;
#80742=CARTESIAN_POINT('Ctrl Pts',(50.2163057580144,249.044182463132,31.6262287499046)) ;
#80743=CARTESIAN_POINT('Ctrl Pts',(50.2120033490246,249.039323554314,31.6283662815162)) ;
#80744=CARTESIAN_POINT('Ctrl Pts',(50.2078355499091,249.034616864949,31.6310388202893)) ;
#80745=CARTESIAN_POINT('Ctrl Pts',(50.202281776799,249.028344997206,31.6346000941325)) ;
#80746=CARTESIAN_POINT('Ctrl Pts',(50.19702779249,249.02241192312,31.6390704274001)) ;
#80747=CARTESIAN_POINT('Ctrl Pts',(50.1921876023166,249.016948821135,31.6443896684161)) ;
#80748=CARTESIAN_POINT('Ctrl Pts',(50.1912650232226,249.01590751005,31.6454035584456)) ;
#80749=CARTESIAN_POINT('Ctrl Pts',(50.1903575198512,249.014883327718,31.6464484265654)) ;
#80750=CARTESIAN_POINT('Ctrl Pts',(50.1894659542635,249.013877275703,31.6475240412048)) ;
#80751=CARTESIAN_POINT('Ctrl Pts',(50.1869901882417,249.011083595204,31.6505108884023)) ;
#80752=CARTESIAN_POINT('Ctrl Pts',(50.1846371791155,249.008429537609,31.6537346511774)) ;
#80753=CARTESIAN_POINT('Ctrl Pts',(50.1824152135107,249.00592359253,31.657173440575)) ;
#80754=CARTESIAN_POINT('Ctrl Pts',(50.1781917651573,249.001160364154,31.6637097926173)) ;
#80755=CARTESIAN_POINT('Ctrl Pts',(50.1744871031225,248.996983069825,31.6709481856542)) ;
#80756=CARTESIAN_POINT('Ctrl Pts',(50.171343329535,248.99343577979,31.6787187785384)) ;
#80757=CARTESIAN_POINT('Ctrl Pts',(50.1691228001679,248.99093023622,31.6842073511783)) ;
#80758=CARTESIAN_POINT('Ctrl Pts',(50.1671824809342,248.988739496791,31.6899625615029)) ;
#80759=CARTESIAN_POINT('Ctrl Pts',(50.1655454659138,248.986889652768,31.6959327580786)) ;
#80760=CARTESIAN_POINT('Ctrl Pts',(50.1632490573667,248.984294687192,31.7043077639729)) ;
#80761=CARTESIAN_POINT('Ctrl Pts',(50.1615738177969,248.9823977985,31.7130122682104)) ;
#80762=CARTESIAN_POINT('Ctrl Pts',(50.1605681194369,248.981257369768,31.7218950515951)) ;
#80763=CARTESIAN_POINT('Ctrl Pts',(50.1598435441663,248.980435725336,31.7282948285366)) ;
#80764=CARTESIAN_POINT('Ctrl Pts',(50.1594670058305,248.980007368928,31.7347878978623)) ;
#80765=CARTESIAN_POINT('Ctrl Pts',(50.1594670058305,248.980007368928,31.7413203435596)) ;
#80766=CARTESIAN_POINT('Ctrl Pts',(50.1594670058305,248.980007368928,31.7413203435596)) ;
#80767=CARTESIAN_POINT('Ctrl Pts',(50.0843680110922,249.055035615032,31.7413203435596)) ;
#80768=CARTESIAN_POINT('Ctrl Pts',(50.0065782182602,249.132219046747,31.7413203435596)) ;
#80769=CARTESIAN_POINT('Ctrl Pts',(49.8534401351876,249.315445306648,31.7413203435596)) ;
#80770=CARTESIAN_POINT('Ctrl Pts',(49.7859212949379,249.415459142134,31.7413203435596)) ;
#80771=CARTESIAN_POINT('Ctrl Pts',(49.7201766015107,249.512067336446,31.7413203435596)) ;
#80772=CARTESIAN_POINT('Ctrl Pts',(50.1594670058305,248.980007368928,31.7054164275186)) ;
#80773=CARTESIAN_POINT('Ctrl Pts',(50.0843680110922,249.055035615032,31.7054164275186)) ;
#80774=CARTESIAN_POINT('Ctrl Pts',(50.0065782182602,249.132219046747,31.7054164275186)) ;
#80775=CARTESIAN_POINT('Ctrl Pts',(49.8534401351876,249.315445306648,31.7054164275186)) ;
#80776=CARTESIAN_POINT('Ctrl Pts',(49.7859212949379,249.415459142134,31.7054164275186)) ;
#80777=CARTESIAN_POINT('Ctrl Pts',(49.7201766015107,249.512067336446,31.7054164275186)) ;
#80778=CARTESIAN_POINT('Ctrl Pts',(50.1807824490313,249.001342911739,31.6432843125428)) ;
#80779=CARTESIAN_POINT('Ctrl Pts',(50.1057005592276,249.076389407655,31.6432843125428)) ;
#80780=CARTESIAN_POINT('Ctrl Pts',(50.0285181687661,249.153000953896,31.6432843125428)) ;
#80781=CARTESIAN_POINT('Ctrl Pts',(49.8779076504796,249.333206669877,31.6432843125428)) ;
#80782=CARTESIAN_POINT('Ctrl Pts',(49.8108769739463,249.432442440653,31.6432843125428)) ;
#80783=CARTESIAN_POINT('Ctrl Pts',(49.7451095799621,249.529034955354,31.6432843125428)) ;
#80784=CARTESIAN_POINT('Ctrl Pts',(50.2252478710253,249.045850262847,31.6213203435596)) ;
#80785=CARTESIAN_POINT('Ctrl Pts',(50.1501589665769,249.12088927461,31.6213203435596)) ;
#80786=CARTESIAN_POINT('Ctrl Pts',(50.0742782369067,249.19635189491,31.6213203435596)) ;
#80787=CARTESIAN_POINT('Ctrl Pts',(49.9289401473877,249.370244565953,31.6213203435596)) ;
#80788=CARTESIAN_POINT('Ctrl Pts',(49.8628795039616,249.467831583956,31.6213203435596)) ;
#80789=CARTESIAN_POINT('Ctrl Pts',(49.7971214193578,249.564430528784,31.6213203435596)) ;
#80790=CARTESIAN_POINT('Ctrl Pts',(50.2442798226044,249.064900160794,31.6213203435596)) ;
#80791=CARTESIAN_POINT('Ctrl Pts',(50.1691808278661,249.139928406899,31.6213203435596)) ;
#80792=CARTESIAN_POINT('Ctrl Pts',(50.0938629713761,249.214906582534,31.6213203435596)) ;
#80793=CARTESIAN_POINT('Ctrl Pts',(49.9507815308594,249.386095173166,31.6213203435596)) ;
#80794=CARTESIAN_POINT('Ctrl Pts',(49.8851280584615,249.482972237687,31.6213203435596)) ;
#80795=CARTESIAN_POINT('Ctrl Pts',(49.8193833650344,249.579580431999,31.6213203435596)) ;
#80796=CARTESIAN_POINT('Ctrl Pts',(49.7201766015108,249.512067336446,31.7413203435596)) ;
#80797=CARTESIAN_POINT('Ctrl Pts',(49.7412297546283,249.481130891218,31.7413203435596)) ;
#80798=CARTESIAN_POINT('Ctrl Pts',(49.7624973652352,249.449872249108,31.7413203435596)) ;
#80799=CARTESIAN_POINT('Ctrl Pts',(49.7842924699231,249.41849608269,31.7413203435596)) ;
#80800=CARTESIAN_POINT('Ctrl Pts',(49.8052631549654,249.388306748287,31.7413203435596)) ;
#80801=CARTESIAN_POINT('Ctrl Pts',(49.8267219102803,249.358008385841,31.7413203435596)) ;
#80802=CARTESIAN_POINT('Ctrl Pts',(49.8489842023975,249.327813735828,31.7413203435596)) ;
#80803=CARTESIAN_POINT('Ctrl Pts',(49.8624112513967,249.309602446394,31.7413203435596)) ;
#80804=CARTESIAN_POINT('Ctrl Pts',(49.8761313232906,249.291429485407,31.7413203435596)) ;
#80805=CARTESIAN_POINT('Ctrl Pts',(49.8902211372196,249.273347763522,31.7413203435596)) ;
#80806=CARTESIAN_POINT('Ctrl Pts',(49.8972660441841,249.264306902579,31.7413203435596)) ;
#80807=CARTESIAN_POINT('Ctrl Pts',(49.9044034808366,249.25528892965,31.7413203435596)) ;
#80808=CARTESIAN_POINT('Ctrl Pts',(49.9116436307471,249.24630095175,31.7413203435596)) ;
#80809=CARTESIAN_POINT('Ctrl Pts',(49.9156613592195,249.24131331266,31.7413203435596)) ;
#80810=CARTESIAN_POINT('Ctrl Pts',(49.9197107244713,249.236334916271,31.7413203435596)) ;
#80811=CARTESIAN_POINT('Ctrl Pts',(49.9237935226235,249.231367023509,31.7413203435596)) ;
#80812=CARTESIAN_POINT('Ctrl Pts',(49.9265173803749,249.228052670777,31.7413203435596)) ;
#80813=CARTESIAN_POINT('Ctrl Pts',(49.9292561197825,249.224742993849,31.7413203435596)) ;
#80814=CARTESIAN_POINT('Ctrl Pts',(49.9320102844097,249.221438375634,31.7413203435596)) ;
#80815=CARTESIAN_POINT('Ctrl Pts',(49.9325671651966,249.22077019539,31.7413203435596)) ;
#80816=CARTESIAN_POINT('Ctrl Pts',(49.9331246769457,249.220102221623,31.7413203435596)) ;
#80817=CARTESIAN_POINT('Ctrl Pts',(49.933682823282,249.219434458619,31.7413203435596)) ;
#80818=CARTESIAN_POINT('Ctrl Pts',(49.9563305661004,249.192338831929,31.7413203435596)) ;
#80819=CARTESIAN_POINT('Ctrl Pts',(49.9794784000558,249.166234661918,31.7413203435596)) ;
#80820=CARTESIAN_POINT('Ctrl Pts',(50.0028581722231,249.140851884011,31.7413203435596)) ;
#80821=CARTESIAN_POINT('Ctrl Pts',(50.0270883697368,249.114545822612,31.7413203435596)) ;
#80822=CARTESIAN_POINT('Ctrl Pts',(50.0515679747535,249.089014828443,31.7413203435596)) ;
#80823=CARTESIAN_POINT('Ctrl Pts',(50.0760422400472,249.063994621682,31.7413203435596)) ;
#80824=CARTESIAN_POINT('Ctrl Pts',(50.1019094484869,249.037550399732,31.7413203435596)) ;
#80825=CARTESIAN_POINT('Ctrl Pts',(50.1277709218595,249.011676953172,31.7413203435596)) ;
#80826=CARTESIAN_POINT('Ctrl Pts',(50.1533699872708,248.986098890802,31.7413203435596)) ;
#80827=CARTESIAN_POINT('Ctrl Pts',(50.1554040022539,248.98406654465,31.7413203435596)) ;
#80828=CARTESIAN_POINT('Ctrl Pts',(50.1574363812323,248.982036080532,31.7413203435596)) ;
#80829=CARTESIAN_POINT('Ctrl Pts',(50.1594670058306,248.980007368928,31.7413203435596)) ;
#80830=CARTESIAN_POINT('Ctrl Pts',(50.4787029267366,248.780825931436,31.9213203435596)) ;
#80831=CARTESIAN_POINT('Ctrl Pts',(50.4787029267366,248.780825931436,31.5613203435596)) ;
#80832=CARTESIAN_POINT('Ctrl Pts',(50.4156447429845,248.811983636512,31.9213203435596)) ;
#80833=CARTESIAN_POINT('Ctrl Pts',(50.4156447429845,248.811983636512,31.5613203435596)) ;
#80834=CARTESIAN_POINT('Ctrl Pts',(50.3025555244799,248.867862196722,31.9213203435596)) ;
#80835=CARTESIAN_POINT('Ctrl Pts',(50.3025555244799,248.867862196722,31.5613203435596)) ;
#80836=CARTESIAN_POINT('Ctrl Pts',(50.2033540554537,248.945611033121,31.9213203435596)) ;
#80837=CARTESIAN_POINT('Ctrl Pts',(50.2033540554537,248.945611033121,31.5613203435596)) ;
#80838=CARTESIAN_POINT('Ctrl Pts',(50.1594670058306,248.980007368928,31.9213203435596)) ;
#80839=CARTESIAN_POINT('Ctrl Pts',(50.1594670058306,248.980007368928,31.5613203435596)) ;
#80840=CARTESIAN_POINT('',(50.1594669100106,248.980007221364,31.8013203435596)) ;
#80841=CARTESIAN_POINT('',(50.1594670058306,248.980007368928,31.9213203435596)) ;
#80842=CARTESIAN_POINT('',(50.4787029267368,248.780825931436,31.8013203435597)) ;
#80843=CARTESIAN_POINT('Ctrl Pts',(50.4787029267369,248.780825931436,31.8013203435597)) ;
#80844=CARTESIAN_POINT('Ctrl Pts',(50.4117018449641,248.813931863473,31.8013203435597)) ;
#80845=CARTESIAN_POINT('Ctrl Pts',(50.3493334652158,248.845229869203,31.8013203435597)) ;
#80846=CARTESIAN_POINT('Ctrl Pts',(50.2498264402701,248.909548117546,31.8013203435596)) ;
#80847=CARTESIAN_POINT('Ctrl Pts',(50.206102738199,248.943426094878,31.8013203435597)) ;
#80848=CARTESIAN_POINT('Ctrl Pts',(50.1594668438626,248.980007137034,31.8013203435596)) ;
#80849=CARTESIAN_POINT('',(50.4787029267366,248.780825931436,31.9213203435596)) ;
#80850=CARTESIAN_POINT('Ctrl Pts',(50.1594670058306,248.980007368928,31.9213203435596)) ;
#80851=CARTESIAN_POINT('Ctrl Pts',(50.1594670058306,248.980007368928,31.5613203435596)) ;
#80852=CARTESIAN_POINT('Ctrl Pts',(50.081681528341,249.057719566924,31.9213203435596)) ;
#80853=CARTESIAN_POINT('Ctrl Pts',(50.081681528341,249.057719566924,31.5613203435596)) ;
#80854=CARTESIAN_POINT('Ctrl Pts',(49.918276128975,249.220971026696,31.9213203435596)) ;
#80855=CARTESIAN_POINT('Ctrl Pts',(49.918276128975,249.220971026696,31.5613203435596)) ;
#80856=CARTESIAN_POINT('Ctrl Pts',(49.7882872096234,249.411982561231,31.9213203435596)) ;
#80857=CARTESIAN_POINT('Ctrl Pts',(49.7882872096234,249.411982561231,31.5613203435596)) ;
#80858=CARTESIAN_POINT('Ctrl Pts',(49.7201766015108,249.512067336446,31.9213203435596)) ;
#80859=CARTESIAN_POINT('Ctrl Pts',(49.7201766015108,249.512067336446,31.5613203435596)) ;
#80860=CARTESIAN_POINT('',(49.7201769331396,249.512066809238,31.8013203435596)) ;
#80861=CARTESIAN_POINT('',(49.7201766015108,249.512067336446,31.9213203435596)) ;
#80862=CARTESIAN_POINT('Ctrl Pts',(50.1594669089399,248.980007271912,31.8013203435596)) ;
#80863=CARTESIAN_POINT('Ctrl Pts',(50.0792905779469,249.06007991241,31.8013203435597)) ;
#80864=CARTESIAN_POINT('Ctrl Pts',(50.0018980651231,249.137814436292,31.8013203435595)) ;
#80865=CARTESIAN_POINT('Ctrl Pts',(49.8585798215644,249.30927447749,31.8013203435596)) ;
#80866=CARTESIAN_POINT('Ctrl Pts',(49.7903322846594,249.408934973886,31.801320343559)) ;
#80867=CARTESIAN_POINT('Ctrl Pts',(49.7201769220531,249.512066801696,31.8013203435596)) ;
#80868=CARTESIAN_POINT('Origin',(49.7201766015108,249.512067336446,31.9213203435596)) ;
#80869=CARTESIAN_POINT('',(49.0244056225832,250.600744087106,31.8013203435596)) ;
#80870=CARTESIAN_POINT('',(49.0244056225832,250.600744087106,31.9213203435596)) ;
#80871=CARTESIAN_POINT('',(52.5952189936417,245.013472390306,31.8013203435596)) ;
#80872=CARTESIAN_POINT('Origin',(49.0244056225832,250.600744087106,31.9213203435596)) ;
#80873=CARTESIAN_POINT('',(49.6901629806574,250.600744087106,31.8013203435596)) ;
#80874=CARTESIAN_POINT('',(49.6901629806574,250.600744087106,31.9213203435596)) ;
#80875=CARTESIAN_POINT('',(51.3622028112916,250.600744087106,31.8013203435596)) ;
#80876=CARTESIAN_POINT('Origin',(49.6901629806574,250.600744087106,31.9213203435596)) ;
#80877=CARTESIAN_POINT('',(50.2194942475374,249.76854761303,31.8013203435596)) ;
#80878=CARTESIAN_POINT('',(50.2194942475374,249.76854761303,31.9213203435596)) ;
#80879=CARTESIAN_POINT('',(52.8075349928054,245.69971866274,31.8013203435596)) ;
#80880=CARTESIAN_POINT('Ctrl Pts',(50.2194942475374,249.76854761303,31.9213203435596)) ;
#80881=CARTESIAN_POINT('Ctrl Pts',(50.2194942475374,249.76854761303,31.5613203435596)) ;
#80882=CARTESIAN_POINT('Ctrl Pts',(50.2886676861273,249.661674205943,31.9213203435596)) ;
#80883=CARTESIAN_POINT('Ctrl Pts',(50.2886676861273,249.661674205943,31.5613203435596)) ;
#80884=CARTESIAN_POINT('Ctrl Pts',(50.4101984552228,249.473908386807,31.9213203435596)) ;
#80885=CARTESIAN_POINT('Ctrl Pts',(50.4101984552228,249.473908386807,31.5613203435596)) ;
#80886=CARTESIAN_POINT('Ctrl Pts',(50.5438898116334,249.294625894933,31.9213203435596)) ;
#80887=CARTESIAN_POINT('Ctrl Pts',(50.5438898116334,249.294625894933,31.5613203435596)) ;
#80888=CARTESIAN_POINT('Ctrl Pts',(50.6014861107882,249.217388231164,31.9213203435596)) ;
#80889=CARTESIAN_POINT('Ctrl Pts',(50.6014861107882,249.217388231164,31.5613203435596)) ;
#80890=CARTESIAN_POINT('',(50.6014861107881,249.217388231164,31.8013203435596)) ;
#80891=CARTESIAN_POINT('',(50.6014861107882,249.217388231164,31.9213203435596)) ;
#80892=CARTESIAN_POINT('Ctrl Pts',(50.2194942475855,249.768547612949,31.8013203435596)) ;
#80893=CARTESIAN_POINT('Ctrl Pts',(50.2878275213723,249.662972234484,31.8013203435596)) ;
#80894=CARTESIAN_POINT('Ctrl Pts',(50.3569258709686,249.556106723648,31.8013203435596)) ;
#80895=CARTESIAN_POINT('Ctrl Pts',(50.4869845254695,249.370877841352,31.8013203435597)) ;
#80896=CARTESIAN_POINT('Ctrl Pts',(50.5445853180999,249.293693208364,31.8013203435597)) ;
#80897=CARTESIAN_POINT('Ctrl Pts',(50.6014861107882,249.217388231164,31.8013203435597)) ;
#80898=CARTESIAN_POINT('Ctrl Pts',(50.6014861107882,249.217388231164,31.9213203435596)) ;
#80899=CARTESIAN_POINT('Ctrl Pts',(50.6014861107882,249.217388231164,31.5613203435596)) ;
#80900=CARTESIAN_POINT('Ctrl Pts',(50.6467206773926,249.160912010444,31.9213203435596)) ;
#80901=CARTESIAN_POINT('Ctrl Pts',(50.6467206773926,249.160912010444,31.5613203435596)) ;
#80902=CARTESIAN_POINT('Ctrl Pts',(50.7265515411586,249.061241651674,31.9213203435596)) ;
#80903=CARTESIAN_POINT('Ctrl Pts',(50.7265515411586,249.061241651674,31.5613203435596)) ;
#80904=CARTESIAN_POINT('Ctrl Pts',(50.8277518319035,248.983628817758,31.9213203435596)) ;
#80905=CARTESIAN_POINT('Ctrl Pts',(50.8277518319035,248.983628817758,31.5613203435596)) ;
#80906=CARTESIAN_POINT('Ctrl Pts',(50.8716089964922,248.949993748075,31.9213203435596)) ;
#80907=CARTESIAN_POINT('Ctrl Pts',(50.8716089964922,248.949993748075,31.5613203435596)) ;
#80908=CARTESIAN_POINT('',(50.8716089964922,248.949993748075,31.8013203435596)) ;
#80909=CARTESIAN_POINT('',(50.8716089964922,248.949993748075,31.9213203435596)) ;
#80910=CARTESIAN_POINT('Ctrl Pts',(50.6014861107882,249.217388231164,31.8013203435596)) ;
#80911=CARTESIAN_POINT('Ctrl Pts',(50.6431307164356,249.165394145294,31.8013203435596)) ;
#80912=CARTESIAN_POINT('Ctrl Pts',(50.6869793943593,249.109198386675,31.8013203435596)) ;
#80913=CARTESIAN_POINT('Ctrl Pts',(50.7876909072677,249.01365071099,31.8013203435596)) ;
#80914=CARTESIAN_POINT('Ctrl Pts',(50.8311952099577,248.980988011817,31.8013203435596)) ;
#80915=CARTESIAN_POINT('Ctrl Pts',(50.8716089964922,248.949993748075,31.8013203435596)) ;
#80916=CARTESIAN_POINT('Ctrl Pts',(50.8716089964922,248.949993748075,31.9213203435596)) ;
#80917=CARTESIAN_POINT('Ctrl Pts',(50.8716089964922,248.949993748075,31.5613203435596)) ;
#80918=CARTESIAN_POINT('Ctrl Pts',(50.9103827599137,248.926600394466,31.9213203435596)) ;
#80919=CARTESIAN_POINT('Ctrl Pts',(50.9103827599137,248.926600394466,31.5613203435596)) ;
#80920=CARTESIAN_POINT('Ctrl Pts',(50.9859582056058,248.881003501896,31.9213203435596)) ;
#80921=CARTESIAN_POINT('Ctrl Pts',(50.9859582056058,248.881003501896,31.5613203435596)) ;
#80922=CARTESIAN_POINT('Ctrl Pts',(51.0705337876061,248.855836848551,31.9213203435596)) ;
#80923=CARTESIAN_POINT('Ctrl Pts',(51.0705337876061,248.855836848551,31.5613203435596)) ;
#80924=CARTESIAN_POINT('Ctrl Pts',(51.1117181123312,248.84358187378,31.9213203435596)) ;
#80925=CARTESIAN_POINT('Ctrl Pts',(51.1117181123312,248.84358187378,31.5613203435596)) ;
#80926=CARTESIAN_POINT('',(51.1117181123312,248.84358187378,31.8013203435596)) ;
#80927=CARTESIAN_POINT('',(51.1117181123312,248.84358187378,31.9213203435596)) ;
#80928=CARTESIAN_POINT('Ctrl Pts',(50.8716089964922,248.949993748075,31.8013203435596)) ;
#80929=CARTESIAN_POINT('Ctrl Pts',(50.8812952192372,248.944149764571,31.8013203435596)) ;
#80930=CARTESIAN_POINT('Ctrl Pts',(50.8912297604164,248.938152275578,31.8013203435596)) ;
#80931=CARTESIAN_POINT('Ctrl Pts',(50.9015589132419,248.93203979987,31.8013203435596)) ;
#80932=CARTESIAN_POINT('Ctrl Pts',(50.9109223604925,248.926498799091,31.8013203435596)) ;
#80933=CARTESIAN_POINT('Ctrl Pts',(50.920609761348,248.920862580329,31.8013203435596)) ;
#80934=CARTESIAN_POINT('Ctrl Pts',(50.9307457548408,248.915195388481,31.8013203435596)) ;
#80935=CARTESIAN_POINT('Ctrl Pts',(50.93981037248,248.910127219561,31.8013203435596)) ;
#80936=CARTESIAN_POINT('Ctrl Pts',(50.9492336152923,248.905033946057,31.8013203435596)) ;
#80937=CARTESIAN_POINT('Ctrl Pts',(50.9591206958319,248.899997988403,31.8013203435596)) ;
#80938=CARTESIAN_POINT('Ctrl Pts',(50.9640642361016,248.897480009576,31.8013203435596)) ;
#80939=CARTESIAN_POINT('Ctrl Pts',(50.9691240113763,248.894976985261,31.8013203435596)) ;
#80940=CARTESIAN_POINT('Ctrl Pts',(50.9743151389776,248.892503680254,31.8013203435596)) ;
#80941=CARTESIAN_POINT('Ctrl Pts',(50.9769107027783,248.89126702775,31.8013203435596)) ;
#80942=CARTESIAN_POINT('Ctrl Pts',(50.9795391276914,248.890037857353,31.8013203435596)) ;
#80943=CARTESIAN_POINT('Ctrl Pts',(50.9822024529822,248.888818354254,31.8013203435596)) ;
#80944=CARTESIAN_POINT('Ctrl Pts',(50.9838480634011,248.888064849973,31.8013203435596)) ;
#80945=CARTESIAN_POINT('Ctrl Pts',(50.9855069998973,248.887315041046,31.8013203435596)) ;
#80946=CARTESIAN_POINT('Ctrl Pts',(50.987179764526,248.886569490637,31.8013203435596)) ;
#80947=CARTESIAN_POINT('Ctrl Pts',(50.9882142727061,248.886108410827,31.8013203435596)) ;
#80948=CARTESIAN_POINT('Ctrl Pts',(50.9892540707111,248.885648960224,31.8013203435596)) ;
#80949=CARTESIAN_POINT('Ctrl Pts',(50.9902992785986,248.885191280252,31.8013203435596)) ;
#80950=CARTESIAN_POINT('Ctrl Pts',(51.0004197047703,248.880759705994,31.8013203435596)) ;
#80951=CARTESIAN_POINT('Ctrl Pts',(51.0102980961467,248.876817277561,31.8013203435596)) ;
#80952=CARTESIAN_POINT('Ctrl Pts',(51.019926996519,248.873209346358,31.8013203435596)) ;
#80953=CARTESIAN_POINT('Ctrl Pts',(51.0307051781765,248.869170781577,31.8013203435596)) ;
#80954=CARTESIAN_POINT('Ctrl Pts',(51.0411708920461,248.865551634723,31.8013203435596)) ;
#80955=CARTESIAN_POINT('Ctrl Pts',(51.0513403827163,248.862195622714,31.8013203435596)) ;
#80956=CARTESIAN_POINT('Ctrl Pts',(51.0624470976921,248.858530319303,31.8013203435596)) ;
#80957=CARTESIAN_POINT('Ctrl Pts',(51.0732008410539,248.855179721503,31.8013203435596)) ;
#80958=CARTESIAN_POINT('Ctrl Pts',(51.0836485698134,248.851998785607,31.8013203435596)) ;
#80959=CARTESIAN_POINT('Ctrl Pts',(51.0932464252134,248.849076603814,31.8013203435596)) ;
#80960=CARTESIAN_POINT('Ctrl Pts',(51.1025866694188,248.846299062984,31.8013203435596)) ;
#80961=CARTESIAN_POINT('Ctrl Pts',(51.1117181123312,248.84358187378,31.8013203435596)) ;
#80962=CARTESIAN_POINT('Ctrl Pts',(51.1117181123312,248.84358187378,31.9213203435596)) ;
#80963=CARTESIAN_POINT('Ctrl Pts',(51.1117181123312,248.84358187378,31.5613203435596)) ;
#80964=CARTESIAN_POINT('Ctrl Pts',(51.1512264477684,248.83805994343,31.9213203435596)) ;
#80965=CARTESIAN_POINT('Ctrl Pts',(51.1512264477684,248.83805994343,31.5613203435596)) ;
#80966=CARTESIAN_POINT('Ctrl Pts',(51.2489154900931,248.824406316121,31.9213203435596)) ;
#80967=CARTESIAN_POINT('Ctrl Pts',(51.2489154900931,248.824406316121,31.5613203435596)) ;
#80968=CARTESIAN_POINT('Ctrl Pts',(51.3476150025798,248.824453851025,31.9213203435596)) ;
#80969=CARTESIAN_POINT('Ctrl Pts',(51.3476150025798,248.824453851025,31.5613203435596)) ;
#80970=CARTESIAN_POINT('Ctrl Pts',(51.4063975156363,248.824482161408,31.9213203435596)) ;
#80971=CARTESIAN_POINT('Ctrl Pts',(51.4063975156363,248.824482161408,31.5613203435596)) ;
#80972=CARTESIAN_POINT('',(51.4063975156363,248.824482161408,31.8013203435597)) ;
#80973=CARTESIAN_POINT('',(51.4063975156363,248.824482161408,31.9213203435596)) ;
#80974=CARTESIAN_POINT('Ctrl Pts',(51.1117181123309,248.84358187378,31.8013203435596)) ;
#80975=CARTESIAN_POINT('Ctrl Pts',(51.1489587152535,248.838376895812,31.8013203435596)) ;
#80976=CARTESIAN_POINT('Ctrl Pts',(51.1881361258901,248.832747914847,31.8013203435596)) ;
#80977=CARTESIAN_POINT('Ctrl Pts',(51.2926723949292,248.824120149349,31.8013203435596)) ;
#80978=CARTESIAN_POINT('Ctrl Pts',(51.3510126858065,248.824455380393,31.8013203435596)) ;
#80979=CARTESIAN_POINT('Ctrl Pts',(51.4063975153673,248.82448216138,31.8013203435596)) ;
#80980=CARTESIAN_POINT('Origin',(51.4063975156363,248.824482161408,31.9213203435596)) ;
#80981=CARTESIAN_POINT('',(52.0203128398474,248.824482161408,31.8013203435596)) ;
#80982=CARTESIAN_POINT('',(52.0203128398474,248.824482161408,31.9213203435596)) ;
#80983=CARTESIAN_POINT('',(52.5531987578181,248.824482161408,31.8013203435596)) ;
#80984=CARTESIAN_POINT('Ctrl Pts',(50.3149922133507,248.292422193891,31.8013203435596)) ;
#80985=CARTESIAN_POINT('Ctrl Pts',(50.2828566975655,248.278143008832,31.8013203435596)) ;
#80986=CARTESIAN_POINT('Ctrl Pts',(50.2258386057601,248.25332520896,31.8013203435596)) ;
#80987=CARTESIAN_POINT('Ctrl Pts',(50.1613818919158,248.214949841468,31.8013203435596)) ;
#80988=CARTESIAN_POINT('Ctrl Pts',(50.0979033745595,248.164702269118,31.8013203435596)) ;
#80989=CARTESIAN_POINT('Ctrl Pts',(50.0534676836831,248.11466854703,31.8013203435596)) ;
#80990=CARTESIAN_POINT('Ctrl Pts',(50.0176214060562,248.069618732724,31.8013203435596)) ;
#80991=CARTESIAN_POINT('Ctrl Pts',(50.003941798311,248.05231292904,31.8013203435596)) ;
#80992=CARTESIAN_POINT('Ctrl Pts',(50.3149922133507,248.292422193891,31.8372242596007)) ;
#80993=CARTESIAN_POINT('Ctrl Pts',(50.2828566975655,248.278143008832,31.8372242596007)) ;
#80994=CARTESIAN_POINT('Ctrl Pts',(50.2258386057601,248.25332520896,31.8372242596007)) ;
#80995=CARTESIAN_POINT('Ctrl Pts',(50.1613818919158,248.214949841468,31.8372242596007)) ;
#80996=CARTESIAN_POINT('Ctrl Pts',(50.0979033745595,248.164702269118,31.8372242596007)) ;
#80997=CARTESIAN_POINT('Ctrl Pts',(50.0534676836831,248.11466854703,31.8372242596007)) ;
#80998=CARTESIAN_POINT('Ctrl Pts',(50.0176214060562,248.069618732724,31.8372242596007)) ;
#80999=CARTESIAN_POINT('Ctrl Pts',(50.003941798311,248.05231292904,31.8372242596007)) ;
#81000=CARTESIAN_POINT('Ctrl Pts',(50.3272385223701,248.264861695502,31.899356381536)) ;
#81001=CARTESIAN_POINT('Ctrl Pts',(50.2950567106523,248.250556344248,31.899356381536)) ;
#81002=CARTESIAN_POINT('Ctrl Pts',(50.2389374113449,248.226061625423,31.8993563815361)) ;
#81003=CARTESIAN_POINT('Ctrl Pts',(50.1779829811741,248.189696416539,31.899356381536)) ;
#81004=CARTESIAN_POINT('Ctrl Pts',(50.119312163611,248.143252734766,31.8993563815361)) ;
#81005=CARTESIAN_POINT('Ctrl Pts',(50.0767223473644,248.09547863182,31.899356381536)) ;
#81006=CARTESIAN_POINT('Ctrl Pts',(50.0412434526266,248.050937221671,31.8993563815361)) ;
#81007=CARTESIAN_POINT('Ctrl Pts',(50.0276015247282,248.033610776707,31.899356381536)) ;
#81008=CARTESIAN_POINT('Ctrl Pts',(50.3527851388875,248.207368659663,31.9213203435596)) ;
#81009=CARTESIAN_POINT('Ctrl Pts',(50.3206223108221,248.19307403786,31.9213203435596)) ;
#81010=CARTESIAN_POINT('Ctrl Pts',(50.2662434470315,248.169222377751,31.9213203435596)) ;
#81011=CARTESIAN_POINT('Ctrl Pts',(50.2127147686324,248.136999504271,31.9213203435596)) ;
#81012=CARTESIAN_POINT('Ctrl Pts',(50.1640396297653,248.098510538817,31.9213203435596)) ;
#81013=CARTESIAN_POINT('Ctrl Pts',(50.1251782969651,248.055475583572,31.9213203435596)) ;
#81014=CARTESIAN_POINT('Ctrl Pts',(50.0906146688733,248.011914821926,31.9213203435596)) ;
#81015=CARTESIAN_POINT('Ctrl Pts',(50.0769572903495,247.994596840921,31.9213203435596)) ;
#81016=CARTESIAN_POINT('Ctrl Pts',(50.3637195211995,248.182760671606,31.9213203435596)) ;
#81017=CARTESIAN_POINT('Ctrl Pts',(50.3315840054143,248.168481486547,31.9213203435596)) ;
#81018=CARTESIAN_POINT('Ctrl Pts',(50.277927744792,248.144899934299,31.9213203435596)) ;
#81019=CARTESIAN_POINT('Ctrl Pts',(50.2275972966819,248.11444158417,31.9213203435596)) ;
#81020=CARTESIAN_POINT('Ctrl Pts',(50.1831949139989,248.079360616833,31.9213203435596)) ;
#81021=CARTESIAN_POINT('Ctrl Pts',(50.1459091564747,248.038358319183,31.9213203435596)) ;
#81022=CARTESIAN_POINT('Ctrl Pts',(50.1117619973904,247.995204022732,31.9213203435596)) ;
#81023=CARTESIAN_POINT('Ctrl Pts',(50.0980823896452,247.977898219048,31.9213203435596)) ;
#81024=CARTESIAN_POINT('',(50.1042746584503,247.985728410081,31.9213203435596)) ;
#81025=CARTESIAN_POINT('',(50.3549396358571,248.178860256982,31.9213203435596)) ;
#81026=CARTESIAN_POINT('Ctrl Pts',(50.104281874783,247.985736529947,31.9213203435596)) ;
#81027=CARTESIAN_POINT('Ctrl Pts',(50.1158999239824,248.000411090002,31.9213203435596)) ;
#81028=CARTESIAN_POINT('Ctrl Pts',(50.1481620304608,248.040835753353,31.9213203435596)) ;
#81029=CARTESIAN_POINT('Ctrl Pts',(50.1831949139989,248.079360616833,31.9213203435596)) ;
#81030=CARTESIAN_POINT('Ctrl Pts',(50.2275972966819,248.11444158417,31.9213203435596)) ;
#81031=CARTESIAN_POINT('Ctrl Pts',(50.2751776277953,248.143235652944,31.9213203435596)) ;
#81032=CARTESIAN_POINT('Ctrl Pts',(50.3257302482811,248.165883905264,31.9213203435596)) ;
#81033=CARTESIAN_POINT('Ctrl Pts',(50.3549394017728,248.178860783873,31.9213203435596)) ;
#81034=CARTESIAN_POINT('Ctrl Pts',(50.3549344338646,248.178858576757,31.9213203435596)) ;
#81035=CARTESIAN_POINT('Ctrl Pts',(50.3548372871676,248.179134233402,31.9213203435596)) ;
#81036=CARTESIAN_POINT('Ctrl Pts',(50.3547401430246,248.17940989064,31.9213192415563)) ;
#81037=CARTESIAN_POINT('Ctrl Pts',(50.3493944802537,248.194579224157,31.9211981003872)) ;
#81038=CARTESIAN_POINT('Ctrl Pts',(50.3441572278943,248.209463608499,31.9178698499865)) ;
#81039=CARTESIAN_POINT('Ctrl Pts',(50.3352855015944,248.234691751609,31.9066093082206)) ;
#81040=CARTESIAN_POINT('Ctrl Pts',(50.3308425838642,248.247332713497,31.8987051026052)) ;
#81041=CARTESIAN_POINT('Ctrl Pts',(50.3231419161368,248.269243109216,31.8753017780563)) ;
#81042=CARTESIAN_POINT('Ctrl Pts',(50.3202611501902,248.277438595027,31.8623013765578)) ;
#81043=CARTESIAN_POINT('Ctrl Pts',(50.3171983030722,248.286149604156,31.8408116482204)) ;
#81044=CARTESIAN_POINT('Ctrl Pts',(50.3163832809431,248.288467128432,31.8331147727513)) ;
#81045=CARTESIAN_POINT('Ctrl Pts',(50.3152798692463,248.291604448919,31.817383920378)) ;
#81046=CARTESIAN_POINT('Ctrl Pts',(50.3149922133517,248.292422193891,31.8093598799402)) ;
#81047=CARTESIAN_POINT('Ctrl Pts',(50.3149922133517,248.292422193891,31.8013203435596)) ;
#81048=CARTESIAN_POINT('',(50.003941798311,248.05231292904,31.8013203435596)) ;
#81049=CARTESIAN_POINT('Ctrl Pts',(50.3149922133507,248.292422193891,31.8013203435596)) ;
#81050=CARTESIAN_POINT('Ctrl Pts',(50.2828566975655,248.278143008832,31.8013203435596)) ;
#81051=CARTESIAN_POINT('Ctrl Pts',(50.2258386057601,248.25332520896,31.8013203435596)) ;
#81052=CARTESIAN_POINT('Ctrl Pts',(50.1613818919158,248.214949841468,31.8013203435596)) ;
#81053=CARTESIAN_POINT('Ctrl Pts',(50.0979033745595,248.164702269118,31.8013203435596)) ;
#81054=CARTESIAN_POINT('Ctrl Pts',(50.0534676836831,248.11466854703,31.8013203435596)) ;
#81055=CARTESIAN_POINT('Ctrl Pts',(50.0176214060562,248.069618732724,31.8013203435596)) ;
#81056=CARTESIAN_POINT('Ctrl Pts',(50.003941798311,248.05231292904,31.8013203435596)) ;
#81057=CARTESIAN_POINT('Ctrl Pts',(50.1042683656432,247.98571946673,31.9213203435596)) ;
#81058=CARTESIAN_POINT('Ctrl Pts',(50.1040250568153,247.985881647708,31.9213203435596)) ;
#81059=CARTESIAN_POINT('Ctrl Pts',(50.103781744389,247.986043822761,31.9213192416473)) ;
#81060=CARTESIAN_POINT('Ctrl Pts',(50.0903945513106,247.994966336622,31.9211981310143)) ;
#81061=CARTESIAN_POINT('Ctrl Pts',(50.0772500994751,248.003702769267,31.9178712311407)) ;
#81062=CARTESIAN_POINT('Ctrl Pts',(50.0549619051614,248.018496492087,31.9066113625708)) ;
#81063=CARTESIAN_POINT('Ctrl Pts',(50.0437921420014,248.025900949602,31.8987080028825)) ;
#81064=CARTESIAN_POINT('Ctrl Pts',(50.0244291337723,248.038731400036,31.8753079726832)) ;
#81065=CARTESIAN_POINT('Ctrl Pts',(50.0171854200934,248.043530970201,31.8623083641888)) ;
#81066=CARTESIAN_POINT('Ctrl Pts',(50.0094860730131,248.048635324575,31.8408181867668)) ;
#81067=CARTESIAN_POINT('Ctrl Pts',(50.0074375834509,248.04999390866,31.8331201559811)) ;
#81068=CARTESIAN_POINT('Ctrl Pts',(50.0046645494265,248.051833330652,31.8173867221349)) ;
#81069=CARTESIAN_POINT('Ctrl Pts',(50.0039417983113,248.05231292904,31.8093613191834)) ;
#81070=CARTESIAN_POINT('Ctrl Pts',(50.0039417983113,248.05231292904,31.8013203435596)) ;
#81071=CARTESIAN_POINT('Origin',(52.8601564199237,248.246092044717,31.8013203435596)) ;
#81072=CARTESIAN_POINT('',(50.8831605673865,248.24609204701,31.9213203435596)) ;
#81073=CARTESIAN_POINT('Ctrl Pts',(50.8825230539854,248.366092044717,31.8013203435596)) ;
#81074=CARTESIAN_POINT('Ctrl Pts',(50.8825536510344,248.366092044717,31.8103670376983)) ;
#81075=CARTESIAN_POINT('Ctrl Pts',(50.8825842480833,248.365064672731,31.8194133382866)) ;
#81076=CARTESIAN_POINT('Ctrl Pts',(50.8826454342939,248.361007859405,31.8370436695514)) ;
#81077=CARTESIAN_POINT('Ctrl Pts',(50.8826760234556,248.357979112739,31.8456270529255)) ;
#81078=CARTESIAN_POINT('Ctrl Pts',(50.8827371951202,248.350074944028,31.8618952684662)) ;
#81079=CARTESIAN_POINT('Ctrl Pts',(50.8827677776232,248.345200269069,31.8695795901304)) ;
#81080=CARTESIAN_POINT('Ctrl Pts',(50.8828289657752,248.333847798996,31.8836660555295)) ;
#81081=CARTESIAN_POINT('Ctrl Pts',(50.8828595714242,248.327369282324,31.8900666073448)) ;
#81082=CARTESIAN_POINT('Ctrl Pts',(50.8829207658452,248.313144950304,31.9012488492717)) ;
#81083=CARTESIAN_POINT('Ctrl Pts',(50.8829513546172,248.305400457158,31.9060309476799)) ;
#81084=CARTESIAN_POINT('Ctrl Pts',(50.8830125480013,248.28903157296,31.9137395592428)) ;
#81085=CARTESIAN_POINT('Ctrl Pts',(50.8830431526134,248.280407438849,31.9166647706729)) ;
#81086=CARTESIAN_POINT('Ctrl Pts',(50.8831026946499,248.263203725675,31.9204018086563)) ;
#81087=CARTESIAN_POINT('Ctrl Pts',(50.8831316320742,248.254648034126,31.9213203435596)) ;
#81088=CARTESIAN_POINT('Ctrl Pts',(50.8831605694985,248.246092044717,31.9213203435596)) ;
#81089=CARTESIAN_POINT('',(51.9003128398474,248.246092044717,31.9213203435596)) ;
#81090=CARTESIAN_POINT('',(52.8601564199237,248.246092044717,31.9213203435596)) ;
#81091=CARTESIAN_POINT('Origin',(51.9003128398474,248.246092044717,31.8013203435596)) ;
#81092=CARTESIAN_POINT('Origin',(52.2271414578465,247.162763132459,31.8013203435596)) ;
#81093=CARTESIAN_POINT('',(51.9003128398474,247.162763132459,31.9213203435596)) ;
#81094=CARTESIAN_POINT('',(50.7555332764365,247.162763109072,31.9213203435596)) ;
#81095=CARTESIAN_POINT('',(52.2271414578465,247.162763132459,31.9213203435596)) ;
#81096=CARTESIAN_POINT('Ctrl Pts',(50.755533264376,247.162763097565,31.9213203435596)) ;
#81097=CARTESIAN_POINT('Ctrl Pts',(50.7555302176641,247.162471459282,31.9213203435596)) ;
#81098=CARTESIAN_POINT('Ctrl Pts',(50.7555271710895,247.16217982651,31.9213192375922)) ;
#81099=CARTESIAN_POINT('Ctrl Pts',(50.7554291239828,247.152793158216,31.9212481256592)) ;
#81100=CARTESIAN_POINT('Ctrl Pts',(50.7553349634566,247.143760542052,31.9201111028397)) ;
#81101=CARTESIAN_POINT('Ctrl Pts',(50.7551748602209,247.128400885189,31.9164179948109)) ;
#81102=CARTESIAN_POINT('Ctrl Pts',(50.755107856334,247.12197273855,31.9142984267547)) ;
#81103=CARTESIAN_POINT('Ctrl Pts',(50.7549554578127,247.107355434576,31.9080931810874)) ;
#81104=CARTESIAN_POINT('Ctrl Pts',(50.754872649644,247.099417330385,31.903622605644)) ;
#81105=CARTESIAN_POINT('Ctrl Pts',(50.7547816212709,247.090676364211,31.8972777600414)) ;
#81106=CARTESIAN_POINT('Ctrl Pts',(50.7547671299866,247.089284262197,31.8962188977583)) ;
#81107=CARTESIAN_POINT('Ctrl Pts',(50.7547143583256,247.084211613134,31.892175500388)) ;
#81108=CARTESIAN_POINT('Ctrl Pts',(50.7546777262954,247.08068424247,31.8889917050932)) ;
#81109=CARTESIAN_POINT('Ctrl Pts',(50.7545767969812,247.070964671812,31.8791014184334)) ;
#81110=CARTESIAN_POINT('Ctrl Pts',(50.7545184884795,247.065351409733,31.8719088167943)) ;
#81111=CARTESIAN_POINT('Ctrl Pts',(50.7544333895888,247.05718990059,31.8586645250675)) ;
#81112=CARTESIAN_POINT('Ctrl Pts',(50.7544023657846,247.054224758889,31.8528734817062)) ;
#81113=CARTESIAN_POINT('Ctrl Pts',(50.7543498035961,247.049209302586,31.8407445801303)) ;
#81114=CARTESIAN_POINT('Ctrl Pts',(50.7543286439786,247.047195500699,31.8344482431042)) ;
#81115=CARTESIAN_POINT('Ctrl Pts',(50.754292696739,247.043739408648,31.8192922910479)) ;
#81116=CARTESIAN_POINT('Ctrl Pts',(50.7542829156931,247.042763132459,31.8103264364301)) ;
#81117=CARTESIAN_POINT('Ctrl Pts',(50.7542829156931,247.042763132459,31.8013203435596)) ;
#81118=CARTESIAN_POINT('Origin',(51.9003128398474,247.162763132459,31.8013203435596)) ;
#81119=CARTESIAN_POINT('Ctrl Pts',(50.1048968673761,247.225573558217,31.8013203435596)) ;
#81120=CARTESIAN_POINT('Ctrl Pts',(50.1817597432473,247.178096904744,31.8013203435596)) ;
#81121=CARTESIAN_POINT('Ctrl Pts',(50.2633538552322,247.124337723514,31.8013203435596)) ;
#81122=CARTESIAN_POINT('Ctrl Pts',(50.4250243638207,247.069763631682,31.8013203435596)) ;
#81123=CARTESIAN_POINT('Ctrl Pts',(50.5610592144137,247.045740326819,31.8013203435596)) ;
#81124=CARTESIAN_POINT('Ctrl Pts',(50.683716836733,247.044233834523,31.8013203435596)) ;
#81125=CARTESIAN_POINT('Ctrl Pts',(50.7542829156931,247.042763132459,31.8013203435596)) ;
#81126=CARTESIAN_POINT('Ctrl Pts',(50.1048968673761,247.225573558217,31.8102963225699)) ;
#81127=CARTESIAN_POINT('Ctrl Pts',(50.1817597432473,247.178096904744,31.8102963225699)) ;
#81128=CARTESIAN_POINT('Ctrl Pts',(50.2633538552322,247.124337723514,31.8102963225699)) ;
#81129=CARTESIAN_POINT('Ctrl Pts',(50.4250243638207,247.069763631682,31.8102963225699)) ;
#81130=CARTESIAN_POINT('Ctrl Pts',(50.5610592144137,247.045740326819,31.8102963225699)) ;
#81131=CARTESIAN_POINT('Ctrl Pts',(50.683716836733,247.044233834523,31.8102963225699)) ;
#81132=CARTESIAN_POINT('Ctrl Pts',(50.7542829156931,247.042763132459,31.8102963225699)) ;
#81133=CARTESIAN_POINT('Ctrl Pts',(50.106943740414,247.228887366936,31.8462360217477)) ;
#81134=CARTESIAN_POINT('Ctrl Pts',(50.1839062014652,247.181479943549,31.8462360217477)) ;
#81135=CARTESIAN_POINT('Ctrl Pts',(50.2652368455491,247.127832547478,31.8462360217477)) ;
#81136=CARTESIAN_POINT('Ctrl Pts',(50.4259049939851,247.073575134911,31.8462360217477)) ;
#81137=CARTESIAN_POINT('Ctrl Pts',(50.5613241282129,247.049677198827,31.8462360217477)) ;
#81138=CARTESIAN_POINT('Ctrl Pts',(50.683758957624,247.048135273327,31.8462360217477)) ;
#81139=CARTESIAN_POINT('Ctrl Pts',(50.7543640756427,247.046657285836,31.8462360217477)) ;
#81140=CARTESIAN_POINT('Ctrl Pts',(50.125546565256,247.259004624832,31.9024627370647)) ;
#81141=CARTESIAN_POINT('Ctrl Pts',(50.2024640642769,247.211565944533,31.9024627370647)) ;
#81142=CARTESIAN_POINT('Ctrl Pts',(50.2824701436015,247.159314106403,31.9024627370647)) ;
#81143=CARTESIAN_POINT('Ctrl Pts',(50.4339215284549,247.108239835495,31.9024627370647)) ;
#81144=CARTESIAN_POINT('Ctrl Pts',(50.563506491025,247.085162762637,31.9024627370647)) ;
#81145=CARTESIAN_POINT('Ctrl Pts',(50.6845141985273,247.083523653073,31.9024627370647)) ;
#81146=CARTESIAN_POINT('Ctrl Pts',(50.755101690677,247.082048954903,31.9024627370647)) ;
#81147=CARTESIAN_POINT('Ctrl Pts',(50.1538074562361,247.304757920327,31.9213203435596)) ;
#81148=CARTESIAN_POINT('Ctrl Pts',(50.2307764623335,247.257355046955,31.9213203435596)) ;
#81149=CARTESIAN_POINT('Ctrl Pts',(50.3086353659146,247.207175427604,31.9213203435596)) ;
#81150=CARTESIAN_POINT('Ctrl Pts',(50.4460983832065,247.160898427981,31.9213203435596)) ;
#81151=CARTESIAN_POINT('Ctrl Pts',(50.5668502867855,247.139108559787,31.9213203435596)) ;
#81152=CARTESIAN_POINT('Ctrl Pts',(50.6856145710118,247.137293454578,31.9213203435596)) ;
#81153=CARTESIAN_POINT('Ctrl Pts',(50.7562222547982,247.135814988266,31.9213203435596)) ;
#81154=CARTESIAN_POINT('Ctrl Pts',(50.1679584400538,247.327667818836,31.9213203435596)) ;
#81155=CARTESIAN_POINT('Ctrl Pts',(50.244821315925,247.280191165364,31.9213203435596)) ;
#81156=CARTESIAN_POINT('Ctrl Pts',(50.3217536426056,247.231101873625,31.9213203435596)) ;
#81157=CARTESIAN_POINT('Ctrl Pts',(50.4521974658606,247.187269352368,31.9213203435596)) ;
#81158=CARTESIAN_POINT('Ctrl Pts',(50.5684933320555,247.166079789663,31.9213203435596)) ;
#81159=CARTESIAN_POINT('Ctrl Pts',(50.6862172722578,247.164207780954,31.9213203435596)) ;
#81160=CARTESIAN_POINT('Ctrl Pts',(50.7567833512179,247.16273707889,31.9213203435596)) ;
#81161=CARTESIAN_POINT('',(50.1048968673761,247.225573558217,31.8013203435596)) ;
#81162=CARTESIAN_POINT('Ctrl Pts',(50.1048968673761,247.225573558217,31.8013203435596)) ;
#81163=CARTESIAN_POINT('Ctrl Pts',(50.1220003665551,247.215009070557,31.8013203435596)) ;
#81164=CARTESIAN_POINT('Ctrl Pts',(50.1393793345259,247.204269965481,31.8013203435596)) ;
#81165=CARTESIAN_POINT('Ctrl Pts',(50.1572105913275,247.193479920427,31.8013203435596)) ;
#81166=CARTESIAN_POINT('Ctrl Pts',(50.1727805461718,247.184058233771,31.8013203435596)) ;
#81167=CARTESIAN_POINT('Ctrl Pts',(50.1886952218773,247.174597296923,31.8013203435596)) ;
#81168=CARTESIAN_POINT('Ctrl Pts',(50.2050843021405,247.165218387481,31.8013203435596)) ;
#81169=CARTESIAN_POINT('Ctrl Pts',(50.2200254297862,247.156668091742,31.8013203435596)) ;
#81170=CARTESIAN_POINT('Ctrl Pts',(50.2353607337608,247.148185627256,31.8013203435596)) ;
#81171=CARTESIAN_POINT('Ctrl Pts',(50.2512006872648,247.13990263557,31.8013203435596)) ;
#81172=CARTESIAN_POINT('Ctrl Pts',(50.2661930450385,247.132062866674,31.8013203435596)) ;
#81173=CARTESIAN_POINT('Ctrl Pts',(50.2816373481069,247.124401333234,31.8013203435596)) ;
#81174=CARTESIAN_POINT('Ctrl Pts',(50.2976405331232,247.117072828458,31.8013203435596)) ;
#81175=CARTESIAN_POINT('Ctrl Pts',(50.3125234633058,247.110257333617,31.8013203435596)) ;
#81176=CARTESIAN_POINT('Ctrl Pts',(50.3278897012615,247.103729655485,31.8013203435596)) ;
#81177=CARTESIAN_POINT('Ctrl Pts',(50.3438384170975,247.097657116859,31.8013203435596)) ;
#81178=CARTESIAN_POINT('Ctrl Pts',(50.3522456466948,247.094456029888,31.8013203435596)) ;
#81179=CARTESIAN_POINT('Ctrl Pts',(50.3608149655582,247.091382169327,31.8013203435596)) ;
#81180=CARTESIAN_POINT('Ctrl Pts',(50.3695626498277,247.088465738898,31.8013203435596)) ;
#81181=CARTESIAN_POINT('Ctrl Pts',(50.3714498938344,247.087836541995,31.8013203435596)) ;
#81182=CARTESIAN_POINT('Ctrl Pts',(50.3733365725727,247.08721765027,31.8013203435596)) ;
#81183=CARTESIAN_POINT('Ctrl Pts',(50.3752217487968,247.086609092803,31.8013203435596)) ;
#81184=CARTESIAN_POINT('Ctrl Pts',(50.3949270892529,247.080247972865,31.8013203435596)) ;
#81185=CARTESIAN_POINT('Ctrl Pts',(50.41449862599,247.075000960662,31.8013203435596)) ;
#81186=CARTESIAN_POINT('Ctrl Pts',(50.4338781015769,247.07059694525,31.8013203435596)) ;
#81187=CARTESIAN_POINT('Ctrl Pts',(50.4540011902468,247.066023942629,31.8013203435596)) ;
#81188=CARTESIAN_POINT('Ctrl Pts',(50.4739172837181,247.062360157766,31.8013203435596)) ;
#81189=CARTESIAN_POINT('Ctrl Pts',(50.4935782017683,247.059357528583,31.8013203435596)) ;
#81190=CARTESIAN_POINT('Ctrl Pts',(50.5117826362868,247.056577334587,31.8013203435596)) ;
#81191=CARTESIAN_POINT('Ctrl Pts',(50.5297671997357,247.054365030188,31.8013203435596)) ;
#81192=CARTESIAN_POINT('Ctrl Pts',(50.5475093978148,247.052559566174,31.8013203435596)) ;
#81193=CARTESIAN_POINT('Ctrl Pts',(50.5684869881217,247.050424865377,31.8013203435596)) ;
#81194=CARTESIAN_POINT('Ctrl Pts',(50.5891312305048,247.048857239894,31.8013203435596)) ;
#81195=CARTESIAN_POINT('Ctrl Pts',(50.6094626803275,247.047643171334,31.8013203435596)) ;
#81196=CARTESIAN_POINT('Ctrl Pts',(50.6312322488022,247.046343227213,31.8013203435596)) ;
#81197=CARTESIAN_POINT('Ctrl Pts',(50.6526434341527,247.045449355937,31.8013203435596)) ;
#81198=CARTESIAN_POINT('Ctrl Pts',(50.673739904065,247.044759445824,31.8013203435596)) ;
#81199=CARTESIAN_POINT('Ctrl Pts',(50.6977184863756,247.043975283047,31.8013203435596)) ;
#81200=CARTESIAN_POINT('Ctrl Pts',(50.7212907023591,247.043455310561,31.8013203435596)) ;
#81201=CARTESIAN_POINT('Ctrl Pts',(50.7445403358891,247.042966742562,31.8013203435596)) ;
#81202=CARTESIAN_POINT('Ctrl Pts',(50.7477940726226,247.042898368511,31.8013203435596)) ;
#81203=CARTESIAN_POINT('Ctrl Pts',(50.7510415155772,247.04283068806,31.8013203435596)) ;
#81204=CARTESIAN_POINT('Ctrl Pts',(50.7542829156931,247.042763132459,31.8013203435596)) ;
#81205=CARTESIAN_POINT('',(50.1819316941158,247.319027603173,31.9213203435596)) ;
#81206=CARTESIAN_POINT('Ctrl Pts',(50.7555332761922,247.16276309732,31.9213203435596)) ;
#81207=CARTESIAN_POINT('Ctrl Pts',(50.6853831050741,247.164221288387,31.9213203435596)) ;
#81208=CARTESIAN_POINT('Ctrl Pts',(50.568081299126,247.166154863678,31.9213203435596)) ;
#81209=CARTESIAN_POINT('Ctrl Pts',(50.4521974658606,247.187269352368,31.9213203435596)) ;
#81210=CARTESIAN_POINT('Ctrl Pts',(50.3269498697332,247.229355806006,31.9213203435596)) ;
#81211=CARTESIAN_POINT('Ctrl Pts',(50.2541752681168,247.274317645589,31.9213203435596)) ;
#81212=CARTESIAN_POINT('Ctrl Pts',(50.1819308000888,247.319026158513,31.9213203435596)) ;
#81213=CARTESIAN_POINT('Ctrl Pts',(50.1819388265444,247.319021191339,31.9213203435596)) ;
#81214=CARTESIAN_POINT('Ctrl Pts',(50.1817524473267,247.318793998429,31.9213203435596)) ;
#81215=CARTESIAN_POINT('Ctrl Pts',(50.1815660887041,247.318566789193,31.9213192390868)) ;
#81216=CARTESIAN_POINT('Ctrl Pts',(50.1714406029608,247.306219582572,31.9211993432478)) ;
#81217=CARTESIAN_POINT('Ctrl Pts',(50.1615757516659,247.294081074233,31.917946664297)) ;
#81218=CARTESIAN_POINT('Ctrl Pts',(50.1459828532116,247.275031259232,31.9077738491051)) ;
#81219=CARTESIAN_POINT('Ctrl Pts',(50.1367511418837,247.263820791132,31.900294136492)) ;
#81220=CARTESIAN_POINT('Ctrl Pts',(50.1209443533371,247.245047664794,31.8760190448593)) ;
#81221=CARTESIAN_POINT('Ctrl Pts',(50.1150198743948,247.238012576204,31.8631426108606)) ;
#81222=CARTESIAN_POINT('Ctrl Pts',(50.1091216557418,247.230422468868,31.8407001619781)) ;
#81223=CARTESIAN_POINT('Ctrl Pts',(50.1076630070811,247.228494965487,31.8330344212244)) ;
#81224=CARTESIAN_POINT('Ctrl Pts',(50.1055315058664,247.226090096372,31.8173189025619)) ;
#81225=CARTESIAN_POINT('Ctrl Pts',(50.1048968673764,247.225573558217,31.8093263718846)) ;
#81226=CARTESIAN_POINT('Ctrl Pts',(50.1048968673764,247.225573558217,31.8013203435596)) ;
#81227=CARTESIAN_POINT('Origin',(51.9003128398474,243.213135158824,31.8013203435596)) ;
#81228=CARTESIAN_POINT('',(51.9003128398474,243.213135158824,31.9213203435596)) ;
#81229=CARTESIAN_POINT('Ctrl Pts',(49.8975299240168,247.692149180776,31.8013203435596)) ;
#81230=CARTESIAN_POINT('Ctrl Pts',(49.9003120409242,247.662214992781,31.8013203435596)) ;
#81231=CARTESIAN_POINT('Ctrl Pts',(49.9080129919011,247.584369229331,31.8013203435596)) ;
#81232=CARTESIAN_POINT('Ctrl Pts',(49.9228022199243,247.494193108499,31.8013203435597)) ;
#81233=CARTESIAN_POINT('Ctrl Pts',(49.9584226751439,247.413847381454,31.8013203435597)) ;
#81234=CARTESIAN_POINT('Ctrl Pts',(49.978378600925,247.378172811915,31.8013203435596)) ;
#81235=CARTESIAN_POINT('Ctrl Pts',(50.0317423407727,247.303870476782,31.8013203435596)) ;
#81236=CARTESIAN_POINT('Ctrl Pts',(50.0747869844785,247.258178865285,31.8013203435596)) ;
#81237=CARTESIAN_POINT('Ctrl Pts',(50.1049315040526,247.225536051252,31.8013203435596)) ;
#81238=CARTESIAN_POINT('Ctrl Pts',(49.8975299240168,247.692149180776,31.8192723015802)) ;
#81239=CARTESIAN_POINT('Ctrl Pts',(49.9003120409242,247.662214992781,31.8192723015802)) ;
#81240=CARTESIAN_POINT('Ctrl Pts',(49.9080129919011,247.584369229331,31.8192723015802)) ;
#81241=CARTESIAN_POINT('Ctrl Pts',(49.9228022199243,247.494193108499,31.8192723015802)) ;
#81242=CARTESIAN_POINT('Ctrl Pts',(49.9584226751439,247.413847381454,31.8192723015802)) ;
#81243=CARTESIAN_POINT('Ctrl Pts',(49.978378600925,247.378172811915,31.8192723015802)) ;
#81244=CARTESIAN_POINT('Ctrl Pts',(50.0317423407727,247.303870476782,31.8192723015802)) ;
#81245=CARTESIAN_POINT('Ctrl Pts',(50.0747869844785,247.258178865285,31.8192723015802)) ;
#81246=CARTESIAN_POINT('Ctrl Pts',(50.1049315040526,247.225536051252,31.8192723015802)) ;
#81247=CARTESIAN_POINT('Ctrl Pts',(49.9057100722929,247.692909452904,31.8551057858421)) ;
#81248=CARTESIAN_POINT('Ctrl Pts',(49.9084394091396,247.662972763406,31.8551057858421)) ;
#81249=CARTESIAN_POINT('Ctrl Pts',(49.9161458757847,247.585340197531,31.8551057858422)) ;
#81250=CARTESIAN_POINT('Ctrl Pts',(49.9309041124678,247.496274424605,31.8551057858422)) ;
#81251=CARTESIAN_POINT('Ctrl Pts',(49.9656396859993,247.417640984724,31.8551057858422)) ;
#81252=CARTESIAN_POINT('Ctrl Pts',(49.9852635362106,247.38264873378,31.8551057858422)) ;
#81253=CARTESIAN_POINT('Ctrl Pts',(50.0379009729177,247.309294040215,31.8551057858421)) ;
#81254=CARTESIAN_POINT('Ctrl Pts',(50.0808262047872,247.263810918776,31.8551057858421)) ;
#81255=CARTESIAN_POINT('Ctrl Pts',(50.1109669912768,247.231109643768,31.8551057858421)) ;
#81256=CARTESIAN_POINT('Ctrl Pts',(49.9456840251116,247.696624676782,31.9055714461187)) ;
#81257=CARTESIAN_POINT('Ctrl Pts',(49.9484658983372,247.666690477238,31.9055714461187)) ;
#81258=CARTESIAN_POINT('Ctrl Pts',(49.9558946167219,247.590135261357,31.9055714461187)) ;
#81259=CARTESIAN_POINT('Ctrl Pts',(49.9702456835514,247.506232253633,31.9055714461187)) ;
#81260=CARTESIAN_POINT('Ctrl Pts',(50.0013503310202,247.43618856547,31.9055714461187)) ;
#81261=CARTESIAN_POINT('Ctrl Pts',(50.0190652052593,247.404431264816,31.9055714461187)) ;
#81262=CARTESIAN_POINT('Ctrl Pts',(50.0682830773054,247.335769984711,31.9055714461187)) ;
#81263=CARTESIAN_POINT('Ctrl Pts',(50.1103155648094,247.290990135563,31.9055714461187)) ;
#81264=CARTESIAN_POINT('Ctrl Pts',(50.1404606488897,247.258346527721,31.9055714461187)) ;
#81265=CARTESIAN_POINT('Ctrl Pts',(49.9902025919921,247.700762282173,31.9213203435596)) ;
#81266=CARTESIAN_POINT('Ctrl Pts',(49.9929442461564,247.670826176452,31.9213203435596)) ;
#81267=CARTESIAN_POINT('Ctrl Pts',(50.0001605373263,247.595459499129,31.9213203435596)) ;
#81268=CARTESIAN_POINT('Ctrl Pts',(50.0141394662325,247.517389900366,31.9213203435597)) ;
#81269=CARTESIAN_POINT('Ctrl Pts',(50.0409799368062,247.456841829704,31.9213203435597)) ;
#81270=CARTESIAN_POINT('Ctrl Pts',(50.0566598259294,247.428718849235,31.9213203435597)) ;
#81271=CARTESIAN_POINT('Ctrl Pts',(50.1020281310731,247.365264675744,31.9213203435596)) ;
#81272=CARTESIAN_POINT('Ctrl Pts',(50.143164711757,247.321368403535,31.9213203435596)) ;
#81273=CARTESIAN_POINT('Ctrl Pts',(50.1733074140605,247.288679830851,31.9213203435596)) ;
#81274=CARTESIAN_POINT('Ctrl Pts',(50.0170149746567,247.703254255002,31.9213203435596)) ;
#81275=CARTESIAN_POINT('Ctrl Pts',(50.0197970915642,247.673320067007,31.9213203435596)) ;
#81276=CARTESIAN_POINT('Ctrl Pts',(50.0268219567888,247.598676615906,31.9213203435596)) ;
#81277=CARTESIAN_POINT('Ctrl Pts',(50.0405234748466,247.52406549449,31.9213203435597)) ;
#81278=CARTESIAN_POINT('Ctrl Pts',(50.0649401802121,247.46928270932,31.9213203435597)) ;
#81279=CARTESIAN_POINT('Ctrl Pts',(50.0793348143422,247.443327888337,31.9213203435597)) ;
#81280=CARTESIAN_POINT('Ctrl Pts',(50.1224116408749,247.383022857659,31.9213203435596)) ;
#81281=CARTESIAN_POINT('Ctrl Pts',(50.1629442132913,247.339592992793,31.9213203435596)) ;
#81282=CARTESIAN_POINT('Ctrl Pts',(50.1930901774771,247.306948877788,31.9213203435596)) ;
#81283=CARTESIAN_POINT('',(49.8975299240168,247.692149180776,31.8013203435596)) ;
#81284=CARTESIAN_POINT('Ctrl Pts',(49.8975299240168,247.692149180776,31.8013203435596)) ;
#81285=CARTESIAN_POINT('Ctrl Pts',(49.8989209824705,247.677182086779,31.8013203435596)) ;
#81286=CARTESIAN_POINT('Ctrl Pts',(49.9003364541846,247.661913083176,31.8013203435596)) ;
#81287=CARTESIAN_POINT('Ctrl Pts',(49.9019331250822,247.646242176031,31.8013203435596)) ;
#81288=CARTESIAN_POINT('Ctrl Pts',(49.9033173765781,247.63265610974,31.8013203435596)) ;
#81289=CARTESIAN_POINT('Ctrl Pts',(49.9048372301939,247.618767700215,31.8013203435596)) ;
#81290=CARTESIAN_POINT('Ctrl Pts',(49.9066326956466,247.604528684876,31.8013203435596)) ;
#81291=CARTESIAN_POINT('Ctrl Pts',(49.9069082176151,247.602343646155,31.8013203435596)) ;
#81292=CARTESIAN_POINT('Ctrl Pts',(49.9071903212962,247.600150392157,31.8013203435596)) ;
#81293=CARTESIAN_POINT('Ctrl Pts',(49.907479619698,247.597948796284,31.8013203435596)) ;
#81294=CARTESIAN_POINT('Ctrl Pts',(49.9091103249136,247.585538932107,31.8013203435596)) ;
#81295=CARTESIAN_POINT('Ctrl Pts',(49.9109621984763,247.572888414998,31.8013203435596)) ;
#81296=CARTESIAN_POINT('Ctrl Pts',(49.9131777267516,247.559918931878,31.8013203435596)) ;
#81297=CARTESIAN_POINT('Ctrl Pts',(49.915073415318,247.548821758741,31.8013203435597)) ;
#81298=CARTESIAN_POINT('Ctrl Pts',(49.9172352909559,247.537491043414,31.8013203435597)) ;
#81299=CARTESIAN_POINT('Ctrl Pts',(49.9197895184584,247.525894206826,31.8013203435597)) ;
#81300=CARTESIAN_POINT('Ctrl Pts',(49.922187758184,247.515005594058,31.8013203435597)) ;
#81301=CARTESIAN_POINT('Ctrl Pts',(49.9249314068481,247.503882155673,31.8013203435597)) ;
#81302=CARTESIAN_POINT('Ctrl Pts',(49.928164462093,247.492514588819,31.8013203435597)) ;
#81303=CARTESIAN_POINT('Ctrl Pts',(49.9311207392,247.482120186279,31.8013203435597)) ;
#81304=CARTESIAN_POINT('Ctrl Pts',(49.9344860238457,247.471521580022,31.8013203435597)) ;
#81305=CARTESIAN_POINT('Ctrl Pts',(49.9384087813414,247.460728790724,31.8013203435597)) ;
#81306=CARTESIAN_POINT('Ctrl Pts',(49.9416467803634,247.451819996023,31.8013203435597)) ;
#81307=CARTESIAN_POINT('Ctrl Pts',(49.9452650324319,247.442779081571,31.8013203435597)) ;
#81308=CARTESIAN_POINT('Ctrl Pts',(49.9493716598566,247.433622676736,31.8013203435597)) ;
#81309=CARTESIAN_POINT('Ctrl Pts',(49.9493749701299,247.433615295934,31.8013203435597)) ;
#81310=CARTESIAN_POINT('Ctrl Pts',(49.949378280722,247.433607915058,31.8013203435597)) ;
#81311=CARTESIAN_POINT('Ctrl Pts',(49.9493815916327,247.433600534107,31.8013203435597)) ;
#81312=CARTESIAN_POINT('Ctrl Pts',(49.9545038625223,247.422181552888,31.8013203435597)) ;
#81313=CARTESIAN_POINT('Ctrl Pts',(49.9600029742428,247.41143325106,31.8013203435597)) ;
#81314=CARTESIAN_POINT('Ctrl Pts',(49.9657098706998,247.401244562447,31.8013203435597)) ;
#81315=CARTESIAN_POINT('Ctrl Pts',(49.9699155343581,247.393736068514,31.8013203435597)) ;
#81316=CARTESIAN_POINT('Ctrl Pts',(49.974235278962,247.386532044786,31.8013203435596)) ;
#81317=CARTESIAN_POINT('Ctrl Pts',(49.9786177646995,247.379595326503,31.8013203435596)) ;
#81318=CARTESIAN_POINT('Ctrl Pts',(49.9849176615277,247.369623677506,31.8013203435596)) ;
#81319=CARTESIAN_POINT('Ctrl Pts',(49.9913445526255,247.360203543544,31.8013203435596)) ;
#81320=CARTESIAN_POINT('Ctrl Pts',(49.9978236741791,247.351195483027,31.8013203435596)) ;
#81321=CARTESIAN_POINT('Ctrl Pts',(50.0019677316018,247.345433911841,31.8013203435596)) ;
#81322=CARTESIAN_POINT('Ctrl Pts',(50.0061343453035,247.339841446927,31.8013203435596)) ;
#81323=CARTESIAN_POINT('Ctrl Pts',(50.0103138715769,247.334386031064,31.8013203435596)) ;
#81324=CARTESIAN_POINT('Ctrl Pts',(50.0187016326063,247.323437726979,31.8013203435596)) ;
#81325=CARTESIAN_POINT('Ctrl Pts',(50.0271429541399,247.313034619382,31.8013203435596)) ;
#81326=CARTESIAN_POINT('Ctrl Pts',(50.0355400198878,247.303042575351,31.8013203435596)) ;
#81327=CARTESIAN_POINT('Ctrl Pts',(50.0446115661329,247.292247936816,31.8013203435596)) ;
#81328=CARTESIAN_POINT('Ctrl Pts',(50.0536322844746,247.2819334174,31.8013203435596)) ;
#81329=CARTESIAN_POINT('Ctrl Pts',(50.0625395637957,247.271957006048,31.8013203435596)) ;
#81330=CARTESIAN_POINT('Ctrl Pts',(50.0729202410483,247.260330346252,31.8013203435596)) ;
#81331=CARTESIAN_POINT('Ctrl Pts',(50.0831475154001,247.249163200923,31.8013203435596)) ;
#81332=CARTESIAN_POINT('Ctrl Pts',(50.0931900641649,247.238261049293,31.8013203435596)) ;
#81333=CARTESIAN_POINT('Ctrl Pts',(50.0971200610123,247.233994660098,31.8013203435596)) ;
#81334=CARTESIAN_POINT('Ctrl Pts',(50.1010223530526,247.229769113771,31.8013203435596)) ;
#81335=CARTESIAN_POINT('Ctrl Pts',(50.1048968673761,247.225573558217,31.8013203435596)) ;
#81336=CARTESIAN_POINT('',(50.0179285595009,247.693448991958,31.9213203435596)) ;
#81337=CARTESIAN_POINT('Ctrl Pts',(50.1819259253794,247.319035169015,31.9213203435597)) ;
#81338=CARTESIAN_POINT('Ctrl Pts',(50.1554933071014,247.347673462912,31.9213203435596)) ;
#81339=CARTESIAN_POINT('Ctrl Pts',(50.1192219147918,247.387488287097,31.9213203435596)) ;
#81340=CARTESIAN_POINT('Ctrl Pts',(50.0793348143422,247.443327888337,31.9213203435597)) ;
#81341=CARTESIAN_POINT('Ctrl Pts',(50.0649401802121,247.46928270932,31.9213203435597)) ;
#81342=CARTESIAN_POINT('Ctrl Pts',(50.0405234748466,247.52406549449,31.9213203435597)) ;
#81343=CARTESIAN_POINT('Ctrl Pts',(50.0274205901366,247.595416779644,31.9213203435596)) ;
#81344=CARTESIAN_POINT('Ctrl Pts',(50.0204236837674,247.666797631165,31.9213203435596)) ;
#81345=CARTESIAN_POINT('Ctrl Pts',(50.0179289780831,247.693447995904,31.9213203435596)) ;
#81346=CARTESIAN_POINT('Ctrl Pts',(50.017928391634,247.693450066558,31.9213203435596)) ;
#81347=CARTESIAN_POINT('Ctrl Pts',(50.0176360614229,247.693446884448,31.9213203435596)) ;
#81348=CARTESIAN_POINT('Ctrl Pts',(50.0173433514854,247.693443731786,31.921319241072)) ;
#81349=CARTESIAN_POINT('Ctrl Pts',(50.0170506622064,247.693440580217,31.921317036068)) ;
#81350=CARTESIAN_POINT('Ctrl Pts',(50.0086222481347,247.693349826201,31.9212535397677)) ;
#81351=CARTESIAN_POINT('Ctrl Pts',(50.0002543434629,247.693260420416,31.9202814000225)) ;
#81352=CARTESIAN_POINT('Ctrl Pts',(49.9920673812869,247.69317293051,31.9184713729232)) ;
#81353=CARTESIAN_POINT('Ctrl Pts',(49.9913984237448,247.693165781701,31.9183234754181)) ;
#81354=CARTESIAN_POINT('Ctrl Pts',(49.9907306748512,247.693158645656,31.9181699552184)) ;
#81355=CARTESIAN_POINT('Ctrl Pts',(49.9900642015852,247.693151522596,31.9180108360501)) ;
#81356=CARTESIAN_POINT('Ctrl Pts',(49.9833973538999,247.693080269391,31.9164191394086)) ;
#81357=CARTESIAN_POINT('Ctrl Pts',(49.976857424647,247.69301028865,31.9142687128406)) ;
#81358=CARTESIAN_POINT('Ctrl Pts',(49.9705183372566,247.69294212283,31.9115735225365)) ;
#81359=CARTESIAN_POINT('Ctrl Pts',(49.9621346627971,247.692851971047,31.908009034981)) ;
#81360=CARTESIAN_POINT('Ctrl Pts',(49.9541926461795,247.692765943363,31.9035316654796)) ;
#81361=CARTESIAN_POINT('Ctrl Pts',(49.9468699753835,247.69268559923,31.8981932593553)) ;
#81362=CARTESIAN_POINT('Ctrl Pts',(49.9455102810432,247.692670680703,31.8972020089228)) ;
#81363=CARTESIAN_POINT('Ctrl Pts',(49.9441720544978,247.69265596149,31.8961809675201)) ;
#81364=CARTESIAN_POINT('Ctrl Pts',(49.9428566063046,247.692641457862,31.8951303448721)) ;
#81365=CARTESIAN_POINT('Ctrl Pts',(49.942850731994,247.692641393094,31.8951256531756)) ;
#81366=CARTESIAN_POINT('Ctrl Pts',(49.9428448581382,247.69264132833,31.8951209608895)) ;
#81367=CARTESIAN_POINT('Ctrl Pts',(49.9428389847374,247.69264126357,31.8951162680138)) ;
#81368=CARTESIAN_POINT('Ctrl Pts',(49.9390653822337,247.69259965616,31.8921011413717)) ;
#81369=CARTESIAN_POINT('Ctrl Pts',(49.9354794429431,247.692559773032,31.8888427091753)) ;
#81370=CARTESIAN_POINT('Ctrl Pts',(49.932097179084,247.692521650875,31.8853668065556)) ;
#81371=CARTESIAN_POINT('Ctrl Pts',(49.9257440837398,247.692450043897,31.8788378242911)) ;
#81372=CARTESIAN_POINT('Ctrl Pts',(49.9201787710645,247.692385036831,31.871618011282)) ;
#81373=CARTESIAN_POINT('Ctrl Pts',(49.9154588127174,247.692330638236,31.8638856152259)) ;
#81374=CARTESIAN_POINT('Ctrl Pts',(49.913357124184,247.692306415797,31.8604425576961)) ;
#81375=CARTESIAN_POINT('Ctrl Pts',(49.9114231698096,247.692284370314,31.8568969998879)) ;
#81376=CARTESIAN_POINT('Ctrl Pts',(49.9096637197127,247.692265205622,31.8532606519075)) ;
#81377=CARTESIAN_POINT('Ctrl Pts',(49.9086093688806,247.692253721176,31.8510815696331)) ;
#81378=CARTESIAN_POINT('Ctrl Pts',(49.9076176957775,247.692243276832,31.8488698077343)) ;
#81379=CARTESIAN_POINT('Ctrl Pts',(49.9066904861145,247.692233782334,31.8466274426062)) ;
#81380=CARTESIAN_POINT('Ctrl Pts',(49.9032292440959,247.692198339699,31.8382567701338)) ;
#81381=CARTESIAN_POINT('Ctrl Pts',(49.9006995749997,247.692176191016,31.8295510379215)) ;
#81382=CARTESIAN_POINT('Ctrl Pts',(49.899182009376,247.692163157307,31.8206540876558)) ;
#81383=CARTESIAN_POINT('Ctrl Pts',(49.8980956948875,247.692153827426,31.8142854101992)) ;
#81384=CARTESIAN_POINT('Ctrl Pts',(49.8975299240168,247.692149180776,31.807818822737)) ;
#81385=CARTESIAN_POINT('Ctrl Pts',(49.8975299240168,247.692149180776,31.8013203435596)) ;
#81386=CARTESIAN_POINT('Ctrl Pts',(50.0039417983111,248.05231292904,31.8013203435596)) ;
#81387=CARTESIAN_POINT('Ctrl Pts',(49.9880262923894,248.023366957204,31.8013203435596)) ;
#81388=CARTESIAN_POINT('Ctrl Pts',(49.9595768641916,247.972394634097,31.8013203435596)) ;
#81389=CARTESIAN_POINT('Ctrl Pts',(49.9328199880692,247.908444334476,31.8013203435596)) ;
#81390=CARTESIAN_POINT('Ctrl Pts',(49.9115183942193,247.835438884033,31.8013203435596)) ;
#81391=CARTESIAN_POINT('Ctrl Pts',(49.9032281681206,247.770513850496,31.8013203435596)) ;
#81392=CARTESIAN_POINT('Ctrl Pts',(49.8990770736132,247.713887501579,31.8013203435596)) ;
#81393=CARTESIAN_POINT('Ctrl Pts',(49.8975299240168,247.692149180776,31.8013203435596)) ;
#81394=CARTESIAN_POINT('Ctrl Pts',(50.0039417983111,248.05231292904,31.8372242596006)) ;
#81395=CARTESIAN_POINT('Ctrl Pts',(49.9880262923894,248.023366957204,31.8372242596007)) ;
#81396=CARTESIAN_POINT('Ctrl Pts',(49.9595768641916,247.972394634097,31.8372242596006)) ;
#81397=CARTESIAN_POINT('Ctrl Pts',(49.9328199880692,247.908444334476,31.8372242596006)) ;
#81398=CARTESIAN_POINT('Ctrl Pts',(49.9115183942193,247.835438884033,31.8372242596007)) ;
#81399=CARTESIAN_POINT('Ctrl Pts',(49.9032281681206,247.770513850496,31.8372242596007)) ;
#81400=CARTESIAN_POINT('Ctrl Pts',(49.8990770736132,247.713887501579,31.8372242596007)) ;
#81401=CARTESIAN_POINT('Ctrl Pts',(49.8975299240168,247.692149180776,31.8372242596007)) ;
#81402=CARTESIAN_POINT('Ctrl Pts',(50.0303692554824,248.037782190411,31.8993563874716)) ;
#81403=CARTESIAN_POINT('Ctrl Pts',(50.0144401833049,248.008801749279,31.8993563874716)) ;
#81404=CARTESIAN_POINT('Ctrl Pts',(49.9864587570184,247.958566948592,31.8993563874716)) ;
#81405=CARTESIAN_POINT('Ctrl Pts',(49.9611065521,247.897853880215,31.8993563874716)) ;
#81406=CARTESIAN_POINT('Ctrl Pts',(49.9413091559894,247.829989135405,31.8993563874716)) ;
#81407=CARTESIAN_POINT('Ctrl Pts',(49.9332582787006,247.767775968166,31.8993563874716)) ;
#81408=CARTESIAN_POINT('Ctrl Pts',(49.9291299338273,247.711745405093,31.8993563874716)) ;
#81409=CARTESIAN_POINT('Ctrl Pts',(49.9276126240328,247.690008148926,31.8993563874716)) ;
#81410=CARTESIAN_POINT('Ctrl Pts',(50.0854987052327,248.007470094175,31.9213203435596)) ;
#81411=CARTESIAN_POINT('Ctrl Pts',(50.0695751953828,247.978503785867,31.9213203435596)) ;
#81412=CARTESIAN_POINT('Ctrl Pts',(50.0425087956085,247.929736002886,31.9213203435596)) ;
#81413=CARTESIAN_POINT('Ctrl Pts',(50.0201811280109,247.875790500525,31.9213203435596)) ;
#81414=CARTESIAN_POINT('Ctrl Pts',(50.0034820155373,247.818649943681,31.9213203435596)) ;
#81415=CARTESIAN_POINT('Ctrl Pts',(49.9958616134348,247.762060700417,31.9213203435596)) ;
#81416=CARTESIAN_POINT('Ctrl Pts',(49.9918967002071,247.70727950544,31.9213203435596)) ;
#81417=CARTESIAN_POINT('Ctrl Pts',(49.9903671557358,247.68554181276,31.9213203435596)) ;
#81418=CARTESIAN_POINT('Ctrl Pts',(50.1090950367627,247.994496007268,31.9213203435596)) ;
#81419=CARTESIAN_POINT('Ctrl Pts',(50.0931795308409,247.965550035432,31.9213203435596)) ;
#81420=CARTESIAN_POINT('Ctrl Pts',(50.0664946055529,247.917398286899,31.9213203435596)) ;
#81421=CARTESIAN_POINT('Ctrl Pts',(50.0454771499519,247.866351821843,31.9213203435596)) ;
#81422=CARTESIAN_POINT('Ctrl Pts',(50.0300975833916,247.813801452734,31.9213203435596)) ;
#81423=CARTESIAN_POINT('Ctrl Pts',(50.0226500033239,247.759613828492,31.9213203435596)) ;
#81424=CARTESIAN_POINT('Ctrl Pts',(50.0187743001587,247.705368466579,31.9213203435596)) ;
#81425=CARTESIAN_POINT('Ctrl Pts',(50.0172271505622,247.683630145776,31.9213203435596)) ;
#81426=CARTESIAN_POINT('Ctrl Pts',(50.003941798311,248.05231292904,31.8013203435596)) ;
#81427=CARTESIAN_POINT('Ctrl Pts',(49.9973092280089,248.040250089561,31.8013203435596)) ;
#81428=CARTESIAN_POINT('Ctrl Pts',(49.9905098033151,248.027893411311,31.8013203435596)) ;
#81429=CARTESIAN_POINT('Ctrl Pts',(49.9836122391022,248.01504026841,31.8013203435596)) ;
#81430=CARTESIAN_POINT('Ctrl Pts',(49.9781582134433,248.004877061657,31.8013203435596)) ;
#81431=CARTESIAN_POINT('Ctrl Pts',(49.9726428617977,247.994403438057,31.8013203435596)) ;
#81432=CARTESIAN_POINT('Ctrl Pts',(49.9671358038039,247.983508719679,31.8013203435596)) ;
#81433=CARTESIAN_POINT('Ctrl Pts',(49.962297053248,247.973936126715,31.8013203435596)) ;
#81434=CARTESIAN_POINT('Ctrl Pts',(49.9574646433129,247.964038710708,31.8013203435596)) ;
#81435=CARTESIAN_POINT('Ctrl Pts',(49.9527177389226,247.953731217489,31.8013203435596)) ;
#81436=CARTESIAN_POINT('Ctrl Pts',(49.9482194239541,247.943963514746,31.8013203435596)) ;
#81437=CARTESIAN_POINT('Ctrl Pts',(49.9437957899078,247.93382561916,31.8013203435596)) ;
#81438=CARTESIAN_POINT('Ctrl Pts',(49.9395411846259,247.923206079714,31.8013203435596)) ;
#81439=CARTESIAN_POINT('Ctrl Pts',(49.9367748644537,247.916301315525,31.8013203435596)) ;
#81440=CARTESIAN_POINT('Ctrl Pts',(49.9340808270642,247.909192691924,31.8013203435596)) ;
#81441=CARTESIAN_POINT('Ctrl Pts',(49.9314977623415,247.901845815823,31.8013203435596)) ;
#81442=CARTESIAN_POINT('Ctrl Pts',(49.9302062299801,247.898172377772,31.8013203435596)) ;
#81443=CARTESIAN_POINT('Ctrl Pts',(49.9289426182913,247.894439324299,31.8013203435596)) ;
#81444=CARTESIAN_POINT('Ctrl Pts',(49.9277129474339,247.890642007448,31.8013203435596)) ;
#81445=CARTESIAN_POINT('Ctrl Pts',(49.9270587936476,247.888621930952,31.8013203435596)) ;
#81446=CARTESIAN_POINT('Ctrl Pts',(49.9264142593432,247.886583663888,31.8013203435596)) ;
#81447=CARTESIAN_POINT('Ctrl Pts',(49.9257803542142,247.884526476061,31.8013203435596)) ;
#81448=CARTESIAN_POINT('Ctrl Pts',(49.9253459058396,247.883116577534,31.8013203435596)) ;
#81449=CARTESIAN_POINT('Ctrl Pts',(49.9249164515835,247.88169779133,31.8013203435596)) ;
#81450=CARTESIAN_POINT('Ctrl Pts',(49.9244923373195,247.88026987625,31.8013203435596)) ;
#81451=CARTESIAN_POINT('Ctrl Pts',(49.9243720149763,247.879864772949,31.8013203435596)) ;
#81452=CARTESIAN_POINT('Ctrl Pts',(49.9242521035458,247.879458870193,31.8013203435596)) ;
#81453=CARTESIAN_POINT('Ctrl Pts',(49.9241326690729,247.879052359467,31.8013203435596)) ;
#81454=CARTESIAN_POINT('Ctrl Pts',(49.9208603305429,247.867914530669,31.8013203435596)) ;
#81455=CARTESIAN_POINT('Ctrl Pts',(49.9181591310371,247.857063543614,31.8013203435596)) ;
#81456=CARTESIAN_POINT('Ctrl Pts',(49.915855507275,247.846490923394,31.8013203435596)) ;
#81457=CARTESIAN_POINT('Ctrl Pts',(49.9133864593928,247.835159079196,31.8013203435596)) ;
#81458=CARTESIAN_POINT('Ctrl Pts',(49.9113747091496,247.824146848157,31.8013203435596)) ;
#81459=CARTESIAN_POINT('Ctrl Pts',(49.9096664176065,247.813426157519,31.8013203435596)) ;
#81460=CARTESIAN_POINT('Ctrl Pts',(49.9077483672311,247.801389087625,31.8013203435596)) ;
#81461=CARTESIAN_POINT('Ctrl Pts',(49.9062132415599,247.789719440941,31.8013203435596)) ;
#81462=CARTESIAN_POINT('Ctrl Pts',(49.9049089271676,247.778358143172,31.8013203435596)) ;
#81463=CARTESIAN_POINT('Ctrl Pts',(49.9038781189045,247.769379234645,31.8013203435596)) ;
#81464=CARTESIAN_POINT('Ctrl Pts',(49.9029927564946,247.760589341875,31.8013203435596)) ;
#81465=CARTESIAN_POINT('Ctrl Pts',(49.9021997298857,247.751964778757,31.8013203435596)) ;
#81466=CARTESIAN_POINT('Ctrl Pts',(49.9009319351644,247.738176873697,31.8013203435596)) ;
#81467=CARTESIAN_POINT('Ctrl Pts',(49.8998987096635,247.724820112012,31.8013203435596)) ;
#81468=CARTESIAN_POINT('Ctrl Pts',(49.8989443625904,247.71181780161,31.8013203435596)) ;
#81469=CARTESIAN_POINT('Ctrl Pts',(49.8984566596798,247.705173191062,31.8013203435596)) ;
#81470=CARTESIAN_POINT('Ctrl Pts',(49.8979905234979,247.698620862186,31.8013203435596)) ;
#81471=CARTESIAN_POINT('Ctrl Pts',(49.8975299240168,247.692149180776,31.8013203435596)) ;
#81472=CARTESIAN_POINT('Ctrl Pts',(50.0179283156872,247.693449009475,31.9213203435596)) ;
#81473=CARTESIAN_POINT('Ctrl Pts',(50.0192542126488,247.711903817022,31.9213203435596)) ;
#81474=CARTESIAN_POINT('Ctrl Pts',(50.0230986509543,247.762878130318,31.9213203435596)) ;
#81475=CARTESIAN_POINT('Ctrl Pts',(50.0300975833916,247.813801452734,31.9213203435596)) ;
#81476=CARTESIAN_POINT('Ctrl Pts',(50.0454771499519,247.866351821843,31.9213203435596)) ;
#81477=CARTESIAN_POINT('Ctrl Pts',(50.0652213925075,247.914305951343,31.9213203435596)) ;
#81478=CARTESIAN_POINT('Ctrl Pts',(50.0899672457456,247.959705458432,31.9213203435596)) ;
#81479=CARTESIAN_POINT('Ctrl Pts',(50.1042736016154,247.985728991073,31.9213203435596)) ;
#81480=CARTESIAN_POINT('Ctrl Pts',(50.8825961108042,248.366092821008,31.8013203435596)) ;
#81481=CARTESIAN_POINT('Ctrl Pts',(50.7801147995828,248.365003869109,31.8013203435596)) ;
#81482=CARTESIAN_POINT('Ctrl Pts',(50.6724206638963,248.36479492292,31.8013203435596)) ;
#81483=CARTESIAN_POINT('Ctrl Pts',(50.471719498392,248.334437936584,31.8013203435596)) ;
#81484=CARTESIAN_POINT('Ctrl Pts',(50.3915513141507,248.312651528491,31.8013203435596)) ;
#81485=CARTESIAN_POINT('Ctrl Pts',(50.31499221335,248.292422193891,31.8013203435596)) ;
#81486=CARTESIAN_POINT('Ctrl Pts',(50.8825961108042,248.366092821008,31.8372242596007)) ;
#81487=CARTESIAN_POINT('Ctrl Pts',(50.7801147995828,248.365003869109,31.8372242596007)) ;
#81488=CARTESIAN_POINT('Ctrl Pts',(50.6724206638963,248.36479492292,31.8372242596007)) ;
#81489=CARTESIAN_POINT('Ctrl Pts',(50.471719498392,248.334437936584,31.8372242596007)) ;
#81490=CARTESIAN_POINT('Ctrl Pts',(50.3915513141507,248.312651528491,31.8372242596007)) ;
#81491=CARTESIAN_POINT('Ctrl Pts',(50.31499221335,248.292422193891,31.8372242596007)) ;
#81492=CARTESIAN_POINT('Ctrl Pts',(50.8829165559117,248.335935717821,31.8993563735458)) ;
#81493=CARTESIAN_POINT('Ctrl Pts',(50.7804359845514,248.334789190028,31.8993563735458)) ;
#81494=CARTESIAN_POINT('Ctrl Pts',(50.6739766272416,248.334513975409,31.8993563735458)) ;
#81495=CARTESIAN_POINT('Ctrl Pts',(50.4785264203756,248.304964355459,31.8993563735458)) ;
#81496=CARTESIAN_POINT('Ctrl Pts',(50.3992728553965,248.283451733373,31.8993563735458)) ;
#81497=CARTESIAN_POINT('Ctrl Pts',(50.3226967032828,248.263264100802,31.8993563735458)) ;
#81498=CARTESIAN_POINT('Ctrl Pts',(50.8835850255371,248.273026011925,31.9213203435596)) ;
#81499=CARTESIAN_POINT('Ctrl Pts',(50.7811041507587,248.271903096087,31.9213203435596)) ;
#81500=CARTESIAN_POINT('Ctrl Pts',(50.6772024747733,248.271387553944,31.9213203435596)) ;
#81501=CARTESIAN_POINT('Ctrl Pts',(50.4927328800327,248.243483059088,31.9213203435596)) ;
#81502=CARTESIAN_POINT('Ctrl Pts',(50.4153379366858,248.22264313048,31.9213203435596)) ;
#81503=CARTESIAN_POINT('Ctrl Pts',(50.3387687773397,248.202438395848,31.9213203435596)) ;
#81504=CARTESIAN_POINT('Ctrl Pts',(50.8838711418303,248.246099594967,31.9213203435596)) ;
#81505=CARTESIAN_POINT('Ctrl Pts',(50.7813898306089,248.245010643067,31.9213203435596)) ;
#81506=CARTESIAN_POINT('Ctrl Pts',(50.678579872875,248.244375290024,31.9213203435596)) ;
#81507=CARTESIAN_POINT('Ctrl Pts',(50.4988146088647,248.217168446757,31.9213203435596)) ;
#81508=CARTESIAN_POINT('Ctrl Pts',(50.4222069973681,248.196633301102,31.9213203435596)) ;
#81509=CARTESIAN_POINT('Ctrl Pts',(50.3456478965673,248.176403966502,31.9213203435596)) ;
#81510=CARTESIAN_POINT('Ctrl Pts',(50.3549449524769,248.178861357243,31.9213203435596)) ;
#81511=CARTESIAN_POINT('Ctrl Pts',(50.4284115903355,248.198281497898,31.9213203435596)) ;
#81512=CARTESIAN_POINT('Ctrl Pts',(50.5019861952148,248.217648455246,31.9213203435596)) ;
#81513=CARTESIAN_POINT('Ctrl Pts',(50.6783454900482,248.244339817004,31.9213203435596)) ;
#81514=CARTESIAN_POINT('Ctrl Pts',(50.7809146033543,248.245007627582,31.9213203435596)) ;
#81515=CARTESIAN_POINT('Ctrl Pts',(50.8831605632216,248.246092051596,31.9213203435596)) ;
#81516=CARTESIAN_POINT('Origin',(53.7,239.383507185188,31.9213203435596)) ;
#81517=CARTESIAN_POINT('Origin',(68.7473528137424,242.977647186258,31.7413203435596)) ;
#81518=CARTESIAN_POINT('',(68.3897056274848,242.62,31.6213203435596)) ;
#81519=CARTESIAN_POINT('',(69.6,243.830294372515,31.6213203435596)) ;
#81520=CARTESIAN_POINT('',(68.7473528137424,242.977647186258,31.6213203435596)) ;
#81521=CARTESIAN_POINT('',(69.6,244.,31.7413203435596)) ;
#81522=CARTESIAN_POINT('Origin',(69.6,243.830294372515,31.7413203435596)) ;
#81523=CARTESIAN_POINT('',(68.1,242.5,31.7413203435596)) ;
#81524=CARTESIAN_POINT('',(68.6625,243.0625,31.7413203435596)) ;
#81525=CARTESIAN_POINT('Origin',(68.3897056274848,242.62,31.7413203435596)) ;
#81526=CARTESIAN_POINT('Origin',(69.7026471862576,243.727647186258,31.7413203435596)) ;
#81527=CARTESIAN_POINT('',(71.1,242.5,31.7413203435596)) ;
#81528=CARTESIAN_POINT('',(69.7875,243.8125,31.7413203435596)) ;
#81529=CARTESIAN_POINT('',(70.8102943725152,242.62,31.6213203435596)) ;
#81530=CARTESIAN_POINT('',(69.7026471862576,243.727647186258,31.6213203435596)) ;
#81531=CARTESIAN_POINT('Origin',(70.8102943725152,242.62,31.7413203435596)) ;
#81532=CARTESIAN_POINT('Origin',(70.35,242.62,31.7413203435596)) ;
#81533=CARTESIAN_POINT('',(70.35,242.5,31.7413203435596)) ;
#81534=CARTESIAN_POINT('',(70.35,242.62,31.6213203435596)) ;
#81535=CARTESIAN_POINT('Origin',(71.1,242.5,31.9213203435596)) ;
#81536=CARTESIAN_POINT('',(68.1,242.5,31.8013203435596)) ;
#81537=CARTESIAN_POINT('',(68.1,242.5,31.9213203435596)) ;
#81538=CARTESIAN_POINT('',(71.1,242.5,31.8013203435596)) ;
#81539=CARTESIAN_POINT('',(62.4,242.5,31.8013203435596)) ;
#81540=CARTESIAN_POINT('',(71.1,242.5,31.9213203435596)) ;
#81541=CARTESIAN_POINT('Origin',(68.1,242.5,31.9213203435596)) ;
#81542=CARTESIAN_POINT('',(69.6,244.,31.8013203435596)) ;
#81543=CARTESIAN_POINT('',(69.6,244.,31.9213203435596)) ;
#81544=CARTESIAN_POINT('',(63.720876796297,238.120876796297,31.8013203435596)) ;
#81545=CARTESIAN_POINT('Origin',(69.6,243.25,31.6213203435596)) ;
#81546=CARTESIAN_POINT('Origin',(68.22,240.125,31.7413203435596)) ;
#81547=CARTESIAN_POINT('',(68.22,240.12,31.6213203435596)) ;
#81548=CARTESIAN_POINT('',(68.22,240.38,31.6213203435596)) ;
#81549=CARTESIAN_POINT('',(68.22,240.125,31.6213203435596)) ;
#81550=CARTESIAN_POINT('',(68.1,240.5,31.7413203435596)) ;
#81551=CARTESIAN_POINT('Origin',(68.22,240.38,31.7413203435596)) ;
#81552=CARTESIAN_POINT('',(68.1,240.,31.7413203435596)) ;
#81553=CARTESIAN_POINT('',(68.1,240.125,31.7413203435596)) ;
#81554=CARTESIAN_POINT('Origin',(68.22,240.12,31.7413203435596)) ;
#81555=CARTESIAN_POINT('Origin',(68.85,240.38,31.7413203435596)) ;
#81556=CARTESIAN_POINT('',(71.1,240.5,31.7413203435596)) ;
#81557=CARTESIAN_POINT('',(68.85,240.5,31.7413203435596)) ;
#81558=CARTESIAN_POINT('',(70.98,240.38,31.6213203435596)) ;
#81559=CARTESIAN_POINT('',(68.85,240.38,31.6213203435596)) ;
#81560=CARTESIAN_POINT('Origin',(70.98,240.38,31.7413203435596)) ;
#81561=CARTESIAN_POINT('Origin',(70.98,240.375,31.7413203435596)) ;
#81562=CARTESIAN_POINT('',(71.1,240.,31.7413203435596)) ;
#81563=CARTESIAN_POINT('',(71.1,240.375,31.7413203435596)) ;
#81564=CARTESIAN_POINT('',(70.98,240.12,31.6213203435596)) ;
#81565=CARTESIAN_POINT('',(70.98,240.375,31.6213203435596)) ;
#81566=CARTESIAN_POINT('Origin',(70.98,240.12,31.7413203435596)) ;
#81567=CARTESIAN_POINT('Origin',(70.35,240.12,31.7413203435596)) ;
#81568=CARTESIAN_POINT('',(70.35,240.,31.7413203435596)) ;
#81569=CARTESIAN_POINT('',(70.35,240.12,31.6213203435596)) ;
#81570=CARTESIAN_POINT('Origin',(71.1,240.,31.9213203435596)) ;
#81571=CARTESIAN_POINT('',(68.1,240.,31.8013203435596)) ;
#81572=CARTESIAN_POINT('',(68.1,240.,31.9213203435596)) ;
#81573=CARTESIAN_POINT('',(71.1,240.,31.8013203435596)) ;
#81574=CARTESIAN_POINT('',(62.4,240.,31.8013203435596)) ;
#81575=CARTESIAN_POINT('',(71.1,240.,31.9213203435596)) ;
#81576=CARTESIAN_POINT('Origin',(68.1,240.,31.9213203435596)) ;
#81577=CARTESIAN_POINT('',(68.1,240.5,31.8013203435596)) ;
#81578=CARTESIAN_POINT('',(68.1,240.5,31.9213203435596)) ;
#81579=CARTESIAN_POINT('',(68.1,239.691753592594,31.8013203435596)) ;
#81580=CARTESIAN_POINT('Origin',(69.6,240.25,31.6213203435596)) ;
#81581=CARTESIAN_POINT('Origin',(69.4973528137424,236.772352813742,31.7413203435596)) ;
#81582=CARTESIAN_POINT('',(69.6,236.669705627485,31.6213203435596)) ;
#81583=CARTESIAN_POINT('',(68.3897056274848,237.88,31.6213203435596)) ;
#81584=CARTESIAN_POINT('',(69.4973528137424,236.772352813742,31.6213203435596)) ;
#81585=CARTESIAN_POINT('',(68.1,238.,31.7413203435596)) ;
#81586=CARTESIAN_POINT('Origin',(68.3897056274848,237.88,31.7413203435596)) ;
#81587=CARTESIAN_POINT('',(69.6,236.5,31.7413203435596)) ;
#81588=CARTESIAN_POINT('',(69.4125,236.6875,31.7413203435596)) ;
#81589=CARTESIAN_POINT('Origin',(69.6,236.669705627485,31.7413203435596)) ;
#81590=CARTESIAN_POINT('Origin',(68.85,237.88,31.7413203435596)) ;
#81591=CARTESIAN_POINT('',(71.1,238.,31.7413203435596)) ;
#81592=CARTESIAN_POINT('',(68.85,238.,31.7413203435596)) ;
#81593=CARTESIAN_POINT('',(70.8102943725152,237.88,31.6213203435596)) ;
#81594=CARTESIAN_POINT('',(68.85,237.88,31.6213203435596)) ;
#81595=CARTESIAN_POINT('Origin',(70.8102943725152,237.88,31.7413203435596)) ;
#81596=CARTESIAN_POINT('Origin',(70.4526471862576,237.522352813742,31.7413203435596)) ;
#81597=CARTESIAN_POINT('',(70.5375,237.4375,31.7413203435596)) ;
#81598=CARTESIAN_POINT('',(70.4526471862576,237.522352813742,31.6213203435596)) ;
#81599=CARTESIAN_POINT('Origin',(71.1,238.,31.9213203435596)) ;
#81600=CARTESIAN_POINT('',(69.6,236.5,31.8013203435596)) ;
#81601=CARTESIAN_POINT('',(69.6,236.5,31.9213203435596)) ;
#81602=CARTESIAN_POINT('',(71.1,238.,31.8013203435596)) ;
#81603=CARTESIAN_POINT('',(67.095876796297,233.995876796297,31.8013203435596)) ;
#81604=CARTESIAN_POINT('',(71.1,238.,31.9213203435596)) ;
#81605=CARTESIAN_POINT('Origin',(69.6,236.5,31.9213203435596)) ;
#81606=CARTESIAN_POINT('',(68.1,238.,31.8013203435596)) ;
#81607=CARTESIAN_POINT('',(68.1,238.,31.9213203435596)) ;
#81608=CARTESIAN_POINT('',(64.9041232037029,241.195876796297,31.8013203435596)) ;
#81609=CARTESIAN_POINT('Origin',(69.6,237.25,31.6213203435596)) ;
#81610=CARTESIAN_POINT('Origin',(52.4941050300712,244.948850672818,31.8013203435596)) ;
#81611=CARTESIAN_POINT('',(48.8053003149063,250.720744087106,31.9213203435596)) ;
#81612=CARTESIAN_POINT('',(49.61999553422,249.445986003055,31.9213203435596)) ;
#81613=CARTESIAN_POINT('',(52.4941050300712,244.948850672818,31.9213203435596)) ;
#81614=CARTESIAN_POINT('Ctrl Pts',(49.619995533665,249.445986166465,31.9213203435595)) ;
#81615=CARTESIAN_POINT('Ctrl Pts',(49.6203404723475,249.445987337983,31.9213203432281)) ;
#81616=CARTESIAN_POINT('Ctrl Pts',(49.6206841195624,249.445991847541,31.9213192876678)) ;
#81617=CARTESIAN_POINT('Ctrl Pts',(49.6271977972035,249.44614280716,31.9212785208871)) ;
#81618=CARTESIAN_POINT('Ctrl Pts',(49.6317059524695,249.447345115284,31.9208773504705)) ;
#81619=CARTESIAN_POINT('Ctrl Pts',(49.6380743219538,249.44937032073,31.9201693929286)) ;
#81620=CARTESIAN_POINT('Ctrl Pts',(49.641690337665,249.451131784247,31.9195319535847)) ;
#81621=CARTESIAN_POINT('Ctrl Pts',(49.6518044956798,249.45763877911,31.9169593737309)) ;
#81622=CARTESIAN_POINT('Ctrl Pts',(49.6572528688844,249.463335401781,31.9144710691175)) ;
#81623=CARTESIAN_POINT('Ctrl Pts',(49.666878845865,249.473896545401,31.9084510815192)) ;
#81624=CARTESIAN_POINT('Ctrl Pts',(49.6712115535048,249.478917613583,31.9049863994144)) ;
#81625=CARTESIAN_POINT('Ctrl Pts',(49.6783494210367,249.484542782463,31.8989002966151)) ;
#81626=CARTESIAN_POINT('Ctrl Pts',(49.6834227994079,249.487937662943,31.894992295344)) ;
#81627=CARTESIAN_POINT('Ctrl Pts',(49.6989702717527,249.491136363809,31.880164499323)) ;
#81628=CARTESIAN_POINT('Ctrl Pts',(49.7070380162235,249.492141350405,31.8716282984031)) ;
#81629=CARTESIAN_POINT('Ctrl Pts',(49.7162040167626,249.497712159108,31.8523734086746)) ;
#81630=CARTESIAN_POINT('Ctrl Pts',(49.7184485652111,249.500582089905,31.8446052087515)) ;
#81631=CARTESIAN_POINT('Ctrl Pts',(49.7208851754006,249.508221113742,31.8235840752159)) ;
#81632=CARTESIAN_POINT('Ctrl Pts',(49.7201772727542,249.512066286148,31.812221963213)) ;
#81633=CARTESIAN_POINT('Ctrl Pts',(49.7201772727542,249.512066286148,31.8013203435596)) ;
#81634=CARTESIAN_POINT('Origin',(48.8053003149063,250.720744087106,31.8013203435596)) ;
#81635=CARTESIAN_POINT('Ctrl Pts',(50.1645741624171,248.974905023649,31.8013203435596)) ;
#81636=CARTESIAN_POINT('Ctrl Pts',(50.1628717618181,248.976605820465,31.8013203435596)) ;
#81637=CARTESIAN_POINT('Ctrl Pts',(50.161169441236,248.978306941473,31.8013203435596)) ;
#81638=CARTESIAN_POINT('Ctrl Pts',(50.0792906217163,249.060079868447,31.8013203435597)) ;
#81639=CARTESIAN_POINT('Ctrl Pts',(50.0018980844143,249.137814413213,31.8013203435595)) ;
#81640=CARTESIAN_POINT('Ctrl Pts',(49.8585796911378,249.309274633528,31.8013203435596)) ;
#81641=CARTESIAN_POINT('Ctrl Pts',(49.7903320475991,249.408935320061,31.801320343559)) ;
#81642=CARTESIAN_POINT('Ctrl Pts',(49.719851873712,249.512544638728,31.8013203435596)) ;
#81643=CARTESIAN_POINT('Ctrl Pts',(49.7195269576717,249.513021952172,31.8013203435596)) ;
#81644=CARTESIAN_POINT('Ctrl Pts',(49.7192021347817,249.513499261461,31.8013203435596)) ;
#81645=CARTESIAN_POINT('Ctrl Pts',(50.1645741624171,248.974905023649,31.8372242596007)) ;
#81646=CARTESIAN_POINT('Ctrl Pts',(50.1628717618181,248.976605820465,31.8372242596007)) ;
#81647=CARTESIAN_POINT('Ctrl Pts',(50.161169441236,248.978306941473,31.8372242596007)) ;
#81648=CARTESIAN_POINT('Ctrl Pts',(50.0792906217163,249.060079868447,31.8372242596007)) ;
#81649=CARTESIAN_POINT('Ctrl Pts',(50.0018980844143,249.137814413213,31.8372242596006)) ;
#81650=CARTESIAN_POINT('Ctrl Pts',(49.8585796911378,249.309274633528,31.8372242596006)) ;
#81651=CARTESIAN_POINT('Ctrl Pts',(49.7903320475991,249.408935320061,31.8372242596001)) ;
#81652=CARTESIAN_POINT('Ctrl Pts',(49.719851873712,249.512544638728,31.8372242596007)) ;
#81653=CARTESIAN_POINT('Ctrl Pts',(49.7195269576717,249.513021952172,31.8372242596007)) ;
#81654=CARTESIAN_POINT('Ctrl Pts',(49.7192021347817,249.513499261461,31.8372242596007)) ;
#81655=CARTESIAN_POINT('Ctrl Pts',(50.1432587188193,248.953569480441,31.8993563739025)) ;
#81656=CARTESIAN_POINT('Ctrl Pts',(50.1415558219281,248.95526983324,31.8993563739025)) ;
#81657=CARTESIAN_POINT('Ctrl Pts',(50.1398544635708,248.956971826313,31.8993563739025)) ;
#81658=CARTESIAN_POINT('Ctrl Pts',(50.057967123475,249.038735748406,31.8993563739025)) ;
#81659=CARTESIAN_POINT('Ctrl Pts',(49.9798830936785,249.117126688483,31.8993563739025)) ;
#81660=CARTESIAN_POINT('Ctrl Pts',(49.8341996896905,249.291413887079,31.8993563739025)) ;
#81661=CARTESIAN_POINT('Ctrl Pts',(49.7653887727712,249.391960366771,31.8993563739023)) ;
#81662=CARTESIAN_POINT('Ctrl Pts',(49.6949192354727,249.495577339479,31.8993563739025)) ;
#81663=CARTESIAN_POINT('Ctrl Pts',(49.6945936096815,249.496053982978,31.8993563739025)) ;
#81664=CARTESIAN_POINT('Ctrl Pts',(49.6942691558659,249.496531642236,31.8993563739025)) ;
#81665=CARTESIAN_POINT('Ctrl Pts',(50.0987932972223,248.90906212973,31.9213203435596)) ;
#81666=CARTESIAN_POINT('Ctrl Pts',(50.0970906038601,248.91076266462,31.9213203435596)) ;
#81667=CARTESIAN_POINT('Ctrl Pts',(50.095388780737,248.912464241265,31.9213203435596)) ;
#81668=CARTESIAN_POINT('Ctrl Pts',(50.0135099010427,248.994236060385,31.9213203435596)) ;
#81669=CARTESIAN_POINT('Ctrl Pts',(49.9339632706332,249.073967528443,31.9213203435596)) ;
#81670=CARTESIAN_POINT('Ctrl Pts',(49.7833426499648,249.254164571414,31.9213203435596)) ;
#81671=CARTESIAN_POINT('Ctrl Pts',(49.713386826283,249.356572966886,31.9213203435597)) ;
#81672=CARTESIAN_POINT('Ctrl Pts',(49.6429072391231,249.460181618977,31.9213203435596)) ;
#81673=CARTESIAN_POINT('Ctrl Pts',(49.6425819221073,249.460658553386,31.9213203435596)) ;
#81674=CARTESIAN_POINT('Ctrl Pts',(49.6422573169346,249.461136069123,31.9213203435596)) ;
#81675=CARTESIAN_POINT('Ctrl Pts',(50.0797613456432,248.890012231782,31.9213203435596)) ;
#81676=CARTESIAN_POINT('Ctrl Pts',(50.0780589450442,248.891713028598,31.9213203435596)) ;
#81677=CARTESIAN_POINT('Ctrl Pts',(50.0763565126285,248.893414055885,31.9213203435596)) ;
#81678=CARTESIAN_POINT('Ctrl Pts',(49.9944856092052,248.975193684333,31.9213203435596)) ;
#81679=CARTESIAN_POINT('Ctrl Pts',(49.9143096240871,249.055494147431,31.9213203435596)) ;
#81680=CARTESIAN_POINT('Ctrl Pts',(49.761575185646,249.238222792144,31.9213203435596)) ;
#81681=CARTESIAN_POINT('Ctrl Pts',(49.6911343223267,249.341430458474,31.9213203435597)) ;
#81682=CARTESIAN_POINT('Ctrl Pts',(49.6206450819629,249.445031517405,31.9213203435597)) ;
#81683=CARTESIAN_POINT('Ctrl Pts',(49.620320194148,249.445508856619,31.9213203435596)) ;
#81684=CARTESIAN_POINT('Ctrl Pts',(49.619995371258,249.445986165908,31.9213203435596)) ;
#81685=CARTESIAN_POINT('',(50.0797613456432,248.890012231782,31.9213203435596)) ;
#81686=CARTESIAN_POINT('Ctrl Pts',(49.6199955742298,249.445985867652,31.9213203435596)) ;
#81687=CARTESIAN_POINT('Ctrl Pts',(49.6203203294896,249.445508657769,31.9213203435596)) ;
#81688=CARTESIAN_POINT('Ctrl Pts',(49.6206451495996,249.445031417996,31.9213203435597)) ;
#81689=CARTESIAN_POINT('Ctrl Pts',(49.6911343223267,249.341430458474,31.9213203435597)) ;
#81690=CARTESIAN_POINT('Ctrl Pts',(49.761575185646,249.238222792144,31.9213203435596)) ;
#81691=CARTESIAN_POINT('Ctrl Pts',(49.9143096240871,249.055494147431,31.9213203435596)) ;
#81692=CARTESIAN_POINT('Ctrl Pts',(49.9944856092052,248.975193684333,31.9213203435596)) ;
#81693=CARTESIAN_POINT('Ctrl Pts',(50.0763565126285,248.893414055885,31.9213203435596)) ;
#81694=CARTESIAN_POINT('Ctrl Pts',(50.0780589450442,248.891713028598,31.9213203435596)) ;
#81695=CARTESIAN_POINT('Ctrl Pts',(50.0797613456432,248.890012231782,31.9213203435596)) ;
#81696=CARTESIAN_POINT('Ctrl Pts',(50.0797613456432,248.890012231782,31.9213203435596)) ;
#81697=CARTESIAN_POINT('Ctrl Pts',(50.0799550565321,248.890230949474,31.9213203435596)) ;
#81698=CARTESIAN_POINT('Ctrl Pts',(50.0801487695989,248.890449669304,31.9213192394347)) ;
#81699=CARTESIAN_POINT('Ctrl Pts',(50.0803424810526,248.890668386944,31.921317033763)) ;
#81700=CARTESIAN_POINT('Ctrl Pts',(50.0863819669867,248.897487509339,31.9212482658966)) ;
#81701=CARTESIAN_POINT('Ctrl Pts',(50.0923858427197,248.904266041468,31.920113765387)) ;
#81702=CARTESIAN_POINT('Ctrl Pts',(50.098240144254,248.910875306167,31.9179984115576)) ;
#81703=CARTESIAN_POINT('Ctrl Pts',(50.1026283517431,248.915829411226,31.9164128062617)) ;
#81704=CARTESIAN_POINT('Ctrl Pts',(50.1069328634758,248.920688757015,31.9142748253259)) ;
#81705=CARTESIAN_POINT('Ctrl Pts',(50.1111024611988,248.925395931222,31.9116016099452)) ;
#81706=CARTESIAN_POINT('Ctrl Pts',(50.1166571287938,248.93166674912,31.9080403976087)) ;
#81707=CARTESIAN_POINT('Ctrl Pts',(50.1219117234167,248.937598907753,31.9035702316688)) ;
#81708=CARTESIAN_POINT('Ctrl Pts',(50.1267497978321,248.943063509505,31.8982512360342)) ;
#81709=CARTESIAN_POINT('Ctrl Pts',(50.1276721474668,248.944105302788,31.8972372016769)) ;
#81710=CARTESIAN_POINT('Ctrl Pts',(50.1285793102163,248.945130054085,31.8961921802598)) ;
#81711=CARTESIAN_POINT('Ctrl Pts',(50.1294703957101,248.946136786457,31.8951164031763)) ;
#81712=CARTESIAN_POINT('Ctrl Pts',(50.1319444308956,248.948931906936,31.8921295849925)) ;
#81713=CARTESIAN_POINT('Ctrl Pts',(50.1342946961643,248.951588289624,31.8889058568381)) ;
#81714=CARTESIAN_POINT('Ctrl Pts',(50.1365137723335,248.954096684356,31.8854671010793)) ;
#81715=CARTESIAN_POINT('Ctrl Pts',(50.1407310642358,248.958863818055,31.8789318423909)) ;
#81716=CARTESIAN_POINT('Ctrl Pts',(50.1444295692805,248.963045335349,31.8716947525886)) ;
#81717=CARTESIAN_POINT('Ctrl Pts',(50.1475706336284,248.966594182085,31.8639255828771)) ;
#81718=CARTESIAN_POINT('Ctrl Pts',(50.1497901014565,248.969101787879,31.8584359079403)) ;
#81719=CARTESIAN_POINT('Ctrl Pts',(50.1517308057983,248.971293070318,31.8526794530798)) ;
#81720=CARTESIAN_POINT('Ctrl Pts',(50.1533696323212,248.973141935655,31.8467079120488)) ;
#81721=CARTESIAN_POINT('Ctrl Pts',(50.1556680971207,248.97573498125,31.8383327871238)) ;
#81722=CARTESIAN_POINT('Ctrl Pts',(50.1573486404184,248.977627070085,31.8296281500221)) ;
#81723=CARTESIAN_POINT('Ctrl Pts',(50.1583591663423,248.978763132081,31.8207452397396)) ;
#81724=CARTESIAN_POINT('Ctrl Pts',(50.1590537646987,248.979544019316,31.8146394538937)) ;
#81725=CARTESIAN_POINT('Ctrl Pts',(50.1594312220891,248.979967107938,31.8084487630574)) ;
#81726=CARTESIAN_POINT('Ctrl Pts',(50.1594644902513,248.980004403535,31.80221996166)) ;
#81727=CARTESIAN_POINT('Ctrl Pts',(50.1594660914167,248.980006198537,31.8019201752897)) ;
#81728=CARTESIAN_POINT('Ctrl Pts',(50.1594668937473,248.980007097905,31.8016203008231)) ;
#81729=CARTESIAN_POINT('Ctrl Pts',(50.1594668937473,248.980007097905,31.8013203435596)) ;
#81730=CARTESIAN_POINT('Ctrl Pts',(50.4787029267369,248.780825931436,31.8013203435597)) ;
#81731=CARTESIAN_POINT('Ctrl Pts',(50.4117018449641,248.813931863473,31.8013203435597)) ;
#81732=CARTESIAN_POINT('Ctrl Pts',(50.3493334652158,248.845229869203,31.8013203435597)) ;
#81733=CARTESIAN_POINT('Ctrl Pts',(50.2498263991114,248.90954814415,31.8013203435596)) ;
#81734=CARTESIAN_POINT('Ctrl Pts',(50.2061026564305,248.943426158234,31.8013203435597)) ;
#81735=CARTESIAN_POINT('Ctrl Pts',(50.1575737020552,248.981492111274,31.8013203435596)) ;
#81736=CARTESIAN_POINT('Ctrl Pts',(50.1556790282941,248.982976184296,31.8013203435596)) ;
#81737=CARTESIAN_POINT('Ctrl Pts',(50.1537849828817,248.984460636374,31.8013203435596)) ;
#81738=CARTESIAN_POINT('Ctrl Pts',(50.4787029267369,248.780825931436,31.8372242596007)) ;
#81739=CARTESIAN_POINT('Ctrl Pts',(50.4117018449641,248.813931863473,31.8372242596007)) ;
#81740=CARTESIAN_POINT('Ctrl Pts',(50.3493334652158,248.845229869203,31.8372242596007)) ;
#81741=CARTESIAN_POINT('Ctrl Pts',(50.2498263991114,248.90954814415,31.8372242596007)) ;
#81742=CARTESIAN_POINT('Ctrl Pts',(50.2061026564305,248.943426158234,31.8372242596007)) ;
#81743=CARTESIAN_POINT('Ctrl Pts',(50.1575737020552,248.981492111274,31.8372242596007)) ;
#81744=CARTESIAN_POINT('Ctrl Pts',(50.1556790282941,248.982976184296,31.8372242596007)) ;
#81745=CARTESIAN_POINT('Ctrl Pts',(50.1537849828817,248.984460636374,31.8372242596007)) ;
#81746=CARTESIAN_POINT('Ctrl Pts',(50.4653430446037,248.753787678766,31.8993563735393)) ;
#81747=CARTESIAN_POINT('Ctrl Pts',(50.3983338831863,248.786874129495,31.8993563735393)) ;
#81748=CARTESIAN_POINT('Ctrl Pts',(50.3347981036532,248.818711381287,31.8993563735393)) ;
#81749=CARTESIAN_POINT('Ctrl Pts',(50.2320023038783,248.885156890167,31.8993563735392)) ;
#81750=CARTESIAN_POINT('Ctrl Pts',(50.1874911512665,248.919683104852,31.8993563735392)) ;
#81751=CARTESIAN_POINT('Ctrl Pts',(50.1389704723505,248.957755600037,31.8993563735392)) ;
#81752=CARTESIAN_POINT('Ctrl Pts',(50.1370744698898,248.959238465174,31.8993563735392)) ;
#81753=CARTESIAN_POINT('Ctrl Pts',(50.1351811121424,248.96072354406,31.8993563735392)) ;
#81754=CARTESIAN_POINT('Ctrl Pts',(50.4374734494912,248.697384100731,31.9213203435597)) ;
#81755=CARTESIAN_POINT('Ctrl Pts',(50.3704676015478,248.730478540772,31.9213203435597)) ;
#81756=CARTESIAN_POINT('Ctrl Pts',(50.3044864917679,248.763398175418,31.9213203435596)) ;
#81757=CARTESIAN_POINT('Ctrl Pts',(50.1948178799082,248.834278555724,31.9213203435596)) ;
#81758=CARTESIAN_POINT('Ctrl Pts',(50.1486909620483,248.870172693384,31.9213203435596)) ;
#81759=CARTESIAN_POINT('Ctrl Pts',(50.100161151985,248.908238097848,31.9213203435596)) ;
#81760=CARTESIAN_POINT('Ctrl Pts',(50.0982658507559,248.90972158238,31.9213203435596)) ;
#81761=CARTESIAN_POINT('Ctrl Pts',(50.0963722109961,248.911206404212,31.9213203435596)) ;
#81762=CARTESIAN_POINT('Ctrl Pts',(50.4255447919364,248.673242416413,31.9213203435597)) ;
#81763=CARTESIAN_POINT('Ctrl Pts',(50.3585437101636,248.706348348451,31.9213203435597)) ;
#81764=CARTESIAN_POINT('Ctrl Pts',(50.2915142881931,248.739724202851,31.9213203435596)) ;
#81765=CARTESIAN_POINT('Ctrl Pts',(50.1789019553601,248.812502338361,31.9213203435596)) ;
#81766=CARTESIAN_POINT('Ctrl Pts',(50.1320879154728,248.848984582,31.9213203435596)) ;
#81767=CARTESIAN_POINT('Ctrl Pts',(50.0835498156237,248.88704350896,31.9213203435596)) ;
#81768=CARTESIAN_POINT('Ctrl Pts',(50.0816553910555,248.888527779704,31.9213203435596)) ;
#81769=CARTESIAN_POINT('Ctrl Pts',(50.0797613456432,248.890012231782,31.9213203435596)) ;
#81770=CARTESIAN_POINT('',(50.1488121427117,248.836580765127,31.9213203435596)) ;
#81771=CARTESIAN_POINT('Ctrl Pts',(50.0797613456432,248.890012231782,31.9213203435596)) ;
#81772=CARTESIAN_POINT('Ctrl Pts',(50.0816553910555,248.888527779704,31.9213203435596)) ;
#81773=CARTESIAN_POINT('Ctrl Pts',(50.0835498156237,248.88704350896,31.9213203435596)) ;
#81774=CARTESIAN_POINT('Ctrl Pts',(50.1064328415097,248.869100832722,31.9213203435596)) ;
#81775=CARTESIAN_POINT('Ctrl Pts',(50.1274567829485,248.852661400565,31.9213203435596)) ;
#81776=CARTESIAN_POINT('Ctrl Pts',(50.1487729722068,248.836622996822,31.9213203435596)) ;
#81777=CARTESIAN_POINT('Ctrl Pts',(50.1488635747438,248.836554830776,31.9213203435596)) ;
#81778=CARTESIAN_POINT('Ctrl Pts',(50.1494762260617,248.836435221396,31.9213203435596)) ;
#81779=CARTESIAN_POINT('Ctrl Pts',(50.1500888768936,248.836315582823,31.9213193779744)) ;
#81780=CARTESIAN_POINT('Ctrl Pts',(50.2199516118796,248.822669804373,31.9210999975431)) ;
#81781=CARTESIAN_POINT('Ctrl Pts',(50.2932276038533,248.809136345474,31.9086382258559)) ;
#81782=CARTESIAN_POINT('Ctrl Pts',(50.3849253203238,248.794641665557,31.8816049009698)) ;
#81783=CARTESIAN_POINT('Ctrl Pts',(50.4175915222911,248.789807511013,31.8682131659955)) ;
#81784=CARTESIAN_POINT('Ctrl Pts',(50.4513376409524,248.784832870319,31.845780337943)) ;
#81785=CARTESIAN_POINT('Ctrl Pts',(50.4615810717974,248.783331501165,31.8374718315758)) ;
#81786=CARTESIAN_POINT('Ctrl Pts',(50.4718249633557,248.7818318897,31.8237615537037)) ;
#81787=CARTESIAN_POINT('Ctrl Pts',(50.4744069643523,248.781454197681,31.8193773446321)) ;
#81788=CARTESIAN_POINT('Ctrl Pts',(50.4777976781207,248.780958284954,31.8103794553702)) ;
#81789=CARTESIAN_POINT('Ctrl Pts',(50.4787029267369,248.780825931436,31.8059165081512)) ;
#81790=CARTESIAN_POINT('Ctrl Pts',(50.4787029267369,248.780825931436,31.8013203435597)) ;
#81791=CARTESIAN_POINT('Origin',(52.9087880530785,245.764122216876,31.8013203435596)) ;
#81792=CARTESIAN_POINT('',(50.3204922629989,249.833352139877,31.9213203435596)) ;
#81793=CARTESIAN_POINT('Origin',(50.3206219211603,249.83315301197,31.8013178123873)) ;
#81794=CARTESIAN_POINT('',(49.7560530731217,250.720744087106,31.9213203435596)) ;
#81795=CARTESIAN_POINT('',(52.9087880530785,245.764122216876,31.9213203435596)) ;
#81796=CARTESIAN_POINT('Origin',(49.7560530731217,250.720744087106,31.8013203435596)) ;
#81797=CARTESIAN_POINT('Ctrl Pts',(49.6160227907477,248.400697783797,31.8013203435596)) ;
#81798=CARTESIAN_POINT('Ctrl Pts',(49.6198183561661,248.403715262998,31.8013203435596)) ;
#81799=CARTESIAN_POINT('Ctrl Pts',(49.6236165574443,248.406731398897,31.8013203435596)) ;
#81800=CARTESIAN_POINT('Ctrl Pts',(49.7452792733463,248.503611247398,31.8013203435596)) ;
#81801=CARTESIAN_POINT('Ctrl Pts',(49.8575493060997,248.591032492834,31.8013203435596)) ;
#81802=CARTESIAN_POINT('Ctrl Pts',(50.1251937816473,248.718765363451,31.8013203435596)) ;
#81803=CARTESIAN_POINT('Ctrl Pts',(50.2970303169916,248.749913679334,31.8013203435596)) ;
#81804=CARTESIAN_POINT('Ctrl Pts',(50.4787029267368,248.780825931436,31.8013203435596)) ;
#81805=CARTESIAN_POINT('Ctrl Pts',(49.6160227907477,248.400697783797,31.8372242596007)) ;
#81806=CARTESIAN_POINT('Ctrl Pts',(49.6198183561661,248.403715262998,31.8372242596007)) ;
#81807=CARTESIAN_POINT('Ctrl Pts',(49.6236165574443,248.406731398897,31.8372242596007)) ;
#81808=CARTESIAN_POINT('Ctrl Pts',(49.7452792733463,248.503611247398,31.8372242596006)) ;
#81809=CARTESIAN_POINT('Ctrl Pts',(49.8575493060997,248.591032492834,31.8372242596006)) ;
#81810=CARTESIAN_POINT('Ctrl Pts',(50.1251937816473,248.718765363451,31.8372242596007)) ;
#81811=CARTESIAN_POINT('Ctrl Pts',(50.2970303169916,248.749913679334,31.8372242596006)) ;
#81812=CARTESIAN_POINT('Ctrl Pts',(50.4787029267368,248.780825931436,31.8372242596007)) ;
#81813=CARTESIAN_POINT('Ctrl Pts',(49.5972547773324,248.424305311118,31.8993563712368)) ;
#81814=CARTESIAN_POINT('Ctrl Pts',(49.6010468963673,248.427328920395,31.8993563712368)) ;
#81815=CARTESIAN_POINT('Ctrl Pts',(49.6048519513673,248.430333346679,31.8993563712368)) ;
#81816=CARTESIAN_POINT('Ctrl Pts',(49.7264624062265,248.527276869617,31.8993563712368)) ;
#81817=CARTESIAN_POINT('Ctrl Pts',(49.8405567586885,248.61634984787,31.8993563712368)) ;
#81818=CARTESIAN_POINT('Ctrl Pts',(50.1170880290107,248.748336416003,31.8993563712368)) ;
#81819=CARTESIAN_POINT('Ctrl Pts',(50.2918849936094,248.779783116107,31.8993563712368)) ;
#81820=CARTESIAN_POINT('Ctrl Pts',(50.4736440074975,248.810557413234,31.8993563712368)) ;
#81821=CARTESIAN_POINT('Ctrl Pts',(49.5581034674252,248.473552165211,31.9213203435596)) ;
#81822=CARTESIAN_POINT('Ctrl Pts',(49.5618969998779,248.476573260445,31.9213203435596)) ;
#81823=CARTESIAN_POINT('Ctrl Pts',(49.5656988002261,248.479583622788,31.9213203435596)) ;
#81824=CARTESIAN_POINT('Ctrl Pts',(49.6873510258597,248.576449789539,31.9213203435596)) ;
#81825=CARTESIAN_POINT('Ctrl Pts',(49.8050378320701,248.669116635466,31.9213203435596)) ;
#81826=CARTESIAN_POINT('Ctrl Pts',(50.1003231440839,248.810000534578,31.9213203435596)) ;
#81827=CARTESIAN_POINT('Ctrl Pts',(50.2813671912147,248.841748364289,31.9213203435596)) ;
#81828=CARTESIAN_POINT('Ctrl Pts',(50.4630907693605,248.872579238991,31.9213203435596)) ;
#81829=CARTESIAN_POINT('Ctrl Pts',(49.5413460448266,248.494630651413,31.9213203435596)) ;
#81830=CARTESIAN_POINT('Ctrl Pts',(49.545141610245,248.497648130615,31.9213203435596)) ;
#81831=CARTESIAN_POINT('Ctrl Pts',(49.5489391040554,248.500666073732,31.9213203435596)) ;
#81832=CARTESIAN_POINT('Ctrl Pts',(49.6706342383944,248.597464241588,31.9213203435596)) ;
#81833=CARTESIAN_POINT('Ctrl Pts',(49.7898232864642,248.691693931079,31.9213203435596)) ;
#81834=CARTESIAN_POINT('Ctrl Pts',(50.0931714339411,248.836389995259,31.9213203435596)) ;
#81835=CARTESIAN_POINT('Ctrl Pts',(50.2769011952618,248.86821337696,31.9213203435596)) ;
#81836=CARTESIAN_POINT('Ctrl Pts',(50.458573805007,248.899125629062,31.9213203435596)) ;
#81837=CARTESIAN_POINT('',(49.5413460448267,248.494630651413,31.9213203435596)) ;
#81838=CARTESIAN_POINT('Ctrl Pts',(50.1487803566378,248.836532728787,31.9213203435596)) ;
#81839=CARTESIAN_POINT('Ctrl Pts',(50.0725213308391,248.816277003213,31.9213203435596)) ;
#81840=CARTESIAN_POINT('Ctrl Pts',(49.997874147536,248.790933504476,31.9213203435596)) ;
#81841=CARTESIAN_POINT('Ctrl Pts',(49.7898232864642,248.691693931079,31.9213203435596)) ;
#81842=CARTESIAN_POINT('Ctrl Pts',(49.6706342383944,248.597464241588,31.9213203435596)) ;
#81843=CARTESIAN_POINT('Ctrl Pts',(49.5489391040554,248.500666073732,31.9213203435596)) ;
#81844=CARTESIAN_POINT('Ctrl Pts',(49.545141610245,248.497648130615,31.9213203435596)) ;
#81845=CARTESIAN_POINT('Ctrl Pts',(49.5413460448266,248.494630651413,31.9213203435596)) ;
#81846=CARTESIAN_POINT('',(49.6274057472066,248.409748472578,31.8013203435596)) ;
#81847=CARTESIAN_POINT('Ctrl Pts',(49.5413460448268,248.494630651413,31.9213203435596)) ;
#81848=CARTESIAN_POINT('Ctrl Pts',(49.5415551337113,248.494424426691,31.9213203435596)) ;
#81849=CARTESIAN_POINT('Ctrl Pts',(49.5417642221659,248.494218201969,31.9213192401467)) ;
#81850=CARTESIAN_POINT('Ctrl Pts',(49.5532375457974,248.482901999561,31.9211982874866)) ;
#81851=CARTESIAN_POINT('Ctrl Pts',(49.564495812884,248.471797885886,31.9178840333569)) ;
#81852=CARTESIAN_POINT('Ctrl Pts',(49.5835952095543,248.452961415427,31.9066597394761)) ;
#81853=CARTESIAN_POINT('Ctrl Pts',(49.59317857724,248.443510005046,31.8987710966051)) ;
#81854=CARTESIAN_POINT('Ctrl Pts',(49.6097840808936,248.42713046638,31.875408144021)) ;
#81855=CARTESIAN_POINT('Ctrl Pts',(49.6160001139493,248.420998029143,31.8624282825602)) ;
#81856=CARTESIAN_POINT('Ctrl Pts',(49.6226237280662,248.41446363332,31.8409288459213)) ;
#81857=CARTESIAN_POINT('Ctrl Pts',(49.6243900313392,248.412721148843,31.8332103472442)) ;
#81858=CARTESIAN_POINT('Ctrl Pts',(49.6267809902568,248.410362500334,31.8174327379094)) ;
#81859=CARTESIAN_POINT('Ctrl Pts',(49.6274043438977,248.40974760789,31.8093846732346)) ;
#81860=CARTESIAN_POINT('Ctrl Pts',(49.6274043438977,248.40974760789,31.8013203435596)) ;
#81861=CARTESIAN_POINT('Ctrl Pts',(49.6274063177084,248.409749179632,31.8013203435596)) ;
#81862=CARTESIAN_POINT('Ctrl Pts',(49.7452798059519,248.503611662122,31.8013203435596)) ;
#81863=CARTESIAN_POINT('Ctrl Pts',(49.8575495917875,248.591032629178,31.8013203435596)) ;
#81864=CARTESIAN_POINT('Ctrl Pts',(50.1251937816473,248.718765363451,31.8013203435596)) ;
#81865=CARTESIAN_POINT('Ctrl Pts',(50.2970303169916,248.749913679334,31.8013203435596)) ;
#81866=CARTESIAN_POINT('Ctrl Pts',(50.4787029267368,248.780825931436,31.8013203435596)) ;
#81867=CARTESIAN_POINT('Ctrl Pts',(49.3511580123827,247.683686434724,31.8013203435596)) ;
#81868=CARTESIAN_POINT('Ctrl Pts',(49.3513811606149,247.686507812404,31.8013203435596)) ;
#81869=CARTESIAN_POINT('Ctrl Pts',(49.351606496417,247.689330023121,31.8013203435596)) ;
#81870=CARTESIAN_POINT('Ctrl Pts',(49.3630909791246,247.836615729966,31.8013203435595)) ;
#81871=CARTESIAN_POINT('Ctrl Pts',(49.3759860107092,247.970275925653,31.8013203435596)) ;
#81872=CARTESIAN_POINT('Ctrl Pts',(49.4638970144239,248.194828827023,31.8013203435596)) ;
#81873=CARTESIAN_POINT('Ctrl Pts',(49.5415374649235,248.298874984898,31.8013203435596)) ;
#81874=CARTESIAN_POINT('Ctrl Pts',(49.6303717987922,248.413579230883,31.8013203435596)) ;
#81875=CARTESIAN_POINT('Ctrl Pts',(49.6333346667356,248.41741920385,31.8013203435596)) ;
#81876=CARTESIAN_POINT('Ctrl Pts',(49.6362996924823,248.421256236275,31.8013203435596)) ;
#81877=CARTESIAN_POINT('Ctrl Pts',(49.3511580123827,247.683686434724,31.8372242596007)) ;
#81878=CARTESIAN_POINT('Ctrl Pts',(49.3513811606149,247.686507812404,31.8372242596007)) ;
#81879=CARTESIAN_POINT('Ctrl Pts',(49.351606496417,247.689330023121,31.8372242596007)) ;
#81880=CARTESIAN_POINT('Ctrl Pts',(49.3630909791246,247.836615729966,31.8372242596006)) ;
#81881=CARTESIAN_POINT('Ctrl Pts',(49.3759860107092,247.970275925653,31.8372242596006)) ;
#81882=CARTESIAN_POINT('Ctrl Pts',(49.4638970144239,248.194828827023,31.8372242596006)) ;
#81883=CARTESIAN_POINT('Ctrl Pts',(49.5415374649235,248.298874984898,31.8372242596006)) ;
#81884=CARTESIAN_POINT('Ctrl Pts',(49.6303717987922,248.413579230883,31.8372242596007)) ;
#81885=CARTESIAN_POINT('Ctrl Pts',(49.6333346667356,248.41741920385,31.8372242596007)) ;
#81886=CARTESIAN_POINT('Ctrl Pts',(49.6362996924823,248.421256236275,31.8372242596007)) ;
#81887=CARTESIAN_POINT('Ctrl Pts',(49.3210931084848,247.686064326277,31.899356388327)) ;
#81888=CARTESIAN_POINT('Ctrl Pts',(49.3213103584176,247.688889074995,31.899356388327)) ;
#81889=CARTESIAN_POINT('Ctrl Pts',(49.3215472229959,247.69170499457,31.899356388327)) ;
#81890=CARTESIAN_POINT('Ctrl Pts',(49.3329108418495,247.839022547426,31.8993563883269)) ;
#81891=CARTESIAN_POINT('Ctrl Pts',(49.3458237475767,247.975989259365,31.899356388327)) ;
#81892=CARTESIAN_POINT('Ctrl Pts',(49.4378098065694,248.210938101463,31.899356388327)) ;
#81893=CARTESIAN_POINT('Ctrl Pts',(49.5175746100229,248.31737546829,31.899356388327)) ;
#81894=CARTESIAN_POINT('Ctrl Pts',(49.6065149484319,248.432017131571,31.899356388327)) ;
#81895=CARTESIAN_POINT('Ctrl Pts',(49.609462878417,248.435862398147,31.899356388327)) ;
#81896=CARTESIAN_POINT('Ctrl Pts',(49.6124356305256,248.439696934785,31.899356388327)) ;
#81897=CARTESIAN_POINT('Ctrl Pts',(49.2583756984854,247.69102476786,31.9213203435596)) ;
#81898=CARTESIAN_POINT('Ctrl Pts',(49.2585953667594,247.69384813443,31.9213203435596)) ;
#81899=CARTESIAN_POINT('Ctrl Pts',(49.2588267189017,247.696667220839,31.9213203435596)) ;
#81900=CARTESIAN_POINT('Ctrl Pts',(49.2703008601906,247.843927023218,31.9213203435596)) ;
#81901=CARTESIAN_POINT('Ctrl Pts',(49.2828807770222,247.987714515527,31.9213203435596)) ;
#81902=CARTESIAN_POINT('Ctrl Pts',(49.3834849539174,248.244699535025,31.9213203435596)) ;
#81903=CARTESIAN_POINT('Ctrl Pts',(49.4679013933208,248.355809221579,31.9213203435596)) ;
#81904=CARTESIAN_POINT('Ctrl Pts',(49.5567283655309,248.470487025677,31.9213203435596)) ;
#81905=CARTESIAN_POINT('Ctrl Pts',(49.5596840092843,248.474329911232,31.9213203435596)) ;
#81906=CARTESIAN_POINT('Ctrl Pts',(49.5626535935343,248.478165471159,31.9213203435596)) ;
#81907=CARTESIAN_POINT('Ctrl Pts',(49.2315315926766,247.693147920246,31.9213203435596)) ;
#81908=CARTESIAN_POINT('Ctrl Pts',(49.2317547409087,247.695969297926,31.9213203435596)) ;
#81909=CARTESIAN_POINT('Ctrl Pts',(49.2319788244617,247.698792445045,31.9213203435596)) ;
#81910=CARTESIAN_POINT('Ctrl Pts',(49.2435604941406,247.846006907065,31.9213203435596)) ;
#81911=CARTESIAN_POINT('Ctrl Pts',(49.2559363973039,247.992701048677,31.9213203435596)) ;
#81912=CARTESIAN_POINT('Ctrl Pts',(49.3602487491191,248.259175969039,31.9213203435596)) ;
#81913=CARTESIAN_POINT('Ctrl Pts',(49.4466927160512,248.372233027417,31.9213203435596)) ;
#81914=CARTESIAN_POINT('Ctrl Pts',(49.5354156179722,248.486953981746,31.9213203435596)) ;
#81915=CARTESIAN_POINT('Ctrl Pts',(49.53838101908,248.490793618988,31.9213203435596)) ;
#81916=CARTESIAN_POINT('Ctrl Pts',(49.5413460448267,248.494630651413,31.9213203435596)) ;
#81917=CARTESIAN_POINT('',(49.2315315926766,247.693147920246,31.9213203435596)) ;
#81918=CARTESIAN_POINT('Ctrl Pts',(49.5413460448267,248.494630651413,31.9213203435596)) ;
#81919=CARTESIAN_POINT('Ctrl Pts',(49.53838101908,248.490793618988,31.9213203435596)) ;
#81920=CARTESIAN_POINT('Ctrl Pts',(49.5354156179722,248.486953981746,31.9213203435596)) ;
#81921=CARTESIAN_POINT('Ctrl Pts',(49.4466927160512,248.372233027417,31.9213203435596)) ;
#81922=CARTESIAN_POINT('Ctrl Pts',(49.3602487491191,248.259175969039,31.9213203435596)) ;
#81923=CARTESIAN_POINT('Ctrl Pts',(49.2559363973039,247.992701048677,31.9213203435596)) ;
#81924=CARTESIAN_POINT('Ctrl Pts',(49.2435604941406,247.846006907065,31.9213203435596)) ;
#81925=CARTESIAN_POINT('Ctrl Pts',(49.2319788244617,247.698792445045,31.9213203435596)) ;
#81926=CARTESIAN_POINT('Ctrl Pts',(49.2317547409087,247.695969297926,31.9213203435596)) ;
#81927=CARTESIAN_POINT('Ctrl Pts',(49.2315315926766,247.693147920246,31.9213203435596)) ;
#81928=CARTESIAN_POINT('',(49.3518267393442,247.692149029454,31.8013203435596)) ;
#81929=CARTESIAN_POINT('Ctrl Pts',(49.2315315926766,247.693147920246,31.9213203435596)) ;
#81930=CARTESIAN_POINT('Ctrl Pts',(49.2318239505491,247.693145492984,31.9213203435596)) ;
#81931=CARTESIAN_POINT('Ctrl Pts',(49.2321163107771,247.693143065995,31.9213192394382)) ;
#81932=CARTESIAN_POINT('Ctrl Pts',(49.2324086676693,247.693140639281,31.9213170337815)) ;
#81933=CARTESIAN_POINT('Ctrl Pts',(49.2415098317031,247.693065094895,31.9212483709802)) ;
#81934=CARTESIAN_POINT('Ctrl Pts',(49.2505568709384,247.692990108873,31.9201172490698)) ;
#81935=CARTESIAN_POINT('Ctrl Pts',(49.2593794714521,247.692916421526,31.9180080056539)) ;
#81936=CARTESIAN_POINT('Ctrl Pts',(49.2660335770399,247.692860845691,31.9164171902953)) ;
#81937=CARTESIAN_POINT('Ctrl Pts',(49.2725604492711,247.692806003611,31.9142686983227)) ;
#81938=CARTESIAN_POINT('Ctrl Pts',(49.2788818911616,247.692752877869,31.9115798250687)) ;
#81939=CARTESIAN_POINT('Ctrl Pts',(49.2872630385297,247.692682442251,31.9080148404676)) ;
#81940=CARTESIAN_POINT('Ctrl Pts',(49.2951916702454,247.692615698676,31.9035408183158)) ;
#81941=CARTESIAN_POINT('Ctrl Pts',(49.3024934133583,247.692556314186,31.8982175686063)) ;
#81942=CARTESIAN_POINT('Ctrl Pts',(49.3038700446628,247.692545118154,31.8972139517879)) ;
#81943=CARTESIAN_POINT('Ctrl Pts',(49.305224326051,247.692534188902,31.8961800157529)) ;
#81944=CARTESIAN_POINT('Ctrl Pts',(49.3065549752602,247.692523559636,31.8951159825132)) ;
#81945=CARTESIAN_POINT('Ctrl Pts',(49.3103044615355,247.692493608626,31.8921177632971)) ;
#81946=CARTESIAN_POINT('Ctrl Pts',(49.3138665421931,247.69246602184,31.8888807508021)) ;
#81947=CARTESIAN_POINT('Ctrl Pts',(49.3172291832474,247.692440227635,31.8854270573049)) ;
#81948=CARTESIAN_POINT('Ctrl Pts',(49.3235962748799,247.692391386839,31.8788875597455)) ;
#81949=CARTESIAN_POINT('Ctrl Pts',(49.3291801942726,247.692349272201,31.8716460920431)) ;
#81950=CARTESIAN_POINT('Ctrl Pts',(49.333919892969,247.692311699374,31.863872181942)) ;
#81951=CARTESIAN_POINT('Ctrl Pts',(49.3372625857124,247.692285200977,31.85838959865)) ;
#81952=CARTESIAN_POINT('Ctrl Pts',(49.3401847505064,247.692261008218,31.8526410625285)) ;
#81953=CARTESIAN_POINT('Ctrl Pts',(49.3426515861621,247.692239389276,31.8466779100469)) ;
#81954=CARTESIAN_POINT('Ctrl Pts',(49.3461145160436,247.692209040727,31.8383068704645)) ;
#81955=CARTESIAN_POINT('Ctrl Pts',(49.3486435722209,247.692183923337,31.8296066607461)) ;
#81956=CARTESIAN_POINT('Ctrl Pts',(49.3501628732842,247.69216754168,31.8207281380371)) ;
#81957=CARTESIAN_POINT('Ctrl Pts',(49.3511547437465,247.692156846971,31.8149318250899)) ;
#81958=CARTESIAN_POINT('Ctrl Pts',(49.3517153955676,247.692149915258,31.8090589132011)) ;
#81959=CARTESIAN_POINT('Ctrl Pts',(49.3518117389559,247.692148725188,31.8031494394816)) ;
#81960=CARTESIAN_POINT('Ctrl Pts',(49.3518216729152,247.69214860248,31.8025401141059)) ;
#81961=CARTESIAN_POINT('Ctrl Pts',(49.3518266612828,247.692148540243,31.8019304006143)) ;
#81962=CARTESIAN_POINT('Ctrl Pts',(49.3518266612828,247.692148540243,31.8013203435596)) ;
#81963=CARTESIAN_POINT('Ctrl Pts',(49.351826324154,247.69214926056,31.8013203435596)) ;
#81964=CARTESIAN_POINT('Ctrl Pts',(49.363091023437,247.836616189274,31.8013203435595)) ;
#81965=CARTESIAN_POINT('Ctrl Pts',(49.3759860874712,247.970276121727,31.8013203435596)) ;
#81966=CARTESIAN_POINT('Ctrl Pts',(49.4638968212056,248.194828333482,31.8013203435596)) ;
#81967=CARTESIAN_POINT('Ctrl Pts',(49.5415367709703,248.298874054929,31.8013203435596)) ;
#81968=CARTESIAN_POINT('Ctrl Pts',(49.6274052886232,248.409748827735,31.8013203435596)) ;
#81969=CARTESIAN_POINT('Ctrl Pts',(49.5220917256399,247.081756402944,31.8013203435596)) ;
#81970=CARTESIAN_POINT('Ctrl Pts',(49.5208165737813,247.08422041417,31.8013203435596)) ;
#81971=CARTESIAN_POINT('Ctrl Pts',(49.5195423275549,247.086685824071,31.8013203435596)) ;
#81972=CARTESIAN_POINT('Ctrl Pts',(49.4663642430865,247.189248746888,31.8013203435597)) ;
#81973=CARTESIAN_POINT('Ctrl Pts',(49.4195138367936,247.282633469367,31.8013203435596)) ;
#81974=CARTESIAN_POINT('Ctrl Pts',(49.3668547913298,247.471629570943,31.8013203435596)) ;
#81975=CARTESIAN_POINT('Ctrl Pts',(49.3588813375332,247.577652626811,31.8013203435597)) ;
#81976=CARTESIAN_POINT('Ctrl Pts',(49.3516526720405,247.694972349092,31.8013203435596)) ;
#81977=CARTESIAN_POINT('Ctrl Pts',(49.3514748692129,247.697797498201,31.8013203435596)) ;
#81978=CARTESIAN_POINT('Ctrl Pts',(49.3512986166069,247.700621873608,31.8013203435596)) ;
#81979=CARTESIAN_POINT('Ctrl Pts',(49.5220917256399,247.081756402944,31.8372242596007)) ;
#81980=CARTESIAN_POINT('Ctrl Pts',(49.5208165737813,247.08422041417,31.8372242596007)) ;
#81981=CARTESIAN_POINT('Ctrl Pts',(49.5195423275549,247.086685824071,31.8372242596007)) ;
#81982=CARTESIAN_POINT('Ctrl Pts',(49.4663642430865,247.189248746888,31.8372242596007)) ;
#81983=CARTESIAN_POINT('Ctrl Pts',(49.4195138367936,247.282633469367,31.8372242596007)) ;
#81984=CARTESIAN_POINT('Ctrl Pts',(49.3668547913298,247.471629570943,31.8372242596007)) ;
#81985=CARTESIAN_POINT('Ctrl Pts',(49.3588813375332,247.577652626811,31.8372242596007)) ;
#81986=CARTESIAN_POINT('Ctrl Pts',(49.3516526720405,247.694972349092,31.8372242596007)) ;
#81987=CARTESIAN_POINT('Ctrl Pts',(49.3514748692129,247.697797498201,31.8372242596007)) ;
#81988=CARTESIAN_POINT('Ctrl Pts',(49.3512986166069,247.700621873608,31.8372242596007)) ;
#81989=CARTESIAN_POINT('Ctrl Pts',(49.4953071063915,247.067895079317,31.899356402125)) ;
#81990=CARTESIAN_POINT('Ctrl Pts',(49.4940289586876,247.070358373031,31.899356402125)) ;
#81991=CARTESIAN_POINT('Ctrl Pts',(49.4927605208449,247.072825291279,31.899356402125)) ;
#81992=CARTESIAN_POINT('Ctrl Pts',(49.4395322856787,247.175364270832,31.8993564021251)) ;
#81993=CARTESIAN_POINT('Ctrl Pts',(49.3915127800559,247.27075119156,31.899356402125)) ;
#81994=CARTESIAN_POINT('Ctrl Pts',(49.3367241123045,247.467386546691,31.899356402125)) ;
#81995=CARTESIAN_POINT('Ctrl Pts',(49.3287281528714,247.575768514214,31.8993564021251)) ;
#81996=CARTESIAN_POINT('Ctrl Pts',(49.3215552662865,247.69309484099,31.899356402125)) ;
#81997=CARTESIAN_POINT('Ctrl Pts',(49.3213716917485,247.695918082734,31.899356402125)) ;
#81998=CARTESIAN_POINT('Ctrl Pts',(49.3211983870719,247.698743495868,31.899356402125)) ;
#81999=CARTESIAN_POINT('Ctrl Pts',(49.4394325590996,247.038979410387,31.9213203435596)) ;
#82000=CARTESIAN_POINT('Ctrl Pts',(49.4381556394463,247.041442998223,31.9213203435596)) ;
#82001=CARTESIAN_POINT('Ctrl Pts',(49.436884323614,247.043909228964,31.9213203435596)) ;
#82002=CARTESIAN_POINT('Ctrl Pts',(49.3837071618505,247.146462634709,31.9213203435596)) ;
#82003=CARTESIAN_POINT('Ctrl Pts',(49.3331330179417,247.245909737314,31.9213203435597)) ;
#82004=CARTESIAN_POINT('Ctrl Pts',(49.2738726758569,247.45860094103,31.9213203435596)) ;
#82005=CARTESIAN_POINT('Ctrl Pts',(49.2659876314173,247.571865092995,31.9213203435597)) ;
#82006=CARTESIAN_POINT('Ctrl Pts',(49.2587624951247,247.689175844789,31.9213203435596)) ;
#82007=CARTESIAN_POINT('Ctrl Pts',(49.2585817630851,247.692000083707,31.9213203435596)) ;
#82008=CARTESIAN_POINT('Ctrl Pts',(49.2584072499996,247.694825071459,31.9213203435596)) ;
#82009=CARTESIAN_POINT('Ctrl Pts',(49.4155173179348,247.026603020253,31.9213203435596)) ;
#82010=CARTESIAN_POINT('Ctrl Pts',(49.4142421660762,247.029067031478,31.9213203435596)) ;
#82011=CARTESIAN_POINT('Ctrl Pts',(49.4129671275179,247.031532331052,31.9213203435596)) ;
#82012=CARTESIAN_POINT('Ctrl Pts',(49.3598376892698,247.134102605098,31.9213203435596)) ;
#82013=CARTESIAN_POINT('Ctrl Pts',(49.3081508780161,247.235268173893,31.9213203435597)) ;
#82014=CARTESIAN_POINT('Ctrl Pts',(49.2469717443521,247.454851457692,31.9213203435596)) ;
#82015=CARTESIAN_POINT('Ctrl Pts',(49.2391603974573,247.570198843043,31.9213203435597)) ;
#82016=CARTESIAN_POINT('Ctrl Pts',(49.231884888391,247.687498052493,31.9213203435596)) ;
#82017=CARTESIAN_POINT('Ctrl Pts',(49.2317078452825,247.690323544838,31.9213203435596)) ;
#82018=CARTESIAN_POINT('Ctrl Pts',(49.2315315926766,247.693147920246,31.9213203435596)) ;
#82019=CARTESIAN_POINT('',(49.4155173179349,247.026603020253,31.9213203435596)) ;
#82020=CARTESIAN_POINT('Ctrl Pts',(49.2315315926766,247.693147920246,31.9213203435596)) ;
#82021=CARTESIAN_POINT('Ctrl Pts',(49.2317078452825,247.690323544838,31.9213203435596)) ;
#82022=CARTESIAN_POINT('Ctrl Pts',(49.231884888391,247.687498052493,31.9213203435596)) ;
#82023=CARTESIAN_POINT('Ctrl Pts',(49.2391603974573,247.570198843043,31.9213203435597)) ;
#82024=CARTESIAN_POINT('Ctrl Pts',(49.2469717443521,247.454851457692,31.9213203435596)) ;
#82025=CARTESIAN_POINT('Ctrl Pts',(49.3081508780161,247.235268173893,31.9213203435597)) ;
#82026=CARTESIAN_POINT('Ctrl Pts',(49.3598376892698,247.134102605098,31.9213203435596)) ;
#82027=CARTESIAN_POINT('Ctrl Pts',(49.4129671275179,247.031532331052,31.9213203435596)) ;
#82028=CARTESIAN_POINT('Ctrl Pts',(49.4142421660762,247.029067031478,31.9213203435596)) ;
#82029=CARTESIAN_POINT('Ctrl Pts',(49.4155173179348,247.026603020253,31.9213203435596)) ;
#82030=CARTESIAN_POINT('',(49.5182659490466,247.089147608782,31.8013203435596)) ;
#82031=CARTESIAN_POINT('Ctrl Pts',(49.4155173179349,247.026603020253,31.9213203435597)) ;
#82032=CARTESIAN_POINT('Ctrl Pts',(49.4157670319329,247.026755025144,31.9213203435597)) ;
#82033=CARTESIAN_POINT('Ctrl Pts',(49.4160167483516,247.026907031361,31.9213192394375)) ;
#82034=CARTESIAN_POINT('Ctrl Pts',(49.4162664622726,247.027059035989,31.9213170337681)) ;
#82035=CARTESIAN_POINT('Ctrl Pts',(49.4240469768085,247.031795152474,31.9212483101556)) ;
#82036=CARTESIAN_POINT('Ctrl Pts',(49.4317814689462,247.036503062995,31.9201152014319)) ;
#82037=CARTESIAN_POINT('Ctrl Pts',(49.4393237342447,247.04109353787,31.9180023530773)) ;
#82038=CARTESIAN_POINT('Ctrl Pts',(49.4449984731521,247.044547373733,31.9164126632045)) ;
#82039=CARTESIAN_POINT('Ctrl Pts',(49.4505648075892,247.047934953336,31.9142670803829)) ;
#82040=CARTESIAN_POINT('Ctrl Pts',(49.4559561497916,247.051216117542,31.9115828535184)) ;
#82041=CARTESIAN_POINT('Ctrl Pts',(49.4631144221162,247.05557263324,31.9080189122668)) ;
#82042=CARTESIAN_POINT('Ctrl Pts',(49.4698862001626,247.059693958133,31.9035462640003)) ;
#82043=CARTESIAN_POINT('Ctrl Pts',(49.4761217118301,247.063491285742,31.898224590158)) ;
#82044=CARTESIAN_POINT('Ctrl Pts',(49.4773000339027,247.064208865177,31.8972189556431)) ;
#82045=CARTESIAN_POINT('Ctrl Pts',(49.4784591456912,247.064914843391,31.8961828689005)) ;
#82046=CARTESIAN_POINT('Ctrl Pts',(49.4795979337044,247.065608567612,31.8951165526276)) ;
#82047=CARTESIAN_POINT('Ctrl Pts',(49.4827981454019,247.067558065098,31.8921200003544)) ;
#82048=CARTESIAN_POINT('Ctrl Pts',(49.4858380622011,247.069410896474,31.8888848938609)) ;
#82049=CARTESIAN_POINT('Ctrl Pts',(49.4887077644748,247.071160240999,31.8854333041442)) ;
#82050=CARTESIAN_POINT('Ctrl Pts',(49.4941434979626,247.074473814921,31.8788953709304)) ;
#82051=CARTESIAN_POINT('Ctrl Pts',(49.4989104717773,247.077380441405,31.8716555617629)) ;
#82052=CARTESIAN_POINT('Ctrl Pts',(49.5029578808311,247.079846150381,31.8638834627152)) ;
#82053=CARTESIAN_POINT('Ctrl Pts',(49.5058141003531,247.081586178636,31.8583987635578)) ;
#82054=CARTESIAN_POINT('Ctrl Pts',(49.5083114220383,247.083106343917,31.852647864799)) ;
#82055=CARTESIAN_POINT('Ctrl Pts',(49.5104201017535,247.084388545671,31.8466822212965)) ;
#82056=CARTESIAN_POINT('Ctrl Pts',(49.5133796477241,247.08618812434,31.8383094010603)) ;
#82057=CARTESIAN_POINT('Ctrl Pts',(49.5155424607875,247.087499817604,31.8296073353928)) ;
#82058=CARTESIAN_POINT('Ctrl Pts',(49.51684226662,247.088286631527,31.8207269964985)) ;
#82059=CARTESIAN_POINT('Ctrl Pts',(49.5176934522641,247.088801881343,31.8149116533194)) ;
#82060=CARTESIAN_POINT('Ctrl Pts',(49.5181738049218,247.089091627686,31.8090192524275)) ;
#82061=CARTESIAN_POINT('Ctrl Pts',(49.5182538948739,247.08913993916,31.8030902043847)) ;
#82062=CARTESIAN_POINT('Ctrl Pts',(49.518261859298,247.089144743421,31.8025005991682)) ;
#82063=CARTESIAN_POINT('Ctrl Pts',(49.5182658583933,247.089147155091,31.8019106321131)) ;
#82064=CARTESIAN_POINT('Ctrl Pts',(49.5182658583933,247.089147155091,31.8013203435596)) ;
#82065=CARTESIAN_POINT('Ctrl Pts',(49.5182658425303,247.089147741163,31.8013203435596)) ;
#82066=CARTESIAN_POINT('Ctrl Pts',(49.4663641066775,247.189249018786,31.8013203435597)) ;
#82067=CARTESIAN_POINT('Ctrl Pts',(49.4195137987933,247.282633605752,31.8013203435596)) ;
#82068=CARTESIAN_POINT('Ctrl Pts',(49.3668548399605,247.471629396404,31.8013203435596)) ;
#82069=CARTESIAN_POINT('Ctrl Pts',(49.3588813667358,247.577652238505,31.8013203435597)) ;
#82070=CARTESIAN_POINT('Ctrl Pts',(49.3518266315492,247.692149022813,31.8013203435596)) ;
#82071=CARTESIAN_POINT('Ctrl Pts',(49.9728509295514,246.705084314165,31.8013203435596)) ;
#82072=CARTESIAN_POINT('Ctrl Pts',(49.9695706917073,246.706685069535,31.8013203435596)) ;
#82073=CARTESIAN_POINT('Ctrl Pts',(49.966291605231,246.708288233407,31.8013203435596)) ;
#82074=CARTESIAN_POINT('Ctrl Pts',(49.8668375731075,246.756687889626,31.8013203435596)) ;
#82075=CARTESIAN_POINT('Ctrl Pts',(49.7804572807525,246.80081678555,31.8013203435596)) ;
#82076=CARTESIAN_POINT('Ctrl Pts',(49.6421980930019,246.917171131134,31.8013203435596)) ;
#82077=CARTESIAN_POINT('Ctrl Pts',(49.5823727945931,246.998379121351,31.8013203435596)) ;
#82078=CARTESIAN_POINT('Ctrl Pts',(49.5166663659865,247.091411852008,31.8013203435596)) ;
#82079=CARTESIAN_POINT('Ctrl Pts',(49.5150609156944,247.09367591647,31.8013203435596)) ;
#82080=CARTESIAN_POINT('Ctrl Pts',(49.5134574115132,247.095940874776,31.8013203435596)) ;
#82081=CARTESIAN_POINT('Ctrl Pts',(49.9728509295514,246.705084314165,31.8372242596007)) ;
#82082=CARTESIAN_POINT('Ctrl Pts',(49.9695706917073,246.706685069535,31.8372242596007)) ;
#82083=CARTESIAN_POINT('Ctrl Pts',(49.966291605231,246.708288233407,31.8372242596007)) ;
#82084=CARTESIAN_POINT('Ctrl Pts',(49.8668375731075,246.756687889626,31.8372242596006)) ;
#82085=CARTESIAN_POINT('Ctrl Pts',(49.7804572807525,246.80081678555,31.8372242596007)) ;
#82086=CARTESIAN_POINT('Ctrl Pts',(49.6421980930019,246.917171131134,31.8372242596007)) ;
#82087=CARTESIAN_POINT('Ctrl Pts',(49.5823727945931,246.998379121351,31.8372242596007)) ;
#82088=CARTESIAN_POINT('Ctrl Pts',(49.5166663659865,247.091411852008,31.8372242596007)) ;
#82089=CARTESIAN_POINT('Ctrl Pts',(49.5150609156944,247.09367591647,31.8372242596007)) ;
#82090=CARTESIAN_POINT('Ctrl Pts',(49.5134574115132,247.095940874776,31.8372242596007)) ;
#82091=CARTESIAN_POINT('Ctrl Pts',(49.9596243415484,246.677980638409,31.8993564071237)) ;
#82092=CARTESIAN_POINT('Ctrl Pts',(49.9563408931928,246.679577731124,31.8993564071237)) ;
#82093=CARTESIAN_POINT('Ctrl Pts',(49.953067881515,246.681188239656,31.8993564071237)) ;
#82094=CARTESIAN_POINT('Ctrl Pts',(49.8535780165042,246.729519028743,31.8993564071237)) ;
#82095=CARTESIAN_POINT('Ctrl Pts',(49.76458783128,246.77474795192,31.8993564071237)) ;
#82096=CARTESIAN_POINT('Ctrl Pts',(49.6190805221059,246.8971980461,31.8993564071237)) ;
#82097=CARTESIAN_POINT('Ctrl Pts',(49.5577004345458,246.98090485912,31.8993564071237)) ;
#82098=CARTESIAN_POINT('Ctrl Pts',(49.4920542320471,247.073989023636,31.8993564071237)) ;
#82099=CARTESIAN_POINT('Ctrl Pts',(49.4904438528122,247.076245990223,31.8993564071237)) ;
#82100=CARTESIAN_POINT('Ctrl Pts',(49.4888427989645,247.078514666962,31.8993564071237)) ;
#82101=CARTESIAN_POINT('Ctrl Pts',(49.9320327688979,246.621440505869,31.9213203435596)) ;
#82102=CARTESIAN_POINT('Ctrl Pts',(49.9287506364852,246.623039099855,31.9213203435596)) ;
#82103=CARTESIAN_POINT('Ctrl Pts',(49.9254744022225,246.624645982205,31.9213203435597)) ;
#82104=CARTESIAN_POINT('Ctrl Pts',(49.826031455862,246.673033136406,31.9213203435596)) ;
#82105=CARTESIAN_POINT('Ctrl Pts',(49.7315757026825,246.720314831074,31.9213203435597)) ;
#82106=CARTESIAN_POINT('Ctrl Pts',(49.5707926314164,246.855628276461,31.9213203435597)) ;
#82107=CARTESIAN_POINT('Ctrl Pts',(49.5063980993641,246.944612608217,31.9213203435597)) ;
#82108=CARTESIAN_POINT('Ctrl Pts',(49.4407050846512,247.037634688339,31.9213203435597)) ;
#82109=CARTESIAN_POINT('Ctrl Pts',(49.4390970817449,247.039895245817,31.9213203435597)) ;
#82110=CARTESIAN_POINT('Ctrl Pts',(49.4374950235404,247.042162398423,31.9213203435597)) ;
#82111=CARTESIAN_POINT('Ctrl Pts',(49.920223114908,246.597240384684,31.9213203435596)) ;
#82112=CARTESIAN_POINT('Ctrl Pts',(49.9169428770639,246.598841140054,31.9213203435596)) ;
#82113=CARTESIAN_POINT('Ctrl Pts',(49.9136626226905,246.600443322388,31.9213203435597)) ;
#82114=CARTESIAN_POINT('Ctrl Pts',(49.8142599722259,246.648887834106,31.9213203435596)) ;
#82115=CARTESIAN_POINT('Ctrl Pts',(49.7174613505083,246.697007950007,31.9213203435597)) ;
#82116=CARTESIAN_POINT('Ctrl Pts',(49.5501141329755,246.837851580331,31.9213203435597)) ;
#82117=CARTESIAN_POINT('Ctrl Pts',(49.4844674063744,246.929105544499,31.9213203435597)) ;
#82118=CARTESIAN_POINT('Ctrl Pts',(49.4187257048484,247.02207291095,31.9213203435597)) ;
#82119=CARTESIAN_POINT('Ctrl Pts',(49.4171208221161,247.024338061946,31.9213203435597)) ;
#82120=CARTESIAN_POINT('Ctrl Pts',(49.4155173179349,247.026603020253,31.9213203435597)) ;
#82121=CARTESIAN_POINT('',(49.920223114908,246.597240384684,31.9213203435596)) ;
#82122=CARTESIAN_POINT('Ctrl Pts',(49.4155173179349,247.026603020253,31.9213203435597)) ;
#82123=CARTESIAN_POINT('Ctrl Pts',(49.4171208221161,247.024338061946,31.9213203435597)) ;
#82124=CARTESIAN_POINT('Ctrl Pts',(49.4187257048484,247.02207291095,31.9213203435597)) ;
#82125=CARTESIAN_POINT('Ctrl Pts',(49.4844674063744,246.929105544499,31.9213203435597)) ;
#82126=CARTESIAN_POINT('Ctrl Pts',(49.5501141329755,246.837851580331,31.9213203435597)) ;
#82127=CARTESIAN_POINT('Ctrl Pts',(49.7174613505083,246.697007950007,31.9213203435597)) ;
#82128=CARTESIAN_POINT('Ctrl Pts',(49.8142599722259,246.648887834106,31.9213203435596)) ;
#82129=CARTESIAN_POINT('Ctrl Pts',(49.9136626226905,246.600443322388,31.9213203435597)) ;
#82130=CARTESIAN_POINT('Ctrl Pts',(49.9169428770639,246.598841140054,31.9213203435596)) ;
#82131=CARTESIAN_POINT('Ctrl Pts',(49.920223114908,246.597240384684,31.9213203435596)) ;
#82132=CARTESIAN_POINT('',(49.9630124011287,246.709884790551,31.8013203435596)) ;
#82133=CARTESIAN_POINT('Ctrl Pts',(49.920223114908,246.597240384684,31.9213203435596)) ;
#82134=CARTESIAN_POINT('Ctrl Pts',(49.9203270795018,246.597514062031,31.9213203435596)) ;
#82135=CARTESIAN_POINT('Ctrl Pts',(49.9204310420858,246.597787739813,31.9213192401161)) ;
#82136=CARTESIAN_POINT('Ctrl Pts',(49.9261452162948,246.612830383777,31.9211980829694)) ;
#82137=CARTESIAN_POINT('Ctrl Pts',(49.9317497593604,246.627588945362,31.9178730678895)) ;
#82138=CARTESIAN_POINT('Ctrl Pts',(49.9412579376298,246.652605293149,31.9066209866904)) ;
#82139=CARTESIAN_POINT('Ctrl Pts',(49.9460250235365,246.665143275588,31.8987201940233)) ;
#82140=CARTESIAN_POINT('Ctrl Pts',(49.9542795629539,246.686873772146,31.8753276927662)) ;
#82141=CARTESIAN_POINT('Ctrl Pts',(49.9573645028934,246.695004030452,31.8623344826963)) ;
#82142=CARTESIAN_POINT('Ctrl Pts',(49.9606452939414,246.703653016984,31.8408440931569)) ;
#82143=CARTESIAN_POINT('Ctrl Pts',(49.9615186214591,246.705955875339,31.8331409754495)) ;
#82144=CARTESIAN_POINT('Ctrl Pts',(49.9627008150583,246.70907318093,31.8173971266666)) ;
#82145=CARTESIAN_POINT('Ctrl Pts',(49.9630089487856,246.70988574977,31.8093665682248)) ;
#82146=CARTESIAN_POINT('Ctrl Pts',(49.9630089487856,246.70988574977,31.8013203435596)) ;
#82147=CARTESIAN_POINT('Ctrl Pts',(49.9630121174873,246.709884207708,31.8013203435596)) ;
#82148=CARTESIAN_POINT('Ctrl Pts',(49.8668361976932,246.756688592282,31.8013203435596)) ;
#82149=CARTESIAN_POINT('Ctrl Pts',(49.7804567409035,246.80081723987,31.8013203435596)) ;
#82150=CARTESIAN_POINT('Ctrl Pts',(49.6421982418782,246.917171005845,31.8013203435596)) ;
#82151=CARTESIAN_POINT('Ctrl Pts',(49.582373047438,246.998378778135,31.8013203435596)) ;
#82152=CARTESIAN_POINT('Ctrl Pts',(49.5182656747761,247.089147415072,31.8013203435596)) ;
#82153=CARTESIAN_POINT('Ctrl Pts',(50.776581773269,246.600740334078,31.8013203435596)) ;
#82154=CARTESIAN_POINT('Ctrl Pts',(50.6130596458297,246.602023320729,31.8013203435596)) ;
#82155=CARTESIAN_POINT('Ctrl Pts',(50.4553670282039,246.603946729355,31.8013203435597)) ;
#82156=CARTESIAN_POINT('Ctrl Pts',(50.1936350043753,246.645974976166,31.8013203435596)) ;
#82157=CARTESIAN_POINT('Ctrl Pts',(50.0804419933617,246.677083602446,31.8013203435597)) ;
#82158=CARTESIAN_POINT('Ctrl Pts',(49.9595007821451,246.710865673262,31.8013203435596)) ;
#82159=CARTESIAN_POINT('Ctrl Pts',(49.9559857966182,246.711845543641,31.8013203435596)) ;
#82160=CARTESIAN_POINT('Ctrl Pts',(49.9524714701496,246.712826039435,31.8013203435596)) ;
#82161=CARTESIAN_POINT('Ctrl Pts',(50.776581773269,246.600740334078,31.8372242596007)) ;
#82162=CARTESIAN_POINT('Ctrl Pts',(50.6130596458297,246.602023320729,31.8372242596007)) ;
#82163=CARTESIAN_POINT('Ctrl Pts',(50.4553670282039,246.603946729355,31.8372242596007)) ;
#82164=CARTESIAN_POINT('Ctrl Pts',(50.1936350043753,246.645974976166,31.8372242596007)) ;
#82165=CARTESIAN_POINT('Ctrl Pts',(50.0804419933617,246.677083602446,31.8372242596007)) ;
#82166=CARTESIAN_POINT('Ctrl Pts',(49.9595007821451,246.710865673262,31.8372242596007)) ;
#82167=CARTESIAN_POINT('Ctrl Pts',(49.9559857966182,246.711845543641,31.8372242596007)) ;
#82168=CARTESIAN_POINT('Ctrl Pts',(49.9524714701496,246.712826039435,31.8372242596007)) ;
#82169=CARTESIAN_POINT('Ctrl Pts',(50.77634515619,246.570582476921,31.8993563978491)) ;
#82170=CARTESIAN_POINT('Ctrl Pts',(50.6128091505364,246.571822761431,31.8993563978491)) ;
#82171=CARTESIAN_POINT('Ctrl Pts',(50.4535114513267,246.573692836958,31.8993563978491)) ;
#82172=CARTESIAN_POINT('Ctrl Pts',(50.1866740839135,246.616546092373,31.8993563978491)) ;
#82173=CARTESIAN_POINT('Ctrl Pts',(50.0723303628448,246.648016517864,31.8993563978492)) ;
#82174=CARTESIAN_POINT('Ctrl Pts',(49.951396476224,246.681817835341,31.8993563978491)) ;
#82175=CARTESIAN_POINT('Ctrl Pts',(49.9478805798078,246.682794550961,31.8993563978491)) ;
#82176=CARTESIAN_POINT('Ctrl Pts',(49.9443667099431,246.683776681474,31.8993563978491)) ;
#82177=CARTESIAN_POINT('Ctrl Pts',(50.7758515568694,246.507671135686,31.9213203435597)) ;
#82178=CARTESIAN_POINT('Ctrl Pts',(50.6123212405251,246.508928925739,31.9213203435597)) ;
#82179=CARTESIAN_POINT('Ctrl Pts',(50.449664371721,246.510603924041,31.9213203435597)) ;
#82180=CARTESIAN_POINT('Ctrl Pts',(50.1721428735797,246.555157055951,31.9213203435597)) ;
#82181=CARTESIAN_POINT('Ctrl Pts',(50.0554285869099,246.587437349141,31.9213203435597)) ;
#82182=CARTESIAN_POINT('Ctrl Pts',(49.9344891569417,246.621218012807,31.9213203435596)) ;
#82183=CARTESIAN_POINT('Ctrl Pts',(49.9309736859494,246.62219628459,31.9213203435596)) ;
#82184=CARTESIAN_POINT('Ctrl Pts',(49.927459628902,246.623177744958,31.9213203435596)) ;
#82185=CARTESIAN_POINT('Ctrl Pts',(50.7756402880891,246.480744027444,31.9213203435597)) ;
#82186=CARTESIAN_POINT('Ctrl Pts',(50.6121181606498,246.482027014095,31.9213203435597)) ;
#82187=CARTESIAN_POINT('Ctrl Pts',(50.4480217070699,246.483604593335,31.9213203435597)) ;
#82188=CARTESIAN_POINT('Ctrl Pts',(50.1659215683921,246.52888178823,31.9213203435597)) ;
#82189=CARTESIAN_POINT('Ctrl Pts',(50.0481976053291,246.561517875523,31.9213203435597)) ;
#82190=CARTESIAN_POINT('Ctrl Pts',(49.9272523439948,246.595279599443,31.9213203435596)) ;
#82191=CARTESIAN_POINT('Ctrl Pts',(49.9237374413766,246.59625988889,31.9213203435596)) ;
#82192=CARTESIAN_POINT('Ctrl Pts',(49.920223114908,246.597240384684,31.9213203435596)) ;
#82193=CARTESIAN_POINT('',(50.77564028487,246.480744027482,31.9213203435597)) ;
#82194=CARTESIAN_POINT('Ctrl Pts',(49.920223114908,246.597240384684,31.9213203435596)) ;
#82195=CARTESIAN_POINT('Ctrl Pts',(49.9237374413766,246.59625988889,31.9213203435596)) ;
#82196=CARTESIAN_POINT('Ctrl Pts',(49.9272523439948,246.595279599443,31.9213203435596)) ;
#82197=CARTESIAN_POINT('Ctrl Pts',(50.0481976053291,246.561517875523,31.9213203435597)) ;
#82198=CARTESIAN_POINT('Ctrl Pts',(50.1659215683921,246.52888178823,31.9213203435597)) ;
#82199=CARTESIAN_POINT('Ctrl Pts',(50.4480217070699,246.483604593335,31.9213203435597)) ;
#82200=CARTESIAN_POINT('Ctrl Pts',(50.6121181606498,246.482027014095,31.9213203435597)) ;
#82201=CARTESIAN_POINT('Ctrl Pts',(50.7756402880891,246.480744027444,31.9213203435597)) ;
#82202=CARTESIAN_POINT('',(50.7761110356061,246.600744027949,31.8013203435596)) ;
#82203=CARTESIAN_POINT('Ctrl Pts',(50.7756402808459,246.480744027501,31.9213203435597)) ;
#82204=CARTESIAN_POINT('Ctrl Pts',(50.7756414249247,246.481035667445,31.9213203435597)) ;
#82205=CARTESIAN_POINT('Ctrl Pts',(50.7756425689877,246.481327310518,31.9213192394314)) ;
#82206=CARTESIAN_POINT('Ctrl Pts',(50.7756793939496,246.490714130495,31.9212482468609)) ;
#82207=CARTESIAN_POINT('Ctrl Pts',(50.7757148772581,246.499754942601,31.9201131493261)) ;
#82208=CARTESIAN_POINT('Ctrl Pts',(50.7757752384286,246.515127192197,31.9164226980159)) ;
#82209=CARTESIAN_POINT('Ctrl Pts',(50.7758005091845,246.521560106118,31.9143041430243)) ;
#82210=CARTESIAN_POINT('Ctrl Pts',(50.7758578779052,246.536167028899,31.90810382497)) ;
#82211=CARTESIAN_POINT('Ctrl Pts',(50.7758889840361,246.544088046079,31.903638902298)) ;
#82212=CARTESIAN_POINT('Ctrl Pts',(50.7759230860527,246.552806936408,31.8972878004598)) ;
#82213=CARTESIAN_POINT('Ctrl Pts',(50.7759285564978,246.554206855326,31.8962181513507)) ;
#82214=CARTESIAN_POINT('Ctrl Pts',(50.7759483201422,246.559270573818,31.8921590556894)) ;
#82215=CARTESIAN_POINT('Ctrl Pts',(50.7759619611503,246.562777498341,31.8889698646365)) ;
#82216=CARTESIAN_POINT('Ctrl Pts',(50.7759995646949,246.57245412009,31.8790406793499)) ;
#82217=CARTESIAN_POINT('Ctrl Pts',(50.7760212186874,246.578035503319,31.871809093448)) ;
#82218=CARTESIAN_POINT('Ctrl Pts',(50.77605281931,246.586134096496,31.8585433129843)) ;
#82219=CARTESIAN_POINT('Ctrl Pts',(50.7760643339462,246.589069672085,31.8527726268368)) ;
#82220=CARTESIAN_POINT('Ctrl Pts',(50.7760878139232,246.595013606618,31.8384079767118)) ;
#82221=CARTESIAN_POINT('Ctrl Pts',(50.7760979872128,246.597546326518,31.8296999420229)) ;
#82222=CARTESIAN_POINT('Ctrl Pts',(50.7761086558584,246.600170884711,31.8143916078104)) ;
#82223=CARTESIAN_POINT('Ctrl Pts',(50.776111046444,246.600744029292,31.8078756404829)) ;
#82224=CARTESIAN_POINT('Ctrl Pts',(50.776111046444,246.600744029292,31.8013203435596)) ;
#82225=CARTESIAN_POINT('Ctrl Pts',(50.7761110306795,246.600744027501,31.8013203435596)) ;
#82226=CARTESIAN_POINT('Ctrl Pts',(50.7318115553004,246.601091599028,31.8013203435596)) ;
#82227=CARTESIAN_POINT('Ctrl Pts',(50.6879330968571,246.601440518035,31.8013203435596)) ;
#82228=CARTESIAN_POINT('Ctrl Pts',(50.6445235118033,246.602281618153,31.8013203435596)) ;
#82229=CARTESIAN_POINT('Ctrl Pts',(50.5998048884608,246.603148082076,31.8013203435596)) ;
#82230=CARTESIAN_POINT('Ctrl Pts',(50.5555837981124,246.604536553163,31.8013203435596)) ;
#82231=CARTESIAN_POINT('Ctrl Pts',(50.5119042411479,246.606927166115,31.8013203435597)) ;
#82232=CARTESIAN_POINT('Ctrl Pts',(50.4659508748484,246.609442226255,31.8013203435597)) ;
#82233=CARTESIAN_POINT('Ctrl Pts',(50.4205968622638,246.613066290501,31.8013203435597)) ;
#82234=CARTESIAN_POINT('Ctrl Pts',(50.3758849022658,246.618300500973,31.8013203435597)) ;
#82235=CARTESIAN_POINT('Ctrl Pts',(50.3522226439638,246.621070525821,31.8013203435597)) ;
#82236=CARTESIAN_POINT('Ctrl Pts',(50.3287400670188,246.624290568393,31.8013203435597)) ;
#82237=CARTESIAN_POINT('Ctrl Pts',(50.3054426551874,246.628029171234,31.8013203435596)) ;
#82238=CARTESIAN_POINT('Ctrl Pts',(50.300772904059,246.62877853966,31.8013203435596)) ;
#82239=CARTESIAN_POINT('Ctrl Pts',(50.296100662629,246.629550323865,31.8013203435596)) ;
#82240=CARTESIAN_POINT('Ctrl Pts',(50.2914257404912,246.630343819124,31.8013203435596)) ;
#82241=CARTESIAN_POINT('Ctrl Pts',(50.2534216693473,246.636794418593,31.8013203435596)) ;
#82242=CARTESIAN_POINT('Ctrl Pts',(50.2152410381834,246.644683702373,31.8013203435596)) ;
#82243=CARTESIAN_POINT('Ctrl Pts',(50.1767784263017,246.653607486108,31.8013203435596)) ;
#82244=CARTESIAN_POINT('Ctrl Pts',(50.1411378791258,246.661876517243,31.8013203435596)) ;
#82245=CARTESIAN_POINT('Ctrl Pts',(50.1052552397161,246.671033999744,31.8013203435597)) ;
#82246=CARTESIAN_POINT('Ctrl Pts',(50.06904036106,246.680715789108,31.8013203435596)) ;
#82247=CARTESIAN_POINT('Ctrl Pts',(50.0340380172689,246.690073415929,31.8013203435596)) ;
#82248=CARTESIAN_POINT('Ctrl Pts',(49.9987253672562,246.699921219123,31.8013203435596)) ;
#82249=CARTESIAN_POINT('Ctrl Pts',(49.963014268976,246.709884602433,31.8013203435596)) ;
#82250=CARTESIAN_POINT('Origin',(51.9003128398474,244.103994673298,31.8013203435596)) ;
#82251=CARTESIAN_POINT('',(52.0203128398474,250.600744087106,31.8013203435596)) ;
#82252=CARTESIAN_POINT('',(52.0203128398474,244.103994673298,31.8013203435596)) ;
#82253=CARTESIAN_POINT('',(51.9003128398474,250.720744087106,31.9213203435596)) ;
#82254=CARTESIAN_POINT('Origin',(51.9003128398474,250.720744087106,31.8013203435596)) ;
#82255=CARTESIAN_POINT('',(51.9003128398474,248.944482161408,31.9213203435596)) ;
#82256=CARTESIAN_POINT('',(51.9003128398474,244.103994673298,31.9213203435596)) ;
#82257=CARTESIAN_POINT('Origin',(51.9003128398474,248.944482161408,31.8013203435596)) ;
#82258=CARTESIAN_POINT('Origin',(53.1248221837489,246.480744027501,31.8013203435596)) ;
#82259=CARTESIAN_POINT('',(52.6696443674977,246.480744027501,31.9213203435596)) ;
#82260=CARTESIAN_POINT('',(53.1248221837489,246.480744027501,31.9213203435596)) ;
#82261=CARTESIAN_POINT('',(52.5496443674977,246.600744027501,31.8013203435596)) ;
#82262=CARTESIAN_POINT('Origin',(52.6696443674977,246.480744027501,31.8013203435596)) ;
#82263=CARTESIAN_POINT('',(53.1248221837489,246.600744027501,31.8013203435596)) ;
#82264=CARTESIAN_POINT('Origin',(52.6696443674977,244.992125636147,31.8013203435596)) ;
#82265=CARTESIAN_POINT('',(52.6696443674977,250.720744087106,31.9213203435596)) ;
#82266=CARTESIAN_POINT('',(52.6696443674977,244.992125636147,31.9213203435596)) ;
#82267=CARTESIAN_POINT('',(52.5496443674977,250.600744087106,31.8013203435596)) ;
#82268=CARTESIAN_POINT('Origin',(52.6696443674977,250.720744087106,31.8013203435596)) ;
#82269=CARTESIAN_POINT('',(52.5496443674977,244.992125636147,31.8013203435596)) ;
#82270=CARTESIAN_POINT('Origin',(52.8601564199237,250.720744087106,31.8013203435596)) ;
#82271=CARTESIAN_POINT('',(52.8601564199237,250.600744087106,31.8013203435596)) ;
#82272=CARTESIAN_POINT('',(52.8601564199237,250.720744087106,31.9213203435596)) ;
#82273=CARTESIAN_POINT('Ctrl Pts',(51.1117181123309,248.84358187378,31.8013203435596)) ;
#82274=CARTESIAN_POINT('Ctrl Pts',(51.1489587152535,248.838376895812,31.8013203435596)) ;
#82275=CARTESIAN_POINT('Ctrl Pts',(51.1881361258901,248.832747914847,31.8013203435596)) ;
#82276=CARTESIAN_POINT('Ctrl Pts',(51.2926832236002,248.824119255618,31.8013203435596)) ;
#82277=CARTESIAN_POINT('Ctrl Pts',(51.3510329785516,248.824455497164,31.8013203435596)) ;
#82278=CARTESIAN_POINT('Ctrl Pts',(51.4064264123703,248.824482175325,31.8013203435596)) ;
#82279=CARTESIAN_POINT('Ctrl Pts',(51.1117181123309,248.84358187378,31.8372242596007)) ;
#82280=CARTESIAN_POINT('Ctrl Pts',(51.1489587152535,248.838376895812,31.8372242596006)) ;
#82281=CARTESIAN_POINT('Ctrl Pts',(51.1881361258901,248.832747914847,31.8372242596007)) ;
#82282=CARTESIAN_POINT('Ctrl Pts',(51.2926832236002,248.824119255618,31.8372242596007)) ;
#82283=CARTESIAN_POINT('Ctrl Pts',(51.3510329785516,248.824455497164,31.8372242596007)) ;
#82284=CARTESIAN_POINT('Ctrl Pts',(51.4064264123703,248.824482175325,31.8372242596007)) ;
#82285=CARTESIAN_POINT('Ctrl Pts',(51.1158927186706,248.873450368516,31.8993563584643)) ;
#82286=CARTESIAN_POINT('Ctrl Pts',(51.1531387365592,248.86825773829,31.8993563584643)) ;
#82287=CARTESIAN_POINT('Ctrl Pts',(51.191825566714,248.862704407547,31.8993563584643)) ;
#82288=CARTESIAN_POINT('Ctrl Pts',(51.2933967401955,248.854327364572,31.8993563584643)) ;
#82289=CARTESIAN_POINT('Ctrl Pts',(51.3510153287493,248.854633525484,31.8993563584643)) ;
#82290=CARTESIAN_POINT('Ctrl Pts',(51.4064118875128,248.854640990038,31.8993563584643)) ;
#82291=CARTESIAN_POINT('Ctrl Pts',(51.1246012174117,248.935757979734,31.9213203435596)) ;
#82292=CARTESIAN_POINT('Ctrl Pts',(51.1618450140909,248.930560284486,31.9213203435596)) ;
#82293=CARTESIAN_POINT('Ctrl Pts',(51.1995213578042,248.925197579428,31.9213203435596)) ;
#82294=CARTESIAN_POINT('Ctrl Pts',(51.294882734956,248.917325960997,31.9213203435596)) ;
#82295=CARTESIAN_POINT('Ctrl Pts',(51.3509863108044,248.917538881559,31.9213203435596)) ;
#82296=CARTESIAN_POINT('Ctrl Pts',(51.4063815877211,248.917554227501,31.9213203435596)) ;
#82297=CARTESIAN_POINT('Ctrl Pts',(51.1283286027442,248.962426695326,31.9213203435596)) ;
#82298=CARTESIAN_POINT('Ctrl Pts',(51.1655692056668,248.957221717357,31.9213203435596)) ;
#82299=CARTESIAN_POINT('Ctrl Pts',(51.2028151840149,248.951946048557,31.9213203435596)) ;
#82300=CARTESIAN_POINT('Ctrl Pts',(51.2955183598921,248.944287530684,31.9213203435596)) ;
#82301=CARTESIAN_POINT('Ctrl Pts',(51.3509751850771,248.944455483247,31.9213203435596)) ;
#82302=CARTESIAN_POINT('Ctrl Pts',(51.4063686188957,248.944482161408,31.9213203435596)) ;
#82303=CARTESIAN_POINT('',(51.4063686188957,248.944482161408,31.9213203435596)) ;
#82304=CARTESIAN_POINT('Origin',(51.4063542356917,248.944482151675,31.80132034635)) ;
#82305=CARTESIAN_POINT('',(51.1372712358084,248.961175922748,31.9213203435596)) ;
#82306=CARTESIAN_POINT('Ctrl Pts',(51.4063686188957,248.944482161408,31.9213203435596)) ;
#82307=CARTESIAN_POINT('Ctrl Pts',(51.3509751850771,248.944455483247,31.9213203435596)) ;
#82308=CARTESIAN_POINT('Ctrl Pts',(51.2955183598921,248.944287530684,31.9213203435596)) ;
#82309=CARTESIAN_POINT('Ctrl Pts',(51.2058202898626,248.951697786762,31.9213203435596)) ;
#82310=CARTESIAN_POINT('Ctrl Pts',(51.1715427561408,248.956389821489,31.9213203435596)) ;
#82311=CARTESIAN_POINT('Ctrl Pts',(51.1372855628255,248.961174642356,31.9213203435596)) ;
#82312=CARTESIAN_POINT('Ctrl Pts',(51.137257201749,248.961178603667,31.9213203435596)) ;
#82313=CARTESIAN_POINT('Ctrl Pts',(51.1371956772459,248.960893312062,31.9213203435596)) ;
#82314=CARTESIAN_POINT('Ctrl Pts',(51.1371341474076,248.960608021905,31.9213192437131)) ;
#82315=CARTESIAN_POINT('Ctrl Pts',(51.1337432017254,248.944886937038,31.9211981723136)) ;
#82316=CARTESIAN_POINT('Ctrl Pts',(51.130400973083,248.929466879524,31.9178672689546)) ;
#82317=CARTESIAN_POINT('Ctrl Pts',(51.1247267558731,248.903341551515,31.9066018385777)) ;
#82318=CARTESIAN_POINT('Ctrl Pts',(51.1218791521258,248.890256390852,31.8986969526448)) ;
#82319=CARTESIAN_POINT('Ctrl Pts',(51.1169394944018,248.867572728553,31.8752907032164)) ;
#82320=CARTESIAN_POINT('Ctrl Pts',(51.1150914688031,248.859087608765,31.8622865674932)) ;
#82321=CARTESIAN_POINT('Ctrl Pts',(51.1131294333774,248.85007188772,31.8407965086607)) ;
#82322=CARTESIAN_POINT('Ctrl Pts',(51.1126079113899,248.847674181376,31.8331028074907)) ;
#82323=CARTESIAN_POINT('Ctrl Pts',(51.1119020158497,248.844428030261,31.8173781185803)) ;
#82324=CARTESIAN_POINT('Ctrl Pts',(51.1117181123326,248.84358187378,31.8093569350819)) ;
#82325=CARTESIAN_POINT('Ctrl Pts',(51.1117181123326,248.84358187378,31.8013203435596)) ;
#82326=CARTESIAN_POINT('Origin',(52.5531987578181,248.944482161408,31.8013203435596)) ;
#82327=CARTESIAN_POINT('',(52.5531987578181,248.944482161408,31.9213203435596)) ;
#82328=CARTESIAN_POINT('Ctrl Pts',(50.8716089964921,248.949993748075,31.8013203435596)) ;
#82329=CARTESIAN_POINT('Ctrl Pts',(50.9057808422561,248.929376866944,31.8013203435596)) ;
#82330=CARTESIAN_POINT('Ctrl Pts',(50.9426967052446,248.906058928819,31.8013203435596)) ;
#82331=CARTESIAN_POINT('Ctrl Pts',(51.0354893826749,248.865415252228,31.8013203435596)) ;
#82332=CARTESIAN_POINT('Ctrl Pts',(51.0754146033954,248.854384493201,31.8013203435596)) ;
#82333=CARTESIAN_POINT('Ctrl Pts',(51.1117181123318,248.84358187378,31.8013203435596)) ;
#82334=CARTESIAN_POINT('Ctrl Pts',(50.8716089964921,248.949993748075,31.8372242596007)) ;
#82335=CARTESIAN_POINT('Ctrl Pts',(50.9057808422561,248.929376866944,31.8372242596006)) ;
#82336=CARTESIAN_POINT('Ctrl Pts',(50.9426967052446,248.906058928819,31.8372242596006)) ;
#82337=CARTESIAN_POINT('Ctrl Pts',(51.0354893826749,248.865415252228,31.8372242596006)) ;
#82338=CARTESIAN_POINT('Ctrl Pts',(51.0754146033954,248.854384493201,31.8372242596007)) ;
#82339=CARTESIAN_POINT('Ctrl Pts',(51.1117181123318,248.84358187378,31.8372242596007)) ;
#82340=CARTESIAN_POINT('Ctrl Pts',(50.8871887506966,248.975816711032,31.8993563616251)) ;
#82341=CARTESIAN_POINT('Ctrl Pts',(50.9214287856237,248.95524472293,31.8993563616251)) ;
#82342=CARTESIAN_POINT('Ctrl Pts',(50.9575760093834,248.932477758779,31.8993563616251)) ;
#82343=CARTESIAN_POINT('Ctrl Pts',(51.0449515126423,248.894201916256,31.8993563616251)) ;
#82344=CARTESIAN_POINT('Ctrl Pts',(51.0840029923614,248.883367857674,31.8993563616251)) ;
#82345=CARTESIAN_POINT('Ctrl Pts',(51.1203195626634,248.872488087803,31.8993563616251)) ;
#82346=CARTESIAN_POINT('Ctrl Pts',(50.9196891295034,249.02968508835,31.9213203435596)) ;
#82347=CARTESIAN_POINT('Ctrl Pts',(50.95390119474,249.009094686119,31.9213203435596)) ;
#82348=CARTESIAN_POINT('Ctrl Pts',(50.9885819797057,248.987566509174,31.9213203435596)) ;
#82349=CARTESIAN_POINT('Ctrl Pts',(51.0647020317792,248.954225167441,31.9213203435596)) ;
#82350=CARTESIAN_POINT('Ctrl Pts',(51.1019515336979,248.943636451488,31.9213203435596)) ;
#82351=CARTESIAN_POINT('Ctrl Pts',(51.1382627465158,248.93278832703,31.9213203435596)) ;
#82352=CARTESIAN_POINT('Ctrl Pts',(50.9335998429103,249.052741667569,31.9213203435596)) ;
#82353=CARTESIAN_POINT('Ctrl Pts',(50.9677716886743,249.032124786438,31.9213203435596)) ;
#82354=CARTESIAN_POINT('Ctrl Pts',(51.0018475472828,249.0111416709,31.9213203435596)) ;
#82355=CARTESIAN_POINT('Ctrl Pts',(51.0731575641017,248.97991155694,31.9213203435596)) ;
#82356=CARTESIAN_POINT('Ctrl Pts',(51.109639224624,248.969400471664,31.9213203435596)) ;
#82357=CARTESIAN_POINT('Ctrl Pts',(51.1459427335603,248.958597852243,31.9213203435596)) ;
#82358=CARTESIAN_POINT('',(50.9393246912647,249.049285590905,31.9213203435556)) ;
#82359=CARTESIAN_POINT('Ctrl Pts',(51.1372708297894,248.961174555801,31.9213203435596)) ;
#82360=CARTESIAN_POINT('Ctrl Pts',(51.1038423419625,248.97110363352,31.9213203435596)) ;
#82361=CARTESIAN_POINT('Ctrl Pts',(51.0703935287813,248.981122062026,31.9213203435596)) ;
#82362=CARTESIAN_POINT('Ctrl Pts',(51.0038907454527,249.010246855353,31.9213203435596)) ;
#82363=CARTESIAN_POINT('Ctrl Pts',(50.9715854655917,249.02979664263,31.9213203435596)) ;
#82364=CARTESIAN_POINT('Ctrl Pts',(50.9393243991729,249.049285107378,31.9213203435596)) ;
#82365=CARTESIAN_POINT('Ctrl Pts',(50.9393250687946,249.049284702869,31.9213203435485)) ;
#82366=CARTESIAN_POINT('Ctrl Pts',(50.9391605620508,249.049043427891,31.9213203395065)) ;
#82367=CARTESIAN_POINT('Ctrl Pts',(50.9389960528488,249.048802149732,31.9213192316299)) ;
#82368=CARTESIAN_POINT('Ctrl Pts',(50.9388315444401,249.048560873149,31.9213170224859)) ;
#82369=CARTESIAN_POINT('Ctrl Pts',(50.9337013545053,249.041036669922,31.9212481303927)) ;
#82370=CARTESIAN_POINT('Ctrl Pts',(50.928600939845,249.033556486928,31.9201132752162)) ;
#82371=CARTESIAN_POINT('Ctrl Pts',(50.9236275213475,249.02626262057,31.9179971542262)) ;
#82372=CARTESIAN_POINT('Ctrl Pts',(50.9199052479004,249.020803646007,31.9164133782025)) ;
#82373=CARTESIAN_POINT('Ctrl Pts',(50.9162538645725,249.015448621153,31.9142786664762)) ;
#82374=CARTESIAN_POINT('Ctrl Pts',(50.9127164446231,249.010261058044,31.9116100684325)) ;
#82375=CARTESIAN_POINT('Ctrl Pts',(50.9079966071706,249.003339500807,31.9080494651758)) ;
#82376=CARTESIAN_POINT('Ctrl Pts',(50.9035313617411,248.996791787699,31.9035793945282)) ;
#82377=CARTESIAN_POINT('Ctrl Pts',(50.8994175635233,248.990762394863,31.898260203771)) ;
#82378=CARTESIAN_POINT('Ctrl Pts',(50.8986312567895,248.989609943543,31.8972434996719)) ;
#82379=CARTESIAN_POINT('Ctrl Pts',(50.8978578245792,248.988476487402,31.8961956369672)) ;
#82380=CARTESIAN_POINT('Ctrl Pts',(50.8970980036519,248.987363137245,31.8951168504373)) ;
#82381=CARTESIAN_POINT('Ctrl Pts',(50.8949972230907,248.984284906199,31.8921341821659)) ;
#82382=CARTESIAN_POINT('Ctrl Pts',(50.8930003769272,248.98136017739,31.8889152931147)) ;
#82383=CARTESIAN_POINT('Ctrl Pts',(50.8911145493636,248.978598394777,31.8854819951251)) ;
#82384=CARTESIAN_POINT('Ctrl Pts',(50.8875237702891,248.973339721393,31.8789446982823)) ;
#82385=CARTESIAN_POINT('Ctrl Pts',(50.8843740883763,248.968727964332,31.8717049222366)) ;
#82386=CARTESIAN_POINT('Ctrl Pts',(50.8817015988867,248.964812183075,31.8639327628133)) ;
#82387=CARTESIAN_POINT('Ctrl Pts',(50.8798143452646,248.962046944002,31.8584442338293)) ;
#82388=CARTESIAN_POINT('Ctrl Pts',(50.8781653794535,248.959629320532,31.852689084534)) ;
#82389=CARTESIAN_POINT('Ctrl Pts',(50.8767742851082,248.95758806856,31.8467190011286)) ;
#82390=CARTESIAN_POINT('Ctrl Pts',(50.8748228640619,248.954724609246,31.8383441943121)) ;
#82391=CARTESIAN_POINT('Ctrl Pts',(50.8733995571067,248.952631836735,31.8296398838193)) ;
#82392=CARTESIAN_POINT('Ctrl Pts',(50.8725450425081,248.95137357103,31.8207573318203)) ;
#82393=CARTESIAN_POINT('Ctrl Pts',(50.8719290057467,248.950466461975,31.8143537214259)) ;
#82394=CARTESIAN_POINT('Ctrl Pts',(50.8716089964922,248.949993748075,31.8078567218145)) ;
#82395=CARTESIAN_POINT('Ctrl Pts',(50.8716089964922,248.949993748075,31.8013203435596)) ;
#82396=CARTESIAN_POINT('Ctrl Pts',(50.6014861107882,249.217388231164,31.8013203435596)) ;
#82397=CARTESIAN_POINT('Ctrl Pts',(50.6431307164356,249.165394145294,31.8013203435596)) ;
#82398=CARTESIAN_POINT('Ctrl Pts',(50.6869793943593,249.109198386675,31.8013203435596)) ;
#82399=CARTESIAN_POINT('Ctrl Pts',(50.7876909072677,249.01365071099,31.8013203435596)) ;
#82400=CARTESIAN_POINT('Ctrl Pts',(50.8311952099577,248.980988011817,31.8013203435596)) ;
#82401=CARTESIAN_POINT('Ctrl Pts',(50.8716089964922,248.949993748075,31.8013203435596)) ;
#82402=CARTESIAN_POINT('Ctrl Pts',(50.6014861107882,249.217388231164,31.8372242596007)) ;
#82403=CARTESIAN_POINT('Ctrl Pts',(50.6431307164356,249.165394145294,31.8372242596006)) ;
#82404=CARTESIAN_POINT('Ctrl Pts',(50.6869793943593,249.109198386675,31.8372242596007)) ;
#82405=CARTESIAN_POINT('Ctrl Pts',(50.7876909072677,249.01365071099,31.8372242596007)) ;
#82406=CARTESIAN_POINT('Ctrl Pts',(50.8311952099577,248.980988011817,31.8372242596007)) ;
#82407=CARTESIAN_POINT('Ctrl Pts',(50.8716089964922,248.949993748075,31.8372242596007)) ;
#82408=CARTESIAN_POINT('Ctrl Pts',(50.6250252885878,249.236241909622,31.8993563630984)) ;
#82409=CARTESIAN_POINT('Ctrl Pts',(50.6667241194215,249.184277969696,31.8993563630984)) ;
#82410=CARTESIAN_POINT('Ctrl Pts',(50.7099286886098,249.129019052297,31.8993563630984)) ;
#82411=CARTESIAN_POINT('Ctrl Pts',(50.8067675034066,249.037124248324,31.8993563630984)) ;
#82412=CARTESIAN_POINT('Ctrl Pts',(50.8495672969953,249.004964549531,31.8993563630984)) ;
#82413=CARTESIAN_POINT('Ctrl Pts',(50.8899624342195,248.97392501228,31.8993563630984)) ;
#82414=CARTESIAN_POINT('Ctrl Pts',(50.6741295447479,249.275571909355,31.9213203435596)) ;
#82415=CARTESIAN_POINT('Ctrl Pts',(50.7158061341191,249.223595604513,31.9213203435596)) ;
#82416=CARTESIAN_POINT('Ctrl Pts',(50.7577733526272,249.170327174966,31.9213203435596)) ;
#82417=CARTESIAN_POINT('Ctrl Pts',(50.8465626123779,249.086092192121,31.9213203435596)) ;
#82418=CARTESIAN_POINT('Ctrl Pts',(50.8878461126627,249.054868153674,31.9213203435596)) ;
#82419=CARTESIAN_POINT('Ctrl Pts',(50.9282488992462,249.023847186189,31.9213203435596)) ;
#82420=CARTESIAN_POINT('Ctrl Pts',(50.69514699889,249.292405816036,31.9213203435596)) ;
#82421=CARTESIAN_POINT('Ctrl Pts',(50.7367916045374,249.240411730166,31.9213203435596)) ;
#82422=CARTESIAN_POINT('Ctrl Pts',(50.7782468577583,249.18800126692,31.9213203435596)) ;
#82423=CARTESIAN_POINT('Ctrl Pts',(50.8635956083774,249.107051404809,31.9213203435596)) ;
#82424=CARTESIAN_POINT('Ctrl Pts',(50.9042223688458,249.076208986737,31.9213203435596)) ;
#82425=CARTESIAN_POINT('Ctrl Pts',(50.9446361553801,249.045214722995,31.9213203435596)) ;
#82426=CARTESIAN_POINT('',(50.6964442987387,249.290785955645,31.9213203435596)) ;
#82427=CARTESIAN_POINT('Ctrl Pts',(50.939324907591,249.049286844368,31.9213203435596)) ;
#82428=CARTESIAN_POINT('Ctrl Pts',(50.9006704775887,249.078918887735,31.9213203435596)) ;
#82429=CARTESIAN_POINT('Ctrl Pts',(50.8619758937283,249.108587639102,31.9213203435596)) ;
#82430=CARTESIAN_POINT('Ctrl Pts',(50.7787491279644,249.187524883802,31.9213203435596)) ;
#82431=CARTESIAN_POINT('Ctrl Pts',(50.7376533076475,249.239323955441,31.9213203435596)) ;
#82432=CARTESIAN_POINT('Ctrl Pts',(50.6964442808212,249.290785941297,31.9213203435596)) ;
#82433=CARTESIAN_POINT('Ctrl Pts',(50.6964442909169,249.290785882339,31.9213203435596)) ;
#82434=CARTESIAN_POINT('Ctrl Pts',(50.6962133562336,249.290607729158,31.9213203434865)) ;
#82435=CARTESIAN_POINT('Ctrl Pts',(50.69598224445,249.290429791841,31.9213192393805)) ;
#82436=CARTESIAN_POINT('Ctrl Pts',(50.6957514762923,249.290251414378,31.9213170336782)) ;
#82437=CARTESIAN_POINT('Ctrl Pts',(50.6885546406468,249.284688457595,31.9212482456927)) ;
#82438=CARTESIAN_POINT('Ctrl Pts',(50.6814006814086,249.27915858507,31.9201131362439)) ;
#82439=CARTESIAN_POINT('Ctrl Pts',(50.6744256288717,249.273766936644,31.9179969379934)) ;
#82440=CARTESIAN_POINT('Ctrl Pts',(50.6692337901446,249.269753695316,31.9164217584556)) ;
#82441=CARTESIAN_POINT('Ctrl Pts',(50.6641407016877,249.265816738188,31.914301727067)) ;
#82442=CARTESIAN_POINT('Ctrl Pts',(50.6592058288327,249.262002122443,31.9116538260208)) ;
#82443=CARTESIAN_POINT('Ctrl Pts',(50.6525801029015,249.256880491309,31.9080986652011)) ;
#82444=CARTESIAN_POINT('Ctrl Pts',(50.6463125394723,249.25203575774,31.9036331060502)) ;
#82445=CARTESIAN_POINT('Ctrl Pts',(50.6405399600747,249.247574290001,31.8983184908323)) ;
#82446=CARTESIAN_POINT('Ctrl Pts',(50.6394156172124,249.246705316348,31.8972833470474)) ;
#82447=CARTESIAN_POINT('Ctrl Pts',(50.6383101062439,249.245850925699,31.896215850627)) ;
#82448=CARTESIAN_POINT('Ctrl Pts',(50.6372245343117,249.2450119811,31.895116256076)) ;
#82449=CARTESIAN_POINT('Ctrl Pts',(50.6343027290264,249.242753970654,31.8921567090614)) ;
#82450=CARTESIAN_POINT('Ctrl Pts',(50.6315251916768,249.240607714716,31.8889648053869)) ;
#82451=CARTESIAN_POINT('Ctrl Pts',(50.6289010358486,249.238580050955,31.8855618965884)) ;
#82452=CARTESIAN_POINT('Ctrl Pts',(50.6238651781714,249.234688884888,31.8790315815006)) ;
#82453=CARTESIAN_POINT('Ctrl Pts',(50.6194480456435,249.231276008718,31.8717989312328)) ;
#82454=CARTESIAN_POINT('Ctrl Pts',(50.6156976656245,249.228377709018,31.86403439033)) ;
#82455=CARTESIAN_POINT('Ctrl Pts',(50.6130406872218,249.226324391843,31.8585335564466)) ;
#82456=CARTESIAN_POINT('Ctrl Pts',(50.6107188488196,249.224529738816,31.8527646307448)) ;
#82457=CARTESIAN_POINT('Ctrl Pts',(50.6087596898981,249.223015035295,31.8467799131912)) ;
#82458=CARTESIAN_POINT('Ctrl Pts',(50.6060171944983,249.220894703253,31.8384023077914)) ;
#82459=CARTESIAN_POINT('Ctrl Pts',(50.6040141086399,249.219345101931,31.8296947779775)) ;
#82460=CARTESIAN_POINT('Ctrl Pts',(50.6028094856611,249.218412789161,31.8208091193525)) ;
#82461=CARTESIAN_POINT('Ctrl Pts',(50.6019390438936,249.217739114501,31.8143884810815)) ;
#82462=CARTESIAN_POINT('Ctrl Pts',(50.6014861107882,249.217388231164,31.8078740801924)) ;
#82463=CARTESIAN_POINT('Ctrl Pts',(50.6014861107882,249.217388231164,31.8013203435596)) ;
#82464=CARTESIAN_POINT('Ctrl Pts',(50.2194532543318,249.768610947797,31.8013199480773)) ;
#82465=CARTESIAN_POINT('Ctrl Pts',(50.2877998866917,249.663014973847,31.8013199480773)) ;
#82466=CARTESIAN_POINT('Ctrl Pts',(50.3569110677109,249.556127806374,31.8013199480773)) ;
#82467=CARTESIAN_POINT('Ctrl Pts',(50.4869845254701,249.370877841352,31.8013199480774)) ;
#82468=CARTESIAN_POINT('Ctrl Pts',(50.5445853181005,249.293693208364,31.8013199480774)) ;
#82469=CARTESIAN_POINT('Ctrl Pts',(50.6014861107887,249.217388231164,31.8013199480774)) ;
#82470=CARTESIAN_POINT('Ctrl Pts',(50.2194531480909,249.768610879033,31.837223998882)) ;
#82471=CARTESIAN_POINT('Ctrl Pts',(50.2877997804396,249.663014905074,31.837223998882)) ;
#82472=CARTESIAN_POINT('Ctrl Pts',(50.356910962284,249.556127736288,31.837223998882)) ;
#82473=CARTESIAN_POINT('Ctrl Pts',(50.4869844233015,249.37087776663,31.837223998882)) ;
#82474=CARTESIAN_POINT('Ctrl Pts',(50.5445852166412,249.293693132706,31.837223998882)) ;
#82475=CARTESIAN_POINT('Ctrl Pts',(50.6014860093375,249.217388155512,31.837223998882)) ;
#82476=CARTESIAN_POINT('Ctrl Pts',(50.2447714707482,249.784998074696,31.8993564452671)) ;
#82477=CARTESIAN_POINT('Ctrl Pts',(50.3131207689826,249.679404050894,31.8993564452672)) ;
#82478=CARTESIAN_POINT('Ctrl Pts',(50.3820352831163,249.572830004009,31.8993564452671)) ;
#82479=CARTESIAN_POINT('Ctrl Pts',(50.5113322522005,249.388684776835,31.8993564452672)) ;
#82480=CARTESIAN_POINT('Ctrl Pts',(50.5687640133161,249.311723393403,31.8993564452671)) ;
#82481=CARTESIAN_POINT('Ctrl Pts',(50.6256628918907,249.235416911072,31.8993564452672)) ;
#82482=CARTESIAN_POINT('Ctrl Pts',(50.2975873134094,249.819182943984,31.9213204357249)) ;
#82483=CARTESIAN_POINT('Ctrl Pts',(50.3659355722092,249.713588032968,31.9213204357249)) ;
#82484=CARTESIAN_POINT('Ctrl Pts',(50.4344445902855,249.607670461033,31.9213204357248)) ;
#82485=CARTESIAN_POINT('Ctrl Pts',(50.562123374562,249.425831480274,31.9213204357248)) ;
#82486=CARTESIAN_POINT('Ctrl Pts',(50.6191979436028,249.349332056466,31.9213204357248)) ;
#82487=CARTESIAN_POINT('Ctrl Pts',(50.676097607319,249.273026191517,31.9213204357248)) ;
#82488=CARTESIAN_POINT('Ctrl Pts',(50.3201933811436,249.833814642216,31.921320343559)) ;
#82489=CARTESIAN_POINT('Ctrl Pts',(50.3885400996636,249.728218529107,31.921320343559)) ;
#82490=CARTESIAN_POINT('Ctrl Pts',(50.4568763496929,249.622582483817,31.9213203435589)) ;
#82491=CARTESIAN_POINT('Ctrl Pts',(50.5838627947292,249.441730893079,31.9213203435589)) ;
#82492=CARTESIAN_POINT('Ctrl Pts',(50.6407837197257,249.365428572277,31.9213203435589)) ;
#82493=CARTESIAN_POINT('Ctrl Pts',(50.6976845124305,249.28912359509,31.9213203435589)) ;
#82494=CARTESIAN_POINT('Ctrl Pts',(50.6964443401006,249.290786023789,31.9213203435596)) ;
#82495=CARTESIAN_POINT('Ctrl Pts',(50.6399566587065,249.366536825083,31.9213203435596)) ;
#82496=CARTESIAN_POINT('Ctrl Pts',(50.5834651712519,249.442296492374,31.9213203435596)) ;
#82497=CARTESIAN_POINT('Ctrl Pts',(50.4569815065016,249.622432033364,31.9213203435596)) ;
#82498=CARTESIAN_POINT('Ctrl Pts',(50.3887392215019,249.727910011782,31.9213203435597)) ;
#82499=CARTESIAN_POINT('Ctrl Pts',(50.3204922630187,249.833352139651,31.9213203435597)) ;
#82500=CARTESIAN_POINT('Origin',(51.3622028112916,250.720744087106,31.8013203435596)) ;
#82501=CARTESIAN_POINT('',(51.3622028112916,250.720744087106,31.9213203435596)) ;
#82502=CARTESIAN_POINT('Ctrl Pts',(49.3518273473795,247.692149180776,31.9213203435596)) ;
#82503=CARTESIAN_POINT('Ctrl Pts',(49.3518273473795,247.692149180776,31.5613203435596)) ;
#82504=CARTESIAN_POINT('Ctrl Pts',(49.3625435679673,247.827639860195,31.9213203435596)) ;
#82505=CARTESIAN_POINT('Ctrl Pts',(49.3625435679673,247.827639860195,31.5613203435596)) ;
#82506=CARTESIAN_POINT('Ctrl Pts',(49.3836326934911,248.094280502961,31.9213203435596)) ;
#82507=CARTESIAN_POINT('Ctrl Pts',(49.3836326934911,248.094280502961,31.5613203435596)) ;
#82508=CARTESIAN_POINT('Ctrl Pts',(49.5470356170248,248.305739818825,31.9213203435596)) ;
#82509=CARTESIAN_POINT('Ctrl Pts',(49.5470356170248,248.305739818825,31.5613203435596)) ;
#82510=CARTESIAN_POINT('Ctrl Pts',(49.6274070383127,248.40974827469,31.9213203435596)) ;
#82511=CARTESIAN_POINT('Ctrl Pts',(49.6274070383127,248.40974827469,31.5613203435596)) ;
#82512=CARTESIAN_POINT('',(49.6274070383127,248.40974827469,31.9213203435596)) ;
#82513=CARTESIAN_POINT('',(49.3518273473795,247.692149180776,31.9213203435596)) ;
#82514=CARTESIAN_POINT('Ctrl Pts',(49.5182664633806,247.089148063069,31.9213203435596)) ;
#82515=CARTESIAN_POINT('Ctrl Pts',(49.5182664633806,247.089148063069,31.5613203435596)) ;
#82516=CARTESIAN_POINT('Ctrl Pts',(49.4697226969388,247.182950526379,31.9213203435596)) ;
#82517=CARTESIAN_POINT('Ctrl Pts',(49.4697226969388,247.182950526379,31.5613203435596)) ;
#82518=CARTESIAN_POINT('Ctrl Pts',(49.3717947762919,247.372179357529,31.9213203435596)) ;
#82519=CARTESIAN_POINT('Ctrl Pts',(49.3717947762919,247.372179357529,31.5613203435596)) ;
#82520=CARTESIAN_POINT('Ctrl Pts',(49.3585211271629,247.58488411708,31.9213203435596)) ;
#82521=CARTESIAN_POINT('Ctrl Pts',(49.3585211271629,247.58488411708,31.5613203435596)) ;
#82522=CARTESIAN_POINT('Ctrl Pts',(49.3518273473795,247.692149180776,31.9213203435596)) ;
#82523=CARTESIAN_POINT('Ctrl Pts',(49.3518273473795,247.692149180776,31.5613203435596)) ;
#82524=CARTESIAN_POINT('',(49.5182664633806,247.089148063069,31.9213203435596)) ;
#82525=CARTESIAN_POINT('Ctrl Pts',(49.963014268976,246.709884602433,31.9213203435596)) ;
#82526=CARTESIAN_POINT('Ctrl Pts',(49.963014268976,246.709884602433,31.5613203435596)) ;
#82527=CARTESIAN_POINT('Ctrl Pts',(49.8744014403106,246.75312764397,31.9213203435596)) ;
#82528=CARTESIAN_POINT('Ctrl Pts',(49.8744014403106,246.75312764397,31.5613203435596)) ;
#82529=CARTESIAN_POINT('Ctrl Pts',(49.6937403867375,246.841290199679,31.9213203435596)) ;
#82530=CARTESIAN_POINT('Ctrl Pts',(49.6937403867375,246.841290199679,31.5613203435596)) ;
#82531=CARTESIAN_POINT('Ctrl Pts',(49.5774946027845,247.005487996637,31.9213203435596)) ;
#82532=CARTESIAN_POINT('Ctrl Pts',(49.5774946027845,247.005487996637,31.5613203435596)) ;
#82533=CARTESIAN_POINT('Ctrl Pts',(49.5182664633806,247.089148063069,31.9213203435596)) ;
#82534=CARTESIAN_POINT('Ctrl Pts',(49.5182664633806,247.089148063069,31.5613203435596)) ;
#82535=CARTESIAN_POINT('',(49.963014268976,246.709884602433,31.9213203435596)) ;
#82536=CARTESIAN_POINT('Ctrl Pts',(50.7761110306795,246.600744027501,31.9213203435596)) ;
#82537=CARTESIAN_POINT('Ctrl Pts',(50.7761110306795,246.600744027501,31.5613203435596)) ;
#82538=CARTESIAN_POINT('Ctrl Pts',(50.618064325309,246.601984054257,31.9213203435596)) ;
#82539=CARTESIAN_POINT('Ctrl Pts',(50.618064325309,246.601984054257,31.5613203435596)) ;
#82540=CARTESIAN_POINT('Ctrl Pts',(50.341991448014,246.604150108612,31.9213203435596)) ;
#82541=CARTESIAN_POINT('Ctrl Pts',(50.341991448014,246.604150108612,31.5613203435596)) ;
#82542=CARTESIAN_POINT('Ctrl Pts',(50.0765116899345,246.678218863653,31.9213203435596)) ;
#82543=CARTESIAN_POINT('Ctrl Pts',(50.0765116899345,246.678218863653,31.5613203435596)) ;
#82544=CARTESIAN_POINT('Ctrl Pts',(49.963014268976,246.709884602433,31.9213203435596)) ;
#82545=CARTESIAN_POINT('Ctrl Pts',(49.963014268976,246.709884602433,31.5613203435596)) ;
#82546=CARTESIAN_POINT('',(50.7761110306795,246.600744027501,31.9213203435596)) ;
#82547=CARTESIAN_POINT('Origin',(52.5496443674977,246.600744027501,31.9213203435596)) ;
#82548=CARTESIAN_POINT('',(52.5496443674977,246.600744027501,31.9213203435596)) ;
#82549=CARTESIAN_POINT('Origin',(52.5496443674977,250.600744087106,31.9213203435596)) ;
#82550=CARTESIAN_POINT('',(52.5496443674977,250.600744087106,31.9213203435596)) ;
#82551=CARTESIAN_POINT('Origin',(52.0203128398474,250.600744087106,31.9213203435596)) ;
#82552=CARTESIAN_POINT('',(52.0203128398474,250.600744087106,31.9213203435596)) ;
#82553=CARTESIAN_POINT('Origin',(52.0203128398474,248.824482161408,31.9213203435596)) ;
#82554=CARTESIAN_POINT('Origin',(53.7,239.383507185188,31.9213203435596)) ;
#82555=CARTESIAN_POINT('',(79.0999999999999,263.8,31.9213203435596)) ;
#82556=CARTESIAN_POINT('',(79.0999999999999,259.648528137424,31.9213203435596)) ;
#82557=CARTESIAN_POINT('',(79.0999999999999,249.391753592594,31.9213203435596)) ;
#82558=CARTESIAN_POINT('',(78.2,263.8,31.9213203435596)) ;
#82559=CARTESIAN_POINT('',(66.4499999999999,263.8,31.9213203435596)) ;
#82560=CARTESIAN_POINT('',(78.2,263.763591785235,31.9213203435596)) ;
#82561=CARTESIAN_POINT('',(78.2,252.191753592594,31.9213203435596)) ;
#82562=CARTESIAN_POINT('',(76.5,262.026327083856,31.9213203435596)) ;
#82563=CARTESIAN_POINT('Origin',(76.5,263.763591785235,31.9213203435596)) ;
#82564=CARTESIAN_POINT('',(69.9,262.026327083856,31.9213203435596)) ;
#82565=CARTESIAN_POINT('',(64.4,262.026327083856,31.9213203435596)) ;
#82566=CARTESIAN_POINT('',(68.2,263.763591785235,31.9213203435596)) ;
#82567=CARTESIAN_POINT('Origin',(69.9,263.763591785235,31.9213203435596)) ;
#82568=CARTESIAN_POINT('',(68.2,263.8,31.9213203435596)) ;
#82569=CARTESIAN_POINT('',(68.2,251.191753592594,31.9213203435596)) ;
#82570=CARTESIAN_POINT('',(61.5,263.8,31.9213203435596)) ;
#82571=CARTESIAN_POINT('',(66.4499999999999,263.8,31.9213203435596)) ;
#82572=CARTESIAN_POINT('',(64.1,261.2,31.9213203435596)) ;
#82573=CARTESIAN_POINT('Origin',(61.5,261.2,31.9213203435596)) ;
#82574=CARTESIAN_POINT('Origin',(61.5,261.2,31.9213203435596)) ;
#82575=CARTESIAN_POINT('',(56.2,263.8,31.9213203435596)) ;
#82576=CARTESIAN_POINT('',(66.4499999999999,263.8,31.9213203435596)) ;
#82577=CARTESIAN_POINT('',(56.2,263.763591785235,31.9213203435596)) ;
#82578=CARTESIAN_POINT('',(56.2,252.191753592594,31.9213203435596)) ;
#82579=CARTESIAN_POINT('',(54.5,262.026327083856,31.9213203435596)) ;
#82580=CARTESIAN_POINT('Origin',(54.5,263.763591785235,31.9213203435596)) ;
#82581=CARTESIAN_POINT('',(47.9,262.026327083856,31.9213203435596)) ;
#82582=CARTESIAN_POINT('',(53.4,262.026327083856,31.9213203435596)) ;
#82583=CARTESIAN_POINT('',(46.2,263.763591785235,31.9213203435596)) ;
#82584=CARTESIAN_POINT('Origin',(47.9,263.763591785235,31.9213203435596)) ;
#82585=CARTESIAN_POINT('',(46.2,263.8,31.9213203435596)) ;
#82586=CARTESIAN_POINT('',(46.2,251.191753592594,31.9213203435596)) ;
#82587=CARTESIAN_POINT('',(26.3,263.8,31.9213203435596)) ;
#82588=CARTESIAN_POINT('',(66.4499999999999,263.8,31.9213203435596)) ;
#82589=CARTESIAN_POINT('',(26.3,245.6,31.9213203435596)) ;
#82590=CARTESIAN_POINT('',(26.3,252.191753592594,31.9213203435596)) ;
#82591=CARTESIAN_POINT('',(26.8,245.1,31.9213203435596)) ;
#82592=CARTESIAN_POINT('Origin',(26.8,245.6,31.9213203435596)) ;
#82593=CARTESIAN_POINT('',(33.6,245.1,31.9213203435596)) ;
#82594=CARTESIAN_POINT('',(39.95,245.1,31.9213203435596)) ;
#82595=CARTESIAN_POINT('',(34.1,245.6,31.9213203435596)) ;
#82596=CARTESIAN_POINT('Origin',(33.6,245.6,31.9213203435596)) ;
#82597=CARTESIAN_POINT('',(34.1,248.9,31.9213203435596)) ;
#82598=CARTESIAN_POINT('',(34.1000000000001,244.191753592594,31.9213203435596)) ;
#82599=CARTESIAN_POINT('',(34.3,249.1,31.9213203435596)) ;
#82600=CARTESIAN_POINT('Origin',(34.3,248.9,31.9213203435596)) ;
#82601=CARTESIAN_POINT('',(46.1,249.1,31.9213203435596)) ;
#82602=CARTESIAN_POINT('',(49.95,249.1,31.9213203435596)) ;
#82603=CARTESIAN_POINT('',(46.3,248.9,31.9213203435596)) ;
#82604=CARTESIAN_POINT('Origin',(46.1,248.9,31.9213203435596)) ;
#82605=CARTESIAN_POINT('',(46.2999999999999,245.6,31.9213203435596)) ;
#82606=CARTESIAN_POINT('',(46.2999999999999,242.191753592594,31.9213203435596)) ;
#82607=CARTESIAN_POINT('',(46.8,245.1,31.9213203435596)) ;
#82608=CARTESIAN_POINT('Origin',(46.8,245.6,31.9213203435596)) ;
#82609=CARTESIAN_POINT('',(55.3573593128808,245.1,31.9213203435596)) ;
#82610=CARTESIAN_POINT('',(39.95,245.1,31.9213203435596)) ;
#82611=CARTESIAN_POINT('',(56.0573593128807,244.4,31.9213203435596)) ;
#82612=CARTESIAN_POINT('Origin',(55.3573593128808,244.4,31.9213203435596)) ;
#82613=CARTESIAN_POINT('',(56.0573593128808,226.261195155516,31.9213203435596)) ;
#82614=CARTESIAN_POINT('',(56.0573593128807,242.191753592594,31.9213203435596)) ;
#82615=CARTESIAN_POINT('',(56.7626663401537,224.024247053747,31.9213203435596)) ;
#82616=CARTESIAN_POINT('Origin',(59.9573593128808,226.261195155516,31.9213203435596)) ;
#82617=CARTESIAN_POINT('',(61.2884174438392,217.560804636007,31.9213203435596)) ;
#82618=CARTESIAN_POINT('',(52.2889313872861,230.413402709377,31.9213203435596)) ;
#82619=CARTESIAN_POINT('',(63.8058825236653,215.957002501029,31.9213203435596)) ;
#82620=CARTESIAN_POINT('Origin',(64.4831104165663,219.797752737776,31.9213203435596)) ;
#82621=CARTESIAN_POINT('',(75.3227721070991,213.926264133629,31.9213203435596)) ;
#82622=CARTESIAN_POINT('',(56.086380506565,217.318158984277,31.9213203435596)) ;
#82623=CARTESIAN_POINT('',(79.9000000000001,217.767014370377,31.9213203435596)) ;
#82624=CARTESIAN_POINT('Origin',(76.0000000000001,217.767014370377,31.9213203435596)) ;
#82625=CARTESIAN_POINT('',(79.9000000000001,224.305309236676,31.9213203435596)) ;
#82626=CARTESIAN_POINT('',(79.9,228.575260777783,31.9213203435596)) ;
#82627=CARTESIAN_POINT('',(80.1050252531695,224.800283983507,31.9213203435596)) ;
#82628=CARTESIAN_POINT('Origin',(80.6000000000001,224.305309236676,31.9213203435596)) ;
#82629=CARTESIAN_POINT('',(80.9535533905933,225.64881212093,31.9213203435596)) ;
#82630=CARTESIAN_POINT('',(77.061706774654,221.756965504991,31.9213203435596)) ;
#82631=CARTESIAN_POINT('',(81.1,226.002365511524,31.9213203435596)) ;
#82632=CARTESIAN_POINT('Origin',(80.6,226.002365511524,31.9213203435596)) ;
#82633=CARTESIAN_POINT('',(81.1,236.901613323034,31.9213203435596)) ;
#82634=CARTESIAN_POINT('',(81.1,232.568672279644,31.9213203435596)) ;
#82635=CARTESIAN_POINT('',(80.616129032258,237.401353109641,31.9213203435596)) ;
#82636=CARTESIAN_POINT('Origin',(80.6,236.901613323034,31.9213203435596)) ;
#82637=CARTESIAN_POINT('',(78.0999999999999,240.,31.9213203435596)) ;
#82638=CARTESIAN_POINT('Origin',(80.6999999999999,240.,31.9213203435596)) ;
#82639=CARTESIAN_POINT('',(78.0999999999999,244.,31.9213203435596)) ;
#82640=CARTESIAN_POINT('',(78.0999999999999,239.691753592594,31.9213203435596)) ;
#82641=CARTESIAN_POINT('',(80.616129032258,246.598646890358,31.9213203435596)) ;
#82642=CARTESIAN_POINT('Origin',(80.6999999999999,244.,31.9213203435596)) ;
#82643=CARTESIAN_POINT('',(81.1,247.098386676966,31.9213203435596)) ;
#82644=CARTESIAN_POINT('Origin',(80.6,247.098386676966,31.9213203435596)) ;
#82645=CARTESIAN_POINT('',(81.1,257.151471862576,31.9213203435596)) ;
#82646=CARTESIAN_POINT('',(81.1,242.941753592594,31.9213203435596)) ;
#82647=CARTESIAN_POINT('',(80.9535533905932,257.50502525317,31.9213203435596)) ;
#82648=CARTESIAN_POINT('Origin',(80.6,257.151471862576,31.9213203435596)) ;
#82649=CARTESIAN_POINT('',(79.3050252531694,259.153553390593,31.9213203435596)) ;
#82650=CARTESIAN_POINT('',(78.758412525583,259.70016611818,31.9213203435596)) ;
#82651=CARTESIAN_POINT('Origin',(79.7999999999999,259.648528137424,31.9213203435596)) ;
#82652=CARTESIAN_POINT('',(69.6,244.169705627485,31.9213203435596)) ;
#82653=CARTESIAN_POINT('',(67.8102943725152,242.38,31.9213203435596)) ;
#82654=CARTESIAN_POINT('',(63.6360239825547,238.20572961004,31.9213203435596)) ;
#82655=CARTESIAN_POINT('',(71.3897056274848,242.38,31.9213203435596)) ;
#82656=CARTESIAN_POINT('',(66.8639760174453,246.90572961004,31.9213203435596)) ;
#82657=CARTESIAN_POINT('',(62.4,242.38,31.9213203435596)) ;
#82658=CARTESIAN_POINT('',(67.8102943725152,238.12,31.9213203435596)) ;
#82659=CARTESIAN_POINT('',(69.6,236.330294372515,31.9213203435596)) ;
#82660=CARTESIAN_POINT('',(64.8192703899605,241.111023982555,31.9213203435596)) ;
#82661=CARTESIAN_POINT('',(71.3897056274848,238.12,31.9213203435596)) ;
#82662=CARTESIAN_POINT('',(60.9,238.12,31.9213203435596)) ;
#82663=CARTESIAN_POINT('',(67.1807296100394,233.911023982555,31.9213203435596)) ;
#82664=CARTESIAN_POINT('',(67.3,247.9,31.9213203435596)) ;
#82665=CARTESIAN_POINT('',(67.5,248.1,31.9213203435596)) ;
#82666=CARTESIAN_POINT('Origin',(67.3,248.1,31.9213203435596)) ;
#82667=CARTESIAN_POINT('',(64.4999999999999,247.9,31.9213203435596)) ;
#82668=CARTESIAN_POINT('',(59.05,247.9,31.9213203435596)) ;
#82669=CARTESIAN_POINT('',(64.3,248.1,31.9213203435596)) ;
#82670=CARTESIAN_POINT('Origin',(64.4999999999999,248.1,31.9213203435596)) ;
#82671=CARTESIAN_POINT('',(64.3,250.9,31.9213203435596)) ;
#82672=CARTESIAN_POINT('',(64.3,245.191753592594,31.9213203435596)) ;
#82673=CARTESIAN_POINT('',(64.5,251.1,31.9213203435596)) ;
#82674=CARTESIAN_POINT('Origin',(64.5,250.9,31.9213203435596)) ;
#82675=CARTESIAN_POINT('',(64.6,251.1,31.9213203435596)) ;
#82676=CARTESIAN_POINT('',(59.2,251.1,31.9213203435596)) ;
#82677=CARTESIAN_POINT('',(64.6,256.9,31.9213203435596)) ;
#82678=CARTESIAN_POINT('',(64.6,248.191753592594,31.9213203435596)) ;
#82679=CARTESIAN_POINT('',(64.8,257.1,31.9213203435596)) ;
#82680=CARTESIAN_POINT('Origin',(64.8,256.9,31.9213203435596)) ;
#82681=CARTESIAN_POINT('',(67.,257.1,31.9213203435596)) ;
#82682=CARTESIAN_POINT('',(60.4,257.1,31.9213203435596)) ;
#82683=CARTESIAN_POINT('',(67.2,256.9,31.9213203435596)) ;
#82684=CARTESIAN_POINT('Origin',(67.,256.9,31.9213203435596)) ;
#82685=CARTESIAN_POINT('',(67.2,251.1,31.9213203435596)) ;
#82686=CARTESIAN_POINT('',(67.2,245.191753592594,31.9213203435596)) ;
#82687=CARTESIAN_POINT('',(67.3,251.1,31.9213203435596)) ;
#82688=CARTESIAN_POINT('',(60.55,251.1,31.9213203435596)) ;
#82689=CARTESIAN_POINT('',(67.5,250.9,31.9213203435596)) ;
#82690=CARTESIAN_POINT('Origin',(67.3,250.9,31.9213203435596)) ;
#82691=CARTESIAN_POINT('',(67.5,243.691753592594,31.9213203435596)) ;
#82692=CARTESIAN_POINT('',(80.299999999999,230.4,31.9213203435596)) ;
#82693=CARTESIAN_POINT('',(80.299999999999,229.3,31.9213203435596)) ;
#82694=CARTESIAN_POINT('',(80.299999999999,232.441753592594,31.9213203435596)) ;
#82695=CARTESIAN_POINT('',(80.1999999999999,229.3,31.9213203435596)) ;
#82696=CARTESIAN_POINT('',(66.9499999999995,229.3,31.9213203435596)) ;
#82697=CARTESIAN_POINT('',(80.1999999999999,226.7,31.9213203435596)) ;
#82698=CARTESIAN_POINT('',(80.1999999999999,234.391753592594,31.9213203435596)) ;
#82699=CARTESIAN_POINT('',(80.299999999999,226.7,31.9213203435596)) ;
#82700=CARTESIAN_POINT('',(66.4499999999997,226.700000000001,31.9213203435596)) ;
#82701=CARTESIAN_POINT('',(80.2999999999989,225.6,31.9213203435596)) ;
#82702=CARTESIAN_POINT('',(80.299999999999,232.441753592594,31.9213203435596)) ;
#82703=CARTESIAN_POINT('',(80.0999999999989,225.4,31.9213203435596)) ;
#82704=CARTESIAN_POINT('Origin',(80.0999999999989,225.6,31.9213203435596)) ;
#82705=CARTESIAN_POINT('',(76.0414213562366,225.4,31.9213203435596)) ;
#82706=CARTESIAN_POINT('',(64.4499999999996,225.4,31.9213203435596)) ;
#82707=CARTESIAN_POINT('',(75.8999999999993,225.458578643763,31.9213203435596)) ;
#82708=CARTESIAN_POINT('Origin',(76.0414213562366,225.6,31.9213203435596)) ;
#82709=CARTESIAN_POINT('',(75.158578643762,226.2,31.9213203435596)) ;
#82710=CARTESIAN_POINT('',(66.6834125255838,234.675166118178,31.9213203435596)) ;
#82711=CARTESIAN_POINT('',(75.0999999999993,226.341421356237,31.9213203435596)) ;
#82712=CARTESIAN_POINT('Origin',(75.2999999999993,226.341421356237,31.9213203435596)) ;
#82713=CARTESIAN_POINT('',(75.0999999999994,229.658578643763,31.9213203435596)) ;
#82714=CARTESIAN_POINT('',(75.0999999999996,234.941753592594,31.9213203435596)) ;
#82715=CARTESIAN_POINT('',(75.1585786437621,229.8,31.9213203435596)) ;
#82716=CARTESIAN_POINT('Origin',(75.2999999999994,229.658578643763,31.9213203435596)) ;
#82717=CARTESIAN_POINT('',(75.8999999999994,230.541421356237,31.9213203435596)) ;
#82718=CARTESIAN_POINT('',(72.3751661181778,227.016587474416,31.9213203435596)) ;
#82719=CARTESIAN_POINT('',(76.0414213562367,230.6,31.9213203435596)) ;
#82720=CARTESIAN_POINT('Origin',(76.0414213562367,230.4,31.9213203435596)) ;
#82721=CARTESIAN_POINT('',(80.099999999999,230.6,31.9213203435596)) ;
#82722=CARTESIAN_POINT('',(66.9499999999995,230.6,31.9213203435596)) ;
#82723=CARTESIAN_POINT('Origin',(80.099999999999,230.4,31.9213203435596)) ;
#82724=CARTESIAN_POINT('',(71.5999999999999,226.1,31.9213203435596)) ;
#82725=CARTESIAN_POINT('',(71.3999999999999,225.9,31.9213203435596)) ;
#82726=CARTESIAN_POINT('Origin',(71.5999999999999,225.9,31.9213203435596)) ;
#82727=CARTESIAN_POINT('',(71.6999999999999,226.1,31.9213203435596)) ;
#82728=CARTESIAN_POINT('',(62.75,226.1,31.9213203435596)) ;
#82729=CARTESIAN_POINT('',(71.6999999999999,231.9,31.9213203435596)) ;
#82730=CARTESIAN_POINT('',(71.6999999999999,235.691753592594,31.9213203435596)) ;
#82731=CARTESIAN_POINT('',(71.8999999999999,232.1,31.9213203435596)) ;
#82732=CARTESIAN_POINT('Origin',(71.8999999999999,231.9,31.9213203435596)) ;
#82733=CARTESIAN_POINT('',(74.0999999999999,232.1,31.9213203435596)) ;
#82734=CARTESIAN_POINT('',(63.95,232.1,31.9213203435596)) ;
#82735=CARTESIAN_POINT('',(74.2999999999999,231.9,31.9213203435596)) ;
#82736=CARTESIAN_POINT('Origin',(74.0999999999999,231.9,31.9213203435596)) ;
#82737=CARTESIAN_POINT('',(74.2999999999999,226.1,31.9213203435596)) ;
#82738=CARTESIAN_POINT('',(74.2999999999999,232.691753592594,31.9213203435596)) ;
#82739=CARTESIAN_POINT('',(74.3999999999999,226.1,31.9213203435596)) ;
#82740=CARTESIAN_POINT('',(64.1,226.1,31.9213203435596)) ;
#82741=CARTESIAN_POINT('',(74.5999999999999,225.9,31.9213203435596)) ;
#82742=CARTESIAN_POINT('Origin',(74.3999999999999,225.9,31.9213203435596)) ;
#82743=CARTESIAN_POINT('',(74.5999999999999,223.1,31.9213203435596)) ;
#82744=CARTESIAN_POINT('',(74.5999999999999,231.191753592594,31.9213203435596)) ;
#82745=CARTESIAN_POINT('',(74.3999999999999,222.9,31.9213203435596)) ;
#82746=CARTESIAN_POINT('Origin',(74.3999999999999,223.1,31.9213203435596)) ;
#82747=CARTESIAN_POINT('',(71.5999999999999,222.9,31.9213203435596)) ;
#82748=CARTESIAN_POINT('',(62.6,222.9,31.9213203435596)) ;
#82749=CARTESIAN_POINT('',(71.3999999999999,223.1,31.9213203435596)) ;
#82750=CARTESIAN_POINT('Origin',(71.5999999999999,223.1,31.9213203435596)) ;
#82751=CARTESIAN_POINT('',(71.3999999999999,232.691753592594,31.9213203435596)) ;
#82752=CARTESIAN_POINT('',(59.7573593128808,230.1,31.9213203435596)) ;
#82753=CARTESIAN_POINT('',(59.5573593128808,229.9,31.9213203435596)) ;
#82754=CARTESIAN_POINT('Origin',(59.7573593128808,229.9,31.9213203435596)) ;
#82755=CARTESIAN_POINT('',(59.8573593128808,230.1,31.9213203435596)) ;
#82756=CARTESIAN_POINT('',(56.8286796564404,230.1,31.9213203435596)) ;
#82757=CARTESIAN_POINT('',(59.8573593128808,235.9,31.9213203435596)) ;
#82758=CARTESIAN_POINT('',(59.8573593128808,237.691753592594,31.9213203435596)) ;
#82759=CARTESIAN_POINT('',(60.0573593128808,236.1,31.9213203435596)) ;
#82760=CARTESIAN_POINT('Origin',(60.0573593128808,235.9,31.9213203435596)) ;
#82761=CARTESIAN_POINT('',(62.2573593128808,236.1,31.9213203435596)) ;
#82762=CARTESIAN_POINT('',(58.0286796564404,236.1,31.9213203435596)) ;
#82763=CARTESIAN_POINT('',(62.4573593128808,235.9,31.9213203435596)) ;
#82764=CARTESIAN_POINT('Origin',(62.2573593128808,235.9,31.9213203435596)) ;
#82765=CARTESIAN_POINT('',(62.4573593128808,230.1,31.9213203435596)) ;
#82766=CARTESIAN_POINT('',(62.4573593128808,234.691753592594,31.9213203435596)) ;
#82767=CARTESIAN_POINT('',(62.5573593128808,230.1,31.9213203435596)) ;
#82768=CARTESIAN_POINT('',(58.1786796564404,230.1,31.9213203435596)) ;
#82769=CARTESIAN_POINT('',(62.7573593128808,229.9,31.9213203435596)) ;
#82770=CARTESIAN_POINT('Origin',(62.5573593128808,229.9,31.9213203435596)) ;
#82771=CARTESIAN_POINT('',(62.7573593128808,227.1,31.9213203435596)) ;
#82772=CARTESIAN_POINT('',(62.7573593128808,233.191753592594,31.9213203435596)) ;
#82773=CARTESIAN_POINT('',(62.5573593128808,226.9,31.9213203435596)) ;
#82774=CARTESIAN_POINT('Origin',(62.5573593128808,227.1,31.9213203435596)) ;
#82775=CARTESIAN_POINT('',(59.7573593128808,226.9,31.9213203435596)) ;
#82776=CARTESIAN_POINT('',(56.6786796564404,226.9,31.9213203435596)) ;
#82777=CARTESIAN_POINT('',(59.5573593128808,227.1,31.9213203435596)) ;
#82778=CARTESIAN_POINT('Origin',(59.7573593128808,227.1,31.9213203435596)) ;
#82779=CARTESIAN_POINT('',(59.5573593128808,234.691753592594,31.9213203435596)) ;
#82780=CARTESIAN_POINT('',(80.299999999999,253.6,31.9213203435596)) ;
#82781=CARTESIAN_POINT('',(80.299999999999,252.3,31.9213203435596)) ;
#82782=CARTESIAN_POINT('',(80.2999999999989,243.941753592594,31.9213203435596)) ;
#82783=CARTESIAN_POINT('',(80.1999999999999,252.3,31.9213203435596)) ;
#82784=CARTESIAN_POINT('',(66.9499999999999,252.3,31.9213203435596)) ;
#82785=CARTESIAN_POINT('',(80.1999999999999,249.7,31.9213203435596)) ;
#82786=CARTESIAN_POINT('',(80.1999999999999,245.891753592594,31.9213203435596)) ;
#82787=CARTESIAN_POINT('',(80.2999999999989,249.7,31.9213203435596)) ;
#82788=CARTESIAN_POINT('',(66.4500000000001,249.700000000001,31.9213203435596)) ;
#82789=CARTESIAN_POINT('',(80.2999999999989,248.4,31.9213203435596)) ;
#82790=CARTESIAN_POINT('',(80.2999999999989,243.941753592594,31.9213203435596)) ;
#82791=CARTESIAN_POINT('',(76.0414213562365,248.4,31.9213203435596)) ;
#82792=CARTESIAN_POINT('',(64.4499999999996,248.4,31.9213203435596)) ;
#82793=CARTESIAN_POINT('',(75.8999999999992,248.458578643763,31.9213203435596)) ;
#82794=CARTESIAN_POINT('Origin',(76.0414213562365,248.6,31.9213203435596)) ;
#82795=CARTESIAN_POINT('',(75.158578643762,249.2,31.9213203435596)) ;
#82796=CARTESIAN_POINT('',(72.4334125255833,251.925166118179,31.9213203435596)) ;
#82797=CARTESIAN_POINT('',(75.0999999999993,249.341421356237,31.9213203435596)) ;
#82798=CARTESIAN_POINT('Origin',(75.2999999999993,249.341421356237,31.9213203435596)) ;
#82799=CARTESIAN_POINT('',(75.0999999999994,252.658578643763,31.9213203435596)) ;
#82800=CARTESIAN_POINT('',(75.0999999999992,246.441753592594,31.9213203435596)) ;
#82801=CARTESIAN_POINT('',(75.1585786437621,252.8,31.9213203435596)) ;
#82802=CARTESIAN_POINT('Origin',(75.2999999999994,252.658578643763,31.9213203435596)) ;
#82803=CARTESIAN_POINT('',(75.8999999999994,253.541421356237,31.9213203435596)) ;
#82804=CARTESIAN_POINT('',(66.6251661181778,244.266587474416,31.9213203435596)) ;
#82805=CARTESIAN_POINT('',(76.0414213562367,253.6,31.9213203435596)) ;
#82806=CARTESIAN_POINT('Origin',(76.0414213562367,253.4,31.9213203435596)) ;
#82807=CARTESIAN_POINT('',(66.9499999999995,253.6,31.9213203435596)) ;
#82808=CARTESIAN_POINT('',(33.3,254.8,31.9213203435596)) ;
#82809=CARTESIAN_POINT('Origin',(30.6999999999999,254.8,31.9213203435596)) ;
#82810=CARTESIAN_POINT('',(28.1,262.2,31.9213203435596)) ;
#82811=CARTESIAN_POINT('',(28.1,263.3,31.9213203435596)) ;
#82812=CARTESIAN_POINT('',(28.1,251.391753592594,31.9213203435596)) ;
#82813=CARTESIAN_POINT('',(28.2999999999999,263.5,31.9213203435596)) ;
#82814=CARTESIAN_POINT('Origin',(28.2999999999999,263.3,31.9213203435596)) ;
#82815=CARTESIAN_POINT('',(32.3585786437627,263.5,31.9213203435596)) ;
#82816=CARTESIAN_POINT('',(43.45,263.5,31.9213203435596)) ;
#82817=CARTESIAN_POINT('',(32.5,263.441421356237,31.9213203435596)) ;
#82818=CARTESIAN_POINT('Origin',(32.3585786437627,263.3,31.9213203435596)) ;
#82819=CARTESIAN_POINT('',(33.2414213562373,262.7,31.9213203435596)) ;
#82820=CARTESIAN_POINT('',(43.9998338818216,251.941587474416,31.9213203435596)) ;
#82821=CARTESIAN_POINT('',(33.2999999999999,262.558578643763,31.9213203435596)) ;
#82822=CARTESIAN_POINT('Origin',(33.1,262.558578643763,31.9213203435596)) ;
#82823=CARTESIAN_POINT('',(33.2999999999999,259.241421356237,31.9213203435596)) ;
#82824=CARTESIAN_POINT('',(33.2999999999999,248.891753592594,31.9213203435596)) ;
#82825=CARTESIAN_POINT('',(33.2414213562373,259.1,31.9213203435596)) ;
#82826=CARTESIAN_POINT('Origin',(33.1,259.241421356237,31.9213203435596)) ;
#82827=CARTESIAN_POINT('',(32.5,258.358578643763,31.9213203435596)) ;
#82828=CARTESIAN_POINT('',(33.2415874744158,259.100166118179,31.9213203435596)) ;
#82829=CARTESIAN_POINT('',(32.3585786437627,258.3,31.9213203435596)) ;
#82830=CARTESIAN_POINT('Origin',(32.3585786437627,258.5,31.9213203435596)) ;
#82831=CARTESIAN_POINT('',(28.1,258.3,31.9213203435596)) ;
#82832=CARTESIAN_POINT('',(40.95,258.3,31.9213203435596)) ;
#82833=CARTESIAN_POINT('',(28.1,259.6,31.9213203435596)) ;
#82834=CARTESIAN_POINT('',(28.1,251.391753592594,31.9213203435596)) ;
#82835=CARTESIAN_POINT('',(28.1999999999999,259.6,31.9213203435596)) ;
#82836=CARTESIAN_POINT('',(40.9499999999996,259.6,31.9213203435596)) ;
#82837=CARTESIAN_POINT('',(28.1999999999999,262.2,31.9213203435596)) ;
#82838=CARTESIAN_POINT('',(28.1999999999999,249.441753592594,31.9213203435596)) ;
#82839=CARTESIAN_POINT('',(41.45,262.2,31.9213203435596)) ;
#82840=CARTESIAN_POINT('',(55.2649110640673,257.,31.9213203435596)) ;
#82841=CARTESIAN_POINT('Origin',(51.2,257.,31.9213203435596)) ;
#82842=CARTESIAN_POINT('',(79.8149110640674,218.,31.9213203435596)) ;
#82843=CARTESIAN_POINT('Origin',(75.7500000000001,218.,31.9213203435596)) ;
#82844=CARTESIAN_POINT('',(57.8573593128808,241.8,31.9213203435596)) ;
#82845=CARTESIAN_POINT('',(57.9573593128808,241.8,31.9213203435596)) ;
#82846=CARTESIAN_POINT('',(56.3286796564404,241.8,31.9213203435596)) ;
#82847=CARTESIAN_POINT('',(57.8573593128808,243.1,31.9213203435596)) ;
#82848=CARTESIAN_POINT('',(57.8573593128808,241.191753592594,31.9213203435596)) ;
#82849=CARTESIAN_POINT('',(62.1159379566435,243.1,31.9213203435596)) ;
#82850=CARTESIAN_POINT('',(58.3286796564404,243.1,31.9213203435596)) ;
#82851=CARTESIAN_POINT('',(62.2573593128808,243.041421356237,31.9213203435596)) ;
#82852=CARTESIAN_POINT('Origin',(62.1159379566435,242.9,31.9213203435596)) ;
#82853=CARTESIAN_POINT('',(62.9987806691181,242.3,31.9213203435596)) ;
#82854=CARTESIAN_POINT('',(61.2178533664821,244.080927302636,31.9213203435596)) ;
#82855=CARTESIAN_POINT('',(63.0573593128807,242.158578643763,31.9213203435596)) ;
#82856=CARTESIAN_POINT('Origin',(62.8573593128808,242.158578643763,31.9213203435596)) ;
#82857=CARTESIAN_POINT('',(63.0573593128807,238.841421356237,31.9213203435596)) ;
#82858=CARTESIAN_POINT('',(63.0573593128807,238.691753592594,31.9213203435596)) ;
#82859=CARTESIAN_POINT('',(62.998780669118,238.7,31.9213203435596)) ;
#82860=CARTESIAN_POINT('Origin',(62.8573593128808,238.841421356237,31.9213203435596)) ;
#82861=CARTESIAN_POINT('',(62.2573593128808,237.958578643763,31.9213203435596)) ;
#82862=CARTESIAN_POINT('',(60.6596069590762,236.360826289958,31.9213203435596)) ;
#82863=CARTESIAN_POINT('',(62.1159379566435,237.9,31.9213203435596)) ;
#82864=CARTESIAN_POINT('Origin',(62.1159379566435,238.1,31.9213203435596)) ;
#82865=CARTESIAN_POINT('',(57.8573593128808,237.9,31.9213203435596)) ;
#82866=CARTESIAN_POINT('',(55.8286796564404,237.9,31.9213203435596)) ;
#82867=CARTESIAN_POINT('',(57.8573593128808,239.2,31.9213203435596)) ;
#82868=CARTESIAN_POINT('',(57.8573593128808,241.191753592594,31.9213203435596)) ;
#82869=CARTESIAN_POINT('',(57.9573593128808,239.2,31.9213203435596)) ;
#82870=CARTESIAN_POINT('',(55.8286796564404,239.2,31.9213203435596)) ;
#82871=CARTESIAN_POINT('',(57.9573593128808,239.241753592594,31.9213203435596)) ;
#82872=CARTESIAN_POINT('',(77.2649110640673,257.,31.9213203435596)) ;
#82873=CARTESIAN_POINT('Origin',(73.2,257.,31.9213203435596)) ;
#82874=CARTESIAN_POINT('',(66.2568347953872,220.146231446812,31.9213203435596)) ;
#82875=CARTESIAN_POINT('Origin',(64.1568347953873,220.146231446812,31.9213203435596)) ;
#82876=CARTESIAN_POINT('',(37.2999999999999,260.1,31.9213203435596)) ;
#82877=CARTESIAN_POINT('',(37.0999999999999,259.9,31.9213203435596)) ;
#82878=CARTESIAN_POINT('Origin',(37.2999999999999,259.9,31.9213203435596)) ;
#82879=CARTESIAN_POINT('',(43.0999999999999,260.1,31.9213203435596)) ;
#82880=CARTESIAN_POINT('',(48.4499999999999,260.1,31.9213203435596)) ;
#82881=CARTESIAN_POINT('',(43.2999999999999,259.9,31.9213203435596)) ;
#82882=CARTESIAN_POINT('Origin',(43.0999999999999,259.9,31.9213203435596)) ;
#82883=CARTESIAN_POINT('',(43.2999999999999,252.1,31.9213203435596)) ;
#82884=CARTESIAN_POINT('',(43.2999999999999,245.691753592594,31.9213203435596)) ;
#82885=CARTESIAN_POINT('',(43.0999999999999,251.9,31.9213203435596)) ;
#82886=CARTESIAN_POINT('Origin',(43.0999999999999,252.1,31.9213203435596)) ;
#82887=CARTESIAN_POINT('',(37.2999999999999,251.9,31.9213203435596)) ;
#82888=CARTESIAN_POINT('',(45.4499999999999,251.9,31.9213203435596)) ;
#82889=CARTESIAN_POINT('',(37.0999999999999,252.1,31.9213203435596)) ;
#82890=CARTESIAN_POINT('Origin',(37.2999999999999,252.1,31.9213203435596)) ;
#82891=CARTESIAN_POINT('',(37.0999999999999,249.691753592594,31.9213203435596)) ;
#82892=CARTESIAN_POINT('',(59.3,247.9,31.9213203435596)) ;
#82893=CARTESIAN_POINT('',(59.5,248.1,31.9213203435596)) ;
#82894=CARTESIAN_POINT('Origin',(59.3,248.1,31.9213203435596)) ;
#82895=CARTESIAN_POINT('',(56.5,247.9,31.9213203435596)) ;
#82896=CARTESIAN_POINT('',(55.05,247.9,31.9213203435596)) ;
#82897=CARTESIAN_POINT('',(56.3,248.1,31.9213203435596)) ;
#82898=CARTESIAN_POINT('Origin',(56.5,248.1,31.9213203435596)) ;
#82899=CARTESIAN_POINT('',(56.3,250.9,31.9213203435596)) ;
#82900=CARTESIAN_POINT('',(56.3,245.191753592594,31.9213203435596)) ;
#82901=CARTESIAN_POINT('',(56.5,251.1,31.9213203435596)) ;
#82902=CARTESIAN_POINT('Origin',(56.5,250.9,31.9213203435596)) ;
#82903=CARTESIAN_POINT('',(56.6,251.1,31.9213203435596)) ;
#82904=CARTESIAN_POINT('',(55.2,251.1,31.9213203435596)) ;
#82905=CARTESIAN_POINT('',(56.6,256.9,31.9213203435596)) ;
#82906=CARTESIAN_POINT('',(56.6,248.191753592594,31.9213203435596)) ;
#82907=CARTESIAN_POINT('',(56.8,257.1,31.9213203435596)) ;
#82908=CARTESIAN_POINT('Origin',(56.8,256.9,31.9213203435596)) ;
#82909=CARTESIAN_POINT('',(59.,257.1,31.9213203435596)) ;
#82910=CARTESIAN_POINT('',(56.4,257.1,31.9213203435596)) ;
#82911=CARTESIAN_POINT('',(59.2,256.9,31.9213203435596)) ;
#82912=CARTESIAN_POINT('Origin',(59.,256.9,31.9213203435596)) ;
#82913=CARTESIAN_POINT('',(59.2,251.1,31.9213203435596)) ;
#82914=CARTESIAN_POINT('',(59.2,245.191753592594,31.9213203435596)) ;
#82915=CARTESIAN_POINT('',(59.3,251.1,31.9213203435596)) ;
#82916=CARTESIAN_POINT('',(56.55,251.1,31.9213203435596)) ;
#82917=CARTESIAN_POINT('',(59.5,250.9,31.9213203435596)) ;
#82918=CARTESIAN_POINT('Origin',(59.3,250.9,31.9213203435596)) ;
#82919=CARTESIAN_POINT('',(59.5,243.691753592594,31.9213203435596)) ;
#82920=CARTESIAN_POINT('',(67.98,240.62,31.9213203435596)) ;
#82921=CARTESIAN_POINT('',(67.98,239.88,31.9213203435596)) ;
#82922=CARTESIAN_POINT('',(67.98,239.691753592594,31.9213203435596)) ;
#82923=CARTESIAN_POINT('',(71.22,240.62,31.9213203435596)) ;
#82924=CARTESIAN_POINT('',(60.9,240.62,31.9213203435596)) ;
#82925=CARTESIAN_POINT('',(71.22,239.88,31.9213203435596)) ;
#82926=CARTESIAN_POINT('',(71.22,239.941753592594,31.9213203435596)) ;
#82927=CARTESIAN_POINT('',(62.4,239.88,31.9213203435596)) ;
#82928=CARTESIAN_POINT('Origin',(63.6360239825547,238.20572961004,31.8013203435596)) ;
#82929=CARTESIAN_POINT('Origin',(67.8102943725152,242.38,31.8013203435596)) ;
#82930=CARTESIAN_POINT('Origin',(69.6,244.169705627485,31.8013203435596)) ;
#82931=CARTESIAN_POINT('Origin',(62.4,242.38,31.8013203435596)) ;
#82932=CARTESIAN_POINT('Origin',(71.3897056274848,242.38,31.8013203435596)) ;
#82933=CARTESIAN_POINT('Origin',(66.8639760174453,246.90572961004,31.8013203435596)) ;
#82934=CARTESIAN_POINT('',(66.7791232037029,246.820876796297,31.8013203435596)) ;
#82935=CARTESIAN_POINT('Origin',(69.6,244.,31.9213203435596)) ;
#82936=CARTESIAN_POINT('Origin',(67.98,239.691753592594,31.8013203435596)) ;
#82937=CARTESIAN_POINT('Origin',(67.98,239.88,31.8013203435596)) ;
#82938=CARTESIAN_POINT('Origin',(67.98,240.62,31.8013203435596)) ;
#82939=CARTESIAN_POINT('Origin',(62.4,239.88,31.8013203435596)) ;
#82940=CARTESIAN_POINT('Origin',(71.22,239.88,31.8013203435596)) ;
#82941=CARTESIAN_POINT('Origin',(71.22,239.941753592594,31.8013203435596)) ;
#82942=CARTESIAN_POINT('',(71.1,240.5,31.8013203435596)) ;
#82943=CARTESIAN_POINT('',(71.1,239.941753592594,31.8013203435596)) ;
#82944=CARTESIAN_POINT('Origin',(71.22,240.62,31.8013203435596)) ;
#82945=CARTESIAN_POINT('Origin',(60.9,240.62,31.8013203435596)) ;
#82946=CARTESIAN_POINT('',(60.9,240.5,31.8013203435596)) ;
#82947=CARTESIAN_POINT('Origin',(68.1,240.5,31.9213203435596)) ;
#82948=CARTESIAN_POINT('',(71.1,240.5,31.9213203435596)) ;
#82949=CARTESIAN_POINT('Origin',(64.8192703899605,241.111023982555,31.8013203435596)) ;
#82950=CARTESIAN_POINT('Origin',(69.6,236.330294372515,31.8013203435596)) ;
#82951=CARTESIAN_POINT('Origin',(67.8102943725152,238.12,31.8013203435596)) ;
#82952=CARTESIAN_POINT('Origin',(67.1807296100394,233.911023982555,31.8013203435596)) ;
#82953=CARTESIAN_POINT('Origin',(71.3897056274848,238.12,31.8013203435596)) ;
#82954=CARTESIAN_POINT('Origin',(60.9,238.12,31.8013203435596)) ;
#82955=CARTESIAN_POINT('',(60.9,238.,31.8013203435596)) ;
#82956=CARTESIAN_POINT('Origin',(68.1,238.,31.9213203435596)) ;
#82957=CARTESIAN_POINT('Origin',(71.1,240.5,31.9213203435596)) ;
#82958=CARTESIAN_POINT('Ctrl Pts',(50.1048968673761,247.225573558217,31.9213203435596)) ;
#82959=CARTESIAN_POINT('Ctrl Pts',(50.1048968673761,247.225573558217,31.5613203435596)) ;
#82960=CARTESIAN_POINT('Ctrl Pts',(50.1908486902686,247.172482844858,31.9213203435596)) ;
#82961=CARTESIAN_POINT('Ctrl Pts',(50.1908486902686,247.172482844858,31.5613203435596)) ;
#82962=CARTESIAN_POINT('Ctrl Pts',(50.3885184489928,247.05038620808,31.9213203435596)) ;
#82963=CARTESIAN_POINT('Ctrl Pts',(50.3885184489928,247.05038620808,31.5613203435596)) ;
#82964=CARTESIAN_POINT('Ctrl Pts',(50.6222076847147,247.045515776756,31.9213203435596)) ;
#82965=CARTESIAN_POINT('Ctrl Pts',(50.6222076847147,247.045515776756,31.5613203435596)) ;
#82966=CARTESIAN_POINT('Ctrl Pts',(50.7542829156931,247.042763132459,31.9213203435596)) ;
#82967=CARTESIAN_POINT('Ctrl Pts',(50.7542829156931,247.042763132459,31.5613203435596)) ;
#82968=CARTESIAN_POINT('',(50.1048968673761,247.225573558217,31.9213203435596)) ;
#82969=CARTESIAN_POINT('Ctrl Pts',(49.8975299240168,247.692149180776,31.9213203435596)) ;
#82970=CARTESIAN_POINT('Ctrl Pts',(49.8975299240168,247.692149180776,31.5613203435596)) ;
#82971=CARTESIAN_POINT('Ctrl Pts',(49.9059085609628,247.601999233154,31.9213203435596)) ;
#82972=CARTESIAN_POINT('Ctrl Pts',(49.9059085609628,247.601999233154,31.5613203435596)) ;
#82973=CARTESIAN_POINT('Ctrl Pts',(49.9225413218171,247.423039035993,31.9213203435596)) ;
#82974=CARTESIAN_POINT('Ctrl Pts',(49.9225413218171,247.423039035993,31.5613203435596)) ;
#82975=CARTESIAN_POINT('Ctrl Pts',(50.044415803444,247.291066067091,31.9213203435596)) ;
#82976=CARTESIAN_POINT('Ctrl Pts',(50.044415803444,247.291066067091,31.5613203435596)) ;
#82977=CARTESIAN_POINT('Ctrl Pts',(50.1048968673761,247.225573558217,31.9213203435596)) ;
#82978=CARTESIAN_POINT('Ctrl Pts',(50.1048968673761,247.225573558217,31.5613203435596)) ;
#82979=CARTESIAN_POINT('',(49.8975299240168,247.692149180776,31.9213203435596)) ;
#82980=CARTESIAN_POINT('Ctrl Pts',(50.003941798311,248.05231292904,31.9213203435596)) ;
#82981=CARTESIAN_POINT('Ctrl Pts',(50.003941798311,248.05231292904,31.5613203435596)) ;
#82982=CARTESIAN_POINT('Ctrl Pts',(49.9729051299706,247.995865679917,31.9213203435596)) ;
#82983=CARTESIAN_POINT('Ctrl Pts',(49.9729051299706,247.995865679917,31.5613203435596)) ;
#82984=CARTESIAN_POINT('Ctrl Pts',(49.9111525355836,247.883554524574,31.9213203435596)) ;
#82985=CARTESIAN_POINT('Ctrl Pts',(49.9111525355836,247.883554524574,31.5613203435596)) ;
#82986=CARTESIAN_POINT('Ctrl Pts',(49.9020550437817,247.755729655054,31.9213203435596)) ;
#82987=CARTESIAN_POINT('Ctrl Pts',(49.9020550437817,247.755729655054,31.5613203435596)) ;
#82988=CARTESIAN_POINT('Ctrl Pts',(49.8975299240168,247.692149180776,31.9213203435596)) ;
#82989=CARTESIAN_POINT('Ctrl Pts',(49.8975299240168,247.692149180776,31.5613203435596)) ;
#82990=CARTESIAN_POINT('',(50.003941798311,248.05231292904,31.9213203435596)) ;
#82991=CARTESIAN_POINT('Ctrl Pts',(50.3149922133501,248.292422193891,31.9213203435596)) ;
#82992=CARTESIAN_POINT('Ctrl Pts',(50.3149922133501,248.292422193891,31.5613203435596)) ;
#82993=CARTESIAN_POINT('Ctrl Pts',(50.2514495790856,248.264187481871,31.9213203435596)) ;
#82994=CARTESIAN_POINT('Ctrl Pts',(50.2514495790856,248.264187481871,31.5613203435596)) ;
#82995=CARTESIAN_POINT('Ctrl Pts',(50.1280938441034,248.20937524921,31.9213203435596)) ;
#82996=CARTESIAN_POINT('Ctrl Pts',(50.1280938441034,248.20937524921,31.5613203435596)) ;
#82997=CARTESIAN_POINT('Ctrl Pts',(50.044483186211,248.103601044398,31.9213203435596)) ;
#82998=CARTESIAN_POINT('Ctrl Pts',(50.044483186211,248.103601044398,31.5613203435596)) ;
#82999=CARTESIAN_POINT('Ctrl Pts',(50.003941798311,248.05231292904,31.9213203435596)) ;
#83000=CARTESIAN_POINT('Ctrl Pts',(50.003941798311,248.05231292904,31.5613203435596)) ;
#83001=CARTESIAN_POINT('Ctrl Pts',(49.6274070383127,248.40974827469,31.9213203435596)) ;
#83002=CARTESIAN_POINT('Ctrl Pts',(49.6274070383127,248.40974827469,31.5613203435596)) ;
#83003=CARTESIAN_POINT('Ctrl Pts',(49.7398143320343,248.499112212212,31.9213203435596)) ;
#83004=CARTESIAN_POINT('Ctrl Pts',(49.7398143320343,248.499112212212,31.5613203435596)) ;
#83005=CARTESIAN_POINT('Ctrl Pts',(49.9894578389715,248.697579108959,31.9213203435596)) ;
#83006=CARTESIAN_POINT('Ctrl Pts',(49.9894578389715,248.697579108959,31.5613203435596)) ;
#83007=CARTESIAN_POINT('Ctrl Pts',(50.3051550779305,248.751296136815,31.9213203435596)) ;
#83008=CARTESIAN_POINT('Ctrl Pts',(50.3051550779305,248.751296136815,31.5613203435596)) ;
#83009=CARTESIAN_POINT('Ctrl Pts',(50.4787029267366,248.780825931436,31.9213203435596)) ;
#83010=CARTESIAN_POINT('Ctrl Pts',(50.4787029267366,248.780825931436,31.5613203435596)) ;
#83011=CARTESIAN_POINT('Origin',(75.7500000000001,218.,29.7213203435596)) ;
#83012=CARTESIAN_POINT('',(73.7500000000001,218.,29.7213203435596)) ;
#83013=CARTESIAN_POINT('',(77.7500000000001,218.,29.7213203435596)) ;
#83014=CARTESIAN_POINT('Origin',(75.7500000000001,218.,29.7213203435596)) ;
#83015=CARTESIAN_POINT('',(77.8500000000001,218.,29.6213203435596)) ;
#83016=CARTESIAN_POINT('Origin',(77.8500000000001,218.,29.7213203435596)) ;
#83017=CARTESIAN_POINT('Origin',(75.7500000000001,218.,29.6213203435596)) ;
#83018=CARTESIAN_POINT('Origin',(75.7500000000001,218.,29.7213203435596)) ;
#83019=CARTESIAN_POINT('Origin',(75.7500000000001,218.,29.6213203435596)) ;
#83020=CARTESIAN_POINT('',(72.8500000000001,218.,29.6213203435596)) ;
#83021=CARTESIAN_POINT('Origin',(75.7500000000001,218.,29.6213203435596)) ;
#83022=CARTESIAN_POINT('Origin',(75.7500000000001,218.,19.9213203435596)) ;
#83023=CARTESIAN_POINT('',(73.7500000000001,218.,30.1213203435596)) ;
#83024=CARTESIAN_POINT('',(73.7500000000001,218.,19.9213203435596)) ;
#83025=CARTESIAN_POINT('Origin',(75.7500000000001,218.,30.1213203435596)) ;
#83026=CARTESIAN_POINT('Origin',(75.7500000000001,218.,29.7213203435596)) ;
#83027=CARTESIAN_POINT('',(72.7500000000001,218.,29.7213203435596)) ;
#83028=CARTESIAN_POINT('Origin',(75.7500000000001,218.,29.7213203435596)) ;
#83029=CARTESIAN_POINT('Origin',(72.8500000000001,218.,29.7213203435596)) ;
#83030=CARTESIAN_POINT('Origin',(75.7500000000001,218.,28.9213203435596)) ;
#83031=CARTESIAN_POINT('',(72.7500000000001,218.,30.6213203435596)) ;
#83032=CARTESIAN_POINT('Origin',(75.7500000000001,218.,30.6213203435596)) ;
#83033=CARTESIAN_POINT('',(72.7500000000001,218.,28.9213203435596)) ;
#83034=CARTESIAN_POINT('Origin',(75.7500000000001,218.,30.6213203435596)) ;
#83035=CARTESIAN_POINT('',(72.6500000000001,218.,30.7213203435596)) ;
#83036=CARTESIAN_POINT('Origin',(75.7500000000001,218.,30.7213203435596)) ;
#83037=CARTESIAN_POINT('Origin',(72.6500000000001,218.,30.6213203435596)) ;
#83038=CARTESIAN_POINT('Origin',(53.7,239.383507185188,30.7213203435596)) ;
#83039=CARTESIAN_POINT('',(28.1267949192431,263.4,30.7213203435596)) ;
#83040=CARTESIAN_POINT('',(26.3,263.4,30.7213203435596)) ;
#83041=CARTESIAN_POINT('',(66.4499999999999,263.4,30.7213203435596)) ;
#83042=CARTESIAN_POINT('',(28.1,263.3,30.7213203435596)) ;
#83043=CARTESIAN_POINT('Origin',(28.3,263.3,30.7213203435596)) ;
#83044=CARTESIAN_POINT('',(28.1,262.3,30.7213203435596)) ;
#83045=CARTESIAN_POINT('',(28.1,251.391753592594,30.7213203435596)) ;
#83046=CARTESIAN_POINT('',(28.2,262.3,30.7213203435596)) ;
#83047=CARTESIAN_POINT('',(41.45,262.3,30.7213203435596)) ;
#83048=CARTESIAN_POINT('',(28.1999999999999,259.5,30.7213203435596)) ;
#83049=CARTESIAN_POINT('',(28.1999999999999,251.391753592594,30.7213203435596)) ;
#83050=CARTESIAN_POINT('',(28.1999999999999,258.3,30.7213203435596)) ;
#83051=CARTESIAN_POINT('',(28.1999999999999,251.391753592594,30.7213203435596)) ;
#83052=CARTESIAN_POINT('',(32.3585786437627,258.3,30.7213203435596)) ;
#83053=CARTESIAN_POINT('',(40.95,258.3,30.7213203435596)) ;
#83054=CARTESIAN_POINT('',(32.5,258.358578643763,30.7213203435596)) ;
#83055=CARTESIAN_POINT('Origin',(32.3585786437627,258.5,30.7213203435596)) ;
#83056=CARTESIAN_POINT('',(33.2414213562373,259.1,30.7213203435596)) ;
#83057=CARTESIAN_POINT('',(33.2415874744158,259.100166118179,30.7213203435596)) ;
#83058=CARTESIAN_POINT('',(33.3,259.241421356237,30.7213203435596)) ;
#83059=CARTESIAN_POINT('Origin',(33.1,259.241421356237,30.7213203435596)) ;
#83060=CARTESIAN_POINT('',(33.2999999999999,262.558578643763,30.7213203435596)) ;
#83061=CARTESIAN_POINT('',(33.2999999999999,248.891753592594,30.7213203435596)) ;
#83062=CARTESIAN_POINT('',(33.2414213562373,262.7,30.7213203435596)) ;
#83063=CARTESIAN_POINT('Origin',(33.1,262.558578643763,30.7213203435596)) ;
#83064=CARTESIAN_POINT('',(32.5414213562372,263.4,30.7213203435596)) ;
#83065=CARTESIAN_POINT('',(43.9998338818216,251.941587474416,30.7213203435596)) ;
#83066=CARTESIAN_POINT('',(46.2376487793589,263.4,30.7213203435596)) ;
#83067=CARTESIAN_POINT('',(66.4499999999999,263.4,30.7213203435596)) ;
#83068=CARTESIAN_POINT('',(47.9,262.026327083856,30.7213203435596)) ;
#83069=CARTESIAN_POINT('Origin',(47.9,263.763591785235,30.7213203435596)) ;
#83070=CARTESIAN_POINT('',(54.5,262.026327083856,30.7213203435596)) ;
#83071=CARTESIAN_POINT('',(53.4,262.026327083856,30.7213203435596)) ;
#83072=CARTESIAN_POINT('',(56.2,263.763591785235,30.7213203435596)) ;
#83073=CARTESIAN_POINT('Origin',(54.5,263.763591785235,30.7213203435596)) ;
#83074=CARTESIAN_POINT('',(56.2,263.8,30.7213203435596)) ;
#83075=CARTESIAN_POINT('',(56.2,252.191753592594,30.7213203435596)) ;
#83076=CARTESIAN_POINT('',(68.2,263.8,30.7213203435596)) ;
#83077=CARTESIAN_POINT('',(66.4499999999999,263.8,30.7213203435596)) ;
#83078=CARTESIAN_POINT('',(68.2,263.763591785235,30.7213203435596)) ;
#83079=CARTESIAN_POINT('',(68.2,251.191753592594,30.7213203435596)) ;
#83080=CARTESIAN_POINT('',(69.9,262.026327083856,30.7213203435596)) ;
#83081=CARTESIAN_POINT('Origin',(69.9,263.763591785235,30.7213203435596)) ;
#83082=CARTESIAN_POINT('',(76.5,262.026327083856,30.7213203435596)) ;
#83083=CARTESIAN_POINT('',(64.4,262.026327083856,30.7213203435596)) ;
#83084=CARTESIAN_POINT('',(78.162351220641,263.4,30.7213203435596)) ;
#83085=CARTESIAN_POINT('Origin',(76.5,263.763591785235,30.7213203435596)) ;
#83086=CARTESIAN_POINT('',(79.0999999999999,263.4,30.7213203435596)) ;
#83087=CARTESIAN_POINT('',(66.4499999999999,263.4,30.7213203435596)) ;
#83088=CARTESIAN_POINT('',(79.0999999999999,259.648528137424,30.7213203435596)) ;
#83089=CARTESIAN_POINT('',(79.0999999999999,249.391753592594,30.7213203435596)) ;
#83090=CARTESIAN_POINT('',(79.3050252531694,259.153553390593,30.7213203435596)) ;
#83091=CARTESIAN_POINT('Origin',(79.7999999999999,259.648528137424,30.7213203435596)) ;
#83092=CARTESIAN_POINT('',(80.9535533905932,257.50502525317,30.7213203435596)) ;
#83093=CARTESIAN_POINT('',(78.758412525583,259.70016611818,30.7213203435596)) ;
#83094=CARTESIAN_POINT('',(81.1,257.151471862576,30.7213203435596)) ;
#83095=CARTESIAN_POINT('Origin',(80.6,257.151471862576,30.7213203435596)) ;
#83096=CARTESIAN_POINT('',(81.1,247.098386676966,30.7213203435596)) ;
#83097=CARTESIAN_POINT('',(81.1,242.941753592594,30.7213203435596)) ;
#83098=CARTESIAN_POINT('',(80.616129032258,246.598646890358,30.7213203435596)) ;
#83099=CARTESIAN_POINT('Origin',(80.6,247.098386676966,30.7213203435596)) ;
#83100=CARTESIAN_POINT('',(78.0999999999999,244.,30.7213203435596)) ;
#83101=CARTESIAN_POINT('Origin',(80.6999999999999,244.,30.7213203435596)) ;
#83102=CARTESIAN_POINT('',(78.1,240.,30.7213203435596)) ;
#83103=CARTESIAN_POINT('',(78.1,239.691753592594,30.7213203435596)) ;
#83104=CARTESIAN_POINT('',(80.616129032258,237.401353109641,30.7213203435596)) ;
#83105=CARTESIAN_POINT('Origin',(80.6999999999999,240.,30.7213203435596)) ;
#83106=CARTESIAN_POINT('',(81.1,236.901613323034,30.7213203435596)) ;
#83107=CARTESIAN_POINT('Origin',(80.6,236.901613323034,30.7213203435596)) ;
#83108=CARTESIAN_POINT('',(81.1,226.002365511524,30.7213203435596)) ;
#83109=CARTESIAN_POINT('',(81.1,232.568672279644,30.7213203435596)) ;
#83110=CARTESIAN_POINT('',(80.9535533905933,225.64881212093,30.7213203435596)) ;
#83111=CARTESIAN_POINT('Origin',(80.6,226.002365511524,30.7213203435596)) ;
#83112=CARTESIAN_POINT('',(80.1050252531695,224.800283983507,30.7213203435596)) ;
#83113=CARTESIAN_POINT('',(77.061706774654,221.756965504991,30.7213203435596)) ;
#83114=CARTESIAN_POINT('',(79.9000000000001,224.305309236676,30.7213203435596)) ;
#83115=CARTESIAN_POINT('Origin',(80.6000000000001,224.305309236676,30.7213203435596)) ;
#83116=CARTESIAN_POINT('',(79.9000000000001,217.767014370377,30.7213203435596)) ;
#83117=CARTESIAN_POINT('',(79.9,228.575260777783,30.7213203435596)) ;
#83118=CARTESIAN_POINT('',(75.3227721070991,213.926264133629,30.7213203435596)) ;
#83119=CARTESIAN_POINT('Origin',(76.0000000000001,217.767014370377,30.7213203435596)) ;
#83120=CARTESIAN_POINT('',(63.8058825236653,215.957002501029,30.7213203435596)) ;
#83121=CARTESIAN_POINT('',(56.086380506565,217.318158984277,30.7213203435596)) ;
#83122=CARTESIAN_POINT('',(61.2884174438392,217.560804636007,30.7213203435596)) ;
#83123=CARTESIAN_POINT('Origin',(64.4831104165663,219.797752737776,30.7213203435596)) ;
#83124=CARTESIAN_POINT('',(56.7626663401537,224.024247053747,30.7213203435596)) ;
#83125=CARTESIAN_POINT('',(52.288931387286,230.413402709377,30.7213203435596)) ;
#83126=CARTESIAN_POINT('',(56.0573593128808,226.261195155516,30.7213203435596)) ;
#83127=CARTESIAN_POINT('Origin',(59.9573593128808,226.261195155516,30.7213203435596)) ;
#83128=CARTESIAN_POINT('',(56.0573593128807,244.4,30.7213203435596)) ;
#83129=CARTESIAN_POINT('',(56.0573593128807,242.191753592594,30.7213203435596)) ;
#83130=CARTESIAN_POINT('',(55.3573593128808,245.1,30.7213203435596)) ;
#83131=CARTESIAN_POINT('Origin',(55.3573593128808,244.4,30.7213203435596)) ;
#83132=CARTESIAN_POINT('',(46.8,245.1,30.7213203435596)) ;
#83133=CARTESIAN_POINT('',(39.95,245.1,30.7213203435596)) ;
#83134=CARTESIAN_POINT('',(46.2999999999999,245.6,30.7213203435596)) ;
#83135=CARTESIAN_POINT('Origin',(46.8,245.6,30.7213203435596)) ;
#83136=CARTESIAN_POINT('',(46.3,248.9,30.7213203435596)) ;
#83137=CARTESIAN_POINT('',(46.2999999999999,242.191753592594,30.7213203435596)) ;
#83138=CARTESIAN_POINT('',(46.1267949192431,249.,30.7213203435596)) ;
#83139=CARTESIAN_POINT('Ctrl Pts',(46.1267949192431,249.,30.7213203435596)) ;
#83140=CARTESIAN_POINT('Ctrl Pts',(46.1522826614307,249.,30.7213203435596)) ;
#83141=CARTESIAN_POINT('Ctrl Pts',(46.1815269526849,248.99104280001,30.7213203435596)) ;
#83142=CARTESIAN_POINT('Ctrl Pts',(46.2384776727796,248.960391271619,30.7213203435596)) ;
#83143=CARTESIAN_POINT('Ctrl Pts',(46.2722901777919,248.927709822208,30.7213203435596)) ;
#83144=CARTESIAN_POINT('Ctrl Pts',(46.3,248.9,30.7213203435596)) ;
#83145=CARTESIAN_POINT('',(34.2732050807569,249.,30.7213203435596)) ;
#83146=CARTESIAN_POINT('',(49.95,249.,30.7213203435596)) ;
#83147=CARTESIAN_POINT('',(34.1,248.9,30.7213203435596)) ;
#83148=CARTESIAN_POINT('Ctrl Pts',(34.1,248.9,30.7213203435596)) ;
#83149=CARTESIAN_POINT('Ctrl Pts',(34.1277098222081,248.927709822208,30.7213203435596)) ;
#83150=CARTESIAN_POINT('Ctrl Pts',(34.1615223272204,248.960391271619,30.7213203435596)) ;
#83151=CARTESIAN_POINT('Ctrl Pts',(34.2184730473151,248.99104280001,30.7213203435596)) ;
#83152=CARTESIAN_POINT('Ctrl Pts',(34.2477173385693,249.,30.7213203435596)) ;
#83153=CARTESIAN_POINT('Ctrl Pts',(34.2732050807569,249.,30.7213203435596)) ;
#83154=CARTESIAN_POINT('',(34.1,245.6,30.7213203435596)) ;
#83155=CARTESIAN_POINT('',(34.1000000000001,244.191753592594,30.7213203435596)) ;
#83156=CARTESIAN_POINT('',(33.6,245.1,30.7213203435596)) ;
#83157=CARTESIAN_POINT('Origin',(33.6,245.6,30.7213203435596)) ;
#83158=CARTESIAN_POINT('',(26.8,245.1,30.7213203435596)) ;
#83159=CARTESIAN_POINT('',(39.95,245.1,30.7213203435596)) ;
#83160=CARTESIAN_POINT('',(26.3,245.6,30.7213203435596)) ;
#83161=CARTESIAN_POINT('Origin',(26.8,245.6,30.7213203435596)) ;
#83162=CARTESIAN_POINT('',(26.3,252.191753592594,30.7213203435596)) ;
#83163=CARTESIAN_POINT('',(69.2,257.,30.7213203435596)) ;
#83164=CARTESIAN_POINT('Origin',(73.2,257.,30.7213203435596)) ;
#83165=CARTESIAN_POINT('',(74.2999999999999,226.1,30.7213203435596)) ;
#83166=CARTESIAN_POINT('',(74.3999999999999,226.1,30.7213203435596)) ;
#83167=CARTESIAN_POINT('',(64.1,226.1,30.7213203435596)) ;
#83168=CARTESIAN_POINT('',(74.2999999999999,231.9,30.7213203435596)) ;
#83169=CARTESIAN_POINT('',(74.2999999999999,232.691753592594,30.7213203435596)) ;
#83170=CARTESIAN_POINT('',(74.0999999999999,232.1,30.7213203435596)) ;
#83171=CARTESIAN_POINT('Origin',(74.0999999999999,231.9,30.7213203435596)) ;
#83172=CARTESIAN_POINT('',(71.8999999999999,232.1,30.7213203435596)) ;
#83173=CARTESIAN_POINT('',(63.95,232.1,30.7213203435596)) ;
#83174=CARTESIAN_POINT('',(71.6999999999999,231.9,30.7213203435596)) ;
#83175=CARTESIAN_POINT('Origin',(71.8999999999999,231.9,30.7213203435596)) ;
#83176=CARTESIAN_POINT('',(71.6999999999999,226.1,30.7213203435596)) ;
#83177=CARTESIAN_POINT('',(71.6999999999999,235.691753592594,30.7213203435596)) ;
#83178=CARTESIAN_POINT('',(71.5999999999999,226.1,30.7213203435596)) ;
#83179=CARTESIAN_POINT('',(62.75,226.1,30.7213203435596)) ;
#83180=CARTESIAN_POINT('',(71.3999999999999,225.9,30.7213203435596)) ;
#83181=CARTESIAN_POINT('Origin',(71.5999999999999,225.9,30.7213203435596)) ;
#83182=CARTESIAN_POINT('',(71.3999999999999,223.1,30.7213203435596)) ;
#83183=CARTESIAN_POINT('',(71.3999999999999,232.691753592594,30.7213203435596)) ;
#83184=CARTESIAN_POINT('',(71.5999999999999,222.9,30.7213203435596)) ;
#83185=CARTESIAN_POINT('Origin',(71.5999999999999,223.1,30.7213203435596)) ;
#83186=CARTESIAN_POINT('',(74.3999999999999,222.9,30.7213203435596)) ;
#83187=CARTESIAN_POINT('',(62.6,222.9,30.7213203435596)) ;
#83188=CARTESIAN_POINT('',(74.5999999999999,223.1,30.7213203435596)) ;
#83189=CARTESIAN_POINT('Origin',(74.3999999999999,223.1,30.7213203435596)) ;
#83190=CARTESIAN_POINT('',(74.6,225.9,30.7213203435596)) ;
#83191=CARTESIAN_POINT('',(74.5999999999999,231.191753592594,30.7213203435596)) ;
#83192=CARTESIAN_POINT('Origin',(74.3999999999999,225.9,30.7213203435596)) ;
#83193=CARTESIAN_POINT('',(28.1,254.8,30.7213203435596)) ;
#83194=CARTESIAN_POINT('Origin',(30.7,254.8,30.7213203435596)) ;
#83195=CARTESIAN_POINT('',(59.,261.2,30.7213203435596)) ;
#83196=CARTESIAN_POINT('Origin',(61.5,261.2,30.7213203435596)) ;
#83197=CARTESIAN_POINT('',(80.299999999999,252.4,30.7213203435596)) ;
#83198=CARTESIAN_POINT('',(80.199999999999,252.4,30.7213203435596)) ;
#83199=CARTESIAN_POINT('',(66.9499999999999,252.4,30.7213203435596)) ;
#83200=CARTESIAN_POINT('',(80.299999999999,253.4,30.7213203435596)) ;
#83201=CARTESIAN_POINT('',(80.2999999999989,243.941753592594,30.7213203435596)) ;
#83202=CARTESIAN_POINT('',(80.099999999999,253.6,30.7213203435596)) ;
#83203=CARTESIAN_POINT('Origin',(80.099999999999,253.4,30.7213203435596)) ;
#83204=CARTESIAN_POINT('',(76.0414213562367,253.6,30.7213203435596)) ;
#83205=CARTESIAN_POINT('',(66.9499999999995,253.6,30.7213203435596)) ;
#83206=CARTESIAN_POINT('',(75.8999999999994,253.541421356237,30.7213203435596)) ;
#83207=CARTESIAN_POINT('Origin',(76.0414213562367,253.4,30.7213203435596)) ;
#83208=CARTESIAN_POINT('',(75.1585786437621,252.8,30.7213203435596)) ;
#83209=CARTESIAN_POINT('',(66.6251661181778,244.266587474416,30.7213203435596)) ;
#83210=CARTESIAN_POINT('',(75.0999999999994,252.658578643763,30.7213203435596)) ;
#83211=CARTESIAN_POINT('Origin',(75.2999999999994,252.658578643763,30.7213203435596)) ;
#83212=CARTESIAN_POINT('',(75.0999999999993,249.341421356237,30.7213203435596)) ;
#83213=CARTESIAN_POINT('',(75.0999999999992,246.441753592594,30.7213203435596)) ;
#83214=CARTESIAN_POINT('',(75.158578643762,249.2,30.7213203435596)) ;
#83215=CARTESIAN_POINT('Origin',(75.2999999999993,249.341421356237,30.7213203435596)) ;
#83216=CARTESIAN_POINT('',(75.8999999999992,248.458578643763,30.7213203435596)) ;
#83217=CARTESIAN_POINT('',(72.4334125255833,251.925166118179,30.7213203435596)) ;
#83218=CARTESIAN_POINT('',(76.0414213562365,248.4,30.7213203435596)) ;
#83219=CARTESIAN_POINT('Origin',(76.0414213562365,248.6,30.7213203435596)) ;
#83220=CARTESIAN_POINT('',(80.0999999999989,248.4,30.7213203435596)) ;
#83221=CARTESIAN_POINT('',(64.4499999999996,248.4,30.7213203435596)) ;
#83222=CARTESIAN_POINT('',(80.2999999999989,248.6,30.7213203435596)) ;
#83223=CARTESIAN_POINT('Origin',(80.0999999999989,248.6,30.7213203435596)) ;
#83224=CARTESIAN_POINT('',(80.2999999999989,249.6,30.7213203435596)) ;
#83225=CARTESIAN_POINT('',(80.2999999999989,243.941753592594,30.7213203435596)) ;
#83226=CARTESIAN_POINT('',(80.1999999999999,249.6,30.7213203435596)) ;
#83227=CARTESIAN_POINT('',(66.4500000000001,249.6,30.7213203435596)) ;
#83228=CARTESIAN_POINT('',(80.1999999999989,243.941753592594,30.7213203435596)) ;
#83229=CARTESIAN_POINT('',(62.1568347953873,220.146231446812,30.7213203435596)) ;
#83230=CARTESIAN_POINT('Origin',(64.1568347953873,220.146231446812,30.7213203435596)) ;
#83231=CARTESIAN_POINT('',(80.099999999999,230.5,30.7213203435596)) ;
#83232=CARTESIAN_POINT('',(76.0414213562367,230.5,30.7213203435596)) ;
#83233=CARTESIAN_POINT('',(66.9499999999995,230.5,30.7213203435596)) ;
#83234=CARTESIAN_POINT('',(75.9707106781181,230.470710678119,30.7213203435596)) ;
#83235=CARTESIAN_POINT('Origin',(76.0414213562367,230.4,30.7213203435596)) ;
#83236=CARTESIAN_POINT('',(75.2292893218808,229.729289321881,30.7213203435596)) ;
#83237=CARTESIAN_POINT('',(72.4458767962964,226.945876796297,30.7213203435596)) ;
#83238=CARTESIAN_POINT('',(75.1999999999994,229.658578643763,30.7213203435596)) ;
#83239=CARTESIAN_POINT('Origin',(75.2999999999994,229.658578643763,30.7213203435596)) ;
#83240=CARTESIAN_POINT('',(75.1999999999993,226.341421356237,30.7213203435596)) ;
#83241=CARTESIAN_POINT('',(75.1999999999996,234.941753592594,30.7213203435596)) ;
#83242=CARTESIAN_POINT('',(75.2292893218806,226.270710678119,30.7213203435596)) ;
#83243=CARTESIAN_POINT('Origin',(75.2999999999993,226.341421356237,30.7213203435596)) ;
#83244=CARTESIAN_POINT('',(75.9707106781179,225.529289321881,30.7213203435596)) ;
#83245=CARTESIAN_POINT('',(66.7541232037024,234.745876796297,30.7213203435596)) ;
#83246=CARTESIAN_POINT('',(76.0414213562366,225.5,30.7213203435596)) ;
#83247=CARTESIAN_POINT('Origin',(76.0414213562366,225.6,30.7213203435596)) ;
#83248=CARTESIAN_POINT('',(80.0999999999989,225.5,30.7213203435596)) ;
#83249=CARTESIAN_POINT('',(64.4499999999996,225.5,30.7213203435596)) ;
#83250=CARTESIAN_POINT('',(80.199999999999,225.6,30.7213203435596)) ;
#83251=CARTESIAN_POINT('Origin',(80.0999999999989,225.6,30.7213203435596)) ;
#83252=CARTESIAN_POINT('',(80.199999999999,226.6,30.7213203435596)) ;
#83253=CARTESIAN_POINT('',(80.199999999999,232.441753592594,30.7213203435596)) ;
#83254=CARTESIAN_POINT('',(80.199999999999,229.4,30.7213203435596)) ;
#83255=CARTESIAN_POINT('',(80.199999999999,232.441753592594,30.7213203435596)) ;
#83256=CARTESIAN_POINT('',(80.199999999999,230.4,30.7213203435596)) ;
#83257=CARTESIAN_POINT('',(80.199999999999,232.441753592594,30.7213203435596)) ;
#83258=CARTESIAN_POINT('Origin',(80.099999999999,230.4,30.7213203435596)) ;
#83259=CARTESIAN_POINT('',(37.0999999999999,259.9,30.7213203435596)) ;
#83260=CARTESIAN_POINT('',(37.2999999999999,260.1,30.7213203435596)) ;
#83261=CARTESIAN_POINT('Origin',(37.2999999999999,259.9,30.7213203435596)) ;
#83262=CARTESIAN_POINT('',(37.0999999999999,252.1,30.7213203435596)) ;
#83263=CARTESIAN_POINT('',(37.0999999999999,249.691753592594,30.7213203435596)) ;
#83264=CARTESIAN_POINT('',(37.2999999999999,251.9,30.7213203435596)) ;
#83265=CARTESIAN_POINT('Origin',(37.2999999999999,252.1,30.7213203435596)) ;
#83266=CARTESIAN_POINT('',(43.0999999999999,251.9,30.7213203435596)) ;
#83267=CARTESIAN_POINT('',(45.4499999999999,251.9,30.7213203435596)) ;
#83268=CARTESIAN_POINT('',(43.2999999999999,252.1,30.7213203435596)) ;
#83269=CARTESIAN_POINT('Origin',(43.0999999999999,252.1,30.7213203435596)) ;
#83270=CARTESIAN_POINT('',(43.2999999999999,259.9,30.7213203435596)) ;
#83271=CARTESIAN_POINT('',(43.2999999999999,245.691753592594,30.7213203435596)) ;
#83272=CARTESIAN_POINT('',(43.0999999999999,260.1,30.7213203435596)) ;
#83273=CARTESIAN_POINT('Origin',(43.0999999999999,259.9,30.7213203435596)) ;
#83274=CARTESIAN_POINT('',(48.4499999999999,260.1,30.7213203435596)) ;
#83275=CARTESIAN_POINT('',(57.9573593128807,242.926794919243,30.7213203435596)) ;
#83276=CARTESIAN_POINT('',(57.9573593128807,241.9,30.7213203435596)) ;
#83277=CARTESIAN_POINT('',(57.9573593128807,241.191753592594,30.7213203435596)) ;
#83278=CARTESIAN_POINT('',(57.9573593128807,239.1,30.7213203435596)) ;
#83279=CARTESIAN_POINT('',(57.9573593128807,241.191753592594,30.7213203435596)) ;
#83280=CARTESIAN_POINT('',(57.9573593128807,238.073205080757,30.7213203435596)) ;
#83281=CARTESIAN_POINT('',(57.9573593128807,241.191753592594,30.7213203435596)) ;
#83282=CARTESIAN_POINT('',(58.0573593128808,237.9,30.7213203435596)) ;
#83283=CARTESIAN_POINT('Ctrl Pts',(58.0573593128808,237.9,30.7213203435596)) ;
#83284=CARTESIAN_POINT('Ctrl Pts',(58.0296494906727,237.927709822208,30.7213203435596)) ;
#83285=CARTESIAN_POINT('Ctrl Pts',(57.9969680412619,237.96152232722,30.7213203435596)) ;
#83286=CARTESIAN_POINT('Ctrl Pts',(57.9663165128706,238.018473047315,30.7213203435596)) ;
#83287=CARTESIAN_POINT('Ctrl Pts',(57.9573593128808,238.047717338569,30.7213203435596)) ;
#83288=CARTESIAN_POINT('Ctrl Pts',(57.9573593128808,238.073205080757,30.7213203435596)) ;
#83289=CARTESIAN_POINT('',(62.1159379566435,237.9,30.7213203435596)) ;
#83290=CARTESIAN_POINT('',(55.8286796564404,237.9,30.7213203435596)) ;
#83291=CARTESIAN_POINT('',(62.2573593128808,237.958578643763,30.7213203435596)) ;
#83292=CARTESIAN_POINT('Origin',(62.1159379566435,238.1,30.7213203435596)) ;
#83293=CARTESIAN_POINT('',(62.998780669118,238.7,30.7213203435596)) ;
#83294=CARTESIAN_POINT('',(60.6596069590762,236.360826289958,30.7213203435596)) ;
#83295=CARTESIAN_POINT('',(63.0573593128808,238.841421356237,30.7213203435596)) ;
#83296=CARTESIAN_POINT('Origin',(62.8573593128807,238.841421356237,30.7213203435596)) ;
#83297=CARTESIAN_POINT('',(63.0573593128807,242.158578643763,30.7213203435596)) ;
#83298=CARTESIAN_POINT('',(63.0573593128807,238.691753592594,30.7213203435596)) ;
#83299=CARTESIAN_POINT('',(62.9987806691181,242.3,30.7213203435596)) ;
#83300=CARTESIAN_POINT('Origin',(62.8573593128807,242.158578643763,30.7213203435596)) ;
#83301=CARTESIAN_POINT('',(62.2573593128808,243.041421356237,30.7213203435596)) ;
#83302=CARTESIAN_POINT('',(61.2178533664821,244.080927302636,30.7213203435596)) ;
#83303=CARTESIAN_POINT('',(62.1159379566435,243.1,30.7213203435596)) ;
#83304=CARTESIAN_POINT('Origin',(62.1159379566435,242.9,30.7213203435596)) ;
#83305=CARTESIAN_POINT('',(58.0573593128808,243.1,30.7213203435596)) ;
#83306=CARTESIAN_POINT('',(58.3286796564404,243.1,30.7213203435596)) ;
#83307=CARTESIAN_POINT('Ctrl Pts',(57.9573593128808,242.926794919243,30.7213203435596)) ;
#83308=CARTESIAN_POINT('Ctrl Pts',(57.9573593128808,242.952282661431,30.7213203435596)) ;
#83309=CARTESIAN_POINT('Ctrl Pts',(57.9663165128706,242.981526952685,30.7213203435596)) ;
#83310=CARTESIAN_POINT('Ctrl Pts',(57.9969680412619,243.03847767278,30.7213203435596)) ;
#83311=CARTESIAN_POINT('Ctrl Pts',(58.0296494906727,243.072290177792,30.7213203435596)) ;
#83312=CARTESIAN_POINT('Ctrl Pts',(58.0573593128808,243.1,30.7213203435596)) ;
#83313=CARTESIAN_POINT('',(62.2841542321239,236.,30.7213203435596)) ;
#83314=CARTESIAN_POINT('',(60.0305643936376,236.,30.7213203435596)) ;
#83315=CARTESIAN_POINT('',(58.0286796564404,236.,30.7213203435596)) ;
#83316=CARTESIAN_POINT('',(59.8573593128808,235.9,30.7213203435596)) ;
#83317=CARTESIAN_POINT('Ctrl Pts',(59.8573593128808,235.9,30.7213203435596)) ;
#83318=CARTESIAN_POINT('Ctrl Pts',(59.8850691350889,235.927709822208,30.7213203435596)) ;
#83319=CARTESIAN_POINT('Ctrl Pts',(59.9188816401012,235.960391271619,30.7213203435596)) ;
#83320=CARTESIAN_POINT('Ctrl Pts',(59.9758323601959,235.99104280001,30.7213203435596)) ;
#83321=CARTESIAN_POINT('Ctrl Pts',(60.0050766514501,236.,30.7213203435596)) ;
#83322=CARTESIAN_POINT('Ctrl Pts',(60.0305643936377,236.,30.7213203435596)) ;
#83323=CARTESIAN_POINT('',(59.8573593128808,230.1,30.7213203435596)) ;
#83324=CARTESIAN_POINT('',(59.8573593128808,237.691753592594,30.7213203435596)) ;
#83325=CARTESIAN_POINT('',(59.7573593128808,230.1,30.7213203435596)) ;
#83326=CARTESIAN_POINT('',(56.8286796564404,230.1,30.7213203435596)) ;
#83327=CARTESIAN_POINT('',(59.5573593128808,229.9,30.7213203435596)) ;
#83328=CARTESIAN_POINT('Origin',(59.7573593128808,229.9,30.7213203435596)) ;
#83329=CARTESIAN_POINT('',(59.5573593128808,227.1,30.7213203435596)) ;
#83330=CARTESIAN_POINT('',(59.5573593128808,234.691753592594,30.7213203435596)) ;
#83331=CARTESIAN_POINT('',(59.7573593128808,226.9,30.7213203435596)) ;
#83332=CARTESIAN_POINT('Origin',(59.7573593128808,227.1,30.7213203435596)) ;
#83333=CARTESIAN_POINT('',(62.5573593128808,226.9,30.7213203435596)) ;
#83334=CARTESIAN_POINT('',(56.6786796564404,226.9,30.7213203435596)) ;
#83335=CARTESIAN_POINT('',(62.7573593128808,227.1,30.7213203435596)) ;
#83336=CARTESIAN_POINT('Origin',(62.5573593128808,227.1,30.7213203435596)) ;
#83337=CARTESIAN_POINT('',(62.7573593128808,229.9,30.7213203435596)) ;
#83338=CARTESIAN_POINT('',(62.7573593128808,233.191753592594,30.7213203435596)) ;
#83339=CARTESIAN_POINT('',(62.5573593128808,230.1,30.7213203435596)) ;
#83340=CARTESIAN_POINT('Origin',(62.5573593128808,229.9,30.7213203435596)) ;
#83341=CARTESIAN_POINT('',(62.4573593128808,230.1,30.7213203435596)) ;
#83342=CARTESIAN_POINT('',(58.1786796564404,230.1,30.7213203435596)) ;
#83343=CARTESIAN_POINT('',(62.4573593128808,235.9,30.7213203435596)) ;
#83344=CARTESIAN_POINT('',(62.4573593128808,234.691753592594,30.7213203435596)) ;
#83345=CARTESIAN_POINT('Ctrl Pts',(62.2841542321239,236.,30.7213203435596)) ;
#83346=CARTESIAN_POINT('Ctrl Pts',(62.3096419743115,236.,30.7213203435596)) ;
#83347=CARTESIAN_POINT('Ctrl Pts',(62.3388862655657,235.99104280001,30.7213203435596)) ;
#83348=CARTESIAN_POINT('Ctrl Pts',(62.3958369856604,235.960391271619,30.7213203435596)) ;
#83349=CARTESIAN_POINT('Ctrl Pts',(62.4296494906727,235.927709822208,30.7213203435596)) ;
#83350=CARTESIAN_POINT('Ctrl Pts',(62.4573593128808,235.9,30.7213203435596)) ;
#83351=CARTESIAN_POINT('',(56.3,250.9,30.7213203435596)) ;
#83352=CARTESIAN_POINT('',(56.5,251.1,30.7213203435596)) ;
#83353=CARTESIAN_POINT('Origin',(56.5,250.9,30.7213203435596)) ;
#83354=CARTESIAN_POINT('',(56.3,248.1,30.7213203435596)) ;
#83355=CARTESIAN_POINT('',(56.3,245.191753592594,30.7213203435596)) ;
#83356=CARTESIAN_POINT('',(56.5,247.9,30.7213203435596)) ;
#83357=CARTESIAN_POINT('Origin',(56.5,248.1,30.7213203435596)) ;
#83358=CARTESIAN_POINT('',(59.3,247.9,30.7213203435596)) ;
#83359=CARTESIAN_POINT('',(55.05,247.9,30.7213203435596)) ;
#83360=CARTESIAN_POINT('',(59.5,248.1,30.7213203435596)) ;
#83361=CARTESIAN_POINT('Origin',(59.3,248.1,30.7213203435596)) ;
#83362=CARTESIAN_POINT('',(59.5,250.9,30.7213203435596)) ;
#83363=CARTESIAN_POINT('',(59.5,243.691753592594,30.7213203435596)) ;
#83364=CARTESIAN_POINT('',(59.3,251.1,30.7213203435596)) ;
#83365=CARTESIAN_POINT('Origin',(59.3,250.9,30.7213203435596)) ;
#83366=CARTESIAN_POINT('',(59.2,251.1,30.7213203435596)) ;
#83367=CARTESIAN_POINT('',(56.55,251.1,30.7213203435596)) ;
#83368=CARTESIAN_POINT('',(59.2,256.9,30.7213203435596)) ;
#83369=CARTESIAN_POINT('',(59.2,245.191753592594,30.7213203435596)) ;
#83370=CARTESIAN_POINT('',(59.,257.1,30.7213203435596)) ;
#83371=CARTESIAN_POINT('Origin',(59.,256.9,30.7213203435596)) ;
#83372=CARTESIAN_POINT('',(56.8,257.1,30.7213203435596)) ;
#83373=CARTESIAN_POINT('',(56.4,257.1,30.7213203435596)) ;
#83374=CARTESIAN_POINT('',(56.6,256.9,30.7213203435596)) ;
#83375=CARTESIAN_POINT('Origin',(56.8,256.9,30.7213203435596)) ;
#83376=CARTESIAN_POINT('',(56.6,251.1,30.7213203435596)) ;
#83377=CARTESIAN_POINT('',(56.6,248.191753592594,30.7213203435596)) ;
#83378=CARTESIAN_POINT('',(55.2,251.1,30.7213203435596)) ;
#83379=CARTESIAN_POINT('',(64.3,250.9,30.7213203435596)) ;
#83380=CARTESIAN_POINT('',(64.4999999999999,251.1,30.7213203435596)) ;
#83381=CARTESIAN_POINT('Origin',(64.4999999999999,250.9,30.7213203435596)) ;
#83382=CARTESIAN_POINT('',(64.3,248.1,30.7213203435596)) ;
#83383=CARTESIAN_POINT('',(64.3,245.191753592594,30.7213203435596)) ;
#83384=CARTESIAN_POINT('',(64.4999999999999,247.9,30.7213203435596)) ;
#83385=CARTESIAN_POINT('Origin',(64.4999999999999,248.1,30.7213203435596)) ;
#83386=CARTESIAN_POINT('',(67.3,247.9,30.7213203435596)) ;
#83387=CARTESIAN_POINT('',(59.05,247.9,30.7213203435596)) ;
#83388=CARTESIAN_POINT('',(67.5,248.1,30.7213203435596)) ;
#83389=CARTESIAN_POINT('Origin',(67.3,248.1,30.7213203435596)) ;
#83390=CARTESIAN_POINT('',(67.5,250.9,30.7213203435596)) ;
#83391=CARTESIAN_POINT('',(67.5,243.691753592594,30.7213203435596)) ;
#83392=CARTESIAN_POINT('',(67.3,251.1,30.7213203435596)) ;
#83393=CARTESIAN_POINT('Origin',(67.3,250.9,30.7213203435596)) ;
#83394=CARTESIAN_POINT('',(67.2,251.1,30.7213203435596)) ;
#83395=CARTESIAN_POINT('',(60.55,251.1,30.7213203435596)) ;
#83396=CARTESIAN_POINT('',(67.2,256.9,30.7213203435596)) ;
#83397=CARTESIAN_POINT('',(67.2,245.191753592594,30.7213203435596)) ;
#83398=CARTESIAN_POINT('',(67.,257.1,30.7213203435596)) ;
#83399=CARTESIAN_POINT('Origin',(67.,256.9,30.7213203435596)) ;
#83400=CARTESIAN_POINT('',(64.8,257.1,30.7213203435596)) ;
#83401=CARTESIAN_POINT('',(60.4,257.1,30.7213203435596)) ;
#83402=CARTESIAN_POINT('',(64.6,256.9,30.7213203435596)) ;
#83403=CARTESIAN_POINT('Origin',(64.8,256.9,30.7213203435596)) ;
#83404=CARTESIAN_POINT('',(64.6,251.1,30.7213203435596)) ;
#83405=CARTESIAN_POINT('',(64.6,248.191753592594,30.7213203435596)) ;
#83406=CARTESIAN_POINT('',(59.2,251.1,30.7213203435596)) ;
#83407=CARTESIAN_POINT('',(47.2001799037401,256.996752829339,30.7213203435596)) ;
#83408=CARTESIAN_POINT('Ctrl Pts',(47.2001799037401,256.996752829339,30.7213203435596)) ;
#83409=CARTESIAN_POINT('Ctrl Pts',(47.1996958934101,257.592950087367,30.7213203435596)) ;
#83410=CARTESIAN_POINT('Ctrl Pts',(47.4713258041952,258.790688157784,30.7213203435596)) ;
#83411=CARTESIAN_POINT('Ctrl Pts',(48.6193980168863,260.233005722467,30.7213203435596)) ;
#83412=CARTESIAN_POINT('Ctrl Pts',(50.2789716629066,261.032977199702,30.7213203435596)) ;
#83413=CARTESIAN_POINT('Ctrl Pts',(52.1193940511311,261.033737473045,30.7213203435596)) ;
#83414=CARTESIAN_POINT('Ctrl Pts',(53.7785648155242,260.233461912991,30.7213203435596)) ;
#83415=CARTESIAN_POINT('Ctrl Pts',(55.0559915567595,258.636262470822,30.7213203435596)) ;
#83416=CARTESIAN_POINT('Ctrl Pts',(55.305635860734,256.985238068826,30.7213203435596)) ;
#83417=CARTESIAN_POINT('Ctrl Pts',(55.0373399291364,255.821578804573,30.7213203435596)) ;
#83418=CARTESIAN_POINT('Ctrl Pts',(54.6764928726381,254.892517415637,30.7213203435596)) ;
#83419=CARTESIAN_POINT('Ctrl Pts',(53.7849806154459,253.771240925762,30.7213203435596)) ;
#83420=CARTESIAN_POINT('Ctrl Pts',(52.1281196619292,252.969136511964,30.7213203435596)) ;
#83421=CARTESIAN_POINT('Ctrl Pts',(50.2846657419234,252.967612937877,30.7213203435596)) ;
#83422=CARTESIAN_POINT('Ctrl Pts',(48.6260586034358,253.762867831118,30.7213203435596)) ;
#83423=CARTESIAN_POINT('Ctrl Pts',(47.4744091088858,255.204607859147,30.7213203435596)) ;
#83424=CARTESIAN_POINT('Ctrl Pts',(47.2006639140701,256.40055557131,30.7213203435596)) ;
#83425=CARTESIAN_POINT('Ctrl Pts',(47.2001799037401,256.996752829339,30.7213203435596)) ;
#83426=CARTESIAN_POINT('Origin',(26.3,263.4,30.3213203435596)) ;
#83427=CARTESIAN_POINT('',(26.2,263.9,30.3213203435596)) ;
#83428=CARTESIAN_POINT('',(26.3,263.8,30.3213203435596)) ;
#83429=CARTESIAN_POINT('Origin',(26.3,263.9,30.3213203435596)) ;
#83430=CARTESIAN_POINT('Origin',(26.3,263.4,30.3213203435596)) ;
#83431=CARTESIAN_POINT('',(26.2,263.4,30.8213203435596)) ;
#83432=CARTESIAN_POINT('Origin',(26.3,263.4,30.8213203435596)) ;
#83433=CARTESIAN_POINT('Origin',(26.2,263.4,30.3213203435596)) ;
#83434=CARTESIAN_POINT('Origin',(26.3,263.9,19.9213203435596)) ;
#83435=CARTESIAN_POINT('',(26.2,263.9,21.9213203435596)) ;
#83436=CARTESIAN_POINT('',(26.3,263.8,21.9213203435596)) ;
#83437=CARTESIAN_POINT('Origin',(26.3,263.9,21.9213203435596)) ;
#83438=CARTESIAN_POINT('',(26.3,263.8,19.9213203435596)) ;
#83439=CARTESIAN_POINT('',(26.2,263.9,19.9213203435596)) ;
#83440=CARTESIAN_POINT('Origin',(28.2,263.9,21.9213203435596)) ;
#83441=CARTESIAN_POINT('',(28.2,263.9,19.9213203435596)) ;
#83442=CARTESIAN_POINT('',(28.2,263.8,20.0213203435596)) ;
#83443=CARTESIAN_POINT('Origin',(28.2,263.9,20.0213203435596)) ;
#83444=CARTESIAN_POINT('Origin',(28.2,263.8,21.9213203435596)) ;
#83445=CARTESIAN_POINT('Origin',(28.2,263.9,21.9213203435596)) ;
#83446=CARTESIAN_POINT('Origin',(66.4499999999999,263.9,20.0213203435596)) ;
#83447=CARTESIAN_POINT('',(35.6,263.9,19.9213203435596)) ;
#83448=CARTESIAN_POINT('',(35.6,263.8,20.0213203435596)) ;
#83449=CARTESIAN_POINT('Origin',(35.6,263.9,20.0213203435596)) ;
#83450=CARTESIAN_POINT('',(66.4499999999999,263.8,20.0213203435596)) ;
#83451=CARTESIAN_POINT('',(66.4499999999999,263.9,19.9213203435596)) ;
#83452=CARTESIAN_POINT('Origin',(35.6,263.9,21.9213203435596)) ;
#83453=CARTESIAN_POINT('',(37.6,263.9,21.9213203435596)) ;
#83454=CARTESIAN_POINT('',(37.5,263.8,21.9213203435596)) ;
#83455=CARTESIAN_POINT('Origin',(37.5,263.9,21.9213203435596)) ;
#83456=CARTESIAN_POINT('Origin',(35.6,263.8,21.9213203435596)) ;
#83457=CARTESIAN_POINT('Origin',(35.6,263.9,21.9213203435596)) ;
#83458=CARTESIAN_POINT('Origin',(37.5,263.9,22.4713203435596)) ;
#83459=CARTESIAN_POINT('',(37.6,263.9,25.0213203435596)) ;
#83460=CARTESIAN_POINT('',(37.5,263.8,25.0213203435596)) ;
#83461=CARTESIAN_POINT('Origin',(37.5,263.9,25.0213203435596)) ;
#83462=CARTESIAN_POINT('',(37.5,263.8,22.4713203435596)) ;
#83463=CARTESIAN_POINT('',(37.6,263.9,22.4713203435596)) ;
#83464=CARTESIAN_POINT('Origin',(40.2,263.9,25.0213203435596)) ;
#83465=CARTESIAN_POINT('',(42.8,263.9,25.0213203435596)) ;
#83466=CARTESIAN_POINT('',(42.9,263.8,25.0213203435596)) ;
#83467=CARTESIAN_POINT('Origin',(42.9,263.9,25.0213203435596)) ;
#83468=CARTESIAN_POINT('Origin',(40.2,263.8,25.0213203435596)) ;
#83469=CARTESIAN_POINT('Origin',(40.2,263.9,25.0213203435596)) ;
#83470=CARTESIAN_POINT('Origin',(42.9,263.9,19.9213203435596)) ;
#83471=CARTESIAN_POINT('',(42.8,263.9,21.9213203435596)) ;
#83472=CARTESIAN_POINT('',(42.9,263.8,21.9213203435596)) ;
#83473=CARTESIAN_POINT('Origin',(42.9,263.9,21.9213203435596)) ;
#83474=CARTESIAN_POINT('',(42.9,263.8,19.9213203435596)) ;
#83475=CARTESIAN_POINT('',(42.8,263.9,19.9213203435596)) ;
#83476=CARTESIAN_POINT('Origin',(44.8,263.9,21.9213203435596)) ;
#83477=CARTESIAN_POINT('',(44.8,263.9,19.9213203435596)) ;
#83478=CARTESIAN_POINT('',(44.8,263.8,20.0213203435596)) ;
#83479=CARTESIAN_POINT('Origin',(44.8,263.9,20.0213203435596)) ;
#83480=CARTESIAN_POINT('Origin',(44.8,263.8,21.9213203435596)) ;
#83481=CARTESIAN_POINT('Origin',(44.8,263.9,21.9213203435596)) ;
#83482=CARTESIAN_POINT('Origin',(66.4499999999999,263.9,20.0213203435596)) ;
#83483=CARTESIAN_POINT('',(77.1999999999999,263.9,19.9213203435596)) ;
#83484=CARTESIAN_POINT('',(77.1999999999999,263.8,20.0213203435596)) ;
#83485=CARTESIAN_POINT('Origin',(77.1999999999999,263.9,20.0213203435596)) ;
#83486=CARTESIAN_POINT('',(66.4499999999999,263.8,20.0213203435596)) ;
#83487=CARTESIAN_POINT('',(66.4499999999999,263.9,19.9213203435596)) ;
#83488=CARTESIAN_POINT('Origin',(77.1999999999999,263.9,21.9213203435596)) ;
#83489=CARTESIAN_POINT('',(79.1999999999999,263.9,21.9213203435596)) ;
#83490=CARTESIAN_POINT('',(79.0999999999999,263.8,21.9213203435596)) ;
#83491=CARTESIAN_POINT('Origin',(79.0999999999999,263.9,21.9213203435596)) ;
#83492=CARTESIAN_POINT('Origin',(77.1999999999999,263.8,21.9213203435596)) ;
#83493=CARTESIAN_POINT('Origin',(77.1999999999999,263.9,21.9213203435596)) ;
#83494=CARTESIAN_POINT('Origin',(79.0999999999999,263.9,19.9213203435596)) ;
#83495=CARTESIAN_POINT('',(79.1999999999999,263.9,30.3213203435596)) ;
#83496=CARTESIAN_POINT('',(79.0999999999999,263.8,30.3213203435596)) ;
#83497=CARTESIAN_POINT('Origin',(79.0999999999999,263.9,30.3213203435596)) ;
#83498=CARTESIAN_POINT('',(79.0999999999999,263.8,19.9213203435596)) ;
#83499=CARTESIAN_POINT('',(79.1999999999999,263.9,19.9213203435596)) ;
#83500=CARTESIAN_POINT('Origin',(79.0999999999999,263.4,30.3213203435596)) ;
#83501=CARTESIAN_POINT('',(79.1999999999999,263.4,30.8213203435596)) ;
#83502=CARTESIAN_POINT('Origin',(79.1999999999999,263.4,30.3213203435596)) ;
#83503=CARTESIAN_POINT('Origin',(79.0999999999999,263.4,30.8213203435596)) ;
#83504=CARTESIAN_POINT('Origin',(79.0999999999999,263.4,30.3213203435596)) ;
#83505=CARTESIAN_POINT('Origin',(79.1999999999999,259.4,19.9213203435596)) ;
#83506=CARTESIAN_POINT('',(79.1999999999999,264.9,21.9213203435596)) ;
#83507=CARTESIAN_POINT('',(79.1999999999999,249.391753592594,21.9213203435596)) ;
#83508=CARTESIAN_POINT('',(79.1999999999999,264.9,30.7213203435596)) ;
#83509=CARTESIAN_POINT('',(79.1999999999999,264.9,19.9213203435596)) ;
#83510=CARTESIAN_POINT('',(79.1999999999999,263.8,31.8213203435596)) ;
#83511=CARTESIAN_POINT('Origin',(79.1999999999999,263.8,30.7213203435596)) ;
#83512=CARTESIAN_POINT('',(79.1999999999999,259.648528137424,31.8213203435596)) ;
#83513=CARTESIAN_POINT('',(79.1999999999999,249.391753592594,31.8213203435596)) ;
#83514=CARTESIAN_POINT('',(79.1999999999999,259.648528137424,30.8213203435596)) ;
#83515=CARTESIAN_POINT('',(79.1999999999999,259.648528137424,19.9213203435596)) ;
#83516=CARTESIAN_POINT('',(79.1999999999999,249.391753592594,30.8213203435596)) ;
#83517=CARTESIAN_POINT('Origin',(77.1999999999999,249.391753592594,21.9213203435596)) ;
#83518=CARTESIAN_POINT('',(77.1999999999999,264.9,19.9213203435596)) ;
#83519=CARTESIAN_POINT('',(77.1999999999999,249.391753592594,19.9213203435596)) ;
#83520=CARTESIAN_POINT('Origin',(77.1999999999999,264.9,21.9213203435596)) ;
#83521=CARTESIAN_POINT('Origin',(53.7,239.383507185188,19.9213203435596)) ;
#83522=CARTESIAN_POINT('',(44.8,264.9,19.9213203435596)) ;
#83523=CARTESIAN_POINT('',(44.8,252.191753592594,19.9213203435596)) ;
#83524=CARTESIAN_POINT('',(66.4499999999999,264.9,19.9213203435596)) ;
#83525=CARTESIAN_POINT('Origin',(44.8,252.191753592594,21.9213203435596)) ;
#83526=CARTESIAN_POINT('',(42.8,264.9,21.9213203435596)) ;
#83527=CARTESIAN_POINT('',(42.8,252.191753592594,21.9213203435596)) ;
#83528=CARTESIAN_POINT('Origin',(44.8,264.9,21.9213203435596)) ;
#83529=CARTESIAN_POINT('Origin',(42.8,265.,19.9213203435596)) ;
#83530=CARTESIAN_POINT('',(42.8,264.9,25.0213203435596)) ;
#83531=CARTESIAN_POINT('',(42.8,265.,25.0213203435596)) ;
#83532=CARTESIAN_POINT('',(42.8,264.9,19.9213203435596)) ;
#83533=CARTESIAN_POINT('Origin',(40.2,265.,25.0213203435596)) ;
#83534=CARTESIAN_POINT('',(37.6,264.9,25.0213203435596)) ;
#83535=CARTESIAN_POINT('',(37.6,265.,25.0213203435596)) ;
#83536=CARTESIAN_POINT('Origin',(40.2,264.9,25.0213203435596)) ;
#83537=CARTESIAN_POINT('Origin',(37.6,265.,25.0213203435596)) ;
#83538=CARTESIAN_POINT('',(37.6,264.9,21.9213203435596)) ;
#83539=CARTESIAN_POINT('',(37.6,252.191753592594,21.9213203435596)) ;
#83540=CARTESIAN_POINT('',(37.6,264.9,22.4713203435596)) ;
#83541=CARTESIAN_POINT('Origin',(35.6,252.191753592594,21.9213203435596)) ;
#83542=CARTESIAN_POINT('',(35.6,264.9,19.9213203435596)) ;
#83543=CARTESIAN_POINT('',(35.6,252.191753592594,19.9213203435596)) ;
#83544=CARTESIAN_POINT('Origin',(35.6,264.9,21.9213203435596)) ;
#83545=CARTESIAN_POINT('Origin',(53.7,239.383507185188,19.9213203435596)) ;
#83546=CARTESIAN_POINT('',(28.2,264.9,19.9213203435596)) ;
#83547=CARTESIAN_POINT('',(28.2,252.191753592594,19.9213203435596)) ;
#83548=CARTESIAN_POINT('',(66.4499999999999,264.9,19.9213203435596)) ;
#83549=CARTESIAN_POINT('Origin',(28.2,252.191753592594,21.9213203435596)) ;
#83550=CARTESIAN_POINT('',(26.2,264.9,21.9213203435596)) ;
#83551=CARTESIAN_POINT('',(26.2,252.191753592594,21.9213203435596)) ;
#83552=CARTESIAN_POINT('Origin',(28.2,264.9,21.9213203435596)) ;
#83553=CARTESIAN_POINT('Origin',(26.2,265.,19.9213203435596)) ;
#83554=CARTESIAN_POINT('',(26.2,245.6,30.8213203435596)) ;
#83555=CARTESIAN_POINT('',(26.2,252.191753592594,30.8213203435596)) ;
#83556=CARTESIAN_POINT('',(26.2,245.6,31.8213203435596)) ;
#83557=CARTESIAN_POINT('',(26.2,245.6,19.9213203435596)) ;
#83558=CARTESIAN_POINT('',(26.2,263.8,31.8213203435596)) ;
#83559=CARTESIAN_POINT('',(26.2,252.191753592594,31.8213203435596)) ;
#83560=CARTESIAN_POINT('',(26.2,264.9,30.7213203435596)) ;
#83561=CARTESIAN_POINT('Origin',(26.2,263.8,30.7213203435596)) ;
#83562=CARTESIAN_POINT('',(26.2,264.9,19.9213203435596)) ;
#83563=CARTESIAN_POINT('Origin',(73.2,257.,29.7213203435596)) ;
#83564=CARTESIAN_POINT('',(70.2,257.,29.7213203435596)) ;
#83565=CARTESIAN_POINT('Origin',(69.2,257.,29.7213203435596)) ;
#83566=CARTESIAN_POINT('Origin',(73.2,257.,29.7213203435596)) ;
#83567=CARTESIAN_POINT('Origin',(73.2,257.,28.9213203435596)) ;
#83568=CARTESIAN_POINT('',(70.2,257.,29.6213203435596)) ;
#83569=CARTESIAN_POINT('',(70.2,257.,28.9213203435596)) ;
#83570=CARTESIAN_POINT('Origin',(73.2,257.,29.6213203435596)) ;
#83571=CARTESIAN_POINT('Ctrl Pts',(48.2000201227716,256.997564528802,29.7391774864168)) ;
#83572=CARTESIAN_POINT('Ctrl Pts',(48.1996571011318,257.444729584704,29.7391774864168)) ;
#83573=CARTESIAN_POINT('Ctrl Pts',(48.4033873306915,258.343067515653,29.7391774864168)) ;
#83574=CARTESIAN_POINT('Ctrl Pts',(49.2644744428091,259.424847087356,29.7391774864168)) ;
#83575=CARTESIAN_POINT('Ctrl Pts',(50.5092023113187,260.024848656503,29.7391774864168)) ;
#83576=CARTESIAN_POINT('Ctrl Pts',(51.8895719273014,260.025418883332,29.7391774864168)) ;
#83577=CARTESIAN_POINT('Ctrl Pts',(53.1339976230268,259.425189243343,29.7391774864168)) ;
#83578=CARTESIAN_POINT('Ctrl Pts',(54.0921043443573,258.227243818021,29.7391774864167)) ;
#83579=CARTESIAN_POINT('Ctrl Pts',(54.2793447377661,256.988928127914,29.7391774864167)) ;
#83580=CARTESIAN_POINT('Ctrl Pts',(54.0781150882907,256.116150279737,29.7391774864167)) ;
#83581=CARTESIAN_POINT('Ctrl Pts',(53.8074694386866,255.419327571605,29.7391774864167)) ;
#83582=CARTESIAN_POINT('Ctrl Pts',(53.138809657118,254.578338020705,29.7391774864167)) ;
#83583=CARTESIAN_POINT('Ctrl Pts',(51.8961163858473,253.976736687915,29.7391774864168)) ;
#83584=CARTESIAN_POINT('Ctrl Pts',(50.5134730340159,253.975593963619,29.7391774864168)) ;
#83585=CARTESIAN_POINT('Ctrl Pts',(49.2694700738971,254.572057959393,29.7391774864168)) ;
#83586=CARTESIAN_POINT('Ctrl Pts',(48.4056998977081,255.653404362029,29.7391774864168)) ;
#83587=CARTESIAN_POINT('Ctrl Pts',(48.2003831444115,256.550399472899,29.7391774864168)) ;
#83588=CARTESIAN_POINT('Ctrl Pts',(48.2000201227716,256.997564528802,29.7391774864168)) ;
#83589=CARTESIAN_POINT('Ctrl Pts',(48.1947380216729,256.997560240638,30.0349280800261)) ;
#83590=CARTESIAN_POINT('Ctrl Pts',(48.1943747281785,257.445060163369,30.0349280800261)) ;
#83591=CARTESIAN_POINT('Ctrl Pts',(48.3987531591452,258.34442732955,30.0349280800261)) ;
#83592=CARTESIAN_POINT('Ctrl Pts',(49.2614119341439,259.427283390293,30.0349280800261)) ;
#83593=CARTESIAN_POINT('Ctrl Pts',(50.5074335198535,260.027951447571,30.0349280800261)) ;
#83594=CARTESIAN_POINT('Ctrl Pts',(51.889675953912,260.028326821561,30.0349280800261)) ;
#83595=CARTESIAN_POINT('Ctrl Pts',(53.1358585454785,259.427468823063,30.0349280800261)) ;
#83596=CARTESIAN_POINT('Ctrl Pts',(54.0948641455133,258.228316050248,30.0349280800261)) ;
#83597=CARTESIAN_POINT('Ctrl Pts',(54.2823703564133,256.988738847751,30.0349280800261)) ;
#83598=CARTESIAN_POINT('Ctrl Pts',(54.0809503109861,256.115159784954,30.0349280800261)) ;
#83599=CARTESIAN_POINT('Ctrl Pts',(53.8099967208346,255.41769815285,30.0349280800261)) ;
#83600=CARTESIAN_POINT('Ctrl Pts',(53.1404967730488,254.575643430502,30.0349280800261)) ;
#83601=CARTESIAN_POINT('Ctrl Pts',(51.8964734498615,253.973593813523,30.0349280800261)) ;
#83602=CARTESIAN_POINT('Ctrl Pts',(50.5123829163539,253.972292508993,30.0349280800261)) ;
#83603=CARTESIAN_POINT('Ctrl Pts',(49.2664516588918,254.569603468298,30.0349280800261)) ;
#83604=CARTESIAN_POINT('Ctrl Pts',(48.4011338558011,255.652030289862,30.0349280800261)) ;
#83605=CARTESIAN_POINT('Ctrl Pts',(48.1951013151674,256.550060317907,30.0349280800261)) ;
#83606=CARTESIAN_POINT('Ctrl Pts',(48.1947380216729,256.997560240638,30.0349280800261)) ;
#83607=CARTESIAN_POINT('Ctrl Pts',(47.9403271495437,256.997353702469,30.5426019839815)) ;
#83608=CARTESIAN_POINT('Ctrl Pts',(47.9399326186896,257.483331374468,30.5426019839815)) ;
#83609=CARTESIAN_POINT('Ctrl Pts',(48.1612323137361,258.459560607115,30.5426019839815)) ;
#83610=CARTESIAN_POINT('Ctrl Pts',(49.0968466073856,259.63517435474,30.5426019839815)) ;
#83611=CARTESIAN_POINT('Ctrl Pts',(50.4495302427206,260.287204473252,30.5426019839815)) ;
#83612=CARTESIAN_POINT('Ctrl Pts',(51.9495193659296,260.287869000223,30.5426019839815)) ;
#83613=CARTESIAN_POINT('Ctrl Pts',(53.3017682744996,259.635582227122,30.5426019839815)) ;
#83614=CARTESIAN_POINT('Ctrl Pts',(54.3429942328016,258.333729835107,30.5426019839814)) ;
#83615=CARTESIAN_POINT('Ctrl Pts',(54.5464577252491,256.988008648977,30.5426019839814)) ;
#83616=CARTESIAN_POINT('Ctrl Pts',(54.3277710414745,256.039510112854,30.5426019839814)) ;
#83617=CARTESIAN_POINT('Ctrl Pts',(54.0336582949932,255.282232103612,30.5426019839814)) ;
#83618=CARTESIAN_POINT('Ctrl Pts',(53.3070386850274,254.368347021547,30.5426019839814)) ;
#83619=CARTESIAN_POINT('Ctrl Pts',(51.9565749304451,253.714527943762,30.5426019839815)) ;
#83620=CARTESIAN_POINT('Ctrl Pts',(50.4540166666556,253.713322223552,30.5426019839815)) ;
#83621=CARTESIAN_POINT('Ctrl Pts',(49.1022665858778,254.361465700547,30.5426019839815)) ;
#83622=CARTESIAN_POINT('Ctrl Pts',(48.163730370093,255.536607705174,30.5426019839815)) ;
#83623=CARTESIAN_POINT('Ctrl Pts',(47.9407216803977,256.511376030469,30.5426019839815)) ;
#83624=CARTESIAN_POINT('Ctrl Pts',(47.9403271495437,256.997353702469,30.5426019839815)) ;
#83625=CARTESIAN_POINT('Ctrl Pts',(47.4220281498853,256.996932932218,30.7213203435596)) ;
#83626=CARTESIAN_POINT('Ctrl Pts',(47.4215709320604,257.560127551602,30.7213203435596)) ;
#83627=CARTESIAN_POINT('Ctrl Pts',(47.6780933089332,258.691513196809,30.7213203435596)) ;
#83628=CARTESIAN_POINT('Ctrl Pts',(48.7624802059068,260.053952562978,30.7213203435596)) ;
#83629=CARTESIAN_POINT('Ctrl Pts',(50.3301356783258,260.809610148858,30.7213203435596)) ;
#83630=CARTESIAN_POINT('Ctrl Pts',(52.0685601808136,260.810356467353,30.7213203435596)) ;
#83631=CARTESIAN_POINT('Ctrl Pts',(53.6357683192668,260.054406114016,30.7213203435596)) ;
#83632=CARTESIAN_POINT('Ctrl Pts',(54.8424566758268,258.545664711818,30.7213203435596)) ;
#83633=CARTESIAN_POINT('Ctrl Pts',(55.0782637682426,256.986081290598,30.7213203435596)) ;
#83634=CARTESIAN_POINT('Ctrl Pts',(54.824825139774,255.886857921965,30.7213203435596)) ;
#83635=CARTESIAN_POINT('Ctrl Pts',(54.4839680197378,255.009241811416,30.7213203435596)) ;
#83636=CARTESIAN_POINT('Ctrl Pts',(53.6418545271852,253.950096561179,30.7213203435596)) ;
#83637=CARTESIAN_POINT('Ctrl Pts',(52.0767670390764,253.192392502866,30.7213203435596)) ;
#83638=CARTESIAN_POINT('Ctrl Pts',(50.3354172573281,253.19097598695,30.7213203435596)) ;
#83639=CARTESIAN_POINT('Ctrl Pts',(48.7687662812976,253.942151697168,30.7213203435596)) ;
#83640=CARTESIAN_POINT('Ctrl Pts',(47.6809963718967,255.304044883527,30.7213203435596)) ;
#83641=CARTESIAN_POINT('Ctrl Pts',(47.4224853677104,256.433738312834,30.7213203435596)) ;
#83642=CARTESIAN_POINT('Ctrl Pts',(47.4220281498854,256.996932932218,30.7213203435596)) ;
#83643=CARTESIAN_POINT('Ctrl Pts',(47.2001799037401,256.996752829339,30.7213203435596)) ;
#83644=CARTESIAN_POINT('Ctrl Pts',(47.1996958934101,257.592950087367,30.7213203435596)) ;
#83645=CARTESIAN_POINT('Ctrl Pts',(47.4713258041952,258.790688157784,30.7213203435596)) ;
#83646=CARTESIAN_POINT('Ctrl Pts',(48.6193980168863,260.233005722467,30.7213203435596)) ;
#83647=CARTESIAN_POINT('Ctrl Pts',(50.2789716629066,261.032977199702,30.7213203435596)) ;
#83648=CARTESIAN_POINT('Ctrl Pts',(52.1193940511311,261.033737473045,30.7213203435596)) ;
#83649=CARTESIAN_POINT('Ctrl Pts',(53.7785648155242,260.233461912991,30.7213203435596)) ;
#83650=CARTESIAN_POINT('Ctrl Pts',(55.0559915567595,258.636262470822,30.7213203435596)) ;
#83651=CARTESIAN_POINT('Ctrl Pts',(55.305635860734,256.985238068826,30.7213203435596)) ;
#83652=CARTESIAN_POINT('Ctrl Pts',(55.0373399291364,255.821578804573,30.7213203435596)) ;
#83653=CARTESIAN_POINT('Ctrl Pts',(54.6764928726381,254.892517415637,30.7213203435596)) ;
#83654=CARTESIAN_POINT('Ctrl Pts',(53.7849806154459,253.771240925762,30.7213203435596)) ;
#83655=CARTESIAN_POINT('Ctrl Pts',(52.1281196619292,252.969136511964,30.7213203435596)) ;
#83656=CARTESIAN_POINT('Ctrl Pts',(50.2846657419234,252.967612937877,30.7213203435596)) ;
#83657=CARTESIAN_POINT('Ctrl Pts',(48.6260586034358,253.762867831118,30.7213203435596)) ;
#83658=CARTESIAN_POINT('Ctrl Pts',(47.4744091088858,255.204607859147,30.7213203435596)) ;
#83659=CARTESIAN_POINT('Ctrl Pts',(47.2006639140701,256.40055557131,30.7213203435596)) ;
#83660=CARTESIAN_POINT('Ctrl Pts',(47.2001799037401,256.996752829339,30.7213203435596)) ;
#83661=CARTESIAN_POINT('',(48.2000203746466,256.99756452918,29.7391774849179)) ;
#83662=CARTESIAN_POINT('Ctrl Pts',(47.2001799037401,256.996752829339,30.7213203435596)) ;
#83663=CARTESIAN_POINT('Ctrl Pts',(47.4220281498853,256.996932932218,30.7213203435596)) ;
#83664=CARTESIAN_POINT('Ctrl Pts',(47.9403271495437,256.997353702469,30.5426019839815)) ;
#83665=CARTESIAN_POINT('Ctrl Pts',(48.1947380216729,256.997560240638,30.0349280800261)) ;
#83666=CARTESIAN_POINT('Ctrl Pts',(48.2000201227716,256.997564528802,29.7391774864168)) ;
#83667=CARTESIAN_POINT('',(48.2000195339838,256.999999959719,29.7391774864168)) ;
#83668=CARTESIAN_POINT('Ctrl Pts',(48.2000208783164,256.997564529727,29.7391774864168)) ;
#83669=CARTESIAN_POINT('Ctrl Pts',(48.2005690937809,256.549587458459,29.7391774864168)) ;
#83670=CARTESIAN_POINT('Ctrl Pts',(48.4059605550267,255.653078047389,29.7391774864168)) ;
#83671=CARTESIAN_POINT('Ctrl Pts',(49.2694700738971,254.572057959393,29.7391774864168)) ;
#83672=CARTESIAN_POINT('Ctrl Pts',(50.5134730340159,253.975593963619,29.7391774864168)) ;
#83673=CARTESIAN_POINT('Ctrl Pts',(51.8961163858473,253.976736687915,29.7391774864168)) ;
#83674=CARTESIAN_POINT('Ctrl Pts',(53.138809657118,254.578338020705,29.7391774864167)) ;
#83675=CARTESIAN_POINT('Ctrl Pts',(53.8074694386866,255.419327571605,29.7391774864167)) ;
#83676=CARTESIAN_POINT('Ctrl Pts',(54.0781150882907,256.116150279737,29.7391774864167)) ;
#83677=CARTESIAN_POINT('Ctrl Pts',(54.2793447377661,256.988928127914,29.7391774864167)) ;
#83678=CARTESIAN_POINT('Ctrl Pts',(54.0921043443573,258.227243818021,29.7391774864167)) ;
#83679=CARTESIAN_POINT('Ctrl Pts',(53.1339976230268,259.425189243343,29.7391774864168)) ;
#83680=CARTESIAN_POINT('Ctrl Pts',(51.8895719273014,260.025418883332,29.7391774864168)) ;
#83681=CARTESIAN_POINT('Ctrl Pts',(50.5092023113187,260.024848656503,29.7391774864168)) ;
#83682=CARTESIAN_POINT('Ctrl Pts',(49.2644744428091,259.424847087356,29.7391774864168)) ;
#83683=CARTESIAN_POINT('Ctrl Pts',(48.4041682584632,258.344048591433,29.7391774864168)) ;
#83684=CARTESIAN_POINT('Ctrl Pts',(48.200212080878,257.447173389509,29.7391774864168)) ;
#83685=CARTESIAN_POINT('Ctrl Pts',(48.2000199116081,256.999999959709,29.7391774864168)) ;
#83686=CARTESIAN_POINT('',(48.2000191563594,256.999999960043,29.7391774864168)) ;
#83687=CARTESIAN_POINT('Origin',(51.2,257.,29.7413203435596)) ;
#83688=CARTESIAN_POINT('',(48.32,257.,29.6213203435596)) ;
#83689=CARTESIAN_POINT('Origin',(48.32,257.,29.7413203435596)) ;
#83690=CARTESIAN_POINT('Origin',(51.2,257.,29.6213203435596)) ;
#83691=CARTESIAN_POINT('Origin',(51.2,257.,29.6213203435596)) ;
#83692=CARTESIAN_POINT('',(53.32,257.,29.6213203435596)) ;
#83693=CARTESIAN_POINT('Origin',(51.2,257.,29.6213203435596)) ;
#83694=CARTESIAN_POINT('Origin',(51.2,257.,29.7413203435596)) ;
#83695=CARTESIAN_POINT('',(49.2,257.,29.7413203435596)) ;
#83696=CARTESIAN_POINT('',(53.2,257.,29.7413203435596)) ;
#83697=CARTESIAN_POINT('Origin',(51.2,257.,29.7413203435596)) ;
#83698=CARTESIAN_POINT('Origin',(53.32,257.,29.7413203435596)) ;
#83699=CARTESIAN_POINT('Origin',(51.2,257.,29.7413203435596)) ;
#83700=CARTESIAN_POINT('Origin',(51.2,257.,19.9213203435596)) ;
#83701=CARTESIAN_POINT('',(49.2,257.,30.1213203435596)) ;
#83702=CARTESIAN_POINT('',(49.2,257.,19.9213203435596)) ;
#83703=CARTESIAN_POINT('Origin',(51.2,257.,30.1213203435596)) ;
#83704=CARTESIAN_POINT('Origin',(73.1999999999999,263.88342319271,27.1425655430194)) ;
#83705=CARTESIAN_POINT('',(73.1999999999999,263.59500851924,29.0950298771693)) ;
#83706=CARTESIAN_POINT('Origin',(73.1999999999999,264.000849166908,27.1672868007454)) ;
#83707=CARTESIAN_POINT('',(73.1999999999999,263.502303802768,28.9528826452449)) ;
#83708=CARTESIAN_POINT('Origin',(73.1999999999999,263.477582545042,29.0703086194433)) ;
#83709=CARTESIAN_POINT('',(75.0499999999999,263.88342319271,27.1425655430194)) ;
#83710=CARTESIAN_POINT('Origin',(73.1999999999999,263.88342319271,27.1425655430194)) ;
#83711=CARTESIAN_POINT('Origin',(73.1999999999999,263.88342319271,27.1425655430194)) ;
#83712=CARTESIAN_POINT('Origin',(73.1999999999999,264.000849166908,27.1672868007454)) ;
#83713=CARTESIAN_POINT('',(75.0499999999999,262.944015399123,26.9447954812117)) ;
#83714=CARTESIAN_POINT('',(75.0499999999999,264.000849166908,27.1672868007454)) ;
#83715=CARTESIAN_POINT('',(73.1999999999999,263.325134789065,25.134478378986)) ;
#83716=CARTESIAN_POINT('Origin',(73.1999999999999,262.944015399123,26.9447954812115)) ;
#83717=CARTESIAN_POINT('Origin',(73.1999999999999,262.944015399123,26.9447954812115)) ;
#83718=CARTESIAN_POINT('Origin',(75.1,264.,27.1713203435596)) ;
#83719=CARTESIAN_POINT('',(76.5,263.20058682584,30.9685329208194)) ;
#83720=CARTESIAN_POINT('',(69.9,263.20058682584,30.9685329208194)) ;
#83721=CARTESIAN_POINT('',(64.4,263.20058682584,30.9685329208194)) ;
#83722=CARTESIAN_POINT('',(76.5,264.010725107507,27.120376082903)) ;
#83723=CARTESIAN_POINT('',(76.5,264.75198938992,23.5993707414376)) ;
#83724=CARTESIAN_POINT('',(77.3539593550092,265.,22.4213203435597)) ;
#83725=CARTESIAN_POINT('Origin',(77.5,264.010725107507,27.1203760829029)) ;
#83726=CARTESIAN_POINT('',(69.0460404446207,265.,22.4213203435596)) ;
#83727=CARTESIAN_POINT('',(26.2,265.,22.4213203435596)) ;
#83728=CARTESIAN_POINT('',(69.9,264.010725107507,27.1203760829029)) ;
#83729=CARTESIAN_POINT('Origin',(68.8999999999999,264.010725107507,27.1203760829029)) ;
#83730=CARTESIAN_POINT('',(69.9,264.709549071618,23.8009622533739)) ;
#83731=CARTESIAN_POINT('Origin',(73.1999999999999,262.944015399123,26.9447954812115)) ;
#83732=CARTESIAN_POINT('',(73.1999999999999,263.232430072592,24.9923311470616)) ;
#83733=CARTESIAN_POINT('Origin',(73.1999999999999,262.826589424924,26.9200742234855)) ;
#83734=CARTESIAN_POINT('Origin',(73.1999999999999,263.349856046791,25.0170524047876)) ;
#83735=CARTESIAN_POINT('Origin',(75.1,262.825740258016,26.9241077662998)) ;
#83736=CARTESIAN_POINT('',(77.2325869638084,263.799952628918,22.2965990045162)) ;
#83737=CARTESIAN_POINT('',(76.5,262.836465365522,26.8731635056432)) ;
#83738=CARTESIAN_POINT('Ctrl Pts',(77.2324172913864,263.799905257836,22.2968240171558)) ;
#83739=CARTESIAN_POINT('Ctrl Pts',(77.0709872482774,263.754804582325,22.5110522258322)) ;
#83740=CARTESIAN_POINT('Ctrl Pts',(76.6823307971632,263.532544066078,23.5667896780028)) ;
#83741=CARTESIAN_POINT('Ctrl Pts',(76.4999999999999,263.102238319793,25.6107419728579)) ;
#83742=CARTESIAN_POINT('Ctrl Pts',(76.5,262.836465365523,26.8731635056432)) ;
#83743=CARTESIAN_POINT('',(76.5,263.577729647936,23.3521581641778)) ;
#83744=CARTESIAN_POINT('',(69.9,262.836465365522,26.8731635056431)) ;
#83745=CARTESIAN_POINT('',(69.9,263.535289329634,23.5537496761141)) ;
#83746=CARTESIAN_POINT('',(69.1671450699313,263.79990527434,22.2968239387601)) ;
#83747=CARTESIAN_POINT('Ctrl Pts',(69.8999999999999,262.836465365523,26.8731635056431)) ;
#83748=CARTESIAN_POINT('Ctrl Pts',(69.9,263.036041279363,25.9251779149008)) ;
#83749=CARTESIAN_POINT('Ctrl Pts',(69.766510541265,263.46977838237,23.8649266756155)) ;
#83750=CARTESIAN_POINT('Ctrl Pts',(69.3922529932014,263.736480055353,22.598093728948)) ;
#83751=CARTESIAN_POINT('Ctrl Pts',(69.1674817299058,263.79981054868,22.2972738856443)) ;
#83752=CARTESIAN_POINT('',(77.1499999999999,263.8,22.2963739918749)) ;
#83753=CARTESIAN_POINT('Origin',(51.1999999999999,263.88342319271,27.1425655430194)) ;
#83754=CARTESIAN_POINT('',(51.1999999999999,263.59500851924,29.0950298771693)) ;
#83755=CARTESIAN_POINT('Origin',(51.1999999999999,264.000849166908,27.1672868007454)) ;
#83756=CARTESIAN_POINT('',(51.1999999999999,263.502303802768,28.9528826452449)) ;
#83757=CARTESIAN_POINT('Origin',(51.1999999999999,263.477582545042,29.0703086194433)) ;
#83758=CARTESIAN_POINT('',(53.0499999999999,263.88342319271,27.1425655430194)) ;
#83759=CARTESIAN_POINT('Origin',(51.1999999999999,263.88342319271,27.1425655430194)) ;
#83760=CARTESIAN_POINT('Origin',(51.1999999999999,263.88342319271,27.1425655430194)) ;
#83761=CARTESIAN_POINT('Origin',(51.1999999999999,264.000849166908,27.1672868007454)) ;
#83762=CARTESIAN_POINT('',(53.0499999999999,262.944015399123,26.9447954812117)) ;
#83763=CARTESIAN_POINT('',(53.0499999999999,264.000849166908,27.1672868007454)) ;
#83764=CARTESIAN_POINT('',(51.1999999999999,263.325134789065,25.134478378986)) ;
#83765=CARTESIAN_POINT('Origin',(51.1999999999999,262.944015399123,26.9447954812115)) ;
#83766=CARTESIAN_POINT('Origin',(51.1999999999999,262.944015399123,26.9447954812115)) ;
#83767=CARTESIAN_POINT('Origin',(53.1,264.,27.1713203435596)) ;
#83768=CARTESIAN_POINT('',(54.5,263.20058682584,30.9685329208194)) ;
#83769=CARTESIAN_POINT('',(47.9,263.20058682584,30.9685329208194)) ;
#83770=CARTESIAN_POINT('',(53.4,263.20058682584,30.9685329208194)) ;
#83771=CARTESIAN_POINT('',(54.5,264.010725107507,27.120376082903)) ;
#83772=CARTESIAN_POINT('',(54.5,264.75198938992,23.5993707414376)) ;
#83773=CARTESIAN_POINT('',(55.3539343055938,265.,22.4213203435596)) ;
#83774=CARTESIAN_POINT('Origin',(55.5,264.010725107507,27.1203760829029)) ;
#83775=CARTESIAN_POINT('',(47.0460398203948,265.,22.4213203435596)) ;
#83776=CARTESIAN_POINT('',(26.2,265.,22.4213203435596)) ;
#83777=CARTESIAN_POINT('',(47.9,264.010725107507,27.1203760829029)) ;
#83778=CARTESIAN_POINT('Origin',(46.9,264.010725107507,27.1203760829029)) ;
#83779=CARTESIAN_POINT('',(47.9,264.709549071618,23.8009622533739)) ;
#83780=CARTESIAN_POINT('Origin',(51.1999999999999,262.944015399123,26.9447954812115)) ;
#83781=CARTESIAN_POINT('',(51.1999999999999,263.232430072592,24.9923311470617)) ;
#83782=CARTESIAN_POINT('Origin',(51.1999999999999,262.826589424924,26.9200742234856)) ;
#83783=CARTESIAN_POINT('Origin',(51.1999999999999,263.349856046791,25.0170524047876)) ;
#83784=CARTESIAN_POINT('Origin',(53.1,262.825740258016,26.9241077662998)) ;
#83785=CARTESIAN_POINT('',(47.9,262.836465365522,26.8731635056431)) ;
#83786=CARTESIAN_POINT('',(47.1671452090265,263.799905296423,22.2968238338636)) ;
#83787=CARTESIAN_POINT('Ctrl Pts',(47.9,262.836465365523,26.8731635056431)) ;
#83788=CARTESIAN_POINT('Ctrl Pts',(47.9,263.036041279363,25.925177914903)) ;
#83789=CARTESIAN_POINT('Ctrl Pts',(47.7665130315213,263.469780156239,23.8649182497395)) ;
#83790=CARTESIAN_POINT('Ctrl Pts',(47.3922533394392,263.736480301986,22.5980925574409)) ;
#83791=CARTESIAN_POINT('Ctrl Pts',(47.1674817919091,263.799810592846,22.2972736758538)) ;
#83792=CARTESIAN_POINT('',(55.2325867846313,263.799952660996,22.2965988521424)) ;
#83793=CARTESIAN_POINT('',(66.1499999999999,263.8,22.2963739918749)) ;
#83794=CARTESIAN_POINT('',(54.5,262.836465365522,26.8731635056432)) ;
#83795=CARTESIAN_POINT('Ctrl Pts',(55.2324172261571,263.799905321993,22.2968237124103)) ;
#83796=CARTESIAN_POINT('Ctrl Pts',(55.0709869664947,263.754804859476,22.511050909364)) ;
#83797=CARTESIAN_POINT('Ctrl Pts',(54.6823287364216,263.532546092952,23.5667800503536)) ;
#83798=CARTESIAN_POINT('Ctrl Pts',(54.4999999999999,263.102238319793,25.6107419728589)) ;
#83799=CARTESIAN_POINT('Ctrl Pts',(54.5,262.836465365523,26.8731635056432)) ;
#83800=CARTESIAN_POINT('',(54.5,263.577729647936,23.3521581641778)) ;
#83801=CARTESIAN_POINT('',(47.9,263.535289329634,23.5537496761141)) ;
#83802=CARTESIAN_POINT('Origin',(35.6,264.9,21.9213203435596)) ;
#83803=CARTESIAN_POINT('',(35.6,265.,20.0213203435596)) ;
#83804=CARTESIAN_POINT('Origin',(35.6,264.9,20.0213203435596)) ;
#83805=CARTESIAN_POINT('',(37.5,265.,21.9213203435596)) ;
#83806=CARTESIAN_POINT('Origin',(35.6,265.,21.9213203435596)) ;
#83807=CARTESIAN_POINT('Origin',(37.5,264.9,21.9213203435596)) ;
#83808=CARTESIAN_POINT('Origin',(37.5,264.9,22.4713203435596)) ;
#83809=CARTESIAN_POINT('',(37.5,265.,25.0213203435596)) ;
#83810=CARTESIAN_POINT('Origin',(37.5,264.9,25.0213203435596)) ;
#83811=CARTESIAN_POINT('',(37.5,265.,22.4713203435596)) ;
#83812=CARTESIAN_POINT('Origin',(40.2,264.9,25.0213203435596)) ;
#83813=CARTESIAN_POINT('',(42.9,265.,25.0213203435596)) ;
#83814=CARTESIAN_POINT('Origin',(42.9,264.9,25.0213203435596)) ;
#83815=CARTESIAN_POINT('Origin',(40.2,265.,25.0213203435596)) ;
#83816=CARTESIAN_POINT('Origin',(42.9,264.9,19.9213203435596)) ;
#83817=CARTESIAN_POINT('',(42.9,265.,21.9213203435596)) ;
#83818=CARTESIAN_POINT('Origin',(42.9,264.9,21.9213203435596)) ;
#83819=CARTESIAN_POINT('',(42.9,265.,19.9213203435596)) ;
#83820=CARTESIAN_POINT('Origin',(44.8,264.9,21.9213203435596)) ;
#83821=CARTESIAN_POINT('',(44.8,265.,20.0213203435596)) ;
#83822=CARTESIAN_POINT('Origin',(44.8,264.9,20.0213203435596)) ;
#83823=CARTESIAN_POINT('Origin',(44.8,265.,21.9213203435596)) ;
#83824=CARTESIAN_POINT('Origin',(79.1999999999999,265.,19.9213203435596)) ;
#83825=CARTESIAN_POINT('',(28.2,265.,20.0213203435596)) ;
#83826=CARTESIAN_POINT('',(66.4499999999999,265.,20.0213203435596)) ;
#83827=CARTESIAN_POINT('',(26.3,265.,21.9213203435596)) ;
#83828=CARTESIAN_POINT('Origin',(28.2,265.,21.9213203435596)) ;
#83829=CARTESIAN_POINT('',(26.3,265.,30.7213203435596)) ;
#83830=CARTESIAN_POINT('',(26.3,265.,19.9213203435596)) ;
#83831=CARTESIAN_POINT('',(46.9,265.,30.7213203435596)) ;
#83832=CARTESIAN_POINT('',(66.4499999999999,265.,30.7213203435596)) ;
#83833=CARTESIAN_POINT('',(46.9,265.,22.4733813234278)) ;
#83834=CARTESIAN_POINT('',(46.9,265.,19.9213203435596)) ;
#83835=CARTESIAN_POINT('Ctrl Pts',(47.0453687118714,265.,22.4213203435611)) ;
#83836=CARTESIAN_POINT('Ctrl Pts',(47.0190922729071,265.,22.4214536264379)) ;
#83837=CARTESIAN_POINT('Ctrl Pts',(46.992447726076,265.,22.424830164787)) ;
#83838=CARTESIAN_POINT('Ctrl Pts',(46.9546773758358,265.,22.4371420104603)) ;
#83839=CARTESIAN_POINT('Ctrl Pts',(46.9423422478844,265.,22.4425803610722)) ;
#83840=CARTESIAN_POINT('Ctrl Pts',(46.9197422382574,265.,22.4560226634585)) ;
#83841=CARTESIAN_POINT('Ctrl Pts',(46.9095834753162,265.,22.4637992160125)) ;
#83842=CARTESIAN_POINT('Ctrl Pts',(46.9003152423108,265.,22.4730640569009)) ;
#83843=CARTESIAN_POINT('Ctrl Pts',(46.9001574429778,265.,22.4732225117743)) ;
#83844=CARTESIAN_POINT('Ctrl Pts',(46.9,265.,22.4733813234278)) ;
#83845=CARTESIAN_POINT('',(55.5,265.,22.4733813234278)) ;
#83846=CARTESIAN_POINT('Ctrl Pts',(55.5,265.,22.4733813234278)) ;
#83847=CARTESIAN_POINT('Ctrl Pts',(55.4998440576649,265.,22.4732225009103)) ;
#83848=CARTESIAN_POINT('Ctrl Pts',(55.4996877611835,265.,22.4730640154298)) ;
#83849=CARTESIAN_POINT('Ctrl Pts',(55.4908833110416,265.,22.464175452815)) ;
#83850=CARTESIAN_POINT('Ctrl Pts',(55.4813394787527,265.,22.4566715159258)) ;
#83851=CARTESIAN_POINT('Ctrl Pts',(55.4600552303074,265.,22.4435953221648)) ;
#83852=CARTESIAN_POINT('Ctrl Pts',(55.448466273445,265.,22.4382495306549)) ;
#83853=CARTESIAN_POINT('Ctrl Pts',(55.4106891852956,265.,22.425086339052)) ;
#83854=CARTESIAN_POINT('Ctrl Pts',(55.3829804661023,265.,22.4213867240657)) ;
#83855=CARTESIAN_POINT('Ctrl Pts',(55.3555997571232,265.,22.421320343561)) ;
#83856=CARTESIAN_POINT('',(55.5,265.,30.7213203435596)) ;
#83857=CARTESIAN_POINT('',(55.5,265.,19.9213203435596)) ;
#83858=CARTESIAN_POINT('',(68.9,265.,30.7213203435596)) ;
#83859=CARTESIAN_POINT('',(66.4499999999999,265.,30.7213203435596)) ;
#83860=CARTESIAN_POINT('',(68.8999999999999,265.,22.4733813234278)) ;
#83861=CARTESIAN_POINT('',(68.8999999999999,265.,19.9213203435596)) ;
#83862=CARTESIAN_POINT('Ctrl Pts',(69.0453678447016,265.,22.4213203435607)) ;
#83863=CARTESIAN_POINT('Ctrl Pts',(69.0190920820314,265.,22.4214543901977)) ;
#83864=CARTESIAN_POINT('Ctrl Pts',(68.9924474326331,265.,22.4248305985132)) ;
#83865=CARTESIAN_POINT('Ctrl Pts',(68.9546771660397,265.,22.4371420488168)) ;
#83866=CARTESIAN_POINT('Ctrl Pts',(68.9423421942767,265.,22.4425803275581)) ;
#83867=CARTESIAN_POINT('Ctrl Pts',(68.9197422336765,265.,22.4560226169246)) ;
#83868=CARTESIAN_POINT('Ctrl Pts',(68.9095834355294,265.,22.4637992057439)) ;
#83869=CARTESIAN_POINT('Ctrl Pts',(68.9003152401964,265.,22.4730640573226)) ;
#83870=CARTESIAN_POINT('Ctrl Pts',(68.9001574425991,265.,22.4732225112997)) ;
#83871=CARTESIAN_POINT('Ctrl Pts',(68.8999999999999,265.,22.4733813234278)) ;
#83872=CARTESIAN_POINT('',(77.5,265.,22.4733813234278)) ;
#83873=CARTESIAN_POINT('Ctrl Pts',(77.5,265.,22.4733813234278)) ;
#83874=CARTESIAN_POINT('Ctrl Pts',(77.4998425562135,265.,22.4732225098274)) ;
#83875=CARTESIAN_POINT('Ctrl Pts',(77.4996847618097,265.,22.4730640587698)) ;
#83876=CARTESIAN_POINT('Ctrl Pts',(77.4908533994486,265.,22.4642358680099)) ;
#83877=CARTESIAN_POINT('Ctrl Pts',(77.4812280995991,265.,22.4567689285165)) ;
#83878=CARTESIAN_POINT('Ctrl Pts',(77.4599504800949,265.,22.4437921170525)) ;
#83879=CARTESIAN_POINT('Ctrl Pts',(77.4483957267967,265.,22.438461808421)) ;
#83880=CARTESIAN_POINT('Ctrl Pts',(77.4103406428432,265.,22.4251907142037)) ;
#83881=CARTESIAN_POINT('Ctrl Pts',(77.3822743638663,265.,22.4214616185286)) ;
#83882=CARTESIAN_POINT('Ctrl Pts',(77.3546324333372,265.,22.4213203435609)) ;
#83883=CARTESIAN_POINT('',(77.5,265.,30.7213203435596)) ;
#83884=CARTESIAN_POINT('',(77.5,265.,19.9213203435596)) ;
#83885=CARTESIAN_POINT('',(79.0999999999999,265.,30.7213203435596)) ;
#83886=CARTESIAN_POINT('',(66.4499999999999,265.,30.7213203435596)) ;
#83887=CARTESIAN_POINT('',(79.0999999999999,265.,21.9213203435596)) ;
#83888=CARTESIAN_POINT('',(79.0999999999999,265.,19.9213203435596)) ;
#83889=CARTESIAN_POINT('',(77.1999999999999,265.,20.0213203435596)) ;
#83890=CARTESIAN_POINT('Origin',(77.1999999999999,265.,21.9213203435596)) ;
#83891=CARTESIAN_POINT('',(66.4499999999999,265.,20.0213203435596)) ;
#83892=CARTESIAN_POINT('Origin',(66.4499999999999,264.9,20.0213203435596)) ;
#83893=CARTESIAN_POINT('Origin',(28.2,264.9,20.0213203435596)) ;
#83894=CARTESIAN_POINT('Origin',(79.1999999999999,263.8,19.9213203435596)) ;
#83895=CARTESIAN_POINT('',(78.1993563245317,263.8,30.3213203435596)) ;
#83896=CARTESIAN_POINT('',(66.4499999999999,263.8,30.3213203435596)) ;
#83897=CARTESIAN_POINT('',(78.0420937034656,263.800015547414,27.0760161755151)) ;
#83898=CARTESIAN_POINT('Origin',(76.5,263.8,30.548381323428)) ;
#83899=CARTESIAN_POINT('Ctrl Pts',(78.0420863446217,263.8,27.0760132984819)) ;
#83900=CARTESIAN_POINT('Ctrl Pts',(77.9385797424837,263.8,25.9938609841148)) ;
#83901=CARTESIAN_POINT('Ctrl Pts',(77.847161300073,263.800000000028,24.8253075196437)) ;
#83902=CARTESIAN_POINT('Ctrl Pts',(77.6881616771047,263.800000000028,23.2254574982112)) ;
#83903=CARTESIAN_POINT('Ctrl Pts',(77.6338781282738,263.800000000004,22.806209746512)) ;
#83904=CARTESIAN_POINT('Ctrl Pts',(77.5731133611966,263.800000000004,22.5633014256337)) ;
#83905=CARTESIAN_POINT('Ctrl Pts',(77.5656436952132,263.8,22.5362571159244)) ;
#83906=CARTESIAN_POINT('Ctrl Pts',(77.5525252044025,263.8,22.4970249872318)) ;
#83907=CARTESIAN_POINT('Ctrl Pts',(77.5472664241076,263.8,22.4827534614122)) ;
#83908=CARTESIAN_POINT('Ctrl Pts',(77.5345309823458,263.8,22.4531152552685)) ;
#83909=CARTESIAN_POINT('Ctrl Pts',(77.5266242104818,263.8,22.4374841446812)) ;
#83910=CARTESIAN_POINT('Ctrl Pts',(77.5042152651784,263.8,22.4030141768054)) ;
#83911=CARTESIAN_POINT('Ctrl Pts',(77.4839496773601,263.8,22.3779632317415)) ;
#83912=CARTESIAN_POINT('Ctrl Pts',(77.4178853473915,263.8,22.3331581295801)) ;
#83913=CARTESIAN_POINT('Ctrl Pts',(77.3812322693006,263.8,22.3183191618849)) ;
#83914=CARTESIAN_POINT('Ctrl Pts',(77.307381732694,263.8,22.300232389935)) ;
#83915=CARTESIAN_POINT('Ctrl Pts',(77.2699691807084,263.8,22.2963944605413)) ;
#83916=CARTESIAN_POINT('Ctrl Pts',(77.2327566362305,263.8,22.2963739918766)) ;
#83917=CARTESIAN_POINT('',(68.3578850163,263.800011090529,27.0760152372235)) ;
#83918=CARTESIAN_POINT('Ctrl Pts',(69.1668084099568,263.8,22.296373991876)) ;
#83919=CARTESIAN_POINT('Ctrl Pts',(69.1071461813465,263.8,22.2964240616732)) ;
#83920=CARTESIAN_POINT('Ctrl Pts',(69.0549431451098,263.8,22.3062923346873)) ;
#83921=CARTESIAN_POINT('Ctrl Pts',(68.9802386686246,263.8,22.3351722086986)) ;
#83922=CARTESIAN_POINT('Ctrl Pts',(68.9509341582604,263.8,22.3516916978657)) ;
#83923=CARTESIAN_POINT('Ctrl Pts',(68.9022365717782,263.8,22.3939701968917)) ;
#83924=CARTESIAN_POINT('Ctrl Pts',(68.8864566236587,263.8,22.4156208414979)) ;
#83925=CARTESIAN_POINT('Ctrl Pts',(68.8666952618675,263.8,22.4504498771856)) ;
#83926=CARTESIAN_POINT('Ctrl Pts',(68.8598414559823,263.8,22.4654710745531)) ;
#83927=CARTESIAN_POINT('Ctrl Pts',(68.8477759615529,263.8,22.4957554711451)) ;
#83928=CARTESIAN_POINT('Ctrl Pts',(68.8423101798017,263.8,22.511735034006)) ;
#83929=CARTESIAN_POINT('Ctrl Pts',(68.8256553266128,263.8,22.5652106127884)) ;
#83930=CARTESIAN_POINT('Ctrl Pts',(68.8153865038261,263.8,22.6074723643896)) ;
#83931=CARTESIAN_POINT('Ctrl Pts',(68.7300038445153,263.8,22.9981158670073)) ;
#83932=CARTESIAN_POINT('Ctrl Pts',(68.657295336473,263.799999999949,23.7292165741023)) ;
#83933=CARTESIAN_POINT('Ctrl Pts',(68.5036810339554,263.799999999949,25.4440967856073)) ;
#83934=CARTESIAN_POINT('Ctrl Pts',(68.4331437753965,263.8,26.2891604408503)) ;
#83935=CARTESIAN_POINT('Ctrl Pts',(68.3578902629937,263.8,27.0760131853556)) ;
#83936=CARTESIAN_POINT('',(68.2,263.8,30.5483813234279)) ;
#83937=CARTESIAN_POINT('Origin',(69.9,263.8,30.5483813234279)) ;
#83938=CARTESIAN_POINT('',(68.2,263.8,19.9213203435596)) ;
#83939=CARTESIAN_POINT('',(56.2,263.8,30.548381323428)) ;
#83940=CARTESIAN_POINT('',(56.2,263.8,19.9213203435596)) ;
#83941=CARTESIAN_POINT('',(56.0420937198539,263.800015543961,27.0760161747882)) ;
#83942=CARTESIAN_POINT('Origin',(54.5,263.8,30.548381323428)) ;
#83943=CARTESIAN_POINT('Ctrl Pts',(56.0420863626506,263.8,27.0760132983946)) ;
#83944=CARTESIAN_POINT('Ctrl Pts',(55.9385805509996,263.8,25.9938693510034)) ;
#83945=CARTESIAN_POINT('Ctrl Pts',(55.8471616308305,263.800000000026,24.825314711562)) ;
#83946=CARTESIAN_POINT('Ctrl Pts',(55.6881591543513,263.800000000026,23.2254385528796)) ;
#83947=CARTESIAN_POINT('Ctrl Pts',(55.6338760138876,263.800000000004,22.8061998855569)) ;
#83948=CARTESIAN_POINT('Ctrl Pts',(55.5731125109262,263.800000000004,22.5632984759483)) ;
#83949=CARTESIAN_POINT('Ctrl Pts',(55.5656430417995,263.8,22.536255083441)) ;
#83950=CARTESIAN_POINT('Ctrl Pts',(55.5525248140369,263.8,22.4970239295753)) ;
#83951=CARTESIAN_POINT('Ctrl Pts',(55.5472660822281,263.8,22.4827526087893)) ;
#83952=CARTESIAN_POINT('Ctrl Pts',(55.534530691983,263.8,22.4531146554099)) ;
#83953=CARTESIAN_POINT('Ctrl Pts',(55.5266239224689,263.8,22.4374836332353)) ;
#83954=CARTESIAN_POINT('Ctrl Pts',(55.5042149314907,263.8,22.4030137503595)) ;
#83955=CARTESIAN_POINT('Ctrl Pts',(55.4839492743427,263.8,22.3779628455479)) ;
#83956=CARTESIAN_POINT('Ctrl Pts',(55.4178847304879,263.8,22.3331578097732)) ;
#83957=CARTESIAN_POINT('Ctrl Pts',(55.3812314093916,263.8,22.3183188321358)) ;
#83958=CARTESIAN_POINT('Ctrl Pts',(55.3073810167929,263.8,22.3002321949928)) ;
#83959=CARTESIAN_POINT('Ctrl Pts',(55.2699686939412,263.8,22.2963942886275)) ;
#83960=CARTESIAN_POINT('Ctrl Pts',(55.2327563431054,263.8,22.2963739918746)) ;
#83961=CARTESIAN_POINT('',(46.3578850044002,263.800011088028,27.0760152366969)) ;
#83962=CARTESIAN_POINT('Ctrl Pts',(47.166808626144,263.8,22.2963739918735)) ;
#83963=CARTESIAN_POINT('Ctrl Pts',(47.1071458919983,263.8,22.296423758252)) ;
#83964=CARTESIAN_POINT('Ctrl Pts',(47.0549411454493,263.8,22.3062924794497)) ;
#83965=CARTESIAN_POINT('Ctrl Pts',(46.9802357268767,263.8,22.3351737363304)) ;
#83966=CARTESIAN_POINT('Ctrl Pts',(46.9509317672401,263.8,22.3516933245359)) ;
#83967=CARTESIAN_POINT('Ctrl Pts',(46.902235607331,263.8,22.3939714478775)) ;
#83968=CARTESIAN_POINT('Ctrl Pts',(46.8864560566414,263.8,22.4156216929879)) ;
#83969=CARTESIAN_POINT('Ctrl Pts',(46.8666949613237,263.8,22.450450502502)) ;
#83970=CARTESIAN_POINT('Ctrl Pts',(46.8598412387473,263.8,22.4654715721611)) ;
#83971=CARTESIAN_POINT('Ctrl Pts',(46.8477758406621,263.8,22.4957558005747)) ;
#83972=CARTESIAN_POINT('Ctrl Pts',(46.8423100875593,263.8,22.5117353108167)) ;
#83973=CARTESIAN_POINT('Ctrl Pts',(46.8256552051007,263.8,22.5652110982458)) ;
#83974=CARTESIAN_POINT('Ctrl Pts',(46.8153863576338,263.8,22.6074731645702)) ;
#83975=CARTESIAN_POINT('Ctrl Pts',(46.7300045475566,263.8,22.9981150219511)) ;
#83976=CARTESIAN_POINT('Ctrl Pts',(46.6572960858892,263.799999999947,23.7292172541206)) ;
#83977=CARTESIAN_POINT('Ctrl Pts',(46.5036802672985,263.799999999947,25.4441081278137)) ;
#83978=CARTESIAN_POINT('Ctrl Pts',(46.4331431886047,263.8,26.2891665072701)) ;
#83979=CARTESIAN_POINT('Ctrl Pts',(46.3578902499069,263.8,27.0760131852921)) ;
#83980=CARTESIAN_POINT('',(46.2006436754682,263.8,30.3213203435596)) ;
#83981=CARTESIAN_POINT('Origin',(47.9,263.8,30.5483813234279)) ;
#83982=CARTESIAN_POINT('',(32.5414213562372,263.8,30.3213203435596)) ;
#83983=CARTESIAN_POINT('',(66.4499999999999,263.8,30.3213203435596)) ;
#83984=CARTESIAN_POINT('',(32.4585786437627,263.8,30.3247636574754)) ;
#83985=CARTESIAN_POINT('Origin',(32.5414213562372,263.8,30.8213203435596)) ;
#83986=CARTESIAN_POINT('',(32.3585786437627,263.8,30.331422395003)) ;
#83987=CARTESIAN_POINT('Ctrl Pts',(32.3585786437627,263.8,30.331422395003)) ;
#83988=CARTESIAN_POINT('Ctrl Pts',(32.3919863317222,263.8,30.331422395003)) ;
#83989=CARTESIAN_POINT('Ctrl Pts',(32.4252483895324,263.8,30.3275439731426)) ;
#83990=CARTESIAN_POINT('Ctrl Pts',(32.4585786437628,263.8,30.3247636574754)) ;
#83991=CARTESIAN_POINT('',(28.3,263.8,30.331422395003)) ;
#83992=CARTESIAN_POINT('',(43.45,263.8,30.331422395003)) ;
#83993=CARTESIAN_POINT('',(28.1267949192431,263.8,30.3213203435596)) ;
#83994=CARTESIAN_POINT('Ctrl Pts',(28.1267949192431,263.8,30.3213203435596)) ;
#83995=CARTESIAN_POINT('Ctrl Pts',(28.1557233556092,263.8,30.3213203435596)) ;
#83996=CARTESIAN_POINT('Ctrl Pts',(28.2134628330395,263.8,30.3254695601432)) ;
#83997=CARTESIAN_POINT('Ctrl Pts',(28.2710715636338,263.8,30.331422395003)) ;
#83998=CARTESIAN_POINT('Ctrl Pts',(28.2999999999999,263.8,30.331422395003)) ;
#83999=CARTESIAN_POINT('',(66.4499999999999,263.8,30.3213203435596)) ;
#84000=CARTESIAN_POINT('Origin',(66.4499999999999,264.9,20.0213203435596)) ;
#84001=CARTESIAN_POINT('Origin',(77.1999999999999,264.9,20.0213203435596)) ;
#84002=CARTESIAN_POINT('Origin',(66.4499999999999,263.4,30.3213203435596)) ;
#84003=CARTESIAN_POINT('Ctrl Pts',(46.2376487793589,263.4,30.7213203435596)) ;
#84004=CARTESIAN_POINT('Ctrl Pts',(46.2326137620506,263.424040519058,30.7213203435596)) ;
#84005=CARTESIAN_POINT('Ctrl Pts',(46.2281249082703,263.448476883063,30.71912697103)) ;
#84006=CARTESIAN_POINT('Ctrl Pts',(46.2158136627296,263.525131463702,30.7049856843152)) ;
#84007=CARTESIAN_POINT('Ctrl Pts',(46.2103971054,263.576067017857,30.6840778621322)) ;
#84008=CARTESIAN_POINT('Ctrl Pts',(46.2038518923002,263.660659692702,30.6288392064935)) ;
#84009=CARTESIAN_POINT('Ctrl Pts',(46.2022098218577,263.700010832306,30.591200326939)) ;
#84010=CARTESIAN_POINT('Ctrl Pts',(46.2005618251513,263.760218076329,30.5032121921945)) ;
#84011=CARTESIAN_POINT('Ctrl Pts',(46.2004291717567,263.781074440706,30.4528655341031)) ;
#84012=CARTESIAN_POINT('Ctrl Pts',(46.2004291717567,263.791419913995,30.4037245359795)) ;
#84013=CARTESIAN_POINT('Ctrl Pts',(46.2004291717567,263.796960438797,30.3774070431671)) ;
#84014=CARTESIAN_POINT('Ctrl Pts',(46.2004835410982,263.8,30.3495592495545)) ;
#84015=CARTESIAN_POINT('Ctrl Pts',(46.2006436754682,263.8,30.3213203435596)) ;
#84016=CARTESIAN_POINT('Origin',(32.5414213562372,263.4,30.3213203435596)) ;
#84017=CARTESIAN_POINT('Ctrl Pts',(32.5414213562372,263.8,30.3213203435596)) ;
#84018=CARTESIAN_POINT('Ctrl Pts',(32.5137435539536,263.8,30.3213203435596)) ;
#84019=CARTESIAN_POINT('Ctrl Pts',(32.4860658393229,263.8,30.3224707532589)) ;
#84020=CARTESIAN_POINT('Ctrl Pts',(32.4585786437627,263.8,30.3247636574754)) ;
#84021=CARTESIAN_POINT('Ctrl Pts',(32.5414213562372,263.8,30.4260400986793)) ;
#84022=CARTESIAN_POINT('Ctrl Pts',(32.516647311045,263.799939841784,30.4241767924342)) ;
#84023=CARTESIAN_POINT('Ctrl Pts',(32.4917066372636,263.800050776884,30.4233947555209)) ;
#84024=CARTESIAN_POINT('Ctrl Pts',(32.4668242027051,263.8,30.4236109139464)) ;
#84025=CARTESIAN_POINT('Ctrl Pts',(32.5414213562372,263.713177767049,30.6344981106088)) ;
#84026=CARTESIAN_POINT('Ctrl Pts',(32.5224039013355,263.716415820393,30.6290758165712)) ;
#84027=CARTESIAN_POINT('Ctrl Pts',(32.5029543565148,263.719507392095,30.6243705183387)) ;
#84028=CARTESIAN_POINT('Ctrl Pts',(32.4832538801415,263.722531687981,30.6205688825484)) ;
#84029=CARTESIAN_POINT('Ctrl Pts',(32.5414213562372,263.50471975512,30.7213203435597)) ;
#84030=CARTESIAN_POINT('Ctrl Pts',(32.5248379622831,263.513950857204,30.7183564282524)) ;
#84031=CARTESIAN_POINT('Ctrl Pts',(32.5079533734914,263.523051108391,30.7159641292369)) ;
#84032=CARTESIAN_POINT('Ctrl Pts',(32.4910326442839,263.531986701662,30.7138202314961)) ;
#84033=CARTESIAN_POINT('Ctrl Pts',(32.5414213562372,263.4,30.7213203435596)) ;
#84034=CARTESIAN_POINT('Ctrl Pts',(32.524814674867,263.411071120913,30.7213203435596)) ;
#84035=CARTESIAN_POINT('Ctrl Pts',(32.5082080460886,263.422142206766,30.7215504254995)) ;
#84036=CARTESIAN_POINT('Ctrl Pts',(32.4917157287525,263.43313708499,30.7220090063428)) ;
#84037=CARTESIAN_POINT('',(32.4917157287525,263.43313708499,30.7220090063428)) ;
#84038=CARTESIAN_POINT('Origin',(32.4585786437627,263.4,30.3247636574754)) ;
#84039=CARTESIAN_POINT('Origin',(32.5414213562372,263.4,30.8213203435596)) ;
#84040=CARTESIAN_POINT('Ctrl Pts',(32.4661974061031,263.8,30.3241495482157)) ;
#84041=CARTESIAN_POINT('Ctrl Pts',(32.427775427709,263.8,30.3271273965861)) ;
#84042=CARTESIAN_POINT('Ctrl Pts',(32.3894656419897,263.8,30.3320669171698)) ;
#84043=CARTESIAN_POINT('Ctrl Pts',(32.35094083609,263.8,30.331352667432)) ;
#84044=CARTESIAN_POINT('Ctrl Pts',(32.4739550747079,263.800023048002,30.4237405302309)) ;
#84045=CARTESIAN_POINT('Ctrl Pts',(32.4384840003436,263.799890383199,30.4230691207513)) ;
#84046=CARTESIAN_POINT('Ctrl Pts',(32.3956007239745,263.800015403833,30.4226634961011)) ;
#84047=CARTESIAN_POINT('Ctrl Pts',(32.3494742105276,263.799998368455,30.4227242881205)) ;
#84048=CARTESIAN_POINT('Ctrl Pts',(32.489423057882,263.721324324522,30.6222814519142)) ;
#84049=CARTESIAN_POINT('Ctrl Pts',(32.4598454616252,263.726901760206,30.614607325942)) ;
#84050=CARTESIAN_POINT('Ctrl Pts',(32.4078143613243,263.735991513718,30.6035180183888)) ;
#84051=CARTESIAN_POINT('Ctrl Pts',(32.3465538177013,263.734676655515,30.605126476162)) ;
#84052=CARTESIAN_POINT('Ctrl Pts',(32.4966185134649,263.528321623589,30.7148404386893)) ;
#84053=CARTESIAN_POINT('Ctrl Pts',(32.4704413404425,263.544604892099,30.7105178580992)) ;
#84054=CARTESIAN_POINT('Ctrl Pts',(32.4147657809408,263.57288534838,30.7044385729834)) ;
#84055=CARTESIAN_POINT('Ctrl Pts',(32.3449157225414,263.56879986086,30.7053209268799)) ;
#84056=CARTESIAN_POINT('Ctrl Pts',(32.4971643394536,263.428547221079,30.7219188515075)) ;
#84057=CARTESIAN_POINT('Ctrl Pts',(32.4716769894707,263.448435108365,30.722537008849)) ;
#84058=CARTESIAN_POINT('Ctrl Pts',(32.4160802382908,263.484256591046,30.7235573712385)) ;
#84059=CARTESIAN_POINT('Ctrl Pts',(32.3446178057178,263.479085396975,30.7234098127246)) ;
#84060=CARTESIAN_POINT('',(32.3585786437627,263.48,30.7233407538483)) ;
#84061=CARTESIAN_POINT('Origin',(32.3585786437627,263.4,30.331422395003)) ;
#84062=CARTESIAN_POINT('Ctrl Pts',(32.4917157287525,263.43313708499,30.7220090063427)) ;
#84063=CARTESIAN_POINT('Ctrl Pts',(32.4862531044155,263.437172850683,30.7221280308607)) ;
#84064=CARTESIAN_POINT('Ctrl Pts',(32.4799268910377,263.441637838602,30.7222567124468)) ;
#84065=CARTESIAN_POINT('Ctrl Pts',(32.4726883818981,263.446171330639,30.7223863480612)) ;
#84066=CARTESIAN_POINT('Ctrl Pts',(32.4660437256829,263.450332891461,30.7225053482689)) ;
#84067=CARTESIAN_POINT('Ctrl Pts',(32.4586288871471,263.454550717319,30.7226250788745)) ;
#84068=CARTESIAN_POINT('Ctrl Pts',(32.4504481493401,263.458527237894,30.7227376232999)) ;
#84069=CARTESIAN_POINT('Ctrl Pts',(32.4429648306756,263.462164754625,30.7228405731583)) ;
#84070=CARTESIAN_POINT('Ctrl Pts',(32.4348405192778,263.46559929887,30.7229374604874)) ;
#84071=CARTESIAN_POINT('Ctrl Pts',(32.4261242620743,263.468603798031,30.7230220080826)) ;
#84072=CARTESIAN_POINT('Ctrl Pts',(32.4176398736902,263.471528371869,30.7231043065529)) ;
#84073=CARTESIAN_POINT('Ctrl Pts',(32.4085946242033,263.474044542166,30.7231748710841)) ;
#84074=CARTESIAN_POINT('Ctrl Pts',(32.3990802048924,263.475957726272,30.7232283375603)) ;
#84075=CARTESIAN_POINT('Ctrl Pts',(32.3897735748965,263.477829127564,30.7232806363602)) ;
#84076=CARTESIAN_POINT('Ctrl Pts',(32.3800184348618,263.479122788557,30.7233165339942)) ;
#84077=CARTESIAN_POINT('Ctrl Pts',(32.3699426275149,263.479683772191,30.7233320336986)) ;
#84078=CARTESIAN_POINT('Ctrl Pts',(32.3661959536449,263.479892373115,30.7233377972404)) ;
#84079=CARTESIAN_POINT('Ctrl Pts',(32.3624053322483,263.48,30.7233407538483)) ;
#84080=CARTESIAN_POINT('Ctrl Pts',(32.3585786437627,263.48,30.7233407538483)) ;
#84081=CARTESIAN_POINT('Origin',(43.45,263.4,30.331422395003)) ;
#84082=CARTESIAN_POINT('',(28.3,263.48,30.7233407538483)) ;
#84083=CARTESIAN_POINT('Origin',(28.3,263.4,30.331422395003)) ;
#84084=CARTESIAN_POINT('',(43.45,263.48,30.7233407538483)) ;
#84085=CARTESIAN_POINT('Ctrl Pts',(28.2999999999999,263.8,30.331422395003)) ;
#84086=CARTESIAN_POINT('Ctrl Pts',(28.2710715636338,263.8,30.331422395003)) ;
#84087=CARTESIAN_POINT('Ctrl Pts',(28.2134628330395,263.8,30.3254695601432)) ;
#84088=CARTESIAN_POINT('Ctrl Pts',(28.1557233556092,263.8,30.3213203435596)) ;
#84089=CARTESIAN_POINT('Ctrl Pts',(28.1267949192431,263.8,30.3213203435596)) ;
#84090=CARTESIAN_POINT('Ctrl Pts',(28.2999999999999,263.8,30.4227182887366)) ;
#84091=CARTESIAN_POINT('Ctrl Pts',(28.2656750347894,263.8,30.4227182887366)) ;
#84092=CARTESIAN_POINT('Ctrl Pts',(28.201063490636,263.79998336013,30.4232854950333)) ;
#84093=CARTESIAN_POINT('Ctrl Pts',(28.1511709085951,263.799945547361,30.4243535136987)) ;
#84094=CARTESIAN_POINT('Ctrl Pts',(28.1267949192431,263.8,30.4260400986793)) ;
#84095=CARTESIAN_POINT('Ctrl Pts',(28.2999999999999,263.734854968624,30.6048303319916)) ;
#84096=CARTESIAN_POINT('Ctrl Pts',(28.2549355475455,263.734854968624,30.6048303319916)) ;
#84097=CARTESIAN_POINT('Ctrl Pts',(28.1764296104343,263.723817492061,30.6182710292689)) ;
#84098=CARTESIAN_POINT('Ctrl Pts',(28.1421458519343,263.716108985329,30.6295903534867)) ;
#84099=CARTESIAN_POINT('Ctrl Pts',(28.1267949192431,263.713178038174,30.634498381734)) ;
#84100=CARTESIAN_POINT('Ctrl Pts',(28.3,263.569451342103,30.7050815751016)) ;
#84101=CARTESIAN_POINT('Ctrl Pts',(28.2489802156405,263.569451342103,30.7050815751016)) ;
#84102=CARTESIAN_POINT('Ctrl Pts',(28.1644027263672,263.535328707411,30.7126199315049)) ;
#84103=CARTESIAN_POINT('Ctrl Pts',(28.1383297842868,263.513075353224,30.7186375344111)) ;
#84104=CARTESIAN_POINT('Ctrl Pts',(28.1267949192431,263.50471975512,30.7213203435596)) ;
#84105=CARTESIAN_POINT('Ctrl Pts',(28.3,263.48,30.7233407538483)) ;
#84106=CARTESIAN_POINT('Ctrl Pts',(28.2479288145409,263.48,30.7233407538483)) ;
#84107=CARTESIAN_POINT('Ctrl Pts',(28.1632911232526,263.436809028867,30.7221501868763)) ;
#84108=CARTESIAN_POINT('Ctrl Pts',(28.1383662937896,263.410021104314,30.7213203435596)) ;
#84109=CARTESIAN_POINT('Ctrl Pts',(28.1267949192431,263.4,30.7213203435596)) ;
#84110=CARTESIAN_POINT('Origin',(28.1267949192431,263.4,30.3213203435596)) ;
#84111=CARTESIAN_POINT('Ctrl Pts',(28.3,263.48,30.7233407538483)) ;
#84112=CARTESIAN_POINT('Ctrl Pts',(28.2479288145409,263.48,30.7233407538483)) ;
#84113=CARTESIAN_POINT('Ctrl Pts',(28.1632911232526,263.436809028867,30.7221501868763)) ;
#84114=CARTESIAN_POINT('Ctrl Pts',(28.1383662937896,263.410021104314,30.7213203435596)) ;
#84115=CARTESIAN_POINT('Ctrl Pts',(28.1267949192431,263.4,30.7213203435596)) ;
#84116=CARTESIAN_POINT('Origin',(66.4499999999999,263.4,30.3213203435596)) ;
#84117=CARTESIAN_POINT('Origin',(26.3,252.191753592594,30.8213203435596)) ;
#84118=CARTESIAN_POINT('Origin',(26.3,245.6,30.8213203435596)) ;
#84119=CARTESIAN_POINT('Origin',(28.3,263.3,30.8213203435596)) ;
#84120=CARTESIAN_POINT('',(28.3,263.4,30.8213203435596)) ;
#84121=CARTESIAN_POINT('Origin',(28.3,263.5,30.8213203435596)) ;
#84122=CARTESIAN_POINT('',(28.2,263.3,30.8213203435596)) ;
#84123=CARTESIAN_POINT('Origin',(28.3,263.3,30.8213203435596)) ;
#84124=CARTESIAN_POINT('Origin',(28.1,263.3,30.8213203435596)) ;
#84125=CARTESIAN_POINT('Origin',(43.45,263.5,30.8213203435596)) ;
#84126=CARTESIAN_POINT('',(32.3585786437627,263.4,30.8213203435596)) ;
#84127=CARTESIAN_POINT('Origin',(32.3585786437627,263.5,30.8213203435596)) ;
#84128=CARTESIAN_POINT('',(43.45,263.4,30.8213203435596)) ;
#84129=CARTESIAN_POINT('Origin',(32.3585786437627,263.3,30.8213203435596)) ;
#84130=CARTESIAN_POINT('',(32.4292893218813,263.370710678119,30.8213203435596)) ;
#84131=CARTESIAN_POINT('Origin',(32.5,263.441421356237,30.8213203435596)) ;
#84132=CARTESIAN_POINT('Origin',(32.3585786437627,263.3,30.8213203435596)) ;
#84133=CARTESIAN_POINT('Origin',(43.9998338818216,251.941587474416,30.8213203435596)) ;
#84134=CARTESIAN_POINT('',(33.1707106781186,262.629289321881,30.8213203435596)) ;
#84135=CARTESIAN_POINT('Origin',(33.2414213562373,262.7,30.8213203435596)) ;
#84136=CARTESIAN_POINT('',(43.929123203703,251.870876796297,30.8213203435596)) ;
#84137=CARTESIAN_POINT('Origin',(66.4499999999999,263.4,30.3213203435596)) ;
#84138=CARTESIAN_POINT('Ctrl Pts',(78.1993563245318,263.8,30.3213203435596)) ;
#84139=CARTESIAN_POINT('Ctrl Pts',(78.1995164589018,263.8,30.3495592495545)) ;
#84140=CARTESIAN_POINT('Ctrl Pts',(78.1995708282433,263.796960438797,30.3774070431671)) ;
#84141=CARTESIAN_POINT('Ctrl Pts',(78.1995708282433,263.781074440706,30.4528655341031)) ;
#84142=CARTESIAN_POINT('Ctrl Pts',(78.1994381748487,263.760218076329,30.5032121921945)) ;
#84143=CARTESIAN_POINT('Ctrl Pts',(78.1977901781423,263.700010832306,30.591200326939)) ;
#84144=CARTESIAN_POINT('Ctrl Pts',(78.1961481076998,263.660659692702,30.6288392064935)) ;
#84145=CARTESIAN_POINT('Ctrl Pts',(78.1896028945999,263.576067017857,30.6840778621322)) ;
#84146=CARTESIAN_POINT('Ctrl Pts',(78.1841863372704,263.525131463702,30.7049856843151)) ;
#84147=CARTESIAN_POINT('Ctrl Pts',(78.1718750917296,263.448476883063,30.71912697103)) ;
#84148=CARTESIAN_POINT('Ctrl Pts',(78.1673862379493,263.424040519058,30.7213203435596)) ;
#84149=CARTESIAN_POINT('Ctrl Pts',(78.162351220641,263.4,30.7213203435596)) ;
#84150=CARTESIAN_POINT('Origin',(76.5,265.241264282414,23.7023759819625)) ;
#84151=CARTESIAN_POINT('Ctrl Pts',(78.0420937034656,263.800015547414,27.0760161755151)) ;
#84152=CARTESIAN_POINT('Ctrl Pts',(77.9130621118948,263.528796412695,27.018917410311)) ;
#84153=CARTESIAN_POINT('Ctrl Pts',(77.4812575809273,263.030548349122,26.9140230811377)) ;
#84154=CARTESIAN_POINT('Ctrl Pts',(76.8382263221145,262.836465365523,26.8731635056432)) ;
#84155=CARTESIAN_POINT('Ctrl Pts',(76.5,262.836465365523,26.8731635056432)) ;
#84156=CARTESIAN_POINT('Origin',(59.8573593128808,230.1,31.8213203435596)) ;
#84157=CARTESIAN_POINT('',(59.9573593128808,230.1,31.8213203435596)) ;
#84158=CARTESIAN_POINT('Origin',(59.8573593128808,230.1,31.8213203435596)) ;
#84159=CARTESIAN_POINT('',(59.8573593128808,230.,31.8213203435596)) ;
#84160=CARTESIAN_POINT('Origin',(59.8573593128808,230.1,31.8213203435596)) ;
#84161=CARTESIAN_POINT('Origin',(59.8573593128808,230.1,31.8213203435596)) ;
#84162=CARTESIAN_POINT('Origin',(56.8286796564404,230.1,31.8213203435596)) ;
#84163=CARTESIAN_POINT('',(59.7573593128808,230.,31.8213203435596)) ;
#84164=CARTESIAN_POINT('Origin',(59.7573593128808,230.1,31.8213203435596)) ;
#84165=CARTESIAN_POINT('',(56.8286796564404,230.,31.8213203435596)) ;
#84166=CARTESIAN_POINT('Origin',(59.7573593128808,229.9,31.8213203435596)) ;
#84167=CARTESIAN_POINT('',(59.6573593128808,229.9,31.8213203435596)) ;
#84168=CARTESIAN_POINT('Origin',(59.5573593128808,229.9,31.8213203435596)) ;
#84169=CARTESIAN_POINT('Origin',(59.7573593128808,229.9,31.8213203435596)) ;
#84170=CARTESIAN_POINT('Origin',(59.8573593128808,230.1,30.8213203435596)) ;
#84171=CARTESIAN_POINT('',(59.9573593128808,230.1,30.8213203435596)) ;
#84172=CARTESIAN_POINT('',(59.8573593128808,230.,30.8213203435596)) ;
#84173=CARTESIAN_POINT('Origin',(59.8573593128808,230.1,30.8213203435596)) ;
#84174=CARTESIAN_POINT('Origin',(59.8573593128808,230.1,30.8213203435596)) ;
#84175=CARTESIAN_POINT('Origin',(59.8573593128808,230.1,30.8213203435596)) ;
#84176=CARTESIAN_POINT('Origin',(59.8573593128808,230.1,19.9213203435596)) ;
#84177=CARTESIAN_POINT('',(59.9573593128808,230.1,19.9213203435596)) ;
#84178=CARTESIAN_POINT('',(59.8573593128808,230.,19.9213203435596)) ;
#84179=CARTESIAN_POINT('Origin',(62.2573593128808,235.9,31.8213203435596)) ;
#84180=CARTESIAN_POINT('',(62.2573593128808,236.,31.8213203435596)) ;
#84181=CARTESIAN_POINT('Origin',(62.2573593128808,236.1,31.8213203435596)) ;
#84182=CARTESIAN_POINT('',(62.3573593128808,235.9,31.8213203435596)) ;
#84183=CARTESIAN_POINT('Origin',(62.2573593128808,235.9,31.8213203435596)) ;
#84184=CARTESIAN_POINT('Origin',(62.4573593128808,235.9,31.8213203435596)) ;
#84185=CARTESIAN_POINT('Origin',(60.0573593128808,235.9,31.8213203435596)) ;
#84186=CARTESIAN_POINT('',(60.0573593128808,236.,31.8213203435596)) ;
#84187=CARTESIAN_POINT('',(59.9573593128808,235.9,31.8213203435596)) ;
#84188=CARTESIAN_POINT('Origin',(60.0573593128808,235.9,31.8213203435596)) ;
#84189=CARTESIAN_POINT('Origin',(60.0573593128808,236.1,31.8213203435596)) ;
#84190=CARTESIAN_POINT('Origin',(59.8573593128808,235.9,31.8213203435596)) ;
#84191=CARTESIAN_POINT('Origin',(58.0286796564404,236.1,31.8213203435596)) ;
#84192=CARTESIAN_POINT('',(58.0286796564404,236.,31.8213203435596)) ;
#84193=CARTESIAN_POINT('Origin',(59.8573593128808,237.691753592594,31.8213203435596)) ;
#84194=CARTESIAN_POINT('',(59.9573593128808,237.691753592594,31.8213203435596)) ;
#84195=CARTESIAN_POINT('Origin',(59.8573593128808,235.9,30.8213203435596)) ;
#84196=CARTESIAN_POINT('',(60.0573593128808,236.,30.8213203435596)) ;
#84197=CARTESIAN_POINT('',(59.9573593128808,235.9,30.8213203435596)) ;
#84198=CARTESIAN_POINT('Origin',(60.0573593128808,235.9,30.8213203435596)) ;
#84199=CARTESIAN_POINT('Origin',(59.8573593128808,235.9,30.8213203435596)) ;
#84200=CARTESIAN_POINT('Origin',(59.8573593128808,236.,30.8213203435596)) ;
#84201=CARTESIAN_POINT('Origin',(60.0573593128808,235.9,19.9213203435596)) ;
#84202=CARTESIAN_POINT('',(59.9573593128808,235.9,19.9213203435596)) ;
#84203=CARTESIAN_POINT('',(60.0573593128808,236.,19.9213203435596)) ;
#84204=CARTESIAN_POINT('Origin',(62.2573593128808,235.9,19.9213203435596)) ;
#84205=CARTESIAN_POINT('',(62.2573593128808,236.,30.8213203435596)) ;
#84206=CARTESIAN_POINT('',(62.3573593128808,235.9,30.8213203435596)) ;
#84207=CARTESIAN_POINT('Origin',(62.2573593128808,235.9,30.8213203435596)) ;
#84208=CARTESIAN_POINT('',(62.3573593128808,235.9,19.9213203435596)) ;
#84209=CARTESIAN_POINT('',(62.2573593128808,236.,19.9213203435596)) ;
#84210=CARTESIAN_POINT('Origin',(62.4573593128808,235.9,30.8213203435596)) ;
#84211=CARTESIAN_POINT('Origin',(62.4573593128808,235.9,30.8213203435596)) ;
#84212=CARTESIAN_POINT('Origin',(62.4573593128808,236.,30.8213203435596)) ;
#84213=CARTESIAN_POINT('Origin',(62.4573593128808,234.691753592594,31.8213203435596)) ;
#84214=CARTESIAN_POINT('',(62.3573593128808,230.1,31.8213203435596)) ;
#84215=CARTESIAN_POINT('Origin',(62.4573593128808,230.1,31.8213203435596)) ;
#84216=CARTESIAN_POINT('',(62.3573593128808,234.691753592594,31.8213203435596)) ;
#84217=CARTESIAN_POINT('Origin',(62.4573593128808,230.1,31.8213203435596)) ;
#84218=CARTESIAN_POINT('',(62.4573593128808,230.,31.8213203435596)) ;
#84219=CARTESIAN_POINT('Origin',(62.4573593128808,230.1,31.8213203435596)) ;
#84220=CARTESIAN_POINT('Origin',(62.4573593128808,230.1,31.8213203435596)) ;
#84221=CARTESIAN_POINT('Origin',(56.8286796564404,230.1,30.8213203435596)) ;
#84222=CARTESIAN_POINT('',(59.7573593128808,230.,30.8213203435596)) ;
#84223=CARTESIAN_POINT('',(56.8286796564404,230.,30.8213203435596)) ;
#84224=CARTESIAN_POINT('Origin',(59.7573593128808,230.1,30.8213203435596)) ;
#84225=CARTESIAN_POINT('Origin',(59.9573593128808,230.,19.9213203435596)) ;
#84226=CARTESIAN_POINT('',(59.7573593128808,230.,19.9213203435596)) ;
#84227=CARTESIAN_POINT('Origin',(58.1786796564404,230.1,31.8213203435596)) ;
#84228=CARTESIAN_POINT('',(62.5573593128808,230.,31.8213203435596)) ;
#84229=CARTESIAN_POINT('',(58.1786796564404,230.,31.8213203435596)) ;
#84230=CARTESIAN_POINT('Origin',(62.5573593128808,230.1,31.8213203435596)) ;
#84231=CARTESIAN_POINT('Origin',(62.4573593128808,230.1,19.9213203435596)) ;
#84232=CARTESIAN_POINT('',(62.3573593128808,230.1,30.8213203435596)) ;
#84233=CARTESIAN_POINT('',(62.3573593128808,230.1,19.9213203435596)) ;
#84234=CARTESIAN_POINT('',(62.4573593128808,230.,30.8213203435596)) ;
#84235=CARTESIAN_POINT('Origin',(62.4573593128808,230.1,30.8213203435596)) ;
#84236=CARTESIAN_POINT('',(62.4573593128808,230.,19.9213203435596)) ;
#84237=CARTESIAN_POINT('Origin',(62.3573593128808,230.,19.9213203435596)) ;
#84238=CARTESIAN_POINT('',(62.3573593128808,234.691753592594,30.8213203435596)) ;
#84239=CARTESIAN_POINT('Origin',(58.0573593128808,237.9,30.8213203435596)) ;
#84240=CARTESIAN_POINT('',(57.9573593128808,238.1,30.8213203435596)) ;
#84241=CARTESIAN_POINT('',(58.0573593128808,238.,30.8213203435596)) ;
#84242=CARTESIAN_POINT('Origin',(58.0573593128808,238.1,30.8213203435596)) ;
#84243=CARTESIAN_POINT('Origin',(58.0573593128808,237.9,30.8213203435596)) ;
#84244=CARTESIAN_POINT('Origin',(57.9573593128808,237.9,30.8213203435596)) ;
#84245=CARTESIAN_POINT('Origin',(58.0573593128808,238.1,19.9213203435596)) ;
#84246=CARTESIAN_POINT('',(57.9573593128808,238.1,31.8213203435596)) ;
#84247=CARTESIAN_POINT('',(58.0573593128808,238.,31.8213203435596)) ;
#84248=CARTESIAN_POINT('Origin',(58.0573593128808,238.1,31.8213203435596)) ;
#84249=CARTESIAN_POINT('',(58.0573593128808,238.,19.9213203435596)) ;
#84250=CARTESIAN_POINT('',(57.9573593128808,238.1,19.9213203435596)) ;
#84251=CARTESIAN_POINT('Ctrl Pts',(58.0573593128808,238.,31.8213203435596)) ;
#84252=CARTESIAN_POINT('Ctrl Pts',(58.0573593128808,238.,31.8736802211195)) ;
#84253=CARTESIAN_POINT('Ctrl Pts',(57.9620790680004,237.95235987756,31.9213203435596)) ;
#84254=CARTESIAN_POINT('Ctrl Pts',(57.8573593128808,237.9,31.9213203435596)) ;
#84255=CARTESIAN_POINT('Ctrl Pts',(58.0274393828466,238.,31.8213203435596)) ;
#84256=CARTESIAN_POINT('Ctrl Pts',(58.0274393828466,238.,31.8577789708945)) ;
#84257=CARTESIAN_POINT('Ctrl Pts',(57.952105757989,237.962333187571,31.9213203435596)) ;
#84258=CARTESIAN_POINT('Ctrl Pts',(57.8573593128808,237.9,31.9213203435596)) ;
#84259=CARTESIAN_POINT('Ctrl Pts',(57.975662586397,238.025132309007,31.8213203435596)) ;
#84260=CARTESIAN_POINT('Ctrl Pts',(57.975662586397,238.025132309007,31.8441177712024)) ;
#84261=CARTESIAN_POINT('Ctrl Pts',(57.9346524654691,237.979786480091,31.9213203435596)) ;
#84262=CARTESIAN_POINT('Ctrl Pts',(57.8573593128808,237.9,31.9213203435596)) ;
#84263=CARTESIAN_POINT('Ctrl Pts',(57.9573593128808,238.077560052474,31.8213203435596)) ;
#84264=CARTESIAN_POINT('Ctrl Pts',(57.9573593128808,238.077560052474,31.8619121713414)) ;
#84265=CARTESIAN_POINT('Ctrl Pts',(57.9171991729491,237.997239772611,31.9213203435596)) ;
#84266=CARTESIAN_POINT('Ctrl Pts',(57.8573593128808,237.9,31.9213203435596)) ;
#84267=CARTESIAN_POINT('Ctrl Pts',(57.9573593128808,238.1,31.8213203435596)) ;
#84268=CARTESIAN_POINT('Ctrl Pts',(57.9573593128808,238.1,31.8736802211195)) ;
#84269=CARTESIAN_POINT('Ctrl Pts',(57.9097191904406,238.00471975512,31.9213203435596)) ;
#84270=CARTESIAN_POINT('Ctrl Pts',(57.8573593128808,237.9,31.9213203435596)) ;
#84271=CARTESIAN_POINT('Origin',(57.8573593128808,237.9,31.8213203435596)) ;
#84272=CARTESIAN_POINT('Origin',(57.8573593128808,237.9,31.8213203435596)) ;
#84273=CARTESIAN_POINT('Origin',(57.8573593128808,241.191753592594,31.8213203435596)) ;
#84274=CARTESIAN_POINT('',(57.9573593128808,239.1,31.8213203435596)) ;
#84275=CARTESIAN_POINT('',(57.9573593128808,241.191753592594,31.8213203435596)) ;
#84276=CARTESIAN_POINT('Origin',(57.8573593128808,239.2,31.8213203435596)) ;
#84277=CARTESIAN_POINT('Origin',(57.9573593128808,243.,19.9213203435596)) ;
#84278=CARTESIAN_POINT('',(57.9573593128808,239.1,22.9213203435596)) ;
#84279=CARTESIAN_POINT('Ctrl Pts',(57.9573593128808,242.9,31.8213203435596)) ;
#84280=CARTESIAN_POINT('Ctrl Pts',(57.9573593128808,242.9,31.8736802211195)) ;
#84281=CARTESIAN_POINT('Ctrl Pts',(57.9097191904406,242.99528024488,31.9213203435596)) ;
#84282=CARTESIAN_POINT('Ctrl Pts',(57.8573593128808,243.1,31.9213203435596)) ;
#84283=CARTESIAN_POINT('Ctrl Pts',(57.9573593128808,242.929919930034,31.8213203435596)) ;
#84284=CARTESIAN_POINT('Ctrl Pts',(57.9573593128808,242.929919930034,31.8577789708945)) ;
#84285=CARTESIAN_POINT('Ctrl Pts',(57.919692500452,243.005253554892,31.9213203435596)) ;
#84286=CARTESIAN_POINT('Ctrl Pts',(57.8573593128808,243.1,31.9213203435596)) ;
#84287=CARTESIAN_POINT('Ctrl Pts',(57.9824916671412,242.981696672186,31.8213203435596)) ;
#84288=CARTESIAN_POINT('Ctrl Pts',(57.9824916671412,242.981696672186,31.8441177712024)) ;
#84289=CARTESIAN_POINT('Ctrl Pts',(57.9371457929719,243.022706847412,31.9213203435596)) ;
#84290=CARTESIAN_POINT('Ctrl Pts',(57.8573593128808,243.1,31.9213203435596)) ;
#84291=CARTESIAN_POINT('Ctrl Pts',(58.0349193653551,243.,31.8213203435596)) ;
#84292=CARTESIAN_POINT('Ctrl Pts',(58.0349193653551,243.,31.8619121713414)) ;
#84293=CARTESIAN_POINT('Ctrl Pts',(57.9545990854919,243.040160139932,31.9213203435596)) ;
#84294=CARTESIAN_POINT('Ctrl Pts',(57.8573593128808,243.1,31.9213203435596)) ;
#84295=CARTESIAN_POINT('Ctrl Pts',(58.0573593128808,243.,31.8213203435596)) ;
#84296=CARTESIAN_POINT('Ctrl Pts',(58.0573593128808,243.,31.8736802211195)) ;
#84297=CARTESIAN_POINT('Ctrl Pts',(57.9620790680004,243.04764012244,31.9213203435596)) ;
#84298=CARTESIAN_POINT('Ctrl Pts',(57.8573593128808,243.1,31.9213203435596)) ;
#84299=CARTESIAN_POINT('',(57.9573593128808,242.9,31.8213203435596)) ;
#84300=CARTESIAN_POINT('',(58.0573593128808,243.,31.8213203435596)) ;
#84301=CARTESIAN_POINT('Origin',(58.0573593128808,242.9,31.8213203435596)) ;
#84302=CARTESIAN_POINT('Origin',(57.8573593128808,243.1,31.8213203435596)) ;
#84303=CARTESIAN_POINT('Origin',(57.8573593128808,243.1,31.8213203435596)) ;
#84304=CARTESIAN_POINT('Origin',(58.0573593128808,242.9,19.9213203435596)) ;
#84305=CARTESIAN_POINT('',(57.9573593128808,242.9,30.8213203435596)) ;
#84306=CARTESIAN_POINT('',(58.0573593128808,243.,30.8213203435596)) ;
#84307=CARTESIAN_POINT('Origin',(58.0573593128808,242.9,30.8213203435596)) ;
#84308=CARTESIAN_POINT('',(58.0573593128808,243.,19.9213203435596)) ;
#84309=CARTESIAN_POINT('',(57.9573593128808,242.9,19.9213203435596)) ;
#84310=CARTESIAN_POINT('Origin',(58.0573593128808,243.1,30.8213203435596)) ;
#84311=CARTESIAN_POINT('Origin',(58.0573593128808,243.1,30.8213203435596)) ;
#84312=CARTESIAN_POINT('Origin',(57.9573593128808,243.1,30.8213203435596)) ;
#84313=CARTESIAN_POINT('Origin',(57.9573593128808,243.,19.9213203435596)) ;
#84314=CARTESIAN_POINT('',(57.9573593128808,241.9,31.8213203435596)) ;
#84315=CARTESIAN_POINT('',(57.9573593128808,241.191753592594,31.8213203435596)) ;
#84316=CARTESIAN_POINT('',(57.9573593128808,241.9,22.9213203435596)) ;
#84317=CARTESIAN_POINT('Origin',(57.8573593128808,241.191753592594,31.8213203435596)) ;
#84318=CARTESIAN_POINT('Origin',(57.8573593128807,241.8,31.8213203435596)) ;
#84319=CARTESIAN_POINT('Origin',(40.95,258.3,30.8213203435596)) ;
#84320=CARTESIAN_POINT('',(32.3585786437627,258.4,30.8213203435596)) ;
#84321=CARTESIAN_POINT('Origin',(32.3585786437627,258.3,30.8213203435596)) ;
#84322=CARTESIAN_POINT('',(28.2,258.4,30.8213203435596)) ;
#84323=CARTESIAN_POINT('Origin',(28.1999999999999,258.3,30.8213203435596)) ;
#84324=CARTESIAN_POINT('',(40.95,258.4,30.8213203435596)) ;
#84325=CARTESIAN_POINT('Origin',(32.3585786437627,258.5,30.8213203435596)) ;
#84326=CARTESIAN_POINT('',(32.4292893218813,258.429289321881,30.8213203435596)) ;
#84327=CARTESIAN_POINT('Origin',(32.5,258.358578643763,30.8213203435596)) ;
#84328=CARTESIAN_POINT('Origin',(32.3585786437627,258.5,30.8213203435596)) ;
#84329=CARTESIAN_POINT('Origin',(33.2415874744158,259.100166118179,30.8213203435596)) ;
#84330=CARTESIAN_POINT('',(33.1707106781186,259.170710678119,30.8213203435596)) ;
#84331=CARTESIAN_POINT('Origin',(33.2414213562373,259.1,30.8213203435596)) ;
#84332=CARTESIAN_POINT('',(33.1708767962972,259.170876796297,30.8213203435596)) ;
#84333=CARTESIAN_POINT('Origin',(33.1,259.241421356237,30.8213203435596)) ;
#84334=CARTESIAN_POINT('',(33.2,259.241421356237,30.8213203435596)) ;
#84335=CARTESIAN_POINT('Origin',(33.3,259.241421356237,30.8213203435596)) ;
#84336=CARTESIAN_POINT('Origin',(33.1,259.241421356237,30.8213203435596)) ;
#84337=CARTESIAN_POINT('Origin',(33.2999999999999,248.891753592594,30.8213203435596)) ;
#84338=CARTESIAN_POINT('',(33.2,262.558578643763,30.8213203435596)) ;
#84339=CARTESIAN_POINT('Origin',(33.2999999999999,262.558578643763,30.8213203435596)) ;
#84340=CARTESIAN_POINT('',(33.2,248.891753592594,30.8213203435596)) ;
#84341=CARTESIAN_POINT('Origin',(33.1,262.558578643763,30.8213203435596)) ;
#84342=CARTESIAN_POINT('Origin',(33.1,262.558578643763,30.8213203435596)) ;
#84343=CARTESIAN_POINT('Origin',(28.1,251.391753592594,30.8213203435596)) ;
#84344=CARTESIAN_POINT('',(28.2,262.3,30.8213203435596)) ;
#84345=CARTESIAN_POINT('Origin',(28.1,262.3,30.8213203435596)) ;
#84346=CARTESIAN_POINT('',(28.2,251.391753592594,30.8213203435596)) ;
#84347=CARTESIAN_POINT('Origin',(28.2,263.4,19.9213203435596)) ;
#84348=CARTESIAN_POINT('',(28.1999999999999,263.3,31.8213203435596)) ;
#84349=CARTESIAN_POINT('',(28.2,263.3,19.9213203435596)) ;
#84350=CARTESIAN_POINT('',(28.2,262.3,31.8213203435596)) ;
#84351=CARTESIAN_POINT('',(28.1999999999999,251.391753592594,31.8213203435596)) ;
#84352=CARTESIAN_POINT('',(28.2,262.3,22.9213203435596)) ;
#84353=CARTESIAN_POINT('Origin',(28.3,263.3,19.9213203435596)) ;
#84354=CARTESIAN_POINT('',(28.2999999999999,263.4,31.8213203435596)) ;
#84355=CARTESIAN_POINT('',(28.3,263.4,19.9213203435596)) ;
#84356=CARTESIAN_POINT('Origin',(28.2999999999999,263.3,31.8213203435596)) ;
#84357=CARTESIAN_POINT('Origin',(33.2,263.4,19.9213203435596)) ;
#84358=CARTESIAN_POINT('',(32.3585786437627,263.4,31.8213203435596)) ;
#84359=CARTESIAN_POINT('',(32.3585786437627,263.4,19.9213203435596)) ;
#84360=CARTESIAN_POINT('',(43.45,263.4,31.8213203435596)) ;
#84361=CARTESIAN_POINT('Origin',(32.3585786437627,263.3,19.9213203435596)) ;
#84362=CARTESIAN_POINT('',(32.4292893218813,263.370710678119,31.8213203435596)) ;
#84363=CARTESIAN_POINT('',(32.4292893218813,263.370710678119,19.9213203435596)) ;
#84364=CARTESIAN_POINT('Origin',(32.3585786437627,263.3,31.8213203435596)) ;
#84365=CARTESIAN_POINT('Origin',(32.8,263.,19.9213203435596)) ;
#84366=CARTESIAN_POINT('',(33.1707106781186,262.629289321881,31.8213203435596)) ;
#84367=CARTESIAN_POINT('',(33.1707106781186,262.629289321881,19.9213203435596)) ;
#84368=CARTESIAN_POINT('',(43.929123203703,251.870876796297,31.8213203435596)) ;
#84369=CARTESIAN_POINT('Origin',(33.1,262.558578643763,19.9213203435596)) ;
#84370=CARTESIAN_POINT('',(33.1999999999999,262.558578643763,31.8213203435596)) ;
#84371=CARTESIAN_POINT('',(33.2,262.558578643763,19.9213203435596)) ;
#84372=CARTESIAN_POINT('Origin',(33.1,262.558578643763,31.8213203435596)) ;
#84373=CARTESIAN_POINT('Origin',(33.2,258.4,19.9213203435596)) ;
#84374=CARTESIAN_POINT('',(33.1999999999999,259.241421356237,31.8213203435596)) ;
#84375=CARTESIAN_POINT('',(33.2,259.241421356237,19.9213203435596)) ;
#84376=CARTESIAN_POINT('',(33.1999999999999,248.891753592594,31.8213203435596)) ;
#84377=CARTESIAN_POINT('Origin',(33.1,259.241421356237,19.9213203435596)) ;
#84378=CARTESIAN_POINT('',(33.1707106781186,259.170710678119,31.8213203435596)) ;
#84379=CARTESIAN_POINT('',(33.1707106781186,259.170710678119,19.9213203435596)) ;
#84380=CARTESIAN_POINT('Origin',(33.1,259.241421356237,31.8213203435596)) ;
#84381=CARTESIAN_POINT('Origin',(32.8,258.8,19.9213203435596)) ;
#84382=CARTESIAN_POINT('',(32.4292893218813,258.429289321881,31.8213203435596)) ;
#84383=CARTESIAN_POINT('',(32.4292893218813,258.429289321881,19.9213203435596)) ;
#84384=CARTESIAN_POINT('',(33.1708767962972,259.170876796297,31.8213203435596)) ;
#84385=CARTESIAN_POINT('Origin',(32.3585786437627,258.5,19.9213203435596)) ;
#84386=CARTESIAN_POINT('',(32.3585786437627,258.4,31.8213203435596)) ;
#84387=CARTESIAN_POINT('',(32.3585786437627,258.4,19.9213203435596)) ;
#84388=CARTESIAN_POINT('Origin',(32.3585786437627,258.5,31.8213203435596)) ;
#84389=CARTESIAN_POINT('Origin',(28.2,258.4,19.9213203435596)) ;
#84390=CARTESIAN_POINT('',(28.1999999999999,258.4,31.8213203435596)) ;
#84391=CARTESIAN_POINT('',(28.2,258.4,19.9213203435596)) ;
#84392=CARTESIAN_POINT('',(40.95,258.4,31.8213203435596)) ;
#84393=CARTESIAN_POINT('Origin',(64.1,226.1,30.8213203435596)) ;
#84394=CARTESIAN_POINT('',(74.3999999999999,226.,30.8213203435596)) ;
#84395=CARTESIAN_POINT('Origin',(74.3999999999999,226.1,30.8213203435596)) ;
#84396=CARTESIAN_POINT('',(74.2999999999999,226.,30.8213203435596)) ;
#84397=CARTESIAN_POINT('',(64.1,226.,30.8213203435596)) ;
#84398=CARTESIAN_POINT('Origin',(74.2999999999999,226.1,30.8213203435596)) ;
#84399=CARTESIAN_POINT('Origin',(74.3999999999999,225.9,30.8213203435596)) ;
#84400=CARTESIAN_POINT('',(74.4999999999999,225.9,30.8213203435596)) ;
#84401=CARTESIAN_POINT('Origin',(74.6,225.9,30.8213203435596)) ;
#84402=CARTESIAN_POINT('Origin',(74.3999999999999,225.9,30.8213203435596)) ;
#84403=CARTESIAN_POINT('Origin',(74.5999999999999,231.191753592594,30.8213203435596)) ;
#84404=CARTESIAN_POINT('',(74.4999999999999,223.1,30.8213203435596)) ;
#84405=CARTESIAN_POINT('Origin',(74.5999999999999,223.1,30.8213203435596)) ;
#84406=CARTESIAN_POINT('',(74.4999999999999,231.191753592594,30.8213203435596)) ;
#84407=CARTESIAN_POINT('Origin',(74.3999999999999,223.1,30.8213203435596)) ;
#84408=CARTESIAN_POINT('',(74.3999999999999,223.,30.8213203435596)) ;
#84409=CARTESIAN_POINT('Origin',(74.3999999999999,222.9,30.8213203435596)) ;
#84410=CARTESIAN_POINT('Origin',(74.3999999999999,223.1,30.8213203435596)) ;
#84411=CARTESIAN_POINT('Origin',(62.6,222.9,30.8213203435596)) ;
#84412=CARTESIAN_POINT('',(71.5999999999999,223.,30.8213203435596)) ;
#84413=CARTESIAN_POINT('Origin',(71.5999999999999,222.9,30.8213203435596)) ;
#84414=CARTESIAN_POINT('',(62.6,223.,30.8213203435596)) ;
#84415=CARTESIAN_POINT('Origin',(71.5999999999999,223.1,30.8213203435596)) ;
#84416=CARTESIAN_POINT('',(71.4999999999999,223.1,30.8213203435596)) ;
#84417=CARTESIAN_POINT('Origin',(71.3999999999999,223.1,30.8213203435596)) ;
#84418=CARTESIAN_POINT('Origin',(71.5999999999999,223.1,30.8213203435596)) ;
#84419=CARTESIAN_POINT('Origin',(71.3999999999999,232.691753592594,30.8213203435596)) ;
#84420=CARTESIAN_POINT('',(71.4999999999999,225.9,30.8213203435596)) ;
#84421=CARTESIAN_POINT('Origin',(71.3999999999999,225.9,30.8213203435596)) ;
#84422=CARTESIAN_POINT('',(71.4999999999999,232.691753592594,30.8213203435596)) ;
#84423=CARTESIAN_POINT('Origin',(71.5999999999999,225.9,30.8213203435596)) ;
#84424=CARTESIAN_POINT('',(71.5999999999999,226.,30.8213203435596)) ;
#84425=CARTESIAN_POINT('Origin',(71.5999999999999,226.1,30.8213203435596)) ;
#84426=CARTESIAN_POINT('Origin',(71.5999999999999,225.9,30.8213203435596)) ;
#84427=CARTESIAN_POINT('Origin',(62.75,226.1,30.8213203435596)) ;
#84428=CARTESIAN_POINT('',(71.6999999999999,226.,30.8213203435596)) ;
#84429=CARTESIAN_POINT('Origin',(71.6999999999999,226.1,30.8213203435596)) ;
#84430=CARTESIAN_POINT('',(62.75,226.,30.8213203435596)) ;
#84431=CARTESIAN_POINT('Origin',(71.6999999999999,235.691753592594,30.8213203435596)) ;
#84432=CARTESIAN_POINT('',(71.7999999999999,231.9,30.8213203435596)) ;
#84433=CARTESIAN_POINT('Origin',(71.6999999999999,231.9,30.8213203435596)) ;
#84434=CARTESIAN_POINT('',(71.7999999999999,226.1,30.8213203435596)) ;
#84435=CARTESIAN_POINT('',(71.7999999999999,235.691753592594,30.8213203435596)) ;
#84436=CARTESIAN_POINT('Origin',(71.6999999999999,226.1,30.8213203435596)) ;
#84437=CARTESIAN_POINT('Origin',(71.8999999999999,231.9,30.8213203435596)) ;
#84438=CARTESIAN_POINT('',(71.8999999999999,232.,30.8213203435596)) ;
#84439=CARTESIAN_POINT('Origin',(71.8999999999999,232.1,30.8213203435596)) ;
#84440=CARTESIAN_POINT('Origin',(71.8999999999999,231.9,30.8213203435596)) ;
#84441=CARTESIAN_POINT('Origin',(63.95,232.1,30.8213203435596)) ;
#84442=CARTESIAN_POINT('',(74.0999999999999,232.,30.8213203435596)) ;
#84443=CARTESIAN_POINT('Origin',(74.0999999999999,232.1,30.8213203435596)) ;
#84444=CARTESIAN_POINT('',(63.95,232.,30.8213203435596)) ;
#84445=CARTESIAN_POINT('Origin',(74.0999999999999,231.9,30.8213203435596)) ;
#84446=CARTESIAN_POINT('',(74.1999999999999,231.9,30.8213203435596)) ;
#84447=CARTESIAN_POINT('Origin',(74.2999999999999,231.9,30.8213203435596)) ;
#84448=CARTESIAN_POINT('Origin',(74.0999999999999,231.9,30.8213203435596)) ;
#84449=CARTESIAN_POINT('Origin',(74.2999999999999,232.691753592594,30.8213203435596)) ;
#84450=CARTESIAN_POINT('',(74.1999999999999,226.1,30.8213203435596)) ;
#84451=CARTESIAN_POINT('Origin',(74.2999999999999,226.1,30.8213203435596)) ;
#84452=CARTESIAN_POINT('',(74.1999999999999,232.691753592594,30.8213203435596)) ;
#84453=CARTESIAN_POINT('Origin',(71.6999999999999,226.1,30.8213203435596)) ;
#84454=CARTESIAN_POINT('Origin',(71.6999999999999,226.1,30.8213203435596)) ;
#84455=CARTESIAN_POINT('Origin',(74.2999999999999,226.1,30.8213203435596)) ;
#84456=CARTESIAN_POINT('Origin',(74.2999999999999,226.1,30.8213203435596)) ;
#84457=CARTESIAN_POINT('Origin',(74.3999999999999,223.1,19.9213203435596)) ;
#84458=CARTESIAN_POINT('',(74.3999999999999,223.,31.8213203435596)) ;
#84459=CARTESIAN_POINT('',(74.3999999999999,223.,19.9213203435596)) ;
#84460=CARTESIAN_POINT('',(74.4999999999999,223.1,31.8213203435596)) ;
#84461=CARTESIAN_POINT('Origin',(74.3999999999999,223.1,31.8213203435596)) ;
#84462=CARTESIAN_POINT('',(74.4999999999999,223.1,19.9213203435596)) ;
#84463=CARTESIAN_POINT('Origin',(71.4999999999999,223.,19.9213203435596)) ;
#84464=CARTESIAN_POINT('',(71.5999999999999,223.,31.8213203435596)) ;
#84465=CARTESIAN_POINT('',(71.5999999999999,223.,19.9213203435596)) ;
#84466=CARTESIAN_POINT('',(62.6,223.,31.8213203435596)) ;
#84467=CARTESIAN_POINT('Origin',(71.5999999999999,223.1,19.9213203435596)) ;
#84468=CARTESIAN_POINT('',(71.4999999999999,223.1,31.8213203435596)) ;
#84469=CARTESIAN_POINT('',(71.4999999999999,223.1,19.9213203435596)) ;
#84470=CARTESIAN_POINT('Origin',(71.5999999999999,223.1,31.8213203435596)) ;
#84471=CARTESIAN_POINT('Origin',(71.4999999999999,226.,19.9213203435596)) ;
#84472=CARTESIAN_POINT('',(71.4999999999999,225.9,31.8213203435596)) ;
#84473=CARTESIAN_POINT('',(71.4999999999999,225.9,19.9213203435596)) ;
#84474=CARTESIAN_POINT('',(71.4999999999999,232.691753592594,31.8213203435596)) ;
#84475=CARTESIAN_POINT('Origin',(71.5999999999999,225.9,19.9213203435596)) ;
#84476=CARTESIAN_POINT('',(71.5999999999999,226.,31.8213203435596)) ;
#84477=CARTESIAN_POINT('',(71.5999999999999,226.,19.9213203435596)) ;
#84478=CARTESIAN_POINT('Origin',(71.5999999999999,225.9,31.8213203435596)) ;
#84479=CARTESIAN_POINT('Origin',(71.7999999999999,226.,19.9213203435596)) ;
#84480=CARTESIAN_POINT('',(71.6999999999999,226.,31.8213203435596)) ;
#84481=CARTESIAN_POINT('',(71.6999999999999,226.,19.9213203435596)) ;
#84482=CARTESIAN_POINT('',(62.75,226.,31.8213203435596)) ;
#84483=CARTESIAN_POINT('Origin',(71.6999999999999,226.1,19.9213203435596)) ;
#84484=CARTESIAN_POINT('',(71.7999999999999,226.1,31.8213203435596)) ;
#84485=CARTESIAN_POINT('',(71.7999999999999,226.1,19.9213203435596)) ;
#84486=CARTESIAN_POINT('Origin',(71.6999999999999,226.1,31.8213203435596)) ;
#84487=CARTESIAN_POINT('Origin',(71.7999999999999,232.,19.9213203435596)) ;
#84488=CARTESIAN_POINT('',(71.7999999999999,231.9,31.8213203435596)) ;
#84489=CARTESIAN_POINT('',(71.7999999999999,231.9,19.9213203435596)) ;
#84490=CARTESIAN_POINT('',(71.7999999999999,235.691753592594,31.8213203435596)) ;
#84491=CARTESIAN_POINT('Origin',(80.0999999999989,248.6,30.8213203435596)) ;
#84492=CARTESIAN_POINT('',(80.0999999999989,248.5,30.8213203435596)) ;
#84493=CARTESIAN_POINT('Origin',(80.0999999999989,248.4,30.8213203435596)) ;
#84494=CARTESIAN_POINT('',(80.199999999999,248.6,30.8213203435596)) ;
#84495=CARTESIAN_POINT('Origin',(80.0999999999989,248.6,30.8213203435596)) ;
#84496=CARTESIAN_POINT('Origin',(80.2999999999989,248.6,30.8213203435596)) ;
#84497=CARTESIAN_POINT('Origin',(80.099999999999,253.4,30.8213203435596)) ;
#84498=CARTESIAN_POINT('',(80.099999999999,253.5,30.8213203435596)) ;
#84499=CARTESIAN_POINT('',(80.199999999999,253.4,30.8213203435596)) ;
#84500=CARTESIAN_POINT('Origin',(80.099999999999,253.4,30.8213203435596)) ;
#84501=CARTESIAN_POINT('Origin',(80.099999999999,253.6,30.8213203435596)) ;
#84502=CARTESIAN_POINT('Origin',(80.299999999999,253.4,30.8213203435596)) ;
#84503=CARTESIAN_POINT('Origin',(66.9499999999995,253.6,30.8213203435596)) ;
#84504=CARTESIAN_POINT('',(76.0414213562367,253.5,30.8213203435596)) ;
#84505=CARTESIAN_POINT('Origin',(76.0414213562367,253.6,30.8213203435596)) ;
#84506=CARTESIAN_POINT('',(66.9499999999995,253.5,30.8213203435596)) ;
#84507=CARTESIAN_POINT('Origin',(76.0414213562367,253.4,30.8213203435596)) ;
#84508=CARTESIAN_POINT('',(75.9707106781181,253.470710678119,30.8213203435596)) ;
#84509=CARTESIAN_POINT('Origin',(75.8999999999994,253.541421356237,30.8213203435596)) ;
#84510=CARTESIAN_POINT('Origin',(76.0414213562367,253.4,30.8213203435596)) ;
#84511=CARTESIAN_POINT('Origin',(66.6251661181778,244.266587474416,30.8213203435596)) ;
#84512=CARTESIAN_POINT('',(75.2292893218808,252.729289321881,30.8213203435596)) ;
#84513=CARTESIAN_POINT('Origin',(75.1585786437621,252.8,30.8213203435596)) ;
#84514=CARTESIAN_POINT('',(66.6958767962964,244.195876796297,30.8213203435596)) ;
#84515=CARTESIAN_POINT('Origin',(75.2999999999994,252.658578643763,30.8213203435596)) ;
#84516=CARTESIAN_POINT('',(75.1999999999994,252.658578643763,30.8213203435596)) ;
#84517=CARTESIAN_POINT('Origin',(75.0999999999994,252.658578643763,30.8213203435596)) ;
#84518=CARTESIAN_POINT('Origin',(75.2999999999994,252.658578643763,30.8213203435596)) ;
#84519=CARTESIAN_POINT('Origin',(75.0999999999992,246.441753592594,30.8213203435596)) ;
#84520=CARTESIAN_POINT('',(75.1999999999993,249.341421356237,30.8213203435596)) ;
#84521=CARTESIAN_POINT('Origin',(75.0999999999993,249.341421356237,30.8213203435596)) ;
#84522=CARTESIAN_POINT('',(75.1999999999992,246.441753592594,30.8213203435596)) ;
#84523=CARTESIAN_POINT('Origin',(75.2999999999993,249.341421356237,30.8213203435596)) ;
#84524=CARTESIAN_POINT('',(75.2292893218807,249.270710678119,30.8213203435596)) ;
#84525=CARTESIAN_POINT('Origin',(75.158578643762,249.2,30.8213203435596)) ;
#84526=CARTESIAN_POINT('Origin',(75.2999999999993,249.341421356237,30.8213203435596)) ;
#84527=CARTESIAN_POINT('Origin',(72.4334125255833,251.925166118179,30.8213203435596)) ;
#84528=CARTESIAN_POINT('',(75.9707106781179,248.529289321881,30.8213203435596)) ;
#84529=CARTESIAN_POINT('Origin',(75.8999999999992,248.458578643763,30.8213203435596)) ;
#84530=CARTESIAN_POINT('',(72.504123203702,251.995876796297,30.8213203435596)) ;
#84531=CARTESIAN_POINT('Origin',(76.0414213562365,248.6,30.8213203435596)) ;
#84532=CARTESIAN_POINT('',(76.0414213562365,248.5,30.8213203435596)) ;
#84533=CARTESIAN_POINT('Origin',(76.0414213562365,248.4,30.8213203435596)) ;
#84534=CARTESIAN_POINT('Origin',(76.0414213562365,248.6,30.8213203435596)) ;
#84535=CARTESIAN_POINT('Origin',(64.4499999999996,248.4,30.8213203435596)) ;
#84536=CARTESIAN_POINT('',(64.4499999999996,248.5,30.8213203435596)) ;
#84537=CARTESIAN_POINT('Origin',(80.2999999999989,243.941753592594,30.8213203435596)) ;
#84538=CARTESIAN_POINT('',(80.199999999999,252.4,30.8213203435596)) ;
#84539=CARTESIAN_POINT('Origin',(80.299999999999,252.4,30.8213203435596)) ;
#84540=CARTESIAN_POINT('',(80.1999999999989,243.941753592594,30.8213203435596)) ;
#84541=CARTESIAN_POINT('Origin',(80.099999999999,253.4,19.9213203435596)) ;
#84542=CARTESIAN_POINT('',(80.199999999999,253.4,31.8213203435596)) ;
#84543=CARTESIAN_POINT('',(80.099999999999,253.5,31.8213203435596)) ;
#84544=CARTESIAN_POINT('Origin',(80.099999999999,253.4,31.8213203435596)) ;
#84545=CARTESIAN_POINT('',(80.099999999999,253.5,19.9213203435596)) ;
#84546=CARTESIAN_POINT('',(80.199999999999,253.4,19.9213203435596)) ;
#84547=CARTESIAN_POINT('Ctrl Pts',(80.099999999999,253.5,31.8213203435596)) ;
#84548=CARTESIAN_POINT('Ctrl Pts',(80.099999999999,253.5,31.8736802211195)) ;
#84549=CARTESIAN_POINT('Ctrl Pts',(80.1952802448793,253.54764012244,31.9213203435596)) ;
#84550=CARTESIAN_POINT('Ctrl Pts',(80.299999999999,253.6,31.9213203435596)) ;
#84551=CARTESIAN_POINT('Ctrl Pts',(80.1299199300332,253.5,31.8213203435596)) ;
#84552=CARTESIAN_POINT('Ctrl Pts',(80.1299199300331,253.5,31.8577789708945)) ;
#84553=CARTESIAN_POINT('Ctrl Pts',(80.2052535548907,253.537666812429,31.9213203435596)) ;
#84554=CARTESIAN_POINT('Ctrl Pts',(80.299999999999,253.6,31.9213203435596)) ;
#84555=CARTESIAN_POINT('Ctrl Pts',(80.1816963524867,253.474867379293,31.8213203435596)) ;
#84556=CARTESIAN_POINT('Ctrl Pts',(80.1816963524867,253.474867379293,31.8441177712024)) ;
#84557=CARTESIAN_POINT('Ctrl Pts',(80.2227068474107,253.520213519909,31.9213203435596)) ;
#84558=CARTESIAN_POINT('Ctrl Pts',(80.299999999999,253.6,31.9213203435596)) ;
#84559=CARTESIAN_POINT('Ctrl Pts',(80.199999999999,253.422439947526,31.8213203435596)) ;
#84560=CARTESIAN_POINT('Ctrl Pts',(80.199999999999,253.422439947526,31.8619121713415)) ;
#84561=CARTESIAN_POINT('Ctrl Pts',(80.2401601399306,253.502760227389,31.9213203435596)) ;
#84562=CARTESIAN_POINT('Ctrl Pts',(80.299999999999,253.6,31.9213203435596)) ;
#84563=CARTESIAN_POINT('Ctrl Pts',(80.199999999999,253.4,31.8213203435596)) ;
#84564=CARTESIAN_POINT('Ctrl Pts',(80.199999999999,253.4,31.8736802211195)) ;
#84565=CARTESIAN_POINT('Ctrl Pts',(80.2476401224392,253.49528024488,31.9213203435596)) ;
#84566=CARTESIAN_POINT('Ctrl Pts',(80.299999999999,253.6,31.9213203435596)) ;
#84567=CARTESIAN_POINT('Origin',(80.299999999999,253.6,31.8213203435596)) ;
#84568=CARTESIAN_POINT('Origin',(80.299999999999,253.6,31.8213203435596)) ;
#84569=CARTESIAN_POINT('Origin',(80.0999999999989,248.6,19.9213203435596)) ;
#84570=CARTESIAN_POINT('',(80.0999999999989,248.5,31.8213203435596)) ;
#84571=CARTESIAN_POINT('',(80.199999999999,248.6,31.8213203435596)) ;
#84572=CARTESIAN_POINT('Origin',(80.0999999999989,248.6,31.8213203435596)) ;
#84573=CARTESIAN_POINT('',(80.199999999999,248.6,19.9213203435596)) ;
#84574=CARTESIAN_POINT('',(80.0999999999989,248.5,19.9213203435596)) ;
#84575=CARTESIAN_POINT('Ctrl Pts',(80.299999999999,248.4,31.9213203435596)) ;
#84576=CARTESIAN_POINT('Ctrl Pts',(80.1952802448793,248.45235987756,31.9213203435597)) ;
#84577=CARTESIAN_POINT('Ctrl Pts',(80.0999999999989,248.5,31.8736802211194)) ;
#84578=CARTESIAN_POINT('Ctrl Pts',(80.0999999999989,248.5,31.8213203435596)) ;
#84579=CARTESIAN_POINT('Ctrl Pts',(80.299999999999,248.4,31.9213203435596)) ;
#84580=CARTESIAN_POINT('Ctrl Pts',(80.2052535548907,248.462333187571,31.9213203435597)) ;
#84581=CARTESIAN_POINT('Ctrl Pts',(80.1299199300331,248.5,31.8577789708944)) ;
#84582=CARTESIAN_POINT('Ctrl Pts',(80.1299199300331,248.5,31.8213203435596)) ;
#84583=CARTESIAN_POINT('Ctrl Pts',(80.299999999999,248.4,31.9213203435596)) ;
#84584=CARTESIAN_POINT('Ctrl Pts',(80.2227068474107,248.479786480091,31.9213203435597)) ;
#84585=CARTESIAN_POINT('Ctrl Pts',(80.1816963988781,248.525132582043,31.8441177712024)) ;
#84586=CARTESIAN_POINT('Ctrl Pts',(80.1816963988781,248.525132582043,31.8213203435596)) ;
#84587=CARTESIAN_POINT('Ctrl Pts',(80.299999999999,248.4,31.9213203435596)) ;
#84588=CARTESIAN_POINT('Ctrl Pts',(80.2401601399306,248.497239772611,31.9213203435597)) ;
#84589=CARTESIAN_POINT('Ctrl Pts',(80.1999999999989,248.577560052474,31.8619121713414)) ;
#84590=CARTESIAN_POINT('Ctrl Pts',(80.1999999999989,248.577560052474,31.8213203435596)) ;
#84591=CARTESIAN_POINT('Ctrl Pts',(80.299999999999,248.4,31.9213203435596)) ;
#84592=CARTESIAN_POINT('Ctrl Pts',(80.2476401224392,248.50471975512,31.9213203435597)) ;
#84593=CARTESIAN_POINT('Ctrl Pts',(80.1999999999989,248.6,31.8736802211195)) ;
#84594=CARTESIAN_POINT('Ctrl Pts',(80.1999999999989,248.6,31.8213203435596)) ;
#84595=CARTESIAN_POINT('Origin',(80.2999999999989,248.4,31.8213203435596)) ;
#84596=CARTESIAN_POINT('Origin',(80.2999999999989,248.4,31.8213203435596)) ;
#84597=CARTESIAN_POINT('Origin',(80.2999999999989,243.941753592594,30.8213203435596)) ;
#84598=CARTESIAN_POINT('',(80.199999999999,249.6,30.8213203435596)) ;
#84599=CARTESIAN_POINT('Origin',(80.2999999999989,249.6,30.8213203435596)) ;
#84600=CARTESIAN_POINT('',(80.1999999999989,243.941753592594,30.8213203435596)) ;
#84601=CARTESIAN_POINT('Origin',(80.199999999999,248.5,19.9213203435596)) ;
#84602=CARTESIAN_POINT('',(80.199999999999,252.4,31.8213203435596)) ;
#84603=CARTESIAN_POINT('',(80.199999999999,252.4,22.9213203435596)) ;
#84604=CARTESIAN_POINT('',(80.1999999999989,243.941753592594,31.8213203435596)) ;
#84605=CARTESIAN_POINT('Origin',(64.4999999999999,250.9,30.8213203435596)) ;
#84606=CARTESIAN_POINT('',(64.4999999999999,251.,30.8213203435596)) ;
#84607=CARTESIAN_POINT('Origin',(64.4999999999999,251.1,30.8213203435596)) ;
#84608=CARTESIAN_POINT('',(64.3999999999999,250.9,30.8213203435596)) ;
#84609=CARTESIAN_POINT('Origin',(64.4999999999999,250.9,30.8213203435596)) ;
#84610=CARTESIAN_POINT('Origin',(64.3,250.9,30.8213203435596)) ;
#84611=CARTESIAN_POINT('Origin',(59.2,251.1,30.8213203435596)) ;
#84612=CARTESIAN_POINT('',(64.6,251.,30.8213203435596)) ;
#84613=CARTESIAN_POINT('Origin',(64.6,251.1,30.8213203435596)) ;
#84614=CARTESIAN_POINT('',(59.2,251.,30.8213203435596)) ;
#84615=CARTESIAN_POINT('Origin',(64.6,248.191753592594,30.8213203435596)) ;
#84616=CARTESIAN_POINT('',(64.7,256.9,30.8213203435596)) ;
#84617=CARTESIAN_POINT('Origin',(64.6,256.9,30.8213203435596)) ;
#84618=CARTESIAN_POINT('',(64.7,251.1,30.8213203435596)) ;
#84619=CARTESIAN_POINT('',(64.7,248.191753592594,30.8213203435596)) ;
#84620=CARTESIAN_POINT('Origin',(64.6,251.1,30.8213203435596)) ;
#84621=CARTESIAN_POINT('Origin',(64.8,256.9,30.8213203435596)) ;
#84622=CARTESIAN_POINT('',(64.8,257.,30.8213203435596)) ;
#84623=CARTESIAN_POINT('Origin',(64.8,257.1,30.8213203435596)) ;
#84624=CARTESIAN_POINT('Origin',(64.8,256.9,30.8213203435596)) ;
#84625=CARTESIAN_POINT('Origin',(60.4,257.1,30.8213203435596)) ;
#84626=CARTESIAN_POINT('',(67.,257.,30.8213203435596)) ;
#84627=CARTESIAN_POINT('Origin',(67.,257.1,30.8213203435596)) ;
#84628=CARTESIAN_POINT('',(60.4,257.,30.8213203435596)) ;
#84629=CARTESIAN_POINT('Origin',(67.,256.9,30.8213203435596)) ;
#84630=CARTESIAN_POINT('',(67.1,256.9,30.8213203435596)) ;
#84631=CARTESIAN_POINT('Origin',(67.2,256.9,30.8213203435596)) ;
#84632=CARTESIAN_POINT('Origin',(67.,256.9,30.8213203435596)) ;
#84633=CARTESIAN_POINT('Origin',(67.2,245.191753592594,30.8213203435596)) ;
#84634=CARTESIAN_POINT('',(67.1,251.1,30.8213203435596)) ;
#84635=CARTESIAN_POINT('Origin',(67.2,251.1,30.8213203435596)) ;
#84636=CARTESIAN_POINT('',(67.1,245.191753592594,30.8213203435596)) ;
#84637=CARTESIAN_POINT('Origin',(64.6,251.1,30.8213203435596)) ;
#84638=CARTESIAN_POINT('Origin',(64.6,251.1,30.8213203435596)) ;
#84639=CARTESIAN_POINT('Origin',(60.55,251.1,30.8213203435596)) ;
#84640=CARTESIAN_POINT('',(67.3,251.,30.8213203435596)) ;
#84641=CARTESIAN_POINT('Origin',(67.3,251.1,30.8213203435596)) ;
#84642=CARTESIAN_POINT('',(67.2,251.,30.8213203435596)) ;
#84643=CARTESIAN_POINT('',(60.55,251.,30.8213203435596)) ;
#84644=CARTESIAN_POINT('Origin',(67.2,251.1,30.8213203435596)) ;
#84645=CARTESIAN_POINT('Origin',(67.3,250.9,30.8213203435596)) ;
#84646=CARTESIAN_POINT('',(67.4,250.9,30.8213203435596)) ;
#84647=CARTESIAN_POINT('Origin',(67.5,250.9,30.8213203435596)) ;
#84648=CARTESIAN_POINT('Origin',(67.3,250.9,30.8213203435596)) ;
#84649=CARTESIAN_POINT('Origin',(67.2,251.1,30.8213203435596)) ;
#84650=CARTESIAN_POINT('Origin',(67.2,251.1,30.8213203435596)) ;
#84651=CARTESIAN_POINT('Origin',(64.7,251.,19.9213203435596)) ;
#84652=CARTESIAN_POINT('',(64.6,251.,31.8213203435596)) ;
#84653=CARTESIAN_POINT('',(64.6,251.,19.9213203435596)) ;
#84654=CARTESIAN_POINT('',(64.5,251.,31.8213203435596)) ;
#84655=CARTESIAN_POINT('',(59.2,251.,31.8213203435596)) ;
#84656=CARTESIAN_POINT('',(64.5,251.,19.9213203435596)) ;
#84657=CARTESIAN_POINT('Origin',(64.6,251.1,19.9213203435596)) ;
#84658=CARTESIAN_POINT('',(64.7,251.1,31.8213203435596)) ;
#84659=CARTESIAN_POINT('',(64.7,251.1,19.9213203435596)) ;
#84660=CARTESIAN_POINT('Origin',(64.6,251.1,31.8213203435596)) ;
#84661=CARTESIAN_POINT('Origin',(64.7,257.,19.9213203435596)) ;
#84662=CARTESIAN_POINT('',(64.7,256.9,31.8213203435596)) ;
#84663=CARTESIAN_POINT('',(64.7,256.9,19.9213203435596)) ;
#84664=CARTESIAN_POINT('',(64.7,248.191753592594,31.8213203435596)) ;
#84665=CARTESIAN_POINT('Origin',(64.8,256.9,19.9213203435596)) ;
#84666=CARTESIAN_POINT('',(64.8,257.,31.8213203435596)) ;
#84667=CARTESIAN_POINT('',(64.8,257.,19.9213203435596)) ;
#84668=CARTESIAN_POINT('Origin',(64.8,256.9,31.8213203435596)) ;
#84669=CARTESIAN_POINT('Origin',(67.1,257.,19.9213203435596)) ;
#84670=CARTESIAN_POINT('',(67.,257.,31.8213203435596)) ;
#84671=CARTESIAN_POINT('',(67.,257.,19.9213203435596)) ;
#84672=CARTESIAN_POINT('',(60.4,257.,31.8213203435596)) ;
#84673=CARTESIAN_POINT('Origin',(67.,256.9,19.9213203435596)) ;
#84674=CARTESIAN_POINT('',(67.1,256.9,31.8213203435596)) ;
#84675=CARTESIAN_POINT('',(67.1,256.9,19.9213203435596)) ;
#84676=CARTESIAN_POINT('Origin',(67.,256.9,31.8213203435596)) ;
#84677=CARTESIAN_POINT('Origin',(67.1,251.,19.9213203435596)) ;
#84678=CARTESIAN_POINT('',(67.1,251.1,31.8213203435596)) ;
#84679=CARTESIAN_POINT('',(67.1,251.1,19.9213203435596)) ;
#84680=CARTESIAN_POINT('',(67.1,245.191753592594,31.8213203435596)) ;
#84681=CARTESIAN_POINT('Origin',(67.2,251.1,19.9213203435596)) ;
#84682=CARTESIAN_POINT('',(67.2,251.,31.8213203435596)) ;
#84683=CARTESIAN_POINT('',(67.2,251.,19.9213203435596)) ;
#84684=CARTESIAN_POINT('Origin',(67.2,251.1,31.8213203435596)) ;
#84685=CARTESIAN_POINT('Origin',(67.4,251.,19.9213203435596)) ;
#84686=CARTESIAN_POINT('',(67.3,251.,31.8213203435596)) ;
#84687=CARTESIAN_POINT('',(67.3,251.,19.9213203435596)) ;
#84688=CARTESIAN_POINT('',(60.55,251.,31.8213203435596)) ;
#84689=CARTESIAN_POINT('Origin',(56.5,250.9,30.8213203435596)) ;
#84690=CARTESIAN_POINT('',(56.5,251.,30.8213203435596)) ;
#84691=CARTESIAN_POINT('Origin',(56.5,251.1,30.8213203435596)) ;
#84692=CARTESIAN_POINT('',(56.3999999999999,250.9,30.8213203435596)) ;
#84693=CARTESIAN_POINT('Origin',(56.5,250.9,30.8213203435596)) ;
#84694=CARTESIAN_POINT('Origin',(56.3,250.9,30.8213203435596)) ;
#84695=CARTESIAN_POINT('Origin',(55.2,251.1,30.8213203435596)) ;
#84696=CARTESIAN_POINT('',(56.6,251.,30.8213203435596)) ;
#84697=CARTESIAN_POINT('Origin',(56.6,251.1,30.8213203435596)) ;
#84698=CARTESIAN_POINT('',(55.2,251.,30.8213203435596)) ;
#84699=CARTESIAN_POINT('Origin',(56.6,248.191753592594,30.8213203435596)) ;
#84700=CARTESIAN_POINT('',(56.7,256.9,30.8213203435596)) ;
#84701=CARTESIAN_POINT('Origin',(56.6,256.9,30.8213203435596)) ;
#84702=CARTESIAN_POINT('',(56.7,251.1,30.8213203435596)) ;
#84703=CARTESIAN_POINT('',(56.7,248.191753592594,30.8213203435596)) ;
#84704=CARTESIAN_POINT('Origin',(56.6,251.1,30.8213203435596)) ;
#84705=CARTESIAN_POINT('Origin',(56.8,256.9,30.8213203435596)) ;
#84706=CARTESIAN_POINT('',(56.8,257.,30.8213203435596)) ;
#84707=CARTESIAN_POINT('Origin',(56.8,257.1,30.8213203435596)) ;
#84708=CARTESIAN_POINT('Origin',(56.8,256.9,30.8213203435596)) ;
#84709=CARTESIAN_POINT('Origin',(56.4,257.1,30.8213203435596)) ;
#84710=CARTESIAN_POINT('',(59.,257.,30.8213203435596)) ;
#84711=CARTESIAN_POINT('Origin',(59.,257.1,30.8213203435596)) ;
#84712=CARTESIAN_POINT('',(56.4,257.,30.8213203435596)) ;
#84713=CARTESIAN_POINT('Origin',(59.,256.9,30.8213203435596)) ;
#84714=CARTESIAN_POINT('',(59.1,256.9,30.8213203435596)) ;
#84715=CARTESIAN_POINT('Origin',(59.2,256.9,30.8213203435596)) ;
#84716=CARTESIAN_POINT('Origin',(59.,256.9,30.8213203435596)) ;
#84717=CARTESIAN_POINT('Origin',(59.2,245.191753592594,30.8213203435596)) ;
#84718=CARTESIAN_POINT('',(59.1,251.1,30.8213203435596)) ;
#84719=CARTESIAN_POINT('Origin',(59.2,251.1,30.8213203435596)) ;
#84720=CARTESIAN_POINT('',(59.1,245.191753592594,30.8213203435596)) ;
#84721=CARTESIAN_POINT('Origin',(56.6,251.1,30.8213203435596)) ;
#84722=CARTESIAN_POINT('Origin',(56.6,251.1,30.8213203435596)) ;
#84723=CARTESIAN_POINT('Origin',(56.55,251.1,30.8213203435596)) ;
#84724=CARTESIAN_POINT('',(59.3,251.,30.8213203435596)) ;
#84725=CARTESIAN_POINT('Origin',(59.3,251.1,30.8213203435596)) ;
#84726=CARTESIAN_POINT('',(59.2,251.,30.8213203435596)) ;
#84727=CARTESIAN_POINT('',(56.55,251.,30.8213203435596)) ;
#84728=CARTESIAN_POINT('Origin',(59.2,251.1,30.8213203435596)) ;
#84729=CARTESIAN_POINT('Origin',(59.3,250.9,30.8213203435596)) ;
#84730=CARTESIAN_POINT('',(59.4,250.9,30.8213203435596)) ;
#84731=CARTESIAN_POINT('Origin',(59.5,250.9,30.8213203435596)) ;
#84732=CARTESIAN_POINT('Origin',(59.3,250.9,30.8213203435596)) ;
#84733=CARTESIAN_POINT('Origin',(59.2,251.1,30.8213203435596)) ;
#84734=CARTESIAN_POINT('Origin',(59.2,251.1,30.8213203435596)) ;
#84735=CARTESIAN_POINT('Origin',(56.7,251.,19.9213203435596)) ;
#84736=CARTESIAN_POINT('',(56.6,251.,31.8213203435596)) ;
#84737=CARTESIAN_POINT('',(56.6,251.,19.9213203435596)) ;
#84738=CARTESIAN_POINT('',(56.5,251.,31.8213203435596)) ;
#84739=CARTESIAN_POINT('',(55.2,251.,31.8213203435596)) ;
#84740=CARTESIAN_POINT('',(56.5,251.,19.9213203435596)) ;
#84741=CARTESIAN_POINT('Origin',(56.6,251.1,19.9213203435596)) ;
#84742=CARTESIAN_POINT('',(56.7,251.1,31.8213203435596)) ;
#84743=CARTESIAN_POINT('',(56.7,251.1,19.9213203435596)) ;
#84744=CARTESIAN_POINT('Origin',(56.6,251.1,31.8213203435596)) ;
#84745=CARTESIAN_POINT('Origin',(56.7,257.,19.9213203435596)) ;
#84746=CARTESIAN_POINT('',(56.7,256.9,31.8213203435596)) ;
#84747=CARTESIAN_POINT('',(56.7,256.9,19.9213203435596)) ;
#84748=CARTESIAN_POINT('',(56.7,248.191753592594,31.8213203435596)) ;
#84749=CARTESIAN_POINT('Origin',(56.8,256.9,19.9213203435596)) ;
#84750=CARTESIAN_POINT('',(56.8,257.,31.8213203435596)) ;
#84751=CARTESIAN_POINT('',(56.8,257.,19.9213203435596)) ;
#84752=CARTESIAN_POINT('Origin',(56.8,256.9,31.8213203435596)) ;
#84753=CARTESIAN_POINT('Origin',(59.1,257.,19.9213203435596)) ;
#84754=CARTESIAN_POINT('',(59.,257.,31.8213203435596)) ;
#84755=CARTESIAN_POINT('',(59.,257.,19.9213203435596)) ;
#84756=CARTESIAN_POINT('',(56.4,257.,31.8213203435596)) ;
#84757=CARTESIAN_POINT('Origin',(59.,256.9,19.9213203435596)) ;
#84758=CARTESIAN_POINT('',(59.1,256.9,31.8213203435596)) ;
#84759=CARTESIAN_POINT('',(59.1,256.9,19.9213203435596)) ;
#84760=CARTESIAN_POINT('Origin',(59.,256.9,31.8213203435596)) ;
#84761=CARTESIAN_POINT('Origin',(59.1,251.,19.9213203435596)) ;
#84762=CARTESIAN_POINT('',(59.1,251.1,31.8213203435596)) ;
#84763=CARTESIAN_POINT('',(59.1,251.1,19.9213203435596)) ;
#84764=CARTESIAN_POINT('',(59.1,245.191753592594,31.8213203435596)) ;
#84765=CARTESIAN_POINT('Origin',(59.2,251.1,19.9213203435596)) ;
#84766=CARTESIAN_POINT('',(59.2,251.,31.8213203435596)) ;
#84767=CARTESIAN_POINT('',(59.2,251.,19.9213203435596)) ;
#84768=CARTESIAN_POINT('Origin',(59.2,251.1,31.8213203435596)) ;
#84769=CARTESIAN_POINT('Origin',(59.4,251.,19.9213203435596)) ;
#84770=CARTESIAN_POINT('',(59.3,251.,31.8213203435596)) ;
#84771=CARTESIAN_POINT('',(59.3,251.,19.9213203435596)) ;
#84772=CARTESIAN_POINT('',(56.55,251.,31.8213203435596)) ;
#84773=CARTESIAN_POINT('Origin',(62.4573593128808,234.691753592594,30.8213203435596)) ;
#84774=CARTESIAN_POINT('Origin',(62.4573593128808,230.1,30.8213203435596)) ;
#84775=CARTESIAN_POINT('Origin',(58.1786796564404,230.1,30.8213203435596)) ;
#84776=CARTESIAN_POINT('',(62.5573593128808,230.,30.8213203435596)) ;
#84777=CARTESIAN_POINT('Origin',(62.5573593128808,230.1,30.8213203435596)) ;
#84778=CARTESIAN_POINT('',(58.1786796564404,230.,30.8213203435596)) ;
#84779=CARTESIAN_POINT('Origin',(62.4573593128808,230.1,30.8213203435596)) ;
#84780=CARTESIAN_POINT('Origin',(62.5573593128808,229.9,30.8213203435596)) ;
#84781=CARTESIAN_POINT('',(62.6573593128808,229.9,30.8213203435596)) ;
#84782=CARTESIAN_POINT('Origin',(62.7573593128808,229.9,30.8213203435596)) ;
#84783=CARTESIAN_POINT('Origin',(62.5573593128808,229.9,30.8213203435596)) ;
#84784=CARTESIAN_POINT('Origin',(62.4573593128808,230.1,30.8213203435596)) ;
#84785=CARTESIAN_POINT('Origin',(62.6573593128808,230.,19.9213203435596)) ;
#84786=CARTESIAN_POINT('',(62.5573593128808,230.,19.9213203435596)) ;
#84787=CARTESIAN_POINT('Origin',(59.8573593128808,237.691753592594,30.8213203435596)) ;
#84788=CARTESIAN_POINT('',(59.9573593128808,237.691753592594,30.8213203435596)) ;
#84789=CARTESIAN_POINT('Origin',(59.7573593128808,229.9,30.8213203435596)) ;
#84790=CARTESIAN_POINT('',(59.6573593128808,229.9,30.8213203435596)) ;
#84791=CARTESIAN_POINT('Origin',(59.7573593128808,229.9,30.8213203435596)) ;
#84792=CARTESIAN_POINT('Origin',(59.5573593128808,229.9,30.8213203435596)) ;
#84793=CARTESIAN_POINT('Origin',(59.9573593128808,236.,19.9213203435596)) ;
#84794=CARTESIAN_POINT('Origin',(55.8286796564404,237.9,30.8213203435596)) ;
#84795=CARTESIAN_POINT('',(62.1159379566435,238.,30.8213203435596)) ;
#84796=CARTESIAN_POINT('',(55.8286796564404,238.,30.8213203435596)) ;
#84797=CARTESIAN_POINT('Origin',(62.1159379566435,237.9,30.8213203435596)) ;
#84798=CARTESIAN_POINT('Origin',(62.1159379566435,238.1,30.8213203435596)) ;
#84799=CARTESIAN_POINT('',(62.1866486347621,238.029289321881,30.8213203435596)) ;
#84800=CARTESIAN_POINT('Origin',(62.2573593128808,237.958578643763,30.8213203435596)) ;
#84801=CARTESIAN_POINT('Origin',(62.1159379566435,238.1,30.8213203435596)) ;
#84802=CARTESIAN_POINT('Origin',(60.6596069590762,236.360826289958,30.8213203435596)) ;
#84803=CARTESIAN_POINT('',(62.9280699909994,238.770710678119,30.8213203435596)) ;
#84804=CARTESIAN_POINT('Origin',(62.998780669118,238.7,30.8213203435596)) ;
#84805=CARTESIAN_POINT('',(60.5888962809576,236.431536968077,30.8213203435596)) ;
#84806=CARTESIAN_POINT('Origin',(62.8573593128807,238.841421356237,30.8213203435596)) ;
#84807=CARTESIAN_POINT('',(62.9573593128807,238.841421356237,30.8213203435596)) ;
#84808=CARTESIAN_POINT('Origin',(63.0573593128808,238.841421356237,30.8213203435596)) ;
#84809=CARTESIAN_POINT('Origin',(62.8573593128807,238.841421356237,30.8213203435596)) ;
#84810=CARTESIAN_POINT('Origin',(63.0573593128807,238.691753592594,30.8213203435596)) ;
#84811=CARTESIAN_POINT('',(62.9573593128807,242.158578643763,30.8213203435596)) ;
#84812=CARTESIAN_POINT('Origin',(63.0573593128807,242.158578643763,30.8213203435596)) ;
#84813=CARTESIAN_POINT('',(62.9573593128807,238.691753592594,30.8213203435596)) ;
#84814=CARTESIAN_POINT('Origin',(62.8573593128807,242.158578643763,30.8213203435596)) ;
#84815=CARTESIAN_POINT('',(62.9280699909994,242.229289321881,30.8213203435596)) ;
#84816=CARTESIAN_POINT('Origin',(62.9987806691181,242.3,30.8213203435596)) ;
#84817=CARTESIAN_POINT('Origin',(62.8573593128807,242.158578643763,30.8213203435596)) ;
#84818=CARTESIAN_POINT('Origin',(61.2178533664821,244.080927302636,30.8213203435596)) ;
#84819=CARTESIAN_POINT('',(62.1866486347621,242.970710678119,30.8213203435596)) ;
#84820=CARTESIAN_POINT('Origin',(62.2573593128808,243.041421356237,30.8213203435596)) ;
#84821=CARTESIAN_POINT('',(61.1471426883634,244.010216624517,30.8213203435596)) ;
#84822=CARTESIAN_POINT('Origin',(62.1159379566435,242.9,30.8213203435596)) ;
#84823=CARTESIAN_POINT('',(62.1159379566435,243.,30.8213203435596)) ;
#84824=CARTESIAN_POINT('Origin',(62.1159379566435,243.1,30.8213203435596)) ;
#84825=CARTESIAN_POINT('Origin',(62.1159379566435,242.9,30.8213203435596)) ;
#84826=CARTESIAN_POINT('Origin',(58.3286796564404,243.1,30.8213203435596)) ;
#84827=CARTESIAN_POINT('',(58.3286796564404,243.,30.8213203435596)) ;
#84828=CARTESIAN_POINT('Origin',(62.9573593128807,243.,19.9213203435596)) ;
#84829=CARTESIAN_POINT('',(62.1159379566435,243.,31.8213203435596)) ;
#84830=CARTESIAN_POINT('',(62.1159379566435,243.,19.9213203435596)) ;
#84831=CARTESIAN_POINT('',(58.3286796564404,243.,31.8213203435596)) ;
#84832=CARTESIAN_POINT('Origin',(62.1159379566435,242.9,19.9213203435596)) ;
#84833=CARTESIAN_POINT('',(62.1866486347621,242.970710678119,31.8213203435596)) ;
#84834=CARTESIAN_POINT('',(62.1866486347621,242.970710678119,19.9213203435596)) ;
#84835=CARTESIAN_POINT('Origin',(62.1159379566435,242.9,31.8213203435596)) ;
#84836=CARTESIAN_POINT('Origin',(62.5573593128807,242.6,19.9213203435596)) ;
#84837=CARTESIAN_POINT('',(62.9280699909994,242.229289321881,31.8213203435596)) ;
#84838=CARTESIAN_POINT('',(62.9280699909994,242.229289321881,19.9213203435596)) ;
#84839=CARTESIAN_POINT('',(61.1471426883634,244.010216624517,31.8213203435596)) ;
#84840=CARTESIAN_POINT('Origin',(62.8573593128807,242.158578643763,19.9213203435596)) ;
#84841=CARTESIAN_POINT('',(62.9573593128807,242.158578643763,31.8213203435596)) ;
#84842=CARTESIAN_POINT('',(62.9573593128807,242.158578643763,19.9213203435596)) ;
#84843=CARTESIAN_POINT('Origin',(62.8573593128807,242.158578643763,31.8213203435596)) ;
#84844=CARTESIAN_POINT('Origin',(62.9573593128807,238.,19.9213203435596)) ;
#84845=CARTESIAN_POINT('',(62.9573593128807,238.841421356237,31.8213203435596)) ;
#84846=CARTESIAN_POINT('',(62.9573593128807,238.841421356237,19.9213203435596)) ;
#84847=CARTESIAN_POINT('',(62.9573593128807,238.691753592594,31.8213203435596)) ;
#84848=CARTESIAN_POINT('Origin',(62.8573593128807,238.841421356237,19.9213203435596)) ;
#84849=CARTESIAN_POINT('',(62.9280699909994,238.770710678119,31.8213203435596)) ;
#84850=CARTESIAN_POINT('',(62.9280699909994,238.770710678119,19.9213203435596)) ;
#84851=CARTESIAN_POINT('Origin',(62.8573593128807,238.841421356237,31.8213203435596)) ;
#84852=CARTESIAN_POINT('Origin',(62.5573593128807,238.4,19.9213203435596)) ;
#84853=CARTESIAN_POINT('',(62.1866486347621,238.029289321881,31.8213203435596)) ;
#84854=CARTESIAN_POINT('',(62.1866486347621,238.029289321881,19.9213203435596)) ;
#84855=CARTESIAN_POINT('',(60.5888962809576,236.431536968077,31.8213203435596)) ;
#84856=CARTESIAN_POINT('Origin',(62.1159379566435,238.1,19.9213203435596)) ;
#84857=CARTESIAN_POINT('',(62.1159379566435,238.,31.8213203435596)) ;
#84858=CARTESIAN_POINT('',(62.1159379566435,238.,19.9213203435596)) ;
#84859=CARTESIAN_POINT('Origin',(62.1159379566435,238.1,31.8213203435596)) ;
#84860=CARTESIAN_POINT('Origin',(57.9573593128808,238.,19.9213203435596)) ;
#84861=CARTESIAN_POINT('',(55.8286796564404,238.,31.8213203435596)) ;
#84862=CARTESIAN_POINT('Origin',(59.7573593128808,229.9,19.9213203435596)) ;
#84863=CARTESIAN_POINT('',(59.6573593128808,229.9,19.9213203435596)) ;
#84864=CARTESIAN_POINT('Origin',(62.5573593128808,227.1,30.8213203435596)) ;
#84865=CARTESIAN_POINT('',(62.5573593128808,227.,30.8213203435596)) ;
#84866=CARTESIAN_POINT('Origin',(62.5573593128808,226.9,30.8213203435596)) ;
#84867=CARTESIAN_POINT('',(62.6573593128808,227.1,30.8213203435596)) ;
#84868=CARTESIAN_POINT('Origin',(62.5573593128808,227.1,30.8213203435596)) ;
#84869=CARTESIAN_POINT('Origin',(62.7573593128808,227.1,30.8213203435596)) ;
#84870=CARTESIAN_POINT('Origin',(59.6573593128808,227.,19.9213203435596)) ;
#84871=CARTESIAN_POINT('',(59.7573593128808,227.,30.8213203435596)) ;
#84872=CARTESIAN_POINT('',(56.6786796564404,227.,30.8213203435596)) ;
#84873=CARTESIAN_POINT('',(59.7573593128808,227.,31.8213203435596)) ;
#84874=CARTESIAN_POINT('',(59.7573593128808,227.,19.9213203435596)) ;
#84875=CARTESIAN_POINT('',(62.5573593128808,227.,31.8213203435596)) ;
#84876=CARTESIAN_POINT('',(56.6786796564404,227.,31.8213203435596)) ;
#84877=CARTESIAN_POINT('',(62.5573593128808,227.,19.9213203435596)) ;
#84878=CARTESIAN_POINT('Origin',(62.5573593128808,229.9,31.8213203435596)) ;
#84879=CARTESIAN_POINT('',(62.6573593128808,229.9,31.8213203435596)) ;
#84880=CARTESIAN_POINT('Origin',(62.5573593128808,229.9,31.8213203435596)) ;
#84881=CARTESIAN_POINT('Origin',(62.7573593128808,229.9,31.8213203435596)) ;
#84882=CARTESIAN_POINT('Origin',(62.5573593128808,229.9,19.9213203435596)) ;
#84883=CARTESIAN_POINT('',(62.6573593128808,229.9,19.9213203435596)) ;
#84884=CARTESIAN_POINT('Origin',(59.7573593128808,227.1,31.8213203435596)) ;
#84885=CARTESIAN_POINT('Origin',(59.7573593128808,226.9,31.8213203435596)) ;
#84886=CARTESIAN_POINT('',(59.6573593128808,227.1,31.8213203435596)) ;
#84887=CARTESIAN_POINT('Origin',(59.7573593128808,227.1,31.8213203435596)) ;
#84888=CARTESIAN_POINT('Origin',(59.5573593128808,227.1,31.8213203435596)) ;
#84889=CARTESIAN_POINT('Origin',(62.5573593128808,227.1,31.8213203435596)) ;
#84890=CARTESIAN_POINT('',(62.6573593128808,227.1,31.8213203435596)) ;
#84891=CARTESIAN_POINT('Origin',(62.7573593128808,227.1,31.8213203435596)) ;
#84892=CARTESIAN_POINT('Origin',(62.5573593128808,227.1,31.8213203435596)) ;
#84893=CARTESIAN_POINT('Origin',(62.5573593128808,226.9,31.8213203435596)) ;
#84894=CARTESIAN_POINT('Origin',(62.7573593128808,233.191753592594,31.8213203435596)) ;
#84895=CARTESIAN_POINT('',(62.6573593128808,233.191753592594,31.8213203435596)) ;
#84896=CARTESIAN_POINT('Origin',(62.5573593128808,227.1,19.9213203435596)) ;
#84897=CARTESIAN_POINT('',(62.6573593128808,227.1,19.9213203435596)) ;
#84898=CARTESIAN_POINT('Origin',(56.6786796564404,226.9,31.8213203435596)) ;
#84899=CARTESIAN_POINT('Origin',(59.7573593128808,227.1,30.8213203435596)) ;
#84900=CARTESIAN_POINT('',(59.6573593128808,227.1,30.8213203435596)) ;
#84901=CARTESIAN_POINT('Origin',(59.7573593128808,227.1,30.8213203435596)) ;
#84902=CARTESIAN_POINT('Origin',(59.7573593128808,226.9,30.8213203435596)) ;
#84903=CARTESIAN_POINT('Origin',(59.5573593128808,227.1,30.8213203435596)) ;
#84904=CARTESIAN_POINT('Origin',(56.6786796564404,226.9,30.8213203435596)) ;
#84905=CARTESIAN_POINT('Origin',(59.5573593128808,234.691753592594,30.8213203435596)) ;
#84906=CARTESIAN_POINT('',(59.6573593128808,234.691753592594,30.8213203435596)) ;
#84907=CARTESIAN_POINT('Origin',(59.7573593128808,227.1,19.9213203435596)) ;
#84908=CARTESIAN_POINT('',(59.6573593128808,227.1,19.9213203435596)) ;
#84909=CARTESIAN_POINT('Origin',(59.5573593128808,234.691753592594,31.8213203435596)) ;
#84910=CARTESIAN_POINT('',(59.6573593128808,234.691753592594,31.8213203435596)) ;
#84911=CARTESIAN_POINT('Origin',(62.6573593128808,227.,19.9213203435596)) ;
#84912=CARTESIAN_POINT('',(62.6573593128808,233.191753592594,30.8213203435596)) ;
#84913=CARTESIAN_POINT('Origin',(62.7573593128808,233.191753592594,30.8213203435596)) ;
#84914=CARTESIAN_POINT('Origin',(64.4999999999999,248.1,30.8213203435596)) ;
#84915=CARTESIAN_POINT('',(64.4999999999999,248.,30.8213203435596)) ;
#84916=CARTESIAN_POINT('Origin',(64.4999999999999,247.9,30.8213203435596)) ;
#84917=CARTESIAN_POINT('',(64.3999999999999,248.1,30.8213203435596)) ;
#84918=CARTESIAN_POINT('Origin',(64.3,248.1,30.8213203435596)) ;
#84919=CARTESIAN_POINT('Origin',(64.4999999999999,248.1,30.8213203435596)) ;
#84920=CARTESIAN_POINT('Origin',(67.3,248.1,30.8213203435596)) ;
#84921=CARTESIAN_POINT('',(67.3,248.,30.8213203435596)) ;
#84922=CARTESIAN_POINT('Origin',(67.3,247.9,30.8213203435596)) ;
#84923=CARTESIAN_POINT('',(67.4,248.1,30.8213203435596)) ;
#84924=CARTESIAN_POINT('Origin',(67.3,248.1,30.8213203435596)) ;
#84925=CARTESIAN_POINT('Origin',(67.5,248.1,30.8213203435596)) ;
#84926=CARTESIAN_POINT('Origin',(64.3999999999999,248.,19.9213203435596)) ;
#84927=CARTESIAN_POINT('',(59.05,248.,30.8213203435596)) ;
#84928=CARTESIAN_POINT('',(64.4999999999999,248.,31.8213203435596)) ;
#84929=CARTESIAN_POINT('',(64.4999999999999,248.,19.9213203435596)) ;
#84930=CARTESIAN_POINT('',(67.3,248.,31.8213203435596)) ;
#84931=CARTESIAN_POINT('',(59.05,248.,31.8213203435596)) ;
#84932=CARTESIAN_POINT('',(67.3,248.,19.9213203435596)) ;
#84933=CARTESIAN_POINT('Origin',(64.8,256.9,31.8213203435596)) ;
#84934=CARTESIAN_POINT('Origin',(64.8,257.1,31.8213203435596)) ;
#84935=CARTESIAN_POINT('Origin',(64.6,256.9,31.8213203435596)) ;
#84936=CARTESIAN_POINT('Origin',(67.,256.9,31.8213203435596)) ;
#84937=CARTESIAN_POINT('Origin',(67.,257.1,31.8213203435596)) ;
#84938=CARTESIAN_POINT('Origin',(67.2,256.9,31.8213203435596)) ;
#84939=CARTESIAN_POINT('Origin',(60.4,257.1,31.8213203435596)) ;
#84940=CARTESIAN_POINT('Origin',(64.6,251.1,31.8213203435596)) ;
#84941=CARTESIAN_POINT('Origin',(64.6,251.1,31.8213203435596)) ;
#84942=CARTESIAN_POINT('Origin',(64.6,251.1,31.8213203435596)) ;
#84943=CARTESIAN_POINT('Origin',(67.2,251.1,31.8213203435596)) ;
#84944=CARTESIAN_POINT('Origin',(67.2,251.1,31.8213203435596)) ;
#84945=CARTESIAN_POINT('Origin',(67.2,251.1,31.8213203435596)) ;
#84946=CARTESIAN_POINT('Origin',(67.2,245.191753592594,31.8213203435596)) ;
#84947=CARTESIAN_POINT('Origin',(64.5,250.9,31.8213203435596)) ;
#84948=CARTESIAN_POINT('',(64.3999999999999,250.9,31.8213203435596)) ;
#84949=CARTESIAN_POINT('Origin',(64.3,250.9,31.8213203435596)) ;
#84950=CARTESIAN_POINT('Origin',(64.5,250.9,31.8213203435596)) ;
#84951=CARTESIAN_POINT('Origin',(64.5,251.1,31.8213203435596)) ;
#84952=CARTESIAN_POINT('Origin',(67.3,250.9,31.8213203435596)) ;
#84953=CARTESIAN_POINT('Origin',(67.3,251.1,31.8213203435596)) ;
#84954=CARTESIAN_POINT('',(67.4,250.9,31.8213203435596)) ;
#84955=CARTESIAN_POINT('Origin',(67.3,250.9,31.8213203435596)) ;
#84956=CARTESIAN_POINT('Origin',(67.5,250.9,31.8213203435596)) ;
#84957=CARTESIAN_POINT('Origin',(60.55,251.1,31.8213203435596)) ;
#84958=CARTESIAN_POINT('Origin',(67.3,250.9,19.9213203435596)) ;
#84959=CARTESIAN_POINT('',(67.4,250.9,19.9213203435596)) ;
#84960=CARTESIAN_POINT('Origin',(64.4999999999999,248.1,31.8213203435596)) ;
#84961=CARTESIAN_POINT('Origin',(64.4999999999999,247.9,31.8213203435596)) ;
#84962=CARTESIAN_POINT('',(64.3999999999999,248.1,31.8213203435596)) ;
#84963=CARTESIAN_POINT('Origin',(64.4999999999999,248.1,31.8213203435596)) ;
#84964=CARTESIAN_POINT('Origin',(64.3,248.1,31.8213203435596)) ;
#84965=CARTESIAN_POINT('Origin',(67.3,248.1,31.8213203435596)) ;
#84966=CARTESIAN_POINT('',(67.4,248.1,31.8213203435596)) ;
#84967=CARTESIAN_POINT('Origin',(67.5,248.1,31.8213203435596)) ;
#84968=CARTESIAN_POINT('Origin',(67.3,248.1,31.8213203435596)) ;
#84969=CARTESIAN_POINT('Origin',(67.3,247.9,31.8213203435596)) ;
#84970=CARTESIAN_POINT('Origin',(67.5,243.691753592594,31.8213203435596)) ;
#84971=CARTESIAN_POINT('',(67.4,243.691753592594,31.8213203435596)) ;
#84972=CARTESIAN_POINT('Origin',(67.3,248.1,19.9213203435596)) ;
#84973=CARTESIAN_POINT('',(67.4,248.1,19.9213203435596)) ;
#84974=CARTESIAN_POINT('Origin',(59.05,247.9,31.8213203435596)) ;
#84975=CARTESIAN_POINT('Origin',(64.4999999999999,248.1,19.9213203435596)) ;
#84976=CARTESIAN_POINT('',(64.3999999999999,248.1,19.9213203435596)) ;
#84977=CARTESIAN_POINT('Origin',(64.3,245.191753592594,31.8213203435596)) ;
#84978=CARTESIAN_POINT('',(64.3999999999999,245.191753592594,31.8213203435596)) ;
#84979=CARTESIAN_POINT('Origin',(64.5,250.9,19.9213203435596)) ;
#84980=CARTESIAN_POINT('',(64.3999999999999,250.9,19.9213203435596)) ;
#84981=CARTESIAN_POINT('Origin',(59.2,251.1,31.8213203435596)) ;
#84982=CARTESIAN_POINT('Origin',(64.6,248.191753592594,31.8213203435596)) ;
#84983=CARTESIAN_POINT('Origin',(59.05,247.9,30.8213203435596)) ;
#84984=CARTESIAN_POINT('Origin',(67.4,248.,19.9213203435596)) ;
#84985=CARTESIAN_POINT('',(67.4,243.691753592594,30.8213203435596)) ;
#84986=CARTESIAN_POINT('Origin',(67.5,243.691753592594,30.8213203435596)) ;
#84987=CARTESIAN_POINT('Origin',(56.5,248.1,30.8213203435596)) ;
#84988=CARTESIAN_POINT('',(56.5,248.,30.8213203435596)) ;
#84989=CARTESIAN_POINT('Origin',(56.5,247.9,30.8213203435596)) ;
#84990=CARTESIAN_POINT('',(56.3999999999999,248.1,30.8213203435596)) ;
#84991=CARTESIAN_POINT('Origin',(56.3,248.1,30.8213203435596)) ;
#84992=CARTESIAN_POINT('Origin',(56.5,248.1,30.8213203435596)) ;
#84993=CARTESIAN_POINT('Origin',(59.3,248.1,30.8213203435596)) ;
#84994=CARTESIAN_POINT('',(59.3,248.,30.8213203435596)) ;
#84995=CARTESIAN_POINT('Origin',(59.3,247.9,30.8213203435596)) ;
#84996=CARTESIAN_POINT('',(59.4,248.1,30.8213203435596)) ;
#84997=CARTESIAN_POINT('Origin',(59.3,248.1,30.8213203435596)) ;
#84998=CARTESIAN_POINT('Origin',(59.5,248.1,30.8213203435596)) ;
#84999=CARTESIAN_POINT('Origin',(56.3999999999999,248.,19.9213203435596)) ;
#85000=CARTESIAN_POINT('',(55.05,248.,30.8213203435596)) ;
#85001=CARTESIAN_POINT('',(56.5,248.,31.8213203435596)) ;
#85002=CARTESIAN_POINT('',(56.5,248.,19.9213203435596)) ;
#85003=CARTESIAN_POINT('',(59.3,248.,31.8213203435596)) ;
#85004=CARTESIAN_POINT('',(55.05,248.,31.8213203435596)) ;
#85005=CARTESIAN_POINT('',(59.3,248.,19.9213203435596)) ;
#85006=CARTESIAN_POINT('Origin',(56.8,256.9,31.8213203435596)) ;
#85007=CARTESIAN_POINT('Origin',(56.6,256.9,31.8213203435596)) ;
#85008=CARTESIAN_POINT('Origin',(56.8,257.1,31.8213203435596)) ;
#85009=CARTESIAN_POINT('Origin',(56.6,251.1,31.8213203435596)) ;
#85010=CARTESIAN_POINT('Origin',(56.6,251.1,31.8213203435596)) ;
#85011=CARTESIAN_POINT('Origin',(56.6,251.1,31.8213203435596)) ;
#85012=CARTESIAN_POINT('Origin',(56.6,248.191753592594,31.8213203435596)) ;
#85013=CARTESIAN_POINT('Origin',(59.,256.9,31.8213203435596)) ;
#85014=CARTESIAN_POINT('Origin',(59.,257.1,31.8213203435596)) ;
#85015=CARTESIAN_POINT('Origin',(59.2,256.9,31.8213203435596)) ;
#85016=CARTESIAN_POINT('Origin',(56.4,257.1,31.8213203435596)) ;
#85017=CARTESIAN_POINT('Origin',(56.5,250.9,31.8213203435596)) ;
#85018=CARTESIAN_POINT('',(56.3999999999999,250.9,31.8213203435596)) ;
#85019=CARTESIAN_POINT('Origin',(56.3,250.9,31.8213203435596)) ;
#85020=CARTESIAN_POINT('Origin',(56.5,250.9,31.8213203435596)) ;
#85021=CARTESIAN_POINT('Origin',(56.5,251.1,31.8213203435596)) ;
#85022=CARTESIAN_POINT('Origin',(59.2,251.1,31.8213203435596)) ;
#85023=CARTESIAN_POINT('Origin',(59.2,251.1,31.8213203435596)) ;
#85024=CARTESIAN_POINT('Origin',(59.2,251.1,31.8213203435596)) ;
#85025=CARTESIAN_POINT('Origin',(59.2,245.191753592594,31.8213203435596)) ;
#85026=CARTESIAN_POINT('Origin',(56.5,248.1,31.8213203435596)) ;
#85027=CARTESIAN_POINT('Origin',(56.5,247.9,31.8213203435596)) ;
#85028=CARTESIAN_POINT('',(56.3999999999999,248.1,31.8213203435596)) ;
#85029=CARTESIAN_POINT('Origin',(56.5,248.1,31.8213203435596)) ;
#85030=CARTESIAN_POINT('Origin',(56.3,248.1,31.8213203435596)) ;
#85031=CARTESIAN_POINT('Origin',(59.3,250.9,31.8213203435596)) ;
#85032=CARTESIAN_POINT('Origin',(59.3,251.1,31.8213203435596)) ;
#85033=CARTESIAN_POINT('',(59.4,250.9,31.8213203435596)) ;
#85034=CARTESIAN_POINT('Origin',(59.3,250.9,31.8213203435596)) ;
#85035=CARTESIAN_POINT('Origin',(59.5,250.9,31.8213203435596)) ;
#85036=CARTESIAN_POINT('Origin',(56.55,251.1,31.8213203435596)) ;
#85037=CARTESIAN_POINT('Origin',(59.3,250.9,19.9213203435596)) ;
#85038=CARTESIAN_POINT('',(59.4,250.9,19.9213203435596)) ;
#85039=CARTESIAN_POINT('Origin',(59.3,248.1,31.8213203435596)) ;
#85040=CARTESIAN_POINT('',(59.4,248.1,31.8213203435596)) ;
#85041=CARTESIAN_POINT('Origin',(59.5,248.1,31.8213203435596)) ;
#85042=CARTESIAN_POINT('Origin',(59.3,248.1,31.8213203435596)) ;
#85043=CARTESIAN_POINT('Origin',(59.3,247.9,31.8213203435596)) ;
#85044=CARTESIAN_POINT('Origin',(59.5,243.691753592594,31.8213203435596)) ;
#85045=CARTESIAN_POINT('',(59.4,243.691753592594,31.8213203435596)) ;
#85046=CARTESIAN_POINT('Origin',(59.3,248.1,19.9213203435596)) ;
#85047=CARTESIAN_POINT('',(59.4,248.1,19.9213203435596)) ;
#85048=CARTESIAN_POINT('Origin',(55.05,247.9,31.8213203435596)) ;
#85049=CARTESIAN_POINT('Origin',(56.5,248.1,19.9213203435596)) ;
#85050=CARTESIAN_POINT('',(56.3999999999999,248.1,19.9213203435596)) ;
#85051=CARTESIAN_POINT('Origin',(56.3,245.191753592594,31.8213203435596)) ;
#85052=CARTESIAN_POINT('',(56.3999999999999,245.191753592594,31.8213203435596)) ;
#85053=CARTESIAN_POINT('Origin',(56.5,250.9,19.9213203435596)) ;
#85054=CARTESIAN_POINT('',(56.3999999999999,250.9,19.9213203435596)) ;
#85055=CARTESIAN_POINT('Origin',(55.2,251.1,31.8213203435596)) ;
#85056=CARTESIAN_POINT('Origin',(55.05,247.9,30.8213203435596)) ;
#85057=CARTESIAN_POINT('Origin',(59.4,248.,19.9213203435596)) ;
#85058=CARTESIAN_POINT('',(59.4,243.691753592594,30.8213203435596)) ;
#85059=CARTESIAN_POINT('Origin',(59.5,243.691753592594,30.8213203435596)) ;
#85060=CARTESIAN_POINT('Origin',(46.1,248.9,31.8213203435596)) ;
#85061=CARTESIAN_POINT('',(46.1,249.,31.8213203435596)) ;
#85062=CARTESIAN_POINT('Origin',(46.1,249.1,31.8213203435596)) ;
#85063=CARTESIAN_POINT('',(46.2,248.9,31.8213203435596)) ;
#85064=CARTESIAN_POINT('Origin',(46.1,248.9,31.8213203435596)) ;
#85065=CARTESIAN_POINT('Origin',(46.3,248.9,31.8213203435596)) ;
#85066=CARTESIAN_POINT('Origin',(34.3,248.9,31.8213203435596)) ;
#85067=CARTESIAN_POINT('',(34.2,248.9,31.8213203435596)) ;
#85068=CARTESIAN_POINT('Origin',(34.1,248.9,31.8213203435596)) ;
#85069=CARTESIAN_POINT('',(34.3,249.,31.8213203435596)) ;
#85070=CARTESIAN_POINT('Origin',(34.3,248.9,31.8213203435596)) ;
#85071=CARTESIAN_POINT('Origin',(34.3,249.1,31.8213203435596)) ;
#85072=CARTESIAN_POINT('Origin',(26.3,264.9,19.9213203435596)) ;
#85073=CARTESIAN_POINT('Origin',(26.3,264.9,21.9213203435596)) ;
#85074=CARTESIAN_POINT('Origin',(26.3,264.9,30.7213203435596)) ;
#85075=CARTESIAN_POINT('Origin',(26.3,263.8,30.7213203435596)) ;
#85076=CARTESIAN_POINT('Origin',(26.3,263.8,31.8213203435596)) ;
#85077=CARTESIAN_POINT('Origin',(26.3,263.8,30.7213203435596)) ;
#85078=CARTESIAN_POINT('Origin',(26.3,252.191753592594,31.8213203435596)) ;
#85079=CARTESIAN_POINT('Origin',(26.3,245.6,31.8213203435596)) ;
#85080=CARTESIAN_POINT('Origin',(26.8,245.6,31.8213203435596)) ;
#85081=CARTESIAN_POINT('',(26.8,245.,31.8213203435596)) ;
#85082=CARTESIAN_POINT('Origin',(26.8,245.1,31.8213203435596)) ;
#85083=CARTESIAN_POINT('Origin',(26.8,245.6,31.8213203435596)) ;
#85084=CARTESIAN_POINT('Origin',(39.95,245.1,31.8213203435596)) ;
#85085=CARTESIAN_POINT('',(33.6,245.,31.8213203435596)) ;
#85086=CARTESIAN_POINT('Origin',(33.6,245.1,31.8213203435596)) ;
#85087=CARTESIAN_POINT('',(39.95,245.,31.8213203435596)) ;
#85088=CARTESIAN_POINT('Origin',(33.6,245.6,31.8213203435596)) ;
#85089=CARTESIAN_POINT('',(34.2,245.6,31.8213203435596)) ;
#85090=CARTESIAN_POINT('Origin',(34.1,245.6,31.8213203435596)) ;
#85091=CARTESIAN_POINT('Origin',(33.6,245.6,31.8213203435596)) ;
#85092=CARTESIAN_POINT('Origin',(34.1000000000001,244.191753592594,31.8213203435596)) ;
#85093=CARTESIAN_POINT('',(34.2000000000001,244.191753592594,31.8213203435596)) ;
#85094=CARTESIAN_POINT('Origin',(28.2,264.9,21.9213203435596)) ;
#85095=CARTESIAN_POINT('Origin',(77.1999999999999,264.9,21.9213203435596)) ;
#85096=CARTESIAN_POINT('Origin',(79.0999999999999,264.9,21.9213203435596)) ;
#85097=CARTESIAN_POINT('Origin',(79.0999999999999,264.9,19.9213203435596)) ;
#85098=CARTESIAN_POINT('Origin',(79.0999999999999,264.9,30.7213203435596)) ;
#85099=CARTESIAN_POINT('Origin',(79.0999999999999,263.8,30.7213203435596)) ;
#85100=CARTESIAN_POINT('Origin',(79.0999999999999,263.8,31.8213203435596)) ;
#85101=CARTESIAN_POINT('Origin',(79.0999999999999,263.8,30.7213203435596)) ;
#85102=CARTESIAN_POINT('Origin',(79.0999999999999,249.391753592594,31.8213203435596)) ;
#85103=CARTESIAN_POINT('Origin',(79.0999999999999,259.648528137424,31.8213203435596)) ;
#85104=CARTESIAN_POINT('Origin',(79.7999999999999,259.648528137424,31.8213203435596)) ;
#85105=CARTESIAN_POINT('',(79.375735931288,259.224264068712,31.8213203435596)) ;
#85106=CARTESIAN_POINT('Origin',(79.3050252531694,259.153553390593,31.8213203435596)) ;
#85107=CARTESIAN_POINT('Origin',(79.7999999999999,259.648528137424,31.8213203435596)) ;
#85108=CARTESIAN_POINT('Origin',(78.758412525583,259.70016611818,31.8213203435596)) ;
#85109=CARTESIAN_POINT('',(81.0242640687119,257.575735931288,31.8213203435596)) ;
#85110=CARTESIAN_POINT('Origin',(80.9535533905932,257.50502525317,31.8213203435596)) ;
#85111=CARTESIAN_POINT('',(78.8291232037016,259.770876796298,31.8213203435596)) ;
#85112=CARTESIAN_POINT('Origin',(80.6,257.151471862576,31.8213203435596)) ;
#85113=CARTESIAN_POINT('',(81.2,257.151471862576,31.8213203435596)) ;
#85114=CARTESIAN_POINT('Origin',(81.1,257.151471862576,31.8213203435596)) ;
#85115=CARTESIAN_POINT('Origin',(80.6,257.151471862576,31.8213203435596)) ;
#85116=CARTESIAN_POINT('Origin',(81.1,242.941753592594,31.8213203435596)) ;
#85117=CARTESIAN_POINT('',(81.2,247.098386676966,31.8213203435596)) ;
#85118=CARTESIAN_POINT('Origin',(81.1,247.098386676966,31.8213203435596)) ;
#85119=CARTESIAN_POINT('',(81.2,242.941753592594,31.8213203435596)) ;
#85120=CARTESIAN_POINT('Origin',(80.6,247.098386676966,31.8213203435596)) ;
#85121=CARTESIAN_POINT('',(80.6193548387097,246.498698933037,31.8213203435596)) ;
#85122=CARTESIAN_POINT('Origin',(80.616129032258,246.598646890358,31.8213203435596)) ;
#85123=CARTESIAN_POINT('Origin',(80.6,247.098386676966,31.8213203435596)) ;
#85124=CARTESIAN_POINT('Origin',(80.6999999999999,244.,31.8213203435596)) ;
#85125=CARTESIAN_POINT('',(78.1999999999999,244.,31.8213203435596)) ;
#85126=CARTESIAN_POINT('Origin',(78.0999999999999,244.,31.8213203435596)) ;
#85127=CARTESIAN_POINT('Origin',(80.6999999999999,244.,31.8213203435596)) ;
#85128=CARTESIAN_POINT('Origin',(78.0999999999999,239.691753592594,31.8213203435596)) ;
#85129=CARTESIAN_POINT('',(78.1999999999999,240.,31.8213203435596)) ;
#85130=CARTESIAN_POINT('Origin',(78.0999999999999,240.,31.8213203435596)) ;
#85131=CARTESIAN_POINT('',(78.1999999999999,239.691753592594,31.8213203435596)) ;
#85132=CARTESIAN_POINT('Origin',(80.6999999999999,240.,31.8213203435596)) ;
#85133=CARTESIAN_POINT('',(80.6193548387097,237.501301066963,31.8213203435596)) ;
#85134=CARTESIAN_POINT('Origin',(80.616129032258,237.401353109641,31.8213203435596)) ;
#85135=CARTESIAN_POINT('Origin',(80.6999999999999,240.,31.8213203435596)) ;
#85136=CARTESIAN_POINT('Origin',(80.6,236.901613323034,31.8213203435596)) ;
#85137=CARTESIAN_POINT('',(81.2,236.901613323034,31.8213203435596)) ;
#85138=CARTESIAN_POINT('Origin',(81.1,236.901613323034,31.8213203435596)) ;
#85139=CARTESIAN_POINT('Origin',(80.6,236.901613323034,31.8213203435596)) ;
#85140=CARTESIAN_POINT('Origin',(81.1,232.568672279644,31.8213203435596)) ;
#85141=CARTESIAN_POINT('',(81.2,226.002365511524,31.8213203435596)) ;
#85142=CARTESIAN_POINT('Origin',(81.1,226.002365511524,31.8213203435596)) ;
#85143=CARTESIAN_POINT('',(81.2,232.568672279644,31.8213203435596)) ;
#85144=CARTESIAN_POINT('Origin',(80.6,226.002365511524,31.8213203435596)) ;
#85145=CARTESIAN_POINT('',(81.0242640687119,225.578101442812,31.8213203435596)) ;
#85146=CARTESIAN_POINT('Origin',(80.9535533905933,225.64881212093,31.8213203435596)) ;
#85147=CARTESIAN_POINT('Origin',(80.6,226.002365511524,31.8213203435596)) ;
#85148=CARTESIAN_POINT('Origin',(77.061706774654,221.756965504991,31.8213203435596)) ;
#85149=CARTESIAN_POINT('',(80.1757359312881,224.729573305388,31.8213203435596)) ;
#85150=CARTESIAN_POINT('Origin',(80.1050252531695,224.800283983507,31.8213203435596)) ;
#85151=CARTESIAN_POINT('',(77.1324174527726,221.686254826872,31.8213203435596)) ;
#85152=CARTESIAN_POINT('Origin',(80.6000000000001,224.305309236676,31.8213203435596)) ;
#85153=CARTESIAN_POINT('',(80.0000000000001,224.305309236676,31.8213203435596)) ;
#85154=CARTESIAN_POINT('Origin',(79.9000000000001,224.305309236676,31.8213203435596)) ;
#85155=CARTESIAN_POINT('Origin',(80.6000000000001,224.305309236676,31.8213203435596)) ;
#85156=CARTESIAN_POINT('Origin',(79.9,228.575260777783,31.8213203435596)) ;
#85157=CARTESIAN_POINT('',(80.0000000000001,217.767014370377,31.8213203435596)) ;
#85158=CARTESIAN_POINT('Origin',(79.9000000000001,217.767014370377,31.8213203435596)) ;
#85159=CARTESIAN_POINT('',(80.,228.575260777783,31.8213203435596)) ;
#85160=CARTESIAN_POINT('Origin',(76.0000000000001,217.767014370377,31.8213203435596)) ;
#85161=CARTESIAN_POINT('',(75.3054072893324,213.827783358328,31.8213203435596)) ;
#85162=CARTESIAN_POINT('Origin',(75.3227721070991,213.926264133629,31.8213203435596)) ;
#85163=CARTESIAN_POINT('Origin',(76.0000000000001,217.767014370377,31.8213203435596)) ;
#85164=CARTESIAN_POINT('Origin',(56.086380506565,217.318158984277,31.8213203435596)) ;
#85165=CARTESIAN_POINT('',(63.7885177058986,215.858521725728,31.8213203435596)) ;
#85166=CARTESIAN_POINT('Origin',(63.8058825236653,215.957002501029,31.8213203435596)) ;
#85167=CARTESIAN_POINT('',(56.0690156887983,217.219678208976,31.8213203435596)) ;
#85168=CARTESIAN_POINT('Origin',(64.4831104165663,219.797752737776,31.8213203435596)) ;
#85169=CARTESIAN_POINT('',(61.2065022394103,217.503446992372,31.8213203435596)) ;
#85170=CARTESIAN_POINT('Origin',(61.2884174438392,217.560804636007,31.8213203435596)) ;
#85171=CARTESIAN_POINT('Origin',(64.4831104165663,219.797752737776,31.8213203435596)) ;
#85172=CARTESIAN_POINT('Origin',(52.2889313872861,230.413402709377,31.8213203435596)) ;
#85173=CARTESIAN_POINT('',(56.6807511357248,223.966889410112,31.8213203435596)) ;
#85174=CARTESIAN_POINT('Origin',(56.7626663401537,224.024247053747,31.8213203435596)) ;
#85175=CARTESIAN_POINT('',(52.2070161828572,230.356045065742,31.8213203435596)) ;
#85176=CARTESIAN_POINT('Origin',(59.9573593128808,226.261195155516,31.8213203435596)) ;
#85177=CARTESIAN_POINT('',(55.9573593128808,226.261195155516,31.8213203435596)) ;
#85178=CARTESIAN_POINT('Origin',(56.0573593128808,226.261195155516,31.8213203435596)) ;
#85179=CARTESIAN_POINT('Origin',(59.9573593128808,226.261195155516,31.8213203435596)) ;
#85180=CARTESIAN_POINT('Origin',(56.0573593128807,242.191753592594,31.8213203435596)) ;
#85181=CARTESIAN_POINT('',(55.9573593128808,244.4,31.8213203435596)) ;
#85182=CARTESIAN_POINT('Origin',(56.0573593128807,244.4,31.8213203435596)) ;
#85183=CARTESIAN_POINT('',(55.9573593128808,242.191753592594,31.8213203435596)) ;
#85184=CARTESIAN_POINT('Origin',(55.3573593128808,244.4,31.8213203435596)) ;
#85185=CARTESIAN_POINT('',(55.3573593128808,245.,31.8213203435596)) ;
#85186=CARTESIAN_POINT('Origin',(55.3573593128808,245.1,31.8213203435596)) ;
#85187=CARTESIAN_POINT('Origin',(55.3573593128808,244.4,31.8213203435596)) ;
#85188=CARTESIAN_POINT('Origin',(39.95,245.1,31.8213203435596)) ;
#85189=CARTESIAN_POINT('',(46.8,245.,31.8213203435596)) ;
#85190=CARTESIAN_POINT('Origin',(46.8,245.1,31.8213203435596)) ;
#85191=CARTESIAN_POINT('',(39.95,245.,31.8213203435596)) ;
#85192=CARTESIAN_POINT('Origin',(46.8,245.6,31.8213203435596)) ;
#85193=CARTESIAN_POINT('',(46.2,245.6,31.8213203435596)) ;
#85194=CARTESIAN_POINT('Origin',(46.2999999999999,245.6,31.8213203435596)) ;
#85195=CARTESIAN_POINT('Origin',(46.8,245.6,31.8213203435596)) ;
#85196=CARTESIAN_POINT('Origin',(46.2999999999999,242.191753592594,31.8213203435596)) ;
#85197=CARTESIAN_POINT('',(46.1999999999999,242.191753592594,31.8213203435596)) ;
#85198=CARTESIAN_POINT('Origin',(34.1,248.9,30.8213203435596)) ;
#85199=CARTESIAN_POINT('',(34.3,249.,30.8213203435596)) ;
#85200=CARTESIAN_POINT('',(34.2,248.9,30.8213203435596)) ;
#85201=CARTESIAN_POINT('Origin',(34.3,248.9,30.8213203435596)) ;
#85202=CARTESIAN_POINT('Origin',(34.1,248.9,30.8213203435596)) ;
#85203=CARTESIAN_POINT('Origin',(34.1,249.,30.8213203435596)) ;
#85204=CARTESIAN_POINT('Origin',(34.3,248.9,19.9213203435596)) ;
#85205=CARTESIAN_POINT('',(34.2,248.9,19.9213203435596)) ;
#85206=CARTESIAN_POINT('',(34.3,249.,19.9213203435596)) ;
#85207=CARTESIAN_POINT('Origin',(49.95,249.1,31.8213203435596)) ;
#85208=CARTESIAN_POINT('',(49.95,249.,31.8213203435596)) ;
#85209=CARTESIAN_POINT('Origin',(46.1,248.9,19.9213203435596)) ;
#85210=CARTESIAN_POINT('',(46.1,249.,30.8213203435596)) ;
#85211=CARTESIAN_POINT('',(46.2,248.9,30.8213203435596)) ;
#85212=CARTESIAN_POINT('Origin',(46.1,248.9,30.8213203435596)) ;
#85213=CARTESIAN_POINT('',(46.2,248.9,19.9213203435596)) ;
#85214=CARTESIAN_POINT('',(46.1,249.,19.9213203435596)) ;
#85215=CARTESIAN_POINT('Origin',(46.3,248.9,30.8213203435596)) ;
#85216=CARTESIAN_POINT('Origin',(46.3,248.9,30.8213203435596)) ;
#85217=CARTESIAN_POINT('Origin',(46.3,249.,30.8213203435596)) ;
#85218=CARTESIAN_POINT('Origin',(66.4499999999999,263.8,30.7213203435596)) ;
#85219=CARTESIAN_POINT('',(77.7056259120663,264.647498436458,31.5708769339063)) ;
#85220=CARTESIAN_POINT('Origin',(78.2,263.8,30.7213203435596)) ;
#85221=CARTESIAN_POINT('Origin',(78.2,263.8,30.7213203435596)) ;
#85222=CARTESIAN_POINT('Origin',(81.2,257.4,19.9213203435596)) ;
#85223=CARTESIAN_POINT('',(81.0242640687119,257.575735931288,30.8213203435596)) ;
#85224=CARTESIAN_POINT('',(81.0242640687119,257.575735931288,19.9213203435596)) ;
#85225=CARTESIAN_POINT('',(79.375735931288,259.224264068712,30.8213203435596)) ;
#85226=CARTESIAN_POINT('',(78.8291232037016,259.770876796298,30.8213203435596)) ;
#85227=CARTESIAN_POINT('',(79.375735931288,259.224264068712,19.9213203435596)) ;
#85228=CARTESIAN_POINT('Origin',(80.6,257.151471862576,19.9213203435596)) ;
#85229=CARTESIAN_POINT('',(81.2,257.151471862576,30.8213203435596)) ;
#85230=CARTESIAN_POINT('',(81.2,257.151471862576,19.9213203435596)) ;
#85231=CARTESIAN_POINT('Origin',(80.6,257.151471862576,30.8213203435596)) ;
#85232=CARTESIAN_POINT('Origin',(81.2,246.5,19.9213203435596)) ;
#85233=CARTESIAN_POINT('',(81.2,247.098386676966,30.8213203435596)) ;
#85234=CARTESIAN_POINT('',(81.2,247.098386676966,19.9213203435596)) ;
#85235=CARTESIAN_POINT('',(81.2,242.941753592594,30.8213203435596)) ;
#85236=CARTESIAN_POINT('Origin',(80.6,247.098386676966,19.9213203435596)) ;
#85237=CARTESIAN_POINT('',(80.6193548387097,246.498698933037,30.8213203435596)) ;
#85238=CARTESIAN_POINT('',(80.6193548387097,246.498698933037,19.9213203435596)) ;
#85239=CARTESIAN_POINT('Origin',(80.6,247.098386676966,30.8213203435596)) ;
#85240=CARTESIAN_POINT('Origin',(80.6999999999999,244.,19.9213203435596)) ;
#85241=CARTESIAN_POINT('',(78.1999999999999,244.,30.8213203435596)) ;
#85242=CARTESIAN_POINT('',(78.1999999999999,244.,19.9213203435596)) ;
#85243=CARTESIAN_POINT('Origin',(80.6999999999999,244.,30.8213203435596)) ;
#85244=CARTESIAN_POINT('Origin',(78.1999999999999,240.,19.9213203435596)) ;
#85245=CARTESIAN_POINT('',(78.1999999999999,240.,30.8213203435596)) ;
#85246=CARTESIAN_POINT('',(78.1999999999999,240.,19.9213203435596)) ;
#85247=CARTESIAN_POINT('',(78.1999999999999,239.691753592594,30.8213203435596)) ;
#85248=CARTESIAN_POINT('Origin',(80.6999999999999,240.,19.9213203435596)) ;
#85249=CARTESIAN_POINT('',(80.6193548387097,237.501301066963,30.8213203435596)) ;
#85250=CARTESIAN_POINT('',(80.6193548387097,237.501301066963,19.9213203435596)) ;
#85251=CARTESIAN_POINT('Origin',(80.6999999999999,240.,30.8213203435596)) ;
#85252=CARTESIAN_POINT('Origin',(80.6,236.901613323034,19.9213203435596)) ;
#85253=CARTESIAN_POINT('',(81.2,236.901613323034,30.8213203435596)) ;
#85254=CARTESIAN_POINT('',(81.2,236.901613323034,19.9213203435596)) ;
#85255=CARTESIAN_POINT('Origin',(80.6,236.901613323034,30.8213203435596)) ;
#85256=CARTESIAN_POINT('Origin',(81.2,225.7538373741,19.9213203435596)) ;
#85257=CARTESIAN_POINT('',(81.2,226.002365511524,30.8213203435596)) ;
#85258=CARTESIAN_POINT('',(81.2,226.002365511524,19.9213203435596)) ;
#85259=CARTESIAN_POINT('',(81.2,232.568672279644,30.8213203435596)) ;
#85260=CARTESIAN_POINT('Origin',(80.6,226.002365511524,19.9213203435596)) ;
#85261=CARTESIAN_POINT('',(81.0242640687119,225.578101442812,30.8213203435596)) ;
#85262=CARTESIAN_POINT('',(81.0242640687119,225.578101442812,19.9213203435596)) ;
#85263=CARTESIAN_POINT('Origin',(80.6,226.002365511524,30.8213203435596)) ;
#85264=CARTESIAN_POINT('Origin',(80.0000000000001,224.5538373741,19.9213203435596)) ;
#85265=CARTESIAN_POINT('',(80.1757359312881,224.729573305388,30.8213203435596)) ;
#85266=CARTESIAN_POINT('',(80.1757359312881,224.729573305388,19.9213203435596)) ;
#85267=CARTESIAN_POINT('',(77.1324174527726,221.686254826872,30.8213203435596)) ;
#85268=CARTESIAN_POINT('Origin',(80.6000000000001,224.305309236676,19.9213203435596)) ;
#85269=CARTESIAN_POINT('',(80.0000000000001,224.305309236676,30.8213203435596)) ;
#85270=CARTESIAN_POINT('',(80.0000000000001,224.305309236676,19.9213203435596)) ;
#85271=CARTESIAN_POINT('Origin',(80.6000000000001,224.305309236676,30.8213203435596)) ;
#85272=CARTESIAN_POINT('Origin',(80.0000000000001,217.767014370377,19.9213203435596)) ;
#85273=CARTESIAN_POINT('',(80.0000000000001,217.767014370377,30.8213203435596)) ;
#85274=CARTESIAN_POINT('',(80.0000000000001,217.767014370377,19.9213203435596)) ;
#85275=CARTESIAN_POINT('',(80.,228.575260777783,30.8213203435596)) ;
#85276=CARTESIAN_POINT('Origin',(76.0000000000001,217.767014370377,19.9213203435596)) ;
#85277=CARTESIAN_POINT('',(75.3054072893324,213.827783358328,30.8213203435596)) ;
#85278=CARTESIAN_POINT('',(75.3054072893324,213.827783358328,19.9213203435596)) ;
#85279=CARTESIAN_POINT('Origin',(76.0000000000001,217.767014370377,30.8213203435596)) ;
#85280=CARTESIAN_POINT('Origin',(62.1568347953873,216.146231446812,19.9213203435596)) ;
#85281=CARTESIAN_POINT('',(63.7885177058986,215.858521725728,30.8213203435596)) ;
#85282=CARTESIAN_POINT('',(63.7885177058986,215.858521725728,19.9213203435596)) ;
#85283=CARTESIAN_POINT('',(56.0690156887983,217.219678208976,30.8213203435596)) ;
#85284=CARTESIAN_POINT('Origin',(64.4831104165663,219.797752737776,19.9213203435596)) ;
#85285=CARTESIAN_POINT('',(61.2065022394103,217.503446992372,30.8213203435596)) ;
#85286=CARTESIAN_POINT('',(61.2065022394103,217.503446992372,19.9213203435596)) ;
#85287=CARTESIAN_POINT('Origin',(64.4831104165663,219.797752737776,30.8213203435596)) ;
#85288=CARTESIAN_POINT('Origin',(55.9573593128808,225.,19.9213203435596)) ;
#85289=CARTESIAN_POINT('',(56.6807511357248,223.966889410112,30.8213203435596)) ;
#85290=CARTESIAN_POINT('',(56.6807511357248,223.966889410112,19.9213203435596)) ;
#85291=CARTESIAN_POINT('',(52.2070161828572,230.356045065742,30.8213203435596)) ;
#85292=CARTESIAN_POINT('Origin',(59.9573593128808,226.261195155516,19.9213203435596)) ;
#85293=CARTESIAN_POINT('',(55.9573593128808,226.261195155516,30.8213203435596)) ;
#85294=CARTESIAN_POINT('',(55.9573593128808,226.261195155516,19.9213203435596)) ;
#85295=CARTESIAN_POINT('Origin',(59.9573593128808,226.261195155516,30.8213203435596)) ;
#85296=CARTESIAN_POINT('Origin',(55.9573593128808,245.,19.9213203435596)) ;
#85297=CARTESIAN_POINT('',(55.9573593128808,244.4,30.8213203435596)) ;
#85298=CARTESIAN_POINT('',(55.9573593128808,244.4,19.9213203435596)) ;
#85299=CARTESIAN_POINT('',(55.9573593128808,242.191753592594,30.8213203435596)) ;
#85300=CARTESIAN_POINT('Origin',(55.3573593128808,244.4,19.9213203435596)) ;
#85301=CARTESIAN_POINT('',(55.3573593128808,245.,30.8213203435596)) ;
#85302=CARTESIAN_POINT('',(55.3573593128808,245.,19.9213203435596)) ;
#85303=CARTESIAN_POINT('Origin',(55.3573593128808,244.4,30.8213203435596)) ;
#85304=CARTESIAN_POINT('Origin',(26.2,245.,19.9213203435596)) ;
#85305=CARTESIAN_POINT('',(46.8,245.,30.8213203435596)) ;
#85306=CARTESIAN_POINT('',(46.8,245.,19.9213203435596)) ;
#85307=CARTESIAN_POINT('',(39.95,245.,30.8213203435596)) ;
#85308=CARTESIAN_POINT('Origin',(46.8,245.6,19.9213203435596)) ;
#85309=CARTESIAN_POINT('',(46.2,245.6,30.8213203435596)) ;
#85310=CARTESIAN_POINT('',(46.2,245.6,19.9213203435596)) ;
#85311=CARTESIAN_POINT('Origin',(46.8,245.6,30.8213203435596)) ;
#85312=CARTESIAN_POINT('Origin',(46.2,245.,19.9213203435596)) ;
#85313=CARTESIAN_POINT('',(46.1999999999999,242.191753592594,30.8213203435596)) ;
#85314=CARTESIAN_POINT('Origin',(46.2999999999999,242.191753592594,30.8213203435596)) ;
#85315=CARTESIAN_POINT('Origin',(46.2999999999999,245.6,30.8213203435596)) ;
#85316=CARTESIAN_POINT('Origin',(79.2999999999999,229.3,25.9213203435596)) ;
#85317=CARTESIAN_POINT('',(79.2999999999999,229.4,25.9213203435596)) ;
#85318=CARTESIAN_POINT('',(79.1999999999999,229.3,25.9213203435596)) ;
#85319=CARTESIAN_POINT('Origin',(79.2999999999999,229.3,25.9213203435596)) ;
#85320=CARTESIAN_POINT('',(79.1999999999999,229.3,30.9213203435596)) ;
#85321=CARTESIAN_POINT('',(79.1999999999999,229.3,25.9213203435596)) ;
#85322=CARTESIAN_POINT('',(79.2999999999999,229.4,30.9213203435596)) ;
#85323=CARTESIAN_POINT('Origin',(79.2999999999999,229.3,30.9213203435596)) ;
#85324=CARTESIAN_POINT('',(79.2999999999999,229.4,25.9213203435596)) ;
#85325=CARTESIAN_POINT('Origin',(80.1999999999999,229.3,30.9213203435596)) ;
#85326=CARTESIAN_POINT('',(80.199999999999,229.4,31.8213203435596)) ;
#85327=CARTESIAN_POINT('Origin',(80.1999999999999,229.3,31.8213203435596)) ;
#85328=CARTESIAN_POINT('Origin',(80.1999999999999,229.4,30.9213203435596)) ;
#85329=CARTESIAN_POINT('Origin',(80.1999999999999,229.3,30.9213203435596)) ;
#85330=CARTESIAN_POINT('Origin',(66.9499999999995,229.3,31.8213203435596)) ;
#85331=CARTESIAN_POINT('Origin',(80.299999999999,229.3,31.8213203435596)) ;
#85332=CARTESIAN_POINT('Origin',(80.1999999999999,234.391753592594,30.9213203435596)) ;
#85333=CARTESIAN_POINT('',(79.1999999999999,226.7,30.9213203435596)) ;
#85334=CARTESIAN_POINT('',(79.1999999999999,234.391753592594,30.9213203435596)) ;
#85335=CARTESIAN_POINT('Origin',(80.1999999999999,226.7,30.9213203435596)) ;
#85336=CARTESIAN_POINT('Origin',(79.1999999999999,229.4,25.9213203435596)) ;
#85337=CARTESIAN_POINT('',(79.1999999999999,226.7,25.9213203435596)) ;
#85338=CARTESIAN_POINT('',(79.1999999999999,226.6,25.9213203435596)) ;
#85339=CARTESIAN_POINT('',(79.1999999999999,226.7,25.9213203435596)) ;
#85340=CARTESIAN_POINT('Origin',(79.6999999999999,228.,25.9213203435596)) ;
#85341=CARTESIAN_POINT('',(80.199999999999,229.4,25.9213203435596)) ;
#85342=CARTESIAN_POINT('',(79.1999999999999,229.4,25.9213203435596)) ;
#85343=CARTESIAN_POINT('',(80.199999999999,226.6,25.9213203435596)) ;
#85344=CARTESIAN_POINT('',(80.199999999999,230.5,25.9213203435596)) ;
#85345=CARTESIAN_POINT('',(79.2999999999999,226.6,25.9213203435596)) ;
#85346=CARTESIAN_POINT('',(80.1999999999999,226.6,25.9213203435596)) ;
#85347=CARTESIAN_POINT('Origin',(79.2999999999999,226.7,25.9213203435596)) ;
#85348=CARTESIAN_POINT('Origin',(79.2999999999999,226.7,25.9213203435596)) ;
#85349=CARTESIAN_POINT('',(79.2999999999999,226.6,30.9213203435596)) ;
#85350=CARTESIAN_POINT('',(79.2999999999999,226.6,25.9213203435596)) ;
#85351=CARTESIAN_POINT('Origin',(79.2999999999999,226.7,30.9213203435596)) ;
#85352=CARTESIAN_POINT('Origin',(80.1999999999999,226.7,30.9213203435596)) ;
#85353=CARTESIAN_POINT('',(80.199999999999,226.6,31.8213203435596)) ;
#85354=CARTESIAN_POINT('Origin',(80.199999999999,226.7,31.8213203435596)) ;
#85355=CARTESIAN_POINT('Origin',(80.1999999999999,226.6,30.9213203435596)) ;
#85356=CARTESIAN_POINT('Origin',(66.4499999999997,226.700000000001,31.8213203435596)) ;
#85357=CARTESIAN_POINT('Origin',(80.299999999999,226.7,31.8213203435596)) ;
#85358=CARTESIAN_POINT('Origin',(79.1999999999999,226.6,25.9213203435596)) ;
#85359=CARTESIAN_POINT('',(80.199999999999,226.6,25.9213203435596)) ;
#85360=CARTESIAN_POINT('',(80.199999999999,226.6,22.9213203435596)) ;
#85361=CARTESIAN_POINT('Origin',(80.099999999999,230.4,31.8213203435596)) ;
#85362=CARTESIAN_POINT('',(80.099999999999,230.5,31.8213203435596)) ;
#85363=CARTESIAN_POINT('Origin',(80.099999999999,230.6,31.8213203435596)) ;
#85364=CARTESIAN_POINT('',(80.199999999999,230.4,31.8213203435596)) ;
#85365=CARTESIAN_POINT('Origin',(80.099999999999,230.4,31.8213203435596)) ;
#85366=CARTESIAN_POINT('Origin',(80.299999999999,230.4,31.8213203435596)) ;
#85367=CARTESIAN_POINT('Origin',(76.0414213562367,230.4,31.8213203435596)) ;
#85368=CARTESIAN_POINT('',(76.0414213562367,230.5,31.8213203435596)) ;
#85369=CARTESIAN_POINT('',(75.9707106781181,230.470710678119,31.8213203435596)) ;
#85370=CARTESIAN_POINT('Origin',(76.0414213562367,230.4,31.8213203435596)) ;
#85371=CARTESIAN_POINT('Origin',(76.0414213562367,230.6,31.8213203435596)) ;
#85372=CARTESIAN_POINT('Origin',(75.8999999999994,230.541421356237,31.8213203435596)) ;
#85373=CARTESIAN_POINT('Origin',(66.9499999999995,230.6,31.8213203435596)) ;
#85374=CARTESIAN_POINT('',(66.9499999999995,230.5,31.8213203435596)) ;
#85375=CARTESIAN_POINT('Origin',(75.2999999999994,229.658578643763,31.8213203435596)) ;
#85376=CARTESIAN_POINT('',(75.2292893218808,229.729289321881,31.8213203435596)) ;
#85377=CARTESIAN_POINT('',(75.1999999999994,229.658578643763,31.8213203435596)) ;
#85378=CARTESIAN_POINT('Origin',(75.2999999999994,229.658578643763,31.8213203435596)) ;
#85379=CARTESIAN_POINT('Origin',(75.1585786437621,229.8,31.8213203435596)) ;
#85380=CARTESIAN_POINT('Origin',(75.0999999999994,229.658578643763,31.8213203435596)) ;
#85381=CARTESIAN_POINT('Origin',(72.3751661181778,227.016587474416,31.8213203435596)) ;
#85382=CARTESIAN_POINT('',(72.4458767962964,226.945876796297,31.8213203435596)) ;
#85383=CARTESIAN_POINT('Origin',(75.2999999999993,226.341421356237,31.8213203435596)) ;
#85384=CARTESIAN_POINT('',(75.1999999999993,226.341421356237,31.8213203435596)) ;
#85385=CARTESIAN_POINT('',(75.2292893218806,226.270710678119,31.8213203435596)) ;
#85386=CARTESIAN_POINT('Origin',(75.2999999999993,226.341421356237,31.8213203435596)) ;
#85387=CARTESIAN_POINT('Origin',(75.0999999999993,226.341421356237,31.8213203435596)) ;
#85388=CARTESIAN_POINT('Origin',(75.158578643762,226.2,31.8213203435596)) ;
#85389=CARTESIAN_POINT('Origin',(75.0999999999996,234.941753592594,31.8213203435596)) ;
#85390=CARTESIAN_POINT('',(75.1999999999996,234.941753592594,31.8213203435596)) ;
#85391=CARTESIAN_POINT('Origin',(76.0414213562366,225.6,31.8213203435596)) ;
#85392=CARTESIAN_POINT('',(75.9707106781179,225.529289321881,31.8213203435596)) ;
#85393=CARTESIAN_POINT('',(76.0414213562366,225.5,31.8213203435596)) ;
#85394=CARTESIAN_POINT('Origin',(76.0414213562366,225.6,31.8213203435596)) ;
#85395=CARTESIAN_POINT('Origin',(75.8999999999993,225.458578643763,31.8213203435596)) ;
#85396=CARTESIAN_POINT('Origin',(76.0414213562366,225.4,31.8213203435596)) ;
#85397=CARTESIAN_POINT('Origin',(66.6834125255838,234.675166118178,31.8213203435596)) ;
#85398=CARTESIAN_POINT('',(66.7541232037024,234.745876796297,31.8213203435596)) ;
#85399=CARTESIAN_POINT('Origin',(80.0999999999989,225.6,31.8213203435596)) ;
#85400=CARTESIAN_POINT('',(80.199999999999,225.6,31.8213203435596)) ;
#85401=CARTESIAN_POINT('Origin',(80.2999999999989,225.6,31.8213203435596)) ;
#85402=CARTESIAN_POINT('',(80.0999999999989,225.5,31.8213203435596)) ;
#85403=CARTESIAN_POINT('Origin',(80.0999999999989,225.6,31.8213203435596)) ;
#85404=CARTESIAN_POINT('Origin',(80.0999999999989,225.4,31.8213203435596)) ;
#85405=CARTESIAN_POINT('Origin',(80.299999999999,232.441753592594,31.8213203435596)) ;
#85406=CARTESIAN_POINT('',(80.199999999999,232.441753592594,31.8213203435596)) ;
#85407=CARTESIAN_POINT('Origin',(80.0999999999989,225.6,19.9213203435596)) ;
#85408=CARTESIAN_POINT('',(80.0999999999989,225.5,19.9213203435596)) ;
#85409=CARTESIAN_POINT('',(80.199999999999,225.6,19.9213203435596)) ;
#85410=CARTESIAN_POINT('Origin',(64.4499999999996,225.4,31.8213203435596)) ;
#85411=CARTESIAN_POINT('',(64.4499999999996,225.5,31.8213203435596)) ;
#85412=CARTESIAN_POINT('Origin',(76.0414213562366,225.6,19.9213203435596)) ;
#85413=CARTESIAN_POINT('',(75.9707106781179,225.529289321881,19.9213203435596)) ;
#85414=CARTESIAN_POINT('',(76.0414213562366,225.5,19.9213203435596)) ;
#85415=CARTESIAN_POINT('Origin',(75.2999999999993,226.341421356237,19.9213203435596)) ;
#85416=CARTESIAN_POINT('',(75.1999999999993,226.341421356237,19.9213203435596)) ;
#85417=CARTESIAN_POINT('',(75.2292893218806,226.270710678119,19.9213203435596)) ;
#85418=CARTESIAN_POINT('Origin',(75.2999999999994,229.658578643763,19.9213203435596)) ;
#85419=CARTESIAN_POINT('',(75.2292893218808,229.729289321881,19.9213203435596)) ;
#85420=CARTESIAN_POINT('',(75.1999999999994,229.658578643763,19.9213203435596)) ;
#85421=CARTESIAN_POINT('Origin',(76.0414213562367,230.4,19.9213203435596)) ;
#85422=CARTESIAN_POINT('',(76.0414213562367,230.5,19.9213203435596)) ;
#85423=CARTESIAN_POINT('',(75.9707106781181,230.470710678119,19.9213203435596)) ;
#85424=CARTESIAN_POINT('Origin',(80.099999999999,230.4,19.9213203435596)) ;
#85425=CARTESIAN_POINT('',(80.199999999999,230.4,19.9213203435596)) ;
#85426=CARTESIAN_POINT('',(80.099999999999,230.5,19.9213203435596)) ;
#85427=CARTESIAN_POINT('Origin',(80.299999999999,232.441753592594,31.8213203435596)) ;
#85428=CARTESIAN_POINT('',(80.199999999999,232.441753592594,31.8213203435596)) ;
#85429=CARTESIAN_POINT('Origin',(75.1999999999993,225.5,19.9213203435596)) ;
#85430=CARTESIAN_POINT('Origin',(80.199999999999,225.5,19.9213203435596)) ;
#85431=CARTESIAN_POINT('Origin',(74.2999999999999,226.1,31.8213203435596)) ;
#85432=CARTESIAN_POINT('',(74.2999999999999,226.,31.8213203435596)) ;
#85433=CARTESIAN_POINT('Origin',(74.2999999999999,226.1,31.8213203435596)) ;
#85434=CARTESIAN_POINT('',(74.1999999999999,226.1,31.8213203435596)) ;
#85435=CARTESIAN_POINT('Origin',(74.2999999999999,226.1,31.8213203435596)) ;
#85436=CARTESIAN_POINT('Origin',(74.2999999999999,226.1,31.8213203435596)) ;
#85437=CARTESIAN_POINT('Origin',(74.3999999999999,225.9,31.8213203435596)) ;
#85438=CARTESIAN_POINT('',(74.3999999999999,226.,31.8213203435596)) ;
#85439=CARTESIAN_POINT('Origin',(74.3999999999999,226.1,31.8213203435596)) ;
#85440=CARTESIAN_POINT('',(74.4999999999999,225.9,31.8213203435596)) ;
#85441=CARTESIAN_POINT('Origin',(74.3999999999999,225.9,31.8213203435596)) ;
#85442=CARTESIAN_POINT('Origin',(74.5999999999999,225.9,31.8213203435596)) ;
#85443=CARTESIAN_POINT('Origin',(64.1,226.1,31.8213203435596)) ;
#85444=CARTESIAN_POINT('',(64.1,226.,31.8213203435596)) ;
#85445=CARTESIAN_POINT('Origin',(74.3999999999999,225.9,19.9213203435596)) ;
#85446=CARTESIAN_POINT('',(74.4999999999999,225.9,19.9213203435596)) ;
#85447=CARTESIAN_POINT('',(74.3999999999999,226.,19.9213203435596)) ;
#85448=CARTESIAN_POINT('Origin',(74.0999999999999,231.9,31.8213203435596)) ;
#85449=CARTESIAN_POINT('',(74.0999999999999,232.,31.8213203435596)) ;
#85450=CARTESIAN_POINT('Origin',(74.0999999999999,232.1,31.8213203435596)) ;
#85451=CARTESIAN_POINT('',(74.1999999999999,231.9,31.8213203435596)) ;
#85452=CARTESIAN_POINT('Origin',(74.0999999999999,231.9,31.8213203435596)) ;
#85453=CARTESIAN_POINT('Origin',(74.2999999999999,231.9,31.8213203435596)) ;
#85454=CARTESIAN_POINT('Origin',(74.3999999999999,223.1,31.8213203435596)) ;
#85455=CARTESIAN_POINT('Origin',(74.5999999999999,223.1,31.8213203435596)) ;
#85456=CARTESIAN_POINT('Origin',(74.3999999999999,222.9,31.8213203435596)) ;
#85457=CARTESIAN_POINT('Origin',(74.5999999999999,231.191753592594,31.8213203435596)) ;
#85458=CARTESIAN_POINT('',(74.4999999999999,231.191753592594,31.8213203435596)) ;
#85459=CARTESIAN_POINT('Origin',(71.8999999999999,231.9,31.8213203435596)) ;
#85460=CARTESIAN_POINT('',(71.8999999999999,232.,31.8213203435596)) ;
#85461=CARTESIAN_POINT('Origin',(71.8999999999999,231.9,31.8213203435596)) ;
#85462=CARTESIAN_POINT('Origin',(71.8999999999999,232.1,31.8213203435596)) ;
#85463=CARTESIAN_POINT('Origin',(71.6999999999999,231.9,31.8213203435596)) ;
#85464=CARTESIAN_POINT('Origin',(63.95,232.1,31.8213203435596)) ;
#85465=CARTESIAN_POINT('',(63.95,232.,31.8213203435596)) ;
#85466=CARTESIAN_POINT('Origin',(71.5999999999999,223.1,31.8213203435596)) ;
#85467=CARTESIAN_POINT('Origin',(71.5999999999999,222.9,31.8213203435596)) ;
#85468=CARTESIAN_POINT('Origin',(71.3999999999999,223.1,31.8213203435596)) ;
#85469=CARTESIAN_POINT('Origin',(62.6,222.9,31.8213203435596)) ;
#85470=CARTESIAN_POINT('Origin',(71.6999999999999,226.1,31.8213203435596)) ;
#85471=CARTESIAN_POINT('Origin',(71.6999999999999,226.1,31.8213203435596)) ;
#85472=CARTESIAN_POINT('Origin',(71.6999999999999,226.1,31.8213203435596)) ;
#85473=CARTESIAN_POINT('Origin',(71.5999999999999,225.9,31.8213203435596)) ;
#85474=CARTESIAN_POINT('Origin',(71.3999999999999,225.9,31.8213203435596)) ;
#85475=CARTESIAN_POINT('Origin',(71.5999999999999,226.1,31.8213203435596)) ;
#85476=CARTESIAN_POINT('Origin',(71.3999999999999,232.691753592594,31.8213203435596)) ;
#85477=CARTESIAN_POINT('Origin',(62.75,226.1,31.8213203435596)) ;
#85478=CARTESIAN_POINT('Origin',(71.6999999999999,235.691753592594,31.8213203435596)) ;
#85479=CARTESIAN_POINT('Origin',(71.8999999999999,231.9,19.9213203435596)) ;
#85480=CARTESIAN_POINT('',(71.8999999999999,232.,19.9213203435596)) ;
#85481=CARTESIAN_POINT('Origin',(74.0999999999999,231.9,19.9213203435596)) ;
#85482=CARTESIAN_POINT('',(74.1999999999999,231.9,19.9213203435596)) ;
#85483=CARTESIAN_POINT('',(74.0999999999999,232.,19.9213203435596)) ;
#85484=CARTESIAN_POINT('Origin',(74.2999999999999,232.691753592594,31.8213203435596)) ;
#85485=CARTESIAN_POINT('',(74.1999999999999,232.691753592594,31.8213203435596)) ;
#85486=CARTESIAN_POINT('Origin',(74.2999999999999,226.1,19.9213203435596)) ;
#85487=CARTESIAN_POINT('',(74.2999999999999,226.,19.9213203435596)) ;
#85488=CARTESIAN_POINT('',(74.1999999999999,226.1,19.9213203435596)) ;
#85489=CARTESIAN_POINT('Origin',(74.4999999999999,223.,19.9213203435596)) ;
#85490=CARTESIAN_POINT('Origin',(74.4999999999999,226.,19.9213203435596)) ;
#85491=CARTESIAN_POINT('Origin',(58.8573593128808,241.8,25.9213203435596)) ;
#85492=CARTESIAN_POINT('',(58.9573593128808,241.8,25.9213203435596)) ;
#85493=CARTESIAN_POINT('',(58.8573593128808,241.9,25.9213203435596)) ;
#85494=CARTESIAN_POINT('Origin',(58.8573593128808,241.8,25.9213203435596)) ;
#85495=CARTESIAN_POINT('',(58.8573593128808,241.9,30.9213203435596)) ;
#85496=CARTESIAN_POINT('',(58.8573593128808,241.9,25.9213203435596)) ;
#85497=CARTESIAN_POINT('',(58.9573593128808,241.8,30.9213203435596)) ;
#85498=CARTESIAN_POINT('Origin',(58.8573593128808,241.8,30.9213203435596)) ;
#85499=CARTESIAN_POINT('',(58.9573593128808,241.8,25.9213203435596)) ;
#85500=CARTESIAN_POINT('Origin',(57.9573593128808,241.8,30.9213203435596)) ;
#85501=CARTESIAN_POINT('Origin',(57.9573593128808,241.8,31.8213203435596)) ;
#85502=CARTESIAN_POINT('Origin',(57.9573593128808,241.8,30.9213203435596)) ;
#85503=CARTESIAN_POINT('Origin',(57.9573593128808,241.9,30.9213203435596)) ;
#85504=CARTESIAN_POINT('Origin',(56.3286796564404,241.8,31.8213203435596)) ;
#85505=CARTESIAN_POINT('Origin',(58.9573593128808,241.9,25.9213203435596)) ;
#85506=CARTESIAN_POINT('',(57.9573593128808,241.9,25.9213203435596)) ;
#85507=CARTESIAN_POINT('',(57.9573593128808,241.9,25.9213203435596)) ;
#85508=CARTESIAN_POINT('',(57.9573593128808,241.9,25.9213203435596)) ;
#85509=CARTESIAN_POINT('Origin',(58.8573593128808,239.2,25.9213203435596)) ;
#85510=CARTESIAN_POINT('',(58.8573593128808,239.1,25.9213203435596)) ;
#85511=CARTESIAN_POINT('',(58.9573593128808,239.2,25.9213203435596)) ;
#85512=CARTESIAN_POINT('Origin',(58.8573593128808,239.2,25.9213203435596)) ;
#85513=CARTESIAN_POINT('',(58.9573593128808,239.2,30.9213203435596)) ;
#85514=CARTESIAN_POINT('',(58.9573593128808,239.2,25.9213203435596)) ;
#85515=CARTESIAN_POINT('',(58.8573593128808,239.1,30.9213203435596)) ;
#85516=CARTESIAN_POINT('Origin',(58.8573593128808,239.2,30.9213203435596)) ;
#85517=CARTESIAN_POINT('',(58.8573593128808,239.1,25.9213203435596)) ;
#85518=CARTESIAN_POINT('Origin',(57.9573593128808,239.2,30.9213203435596)) ;
#85519=CARTESIAN_POINT('Origin',(57.9573593128808,239.2,31.8213203435596)) ;
#85520=CARTESIAN_POINT('Origin',(57.9573593128808,239.1,30.9213203435596)) ;
#85521=CARTESIAN_POINT('Origin',(57.9573593128808,239.2,30.9213203435596)) ;
#85522=CARTESIAN_POINT('Origin',(55.8286796564404,239.2,31.8213203435596)) ;
#85523=CARTESIAN_POINT('Origin',(57.9573593128808,239.241753592594,30.9213203435596)) ;
#85524=CARTESIAN_POINT('',(58.9573593128808,239.241753592594,30.9213203435596)) ;
#85525=CARTESIAN_POINT('Origin',(58.9573593128808,239.1,25.9213203435596)) ;
#85526=CARTESIAN_POINT('',(58.9573593128808,241.9,25.9213203435596)) ;
#85527=CARTESIAN_POINT('Origin',(62.1159379566435,238.1,31.8213203435596)) ;
#85528=CARTESIAN_POINT('Origin',(62.1159379566435,237.9,31.8213203435596)) ;
#85529=CARTESIAN_POINT('Origin',(62.2573593128808,237.958578643763,31.8213203435596)) ;
#85530=CARTESIAN_POINT('Origin',(55.8286796564404,237.9,31.8213203435596)) ;
#85531=CARTESIAN_POINT('Origin',(62.8573593128808,238.841421356237,31.8213203435596)) ;
#85532=CARTESIAN_POINT('Origin',(62.998780669118,238.7,31.8213203435596)) ;
#85533=CARTESIAN_POINT('Origin',(63.0573593128807,238.841421356237,31.8213203435596)) ;
#85534=CARTESIAN_POINT('Origin',(60.6596069590762,236.360826289958,31.8213203435596)) ;
#85535=CARTESIAN_POINT('Origin',(62.8573593128808,242.158578643763,31.8213203435596)) ;
#85536=CARTESIAN_POINT('Origin',(63.0573593128807,242.158578643763,31.8213203435596)) ;
#85537=CARTESIAN_POINT('Origin',(62.9987806691181,242.3,31.8213203435596)) ;
#85538=CARTESIAN_POINT('Origin',(63.0573593128807,238.691753592594,31.8213203435596)) ;
#85539=CARTESIAN_POINT('Origin',(62.1159379566435,242.9,31.8213203435596)) ;
#85540=CARTESIAN_POINT('Origin',(62.2573593128808,243.041421356237,31.8213203435596)) ;
#85541=CARTESIAN_POINT('Origin',(62.1159379566435,243.1,31.8213203435596)) ;
#85542=CARTESIAN_POINT('Origin',(61.2178533664821,244.080927302636,31.8213203435596)) ;
#85543=CARTESIAN_POINT('Origin',(58.3286796564404,243.1,31.8213203435596)) ;
#85544=CARTESIAN_POINT('Origin',(79.2999999999999,252.3,25.9213203435596)) ;
#85545=CARTESIAN_POINT('',(79.2999999999999,252.4,25.9213203435596)) ;
#85546=CARTESIAN_POINT('',(79.1999999999999,252.3,25.9213203435596)) ;
#85547=CARTESIAN_POINT('Origin',(79.2999999999999,252.3,25.9213203435596)) ;
#85548=CARTESIAN_POINT('',(79.1999999999999,252.3,30.9213203435596)) ;
#85549=CARTESIAN_POINT('',(79.1999999999999,252.3,25.9213203435596)) ;
#85550=CARTESIAN_POINT('',(79.2999999999999,252.4,30.9213203435596)) ;
#85551=CARTESIAN_POINT('Origin',(79.2999999999999,252.3,30.9213203435596)) ;
#85552=CARTESIAN_POINT('',(79.2999999999999,252.4,25.9213203435596)) ;
#85553=CARTESIAN_POINT('Origin',(80.1999999999999,252.3,30.9213203435596)) ;
#85554=CARTESIAN_POINT('Origin',(80.1999999999999,252.3,31.8213203435596)) ;
#85555=CARTESIAN_POINT('Origin',(80.1999999999999,252.4,30.9213203435596)) ;
#85556=CARTESIAN_POINT('Origin',(80.1999999999999,252.3,30.9213203435596)) ;
#85557=CARTESIAN_POINT('Origin',(66.9499999999999,252.3,31.8213203435596)) ;
#85558=CARTESIAN_POINT('Origin',(80.299999999999,252.3,31.8213203435596)) ;
#85559=CARTESIAN_POINT('Origin',(80.1999999999999,245.891753592594,30.9213203435596)) ;
#85560=CARTESIAN_POINT('',(79.1999999999999,249.7,30.9213203435596)) ;
#85561=CARTESIAN_POINT('',(79.1999999999999,245.891753592594,30.9213203435596)) ;
#85562=CARTESIAN_POINT('Origin',(80.1999999999999,249.7,30.9213203435596)) ;
#85563=CARTESIAN_POINT('Origin',(79.1999999999999,252.4,25.9213203435596)) ;
#85564=CARTESIAN_POINT('',(79.1999999999999,249.7,25.9213203435596)) ;
#85565=CARTESIAN_POINT('',(79.1999999999999,249.6,25.9213203435596)) ;
#85566=CARTESIAN_POINT('',(79.1999999999999,249.7,25.9213203435596)) ;
#85567=CARTESIAN_POINT('Origin',(79.6999999999999,251.,25.9213203435596)) ;
#85568=CARTESIAN_POINT('',(80.1999999999999,252.4,25.9213203435596)) ;
#85569=CARTESIAN_POINT('',(79.1999999999999,252.4,25.9213203435596)) ;
#85570=CARTESIAN_POINT('',(80.1999999999999,249.6,25.9213203435596)) ;
#85571=CARTESIAN_POINT('',(80.1999999999999,252.4,25.9213203435596)) ;
#85572=CARTESIAN_POINT('',(79.2999999999999,249.6,25.9213203435596)) ;
#85573=CARTESIAN_POINT('',(80.1999999999999,249.6,25.9213203435596)) ;
#85574=CARTESIAN_POINT('Origin',(79.2999999999999,249.7,25.9213203435596)) ;
#85575=CARTESIAN_POINT('Origin',(79.2999999999999,249.7,25.9213203435596)) ;
#85576=CARTESIAN_POINT('',(79.2999999999999,249.6,30.9213203435596)) ;
#85577=CARTESIAN_POINT('',(79.2999999999999,249.6,25.9213203435596)) ;
#85578=CARTESIAN_POINT('Origin',(79.2999999999999,249.7,30.9213203435596)) ;
#85579=CARTESIAN_POINT('Origin',(80.1999999999999,249.7,30.9213203435596)) ;
#85580=CARTESIAN_POINT('',(80.199999999999,249.6,31.8213203435596)) ;
#85581=CARTESIAN_POINT('Origin',(80.199999999999,249.7,31.8213203435596)) ;
#85582=CARTESIAN_POINT('Origin',(80.1999999999999,249.6,30.9213203435596)) ;
#85583=CARTESIAN_POINT('Origin',(66.4500000000001,249.700000000001,31.8213203435596)) ;
#85584=CARTESIAN_POINT('Origin',(80.2999999999989,249.7,31.8213203435596)) ;
#85585=CARTESIAN_POINT('Origin',(79.1999999999999,249.6,25.9213203435596)) ;
#85586=CARTESIAN_POINT('',(80.1999999999999,249.6,25.9213203435596)) ;
#85587=CARTESIAN_POINT('',(80.199999999999,249.6,22.9213203435596)) ;
#85588=CARTESIAN_POINT('Origin',(76.0414213562365,248.6,31.8213203435596)) ;
#85589=CARTESIAN_POINT('',(75.9707106781179,248.529289321881,31.8213203435596)) ;
#85590=CARTESIAN_POINT('',(76.0414213562365,248.5,31.8213203435596)) ;
#85591=CARTESIAN_POINT('Origin',(76.0414213562365,248.6,31.8213203435596)) ;
#85592=CARTESIAN_POINT('Origin',(75.8999999999992,248.458578643763,31.8213203435596)) ;
#85593=CARTESIAN_POINT('Origin',(76.0414213562365,248.4,31.8213203435596)) ;
#85594=CARTESIAN_POINT('Origin',(75.2999999999993,249.341421356237,31.8213203435596)) ;
#85595=CARTESIAN_POINT('',(75.1999999999993,249.341421356237,31.8213203435596)) ;
#85596=CARTESIAN_POINT('',(75.2292893218807,249.270710678119,31.8213203435596)) ;
#85597=CARTESIAN_POINT('Origin',(75.2999999999993,249.341421356237,31.8213203435596)) ;
#85598=CARTESIAN_POINT('Origin',(75.0999999999993,249.341421356237,31.8213203435596)) ;
#85599=CARTESIAN_POINT('Origin',(75.158578643762,249.2,31.8213203435596)) ;
#85600=CARTESIAN_POINT('Origin',(75.2999999999994,252.658578643763,31.8213203435596)) ;
#85601=CARTESIAN_POINT('',(75.2292893218808,252.729289321881,31.8213203435596)) ;
#85602=CARTESIAN_POINT('',(75.1999999999994,252.658578643763,31.8213203435596)) ;
#85603=CARTESIAN_POINT('Origin',(75.2999999999994,252.658578643763,31.8213203435596)) ;
#85604=CARTESIAN_POINT('Origin',(75.1585786437621,252.8,31.8213203435596)) ;
#85605=CARTESIAN_POINT('Origin',(75.0999999999994,252.658578643763,31.8213203435596)) ;
#85606=CARTESIAN_POINT('Origin',(76.0414213562367,253.4,31.8213203435596)) ;
#85607=CARTESIAN_POINT('',(76.0414213562367,253.5,31.8213203435596)) ;
#85608=CARTESIAN_POINT('',(75.9707106781181,253.470710678119,31.8213203435596)) ;
#85609=CARTESIAN_POINT('Origin',(76.0414213562367,253.4,31.8213203435596)) ;
#85610=CARTESIAN_POINT('Origin',(76.0414213562367,253.6,31.8213203435596)) ;
#85611=CARTESIAN_POINT('Origin',(75.8999999999994,253.541421356237,31.8213203435596)) ;
#85612=CARTESIAN_POINT('Origin',(66.9499999999995,253.6,31.8213203435596)) ;
#85613=CARTESIAN_POINT('',(66.9499999999995,253.5,31.8213203435596)) ;
#85614=CARTESIAN_POINT('Origin',(80.2999999999989,243.941753592594,31.8213203435596)) ;
#85615=CARTESIAN_POINT('Origin',(66.6251661181778,244.266587474416,31.8213203435596)) ;
#85616=CARTESIAN_POINT('',(66.6958767962964,244.195876796297,31.8213203435596)) ;
#85617=CARTESIAN_POINT('Origin',(76.0414213562367,253.4,19.9213203435596)) ;
#85618=CARTESIAN_POINT('',(76.0414213562367,253.5,19.9213203435596)) ;
#85619=CARTESIAN_POINT('',(75.9707106781181,253.470710678119,19.9213203435596)) ;
#85620=CARTESIAN_POINT('Origin',(75.0999999999992,246.441753592594,31.8213203435596)) ;
#85621=CARTESIAN_POINT('',(75.1999999999992,246.441753592594,31.8213203435596)) ;
#85622=CARTESIAN_POINT('Origin',(75.2999999999994,252.658578643763,19.9213203435596)) ;
#85623=CARTESIAN_POINT('',(75.2292893218808,252.729289321881,19.9213203435596)) ;
#85624=CARTESIAN_POINT('',(75.1999999999994,252.658578643763,19.9213203435596)) ;
#85625=CARTESIAN_POINT('Origin',(72.4334125255833,251.925166118179,31.8213203435596)) ;
#85626=CARTESIAN_POINT('',(72.504123203702,251.995876796297,31.8213203435596)) ;
#85627=CARTESIAN_POINT('Origin',(75.2999999999993,249.341421356237,19.9213203435596)) ;
#85628=CARTESIAN_POINT('',(75.1999999999993,249.341421356237,19.9213203435596)) ;
#85629=CARTESIAN_POINT('',(75.2292893218807,249.270710678119,19.9213203435596)) ;
#85630=CARTESIAN_POINT('Origin',(64.4499999999996,248.4,31.8213203435596)) ;
#85631=CARTESIAN_POINT('',(64.4499999999996,248.5,31.8213203435596)) ;
#85632=CARTESIAN_POINT('Origin',(76.0414213562365,248.6,19.9213203435596)) ;
#85633=CARTESIAN_POINT('',(75.9707106781179,248.529289321881,19.9213203435596)) ;
#85634=CARTESIAN_POINT('',(76.0414213562365,248.5,19.9213203435596)) ;
#85635=CARTESIAN_POINT('Origin',(80.2999999999989,243.941753592594,31.8213203435596)) ;
#85636=CARTESIAN_POINT('',(80.1999999999989,243.941753592594,31.8213203435596)) ;
#85637=CARTESIAN_POINT('Origin',(75.5999999999994,253.1,19.9213203435596)) ;
#85638=CARTESIAN_POINT('Origin',(75.1999999999994,253.5,19.9213203435596)) ;
#85639=CARTESIAN_POINT('Origin',(75.5999999999993,248.9,19.9213203435596)) ;
#85640=CARTESIAN_POINT('Origin',(75.1999999999993,248.5,19.9213203435596)) ;
#85641=CARTESIAN_POINT('Origin',(80.199999999999,248.5,19.9213203435596)) ;
#85642=CARTESIAN_POINT('Origin',(64.3,245.191753592594,30.8213203435596)) ;
#85643=CARTESIAN_POINT('',(64.3999999999999,245.191753592594,30.8213203435596)) ;
#85644=CARTESIAN_POINT('Origin',(64.3999999999999,251.,19.9213203435596)) ;
#85645=CARTESIAN_POINT('Origin',(56.3,245.191753592594,30.8213203435596)) ;
#85646=CARTESIAN_POINT('',(56.3999999999999,245.191753592594,30.8213203435596)) ;
#85647=CARTESIAN_POINT('Origin',(56.3999999999999,251.,19.9213203435596)) ;
#85648=CARTESIAN_POINT('Origin',(43.0999999999999,252.1,31.8213203435596)) ;
#85649=CARTESIAN_POINT('',(43.1999999999999,252.1,31.8213203435596)) ;
#85650=CARTESIAN_POINT('Origin',(43.2999999999999,252.1,31.8213203435596)) ;
#85651=CARTESIAN_POINT('',(43.0999999999999,252.,31.8213203435596)) ;
#85652=CARTESIAN_POINT('Origin',(43.0999999999999,252.1,31.8213203435596)) ;
#85653=CARTESIAN_POINT('Origin',(43.0999999999999,251.9,31.8213203435596)) ;
#85654=CARTESIAN_POINT('Origin',(43.0999999999999,252.1,30.8213203435596)) ;
#85655=CARTESIAN_POINT('',(43.1999999999999,252.1,30.8213203435596)) ;
#85656=CARTESIAN_POINT('',(43.0999999999999,252.,30.8213203435596)) ;
#85657=CARTESIAN_POINT('Origin',(43.0999999999999,252.1,30.8213203435596)) ;
#85658=CARTESIAN_POINT('Origin',(43.2999999999999,252.1,30.8213203435596)) ;
#85659=CARTESIAN_POINT('Origin',(43.0999999999999,251.9,30.8213203435596)) ;
#85660=CARTESIAN_POINT('Origin',(43.0999999999999,259.9,31.8213203435596)) ;
#85661=CARTESIAN_POINT('',(43.0999999999999,260.,31.8213203435596)) ;
#85662=CARTESIAN_POINT('Origin',(43.0999999999999,260.1,31.8213203435596)) ;
#85663=CARTESIAN_POINT('',(43.1999999999999,259.9,31.8213203435596)) ;
#85664=CARTESIAN_POINT('Origin',(43.0999999999999,259.9,31.8213203435596)) ;
#85665=CARTESIAN_POINT('Origin',(43.2999999999999,259.9,31.8213203435596)) ;
#85666=CARTESIAN_POINT('Origin',(37.2999999999999,252.1,31.8213203435596)) ;
#85667=CARTESIAN_POINT('',(37.1999999999999,252.1,31.8213203435596)) ;
#85668=CARTESIAN_POINT('',(37.2999999999999,252.,31.8213203435596)) ;
#85669=CARTESIAN_POINT('Origin',(37.2999999999999,252.1,31.8213203435596)) ;
#85670=CARTESIAN_POINT('Origin',(37.0999999999999,252.1,31.8213203435596)) ;
#85671=CARTESIAN_POINT('Origin',(37.2999999999999,251.9,31.8213203435596)) ;
#85672=CARTESIAN_POINT('Origin',(37.2999999999999,252.1,30.8213203435596)) ;
#85673=CARTESIAN_POINT('',(37.1999999999999,252.1,30.8213203435596)) ;
#85674=CARTESIAN_POINT('Origin',(37.0999999999999,252.1,30.8213203435596)) ;
#85675=CARTESIAN_POINT('',(37.2999999999999,252.,30.8213203435596)) ;
#85676=CARTESIAN_POINT('Origin',(37.2999999999999,252.1,30.8213203435596)) ;
#85677=CARTESIAN_POINT('Origin',(37.2999999999999,251.9,30.8213203435596)) ;
#85678=CARTESIAN_POINT('Origin',(43.0999999999999,259.9,30.8213203435596)) ;
#85679=CARTESIAN_POINT('',(43.0999999999999,260.,30.8213203435596)) ;
#85680=CARTESIAN_POINT('',(43.1999999999999,259.9,30.8213203435596)) ;
#85681=CARTESIAN_POINT('Origin',(43.0999999999999,259.9,30.8213203435596)) ;
#85682=CARTESIAN_POINT('Origin',(43.0999999999999,260.1,30.8213203435596)) ;
#85683=CARTESIAN_POINT('Origin',(43.2999999999999,259.9,30.8213203435596)) ;
#85684=CARTESIAN_POINT('Origin',(37.2999999999999,259.9,31.8213203435596)) ;
#85685=CARTESIAN_POINT('',(37.1999999999999,259.9,31.8213203435596)) ;
#85686=CARTESIAN_POINT('Origin',(37.0999999999999,259.9,31.8213203435596)) ;
#85687=CARTESIAN_POINT('',(37.2999999999999,260.,31.8213203435596)) ;
#85688=CARTESIAN_POINT('Origin',(37.2999999999999,259.9,31.8213203435596)) ;
#85689=CARTESIAN_POINT('Origin',(37.2999999999999,260.1,31.8213203435596)) ;
#85690=CARTESIAN_POINT('Origin',(37.0999999999999,249.691753592594,31.8213203435596)) ;
#85691=CARTESIAN_POINT('',(37.1999999999999,249.691753592594,31.8213203435596)) ;
#85692=CARTESIAN_POINT('Origin',(37.2999999999999,259.9,30.8213203435596)) ;
#85693=CARTESIAN_POINT('',(37.1999999999999,259.9,30.8213203435596)) ;
#85694=CARTESIAN_POINT('',(37.2999999999999,260.,30.8213203435596)) ;
#85695=CARTESIAN_POINT('Origin',(37.2999999999999,259.9,30.8213203435596)) ;
#85696=CARTESIAN_POINT('Origin',(37.0999999999999,259.9,30.8213203435596)) ;
#85697=CARTESIAN_POINT('Origin',(37.2999999999999,260.1,30.8213203435596)) ;
#85698=CARTESIAN_POINT('Origin',(37.0999999999999,249.691753592594,30.8213203435596)) ;
#85699=CARTESIAN_POINT('',(37.1999999999999,249.691753592594,30.8213203435596)) ;
#85700=CARTESIAN_POINT('Origin',(48.4499999999999,260.1,30.8213203435596)) ;
#85701=CARTESIAN_POINT('',(48.4499999999999,260.,30.8213203435596)) ;
#85702=CARTESIAN_POINT('Origin',(37.2999999999999,259.9,19.9213203435596)) ;
#85703=CARTESIAN_POINT('',(37.1999999999999,259.9,19.9213203435596)) ;
#85704=CARTESIAN_POINT('',(37.2999999999999,260.,19.9213203435596)) ;
#85705=CARTESIAN_POINT('Origin',(48.4499999999999,260.1,31.8213203435596)) ;
#85706=CARTESIAN_POINT('',(48.4499999999999,260.,31.8213203435596)) ;
#85707=CARTESIAN_POINT('Origin',(43.2999999999999,245.691753592594,30.8213203435596)) ;
#85708=CARTESIAN_POINT('',(43.1999999999999,245.691753592594,30.8213203435596)) ;
#85709=CARTESIAN_POINT('Origin',(43.0999999999999,259.9,19.9213203435596)) ;
#85710=CARTESIAN_POINT('',(43.0999999999999,260.,19.9213203435596)) ;
#85711=CARTESIAN_POINT('',(43.1999999999999,259.9,19.9213203435596)) ;
#85712=CARTESIAN_POINT('Origin',(37.2999999999999,252.1,19.9213203435596)) ;
#85713=CARTESIAN_POINT('',(37.2999999999999,252.,19.9213203435596)) ;
#85714=CARTESIAN_POINT('',(37.1999999999999,252.1,19.9213203435596)) ;
#85715=CARTESIAN_POINT('Origin',(45.4499999999999,251.9,30.8213203435596)) ;
#85716=CARTESIAN_POINT('',(45.4499999999999,252.,30.8213203435596)) ;
#85717=CARTESIAN_POINT('Origin',(45.4499999999999,251.9,31.8213203435596)) ;
#85718=CARTESIAN_POINT('',(45.4499999999999,252.,31.8213203435596)) ;
#85719=CARTESIAN_POINT('Origin',(43.2999999999999,245.691753592594,31.8213203435596)) ;
#85720=CARTESIAN_POINT('',(43.1999999999999,245.691753592594,31.8213203435596)) ;
#85721=CARTESIAN_POINT('Origin',(43.0999999999999,252.1,19.9213203435596)) ;
#85722=CARTESIAN_POINT('',(43.1999999999999,252.1,19.9213203435596)) ;
#85723=CARTESIAN_POINT('',(43.0999999999999,252.,19.9213203435596)) ;
#85724=CARTESIAN_POINT('Origin',(37.1999999999999,260.,19.9213203435596)) ;
#85725=CARTESIAN_POINT('Origin',(43.1999999999999,260.,19.9213203435596)) ;
#85726=CARTESIAN_POINT('Origin',(43.1999999999999,252.,19.9213203435596)) ;
#85727=CARTESIAN_POINT('Origin',(37.1999999999999,252.,19.9213203435596)) ;
#85728=CARTESIAN_POINT('Origin',(30.7,254.8,30.8213203435596)) ;
#85729=CARTESIAN_POINT('',(28.1999999999999,254.8,30.8213203435596)) ;
#85730=CARTESIAN_POINT('Origin',(28.1,254.8,30.8213203435596)) ;
#85731=CARTESIAN_POINT('Origin',(30.7,254.8,30.8213203435596)) ;
#85732=CARTESIAN_POINT('Origin',(30.7,254.8,19.9213203435596)) ;
#85733=CARTESIAN_POINT('',(28.2,254.8,31.8213203435596)) ;
#85734=CARTESIAN_POINT('',(28.2,254.8,19.9213203435596)) ;
#85735=CARTESIAN_POINT('',(33.1999999999999,254.8,31.8213203435596)) ;
#85736=CARTESIAN_POINT('Origin',(30.6999999999999,254.8,31.8213203435596)) ;
#85737=CARTESIAN_POINT('Origin',(30.6999999999999,254.8,31.8213203435596)) ;
#85738=CARTESIAN_POINT('Origin',(30.6999999999999,254.8,31.8213203435596)) ;
#85739=CARTESIAN_POINT('Origin',(33.2999999999999,254.8,31.8213203435596)) ;
#85740=CARTESIAN_POINT('Origin',(29.1,262.2,25.9213203435596)) ;
#85741=CARTESIAN_POINT('',(29.1999999999999,262.2,25.9213203435596)) ;
#85742=CARTESIAN_POINT('',(29.1,262.3,25.9213203435596)) ;
#85743=CARTESIAN_POINT('Origin',(29.1,262.2,25.9213203435596)) ;
#85744=CARTESIAN_POINT('',(29.1,262.3,30.9213203435596)) ;
#85745=CARTESIAN_POINT('',(29.1,262.3,25.9213203435596)) ;
#85746=CARTESIAN_POINT('',(29.1999999999999,262.2,30.9213203435596)) ;
#85747=CARTESIAN_POINT('Origin',(29.1,262.2,30.9213203435596)) ;
#85748=CARTESIAN_POINT('',(29.1999999999999,262.2,25.9213203435596)) ;
#85749=CARTESIAN_POINT('Origin',(28.1999999999999,262.2,30.9213203435596)) ;
#85750=CARTESIAN_POINT('Origin',(28.2,262.2,31.8213203435596)) ;
#85751=CARTESIAN_POINT('Origin',(28.1999999999999,262.2,30.9213203435596)) ;
#85752=CARTESIAN_POINT('Origin',(28.1999999999999,262.3,30.9213203435596)) ;
#85753=CARTESIAN_POINT('Origin',(41.45,262.2,31.8213203435596)) ;
#85754=CARTESIAN_POINT('Origin',(28.1,262.2,31.8213203435596)) ;
#85755=CARTESIAN_POINT('Origin',(29.1999999999999,262.3,25.9213203435596)) ;
#85756=CARTESIAN_POINT('',(28.2,262.3,25.9213203435596)) ;
#85757=CARTESIAN_POINT('',(28.2,262.3,25.9213203435596)) ;
#85758=CARTESIAN_POINT('',(28.2,262.3,25.9213203435596)) ;
#85759=CARTESIAN_POINT('Origin',(28.7,260.9,25.9213203435596)) ;
#85760=CARTESIAN_POINT('',(29.1999999999999,259.6,25.9213203435596)) ;
#85761=CARTESIAN_POINT('',(29.1999999999999,262.3,25.9213203435596)) ;
#85762=CARTESIAN_POINT('',(29.1,259.5,25.9213203435596)) ;
#85763=CARTESIAN_POINT('Origin',(29.1,259.6,25.9213203435596)) ;
#85764=CARTESIAN_POINT('',(28.2,259.5,25.9213203435596)) ;
#85765=CARTESIAN_POINT('',(29.1999999999999,259.5,25.9213203435596)) ;
#85766=CARTESIAN_POINT('',(28.2,259.5,25.9213203435596)) ;
#85767=CARTESIAN_POINT('Origin',(29.1999999999999,259.5,25.9213203435596)) ;
#85768=CARTESIAN_POINT('',(29.1999999999999,259.6,30.9213203435596)) ;
#85769=CARTESIAN_POINT('',(29.1999999999999,249.441753592594,30.9213203435596)) ;
#85770=CARTESIAN_POINT('',(29.1999999999999,259.6,25.9213203435596)) ;
#85771=CARTESIAN_POINT('Origin',(29.1,259.6,25.9213203435596)) ;
#85772=CARTESIAN_POINT('',(29.1,259.5,30.9213203435596)) ;
#85773=CARTESIAN_POINT('Origin',(29.1,259.6,30.9213203435596)) ;
#85774=CARTESIAN_POINT('',(29.1,259.5,25.9213203435596)) ;
#85775=CARTESIAN_POINT('Origin',(28.1999999999999,259.6,30.9213203435596)) ;
#85776=CARTESIAN_POINT('',(28.2,259.5,31.8213203435596)) ;
#85777=CARTESIAN_POINT('Origin',(28.1999999999999,259.6,31.8213203435596)) ;
#85778=CARTESIAN_POINT('Origin',(28.2,259.5,30.9213203435596)) ;
#85779=CARTESIAN_POINT('Origin',(28.1999999999999,259.6,30.9213203435596)) ;
#85780=CARTESIAN_POINT('Origin',(40.9499999999996,259.6,31.8213203435596)) ;
#85781=CARTESIAN_POINT('Origin',(28.0999999999999,259.6,31.8213203435596)) ;
#85782=CARTESIAN_POINT('Origin',(28.1999999999999,249.441753592594,30.9213203435596)) ;
#85783=CARTESIAN_POINT('Origin',(32.3585786437627,258.5,31.8213203435596)) ;
#85784=CARTESIAN_POINT('Origin',(32.3585786437627,258.3,31.8213203435596)) ;
#85785=CARTESIAN_POINT('Origin',(32.5,258.358578643763,31.8213203435596)) ;
#85786=CARTESIAN_POINT('Origin',(40.95,258.3,31.8213203435596)) ;
#85787=CARTESIAN_POINT('Origin',(28.1,258.3,31.8213203435596)) ;
#85788=CARTESIAN_POINT('Origin',(33.1,259.241421356237,31.8213203435596)) ;
#85789=CARTESIAN_POINT('Origin',(33.2414213562373,259.1,31.8213203435596)) ;
#85790=CARTESIAN_POINT('Origin',(33.2999999999999,259.241421356237,31.8213203435596)) ;
#85791=CARTESIAN_POINT('Origin',(33.2415874744158,259.100166118179,31.8213203435596)) ;
#85792=CARTESIAN_POINT('Origin',(33.1,262.558578643763,31.8213203435596)) ;
#85793=CARTESIAN_POINT('Origin',(33.2999999999999,262.558578643763,31.8213203435596)) ;
#85794=CARTESIAN_POINT('Origin',(33.2414213562373,262.7,31.8213203435596)) ;
#85795=CARTESIAN_POINT('Origin',(33.2999999999999,248.891753592594,31.8213203435596)) ;
#85796=CARTESIAN_POINT('Origin',(32.3585786437627,263.3,31.8213203435596)) ;
#85797=CARTESIAN_POINT('Origin',(32.5,263.441421356237,31.8213203435596)) ;
#85798=CARTESIAN_POINT('Origin',(32.3585786437627,263.5,31.8213203435596)) ;
#85799=CARTESIAN_POINT('Origin',(43.9998338818216,251.941587474416,31.8213203435596)) ;
#85800=CARTESIAN_POINT('Origin',(28.2999999999999,263.3,31.8213203435596)) ;
#85801=CARTESIAN_POINT('Origin',(28.2999999999999,263.5,31.8213203435596)) ;
#85802=CARTESIAN_POINT('Origin',(28.1,263.3,31.8213203435596)) ;
#85803=CARTESIAN_POINT('Origin',(43.45,263.5,31.8213203435596)) ;
#85804=CARTESIAN_POINT('Origin',(28.1,251.391753592594,31.8213203435596)) ;
#85805=CARTESIAN_POINT('Origin',(28.1,251.391753592594,31.8213203435596)) ;
#85806=CARTESIAN_POINT('',(28.1999999999999,251.391753592594,31.8213203435596)) ;
#85807=CARTESIAN_POINT('Origin',(61.5,261.2,31.8213203435596)) ;
#85808=CARTESIAN_POINT('',(64.,261.2,31.8213203435596)) ;
#85809=CARTESIAN_POINT('Origin',(64.1,261.2,31.8213203435596)) ;
#85810=CARTESIAN_POINT('',(59.,261.2,31.8213203435596)) ;
#85811=CARTESIAN_POINT('Origin',(61.5,261.2,31.8213203435596)) ;
#85812=CARTESIAN_POINT('Origin',(61.5,261.2,31.8213203435596)) ;
#85813=CARTESIAN_POINT('Origin',(61.5,261.2,19.9213203435596)) ;
#85814=CARTESIAN_POINT('',(59.,261.2,19.9213203435596)) ;
#85815=CARTESIAN_POINT('Origin',(64.1568347953873,220.146231446812,31.8213203435596)) ;
#85816=CARTESIAN_POINT('',(66.1568347953873,220.146231446812,31.8213203435596)) ;
#85817=CARTESIAN_POINT('Origin',(66.2568347953873,220.146231446812,31.8213203435596)) ;
#85818=CARTESIAN_POINT('',(62.1568347953873,220.146231446812,31.8213203435596)) ;
#85819=CARTESIAN_POINT('Origin',(64.1568347953873,220.146231446812,31.8213203435596)) ;
#85820=CARTESIAN_POINT('Origin',(64.1568347953873,220.146231446812,31.8213203435596)) ;
#85821=CARTESIAN_POINT('Origin',(64.1568347953873,220.146231446812,19.9213203435596)) ;
#85822=CARTESIAN_POINT('',(62.1568347953873,220.146231446812,19.9213203435596)) ;
#85823=CARTESIAN_POINT('Origin',(79.0999999999999,249.391753592594,30.8213203435596)) ;
#85824=CARTESIAN_POINT('Origin',(79.0999999999999,259.648528137424,30.8213203435596)) ;
#85825=CARTESIAN_POINT('Origin',(79.7999999999999,259.648528137424,30.8213203435596)) ;
#85826=CARTESIAN_POINT('Origin',(79.3050252531694,259.153553390593,30.8213203435596)) ;
#85827=CARTESIAN_POINT('Origin',(79.7999999999999,259.648528137424,30.8213203435596)) ;
#85828=CARTESIAN_POINT('Origin',(78.758412525583,259.70016611818,30.8213203435596)) ;
#85829=CARTESIAN_POINT('Origin',(80.9535533905932,257.50502525317,30.8213203435596)) ;
#85830=CARTESIAN_POINT('Origin',(80.6,257.151471862576,30.8213203435596)) ;
#85831=CARTESIAN_POINT('Origin',(81.1,257.151471862576,30.8213203435596)) ;
#85832=CARTESIAN_POINT('Origin',(81.1,242.941753592594,30.8213203435596)) ;
#85833=CARTESIAN_POINT('Origin',(81.1,247.098386676966,30.8213203435596)) ;
#85834=CARTESIAN_POINT('Origin',(80.6,247.098386676966,30.8213203435596)) ;
#85835=CARTESIAN_POINT('Origin',(80.616129032258,246.598646890358,30.8213203435596)) ;
#85836=CARTESIAN_POINT('Origin',(80.6999999999999,244.,30.8213203435596)) ;
#85837=CARTESIAN_POINT('Origin',(78.0999999999999,244.,30.8213203435596)) ;
#85838=CARTESIAN_POINT('Origin',(78.1,239.691753592594,30.8213203435596)) ;
#85839=CARTESIAN_POINT('Origin',(78.1,240.,30.8213203435596)) ;
#85840=CARTESIAN_POINT('Origin',(80.6999999999999,240.,30.8213203435596)) ;
#85841=CARTESIAN_POINT('Origin',(80.616129032258,237.401353109641,30.8213203435596)) ;
#85842=CARTESIAN_POINT('Origin',(80.6,236.901613323034,30.8213203435596)) ;
#85843=CARTESIAN_POINT('Origin',(81.1,236.901613323034,30.8213203435596)) ;
#85844=CARTESIAN_POINT('Origin',(81.1,232.568672279644,30.8213203435596)) ;
#85845=CARTESIAN_POINT('Origin',(81.1,226.002365511524,30.8213203435596)) ;
#85846=CARTESIAN_POINT('Origin',(80.6,226.002365511524,30.8213203435596)) ;
#85847=CARTESIAN_POINT('Origin',(80.9535533905933,225.64881212093,30.8213203435596)) ;
#85848=CARTESIAN_POINT('Origin',(77.061706774654,221.756965504991,30.8213203435596)) ;
#85849=CARTESIAN_POINT('Origin',(80.1050252531695,224.800283983507,30.8213203435596)) ;
#85850=CARTESIAN_POINT('Origin',(80.6000000000001,224.305309236676,30.8213203435596)) ;
#85851=CARTESIAN_POINT('Origin',(79.9000000000001,224.305309236676,30.8213203435596)) ;
#85852=CARTESIAN_POINT('Origin',(79.9,228.575260777783,30.8213203435596)) ;
#85853=CARTESIAN_POINT('Origin',(79.9000000000001,217.767014370377,30.8213203435596)) ;
#85854=CARTESIAN_POINT('Origin',(76.0000000000001,217.767014370377,30.8213203435596)) ;
#85855=CARTESIAN_POINT('Origin',(75.3227721070991,213.926264133629,30.8213203435596)) ;
#85856=CARTESIAN_POINT('Origin',(56.086380506565,217.318158984277,30.8213203435596)) ;
#85857=CARTESIAN_POINT('Origin',(63.8058825236653,215.957002501029,30.8213203435596)) ;
#85858=CARTESIAN_POINT('Origin',(64.4831104165663,219.797752737776,30.8213203435596)) ;
#85859=CARTESIAN_POINT('Origin',(61.2884174438392,217.560804636007,30.8213203435596)) ;
#85860=CARTESIAN_POINT('Origin',(52.288931387286,230.413402709377,30.8213203435596)) ;
#85861=CARTESIAN_POINT('Origin',(56.7626663401537,224.024247053747,30.8213203435596)) ;
#85862=CARTESIAN_POINT('Origin',(59.9573593128808,226.261195155516,30.8213203435596)) ;
#85863=CARTESIAN_POINT('Origin',(56.0573593128808,226.261195155516,30.8213203435596)) ;
#85864=CARTESIAN_POINT('Origin',(56.0573593128807,242.191753592594,30.8213203435596)) ;
#85865=CARTESIAN_POINT('Origin',(56.0573593128807,244.4,30.8213203435596)) ;
#85866=CARTESIAN_POINT('Origin',(55.3573593128808,244.4,30.8213203435596)) ;
#85867=CARTESIAN_POINT('Origin',(55.3573593128808,245.1,30.8213203435596)) ;
#85868=CARTESIAN_POINT('Origin',(39.95,245.1,30.8213203435596)) ;
#85869=CARTESIAN_POINT('Origin',(46.8,245.1,30.8213203435596)) ;
#85870=CARTESIAN_POINT('Origin',(46.8,245.6,30.8213203435596)) ;
#85871=CARTESIAN_POINT('Origin',(79.7999999999999,259.648528137424,19.9213203435596)) ;
#85872=CARTESIAN_POINT('Origin',(26.8,245.6,30.8213203435596)) ;
#85873=CARTESIAN_POINT('',(26.8,245.,30.8213203435596)) ;
#85874=CARTESIAN_POINT('Origin',(26.8,245.1,30.8213203435596)) ;
#85875=CARTESIAN_POINT('Origin',(26.8,245.6,30.8213203435596)) ;
#85876=CARTESIAN_POINT('Origin',(39.95,245.1,30.8213203435596)) ;
#85877=CARTESIAN_POINT('',(33.6,245.,30.8213203435596)) ;
#85878=CARTESIAN_POINT('Origin',(33.6,245.1,30.8213203435596)) ;
#85879=CARTESIAN_POINT('',(39.95,245.,30.8213203435596)) ;
#85880=CARTESIAN_POINT('Origin',(33.6,245.6,30.8213203435596)) ;
#85881=CARTESIAN_POINT('',(34.2,245.6,30.8213203435596)) ;
#85882=CARTESIAN_POINT('Origin',(34.1,245.6,30.8213203435596)) ;
#85883=CARTESIAN_POINT('Origin',(33.6,245.6,30.8213203435596)) ;
#85884=CARTESIAN_POINT('Origin',(34.1000000000001,244.191753592594,30.8213203435596)) ;
#85885=CARTESIAN_POINT('',(34.2000000000001,244.191753592594,30.8213203435596)) ;
#85886=CARTESIAN_POINT('Origin',(51.2,257.,30.1213203435596)) ;
#85887=CARTESIAN_POINT('',(49.,257.,30.3213203435596)) ;
#85888=CARTESIAN_POINT('Origin',(49.,257.,30.1213203435596)) ;
#85889=CARTESIAN_POINT('Origin',(51.2,257.,30.3213203435596)) ;
#85890=CARTESIAN_POINT('Origin',(51.2,257.,30.3213203435596)) ;
#85891=CARTESIAN_POINT('',(53.8,257.,30.3213203435596)) ;
#85892=CARTESIAN_POINT('Origin',(51.2,257.,30.3213203435596)) ;
#85893=CARTESIAN_POINT('Origin',(51.2,257.,30.5213203435596)) ;
#85894=CARTESIAN_POINT('',(48.4,257.,30.5213203435596)) ;
#85895=CARTESIAN_POINT('',(54.,257.,30.5213203435596)) ;
#85896=CARTESIAN_POINT('Origin',(51.2,257.,30.5213203435596)) ;
#85897=CARTESIAN_POINT('Origin',(53.8,257.,30.5213203435596)) ;
#85898=CARTESIAN_POINT('Origin',(51.2,257.,30.5213203435596)) ;
#85899=CARTESIAN_POINT('Origin',(51.2,257.,30.9213203435596)) ;
#85900=CARTESIAN_POINT('',(48.4,257.,30.8969367901425)) ;
#85901=CARTESIAN_POINT('Origin',(51.2,257.,30.8969367901425)) ;
#85902=CARTESIAN_POINT('',(48.4,257.,30.9213203435596)) ;
#85903=CARTESIAN_POINT('Origin',(51.2,257.,30.8969367901425)) ;
#85904=CARTESIAN_POINT('',(48.3936201934668,257.,30.9470488713393)) ;
#85905=CARTESIAN_POINT('Origin',(48.2,257.,30.8969367901425)) ;
#85906=CARTESIAN_POINT('',(54.0063798065332,257.,30.9470488713393)) ;
#85907=CARTESIAN_POINT('Origin',(51.2,257.,30.9470488713393)) ;
#85908=CARTESIAN_POINT('Origin',(51.2,257.,30.9470488713393)) ;
#85909=CARTESIAN_POINT('Origin',(73.2,257.,30.8969367901425)) ;
#85910=CARTESIAN_POINT('',(70.3999999999999,257.,30.8969367901425)) ;
#85911=CARTESIAN_POINT('Origin',(73.2,257.,30.8969367901425)) ;
#85912=CARTESIAN_POINT('',(70.3936201934668,257.,30.9470488713393)) ;
#85913=CARTESIAN_POINT('Origin',(70.2,257.,30.8969367901425)) ;
#85914=CARTESIAN_POINT('',(76.0063798065332,257.,30.9470488713393)) ;
#85915=CARTESIAN_POINT('Origin',(73.2,257.,30.9470488713393)) ;
#85916=CARTESIAN_POINT('Origin',(73.2,257.,30.9470488713393)) ;
#85917=CARTESIAN_POINT('Origin',(73.2,257.,30.9213203435596)) ;
#85918=CARTESIAN_POINT('',(70.4,257.,30.5213203435596)) ;
#85919=CARTESIAN_POINT('',(70.4,257.,30.9213203435596)) ;
#85920=CARTESIAN_POINT('',(76.,257.,30.5213203435596)) ;
#85921=CARTESIAN_POINT('Origin',(73.2,257.,30.5213203435596)) ;
#85922=CARTESIAN_POINT('Origin',(73.2,257.,30.5213203435596)) ;
#85923=CARTESIAN_POINT('Origin',(73.2,257.,30.5213203435596)) ;
#85924=CARTESIAN_POINT('',(75.8,257.,30.3213203435596)) ;
#85925=CARTESIAN_POINT('Origin',(75.8,257.,30.5213203435596)) ;
#85926=CARTESIAN_POINT('Origin',(73.2,257.,30.3213203435596)) ;
#85927=CARTESIAN_POINT('Origin',(73.2,257.,30.3213203435596)) ;
#85928=CARTESIAN_POINT('',(71.,257.,30.3213203435596)) ;
#85929=CARTESIAN_POINT('Origin',(73.2,257.,30.3213203435596)) ;
#85930=CARTESIAN_POINT('Origin',(73.2,257.,30.1213203435596)) ;
#85931=CARTESIAN_POINT('',(71.2,257.,30.1213203435596)) ;
#85932=CARTESIAN_POINT('Origin',(73.2,257.,30.1213203435596)) ;
#85933=CARTESIAN_POINT('Origin',(71.,257.,30.1213203435596)) ;
#85934=CARTESIAN_POINT('Origin',(73.2,257.,19.9213203435596)) ;
#85935=CARTESIAN_POINT('',(71.2,257.,29.6213203435596)) ;
#85936=CARTESIAN_POINT('Origin',(73.2,257.,29.6213203435596)) ;
#85937=CARTESIAN_POINT('',(71.2,257.,19.9213203435596)) ;
#85938=CARTESIAN_POINT('Origin',(75.7500000000001,218.,30.8969367901425)) ;
#85939=CARTESIAN_POINT('',(72.9500000000001,218.,30.8969367901425)) ;
#85940=CARTESIAN_POINT('Origin',(75.7500000000001,218.,30.8969367901425)) ;
#85941=CARTESIAN_POINT('',(72.9436201934669,218.,30.9470488713393)) ;
#85942=CARTESIAN_POINT('Origin',(72.7500000000001,218.,30.8969367901425)) ;
#85943=CARTESIAN_POINT('',(78.5563798065333,218.,30.9470488713393)) ;
#85944=CARTESIAN_POINT('Origin',(75.7500000000001,218.,30.9470488713393)) ;
#85945=CARTESIAN_POINT('Origin',(75.7500000000001,218.,30.9470488713393)) ;
#85946=CARTESIAN_POINT('Origin',(75.7500000000001,218.,30.9213203435596)) ;
#85947=CARTESIAN_POINT('',(72.9500000000001,218.,30.5213203435596)) ;
#85948=CARTESIAN_POINT('',(72.9500000000001,218.,30.9213203435596)) ;
#85949=CARTESIAN_POINT('',(78.5500000000001,218.,30.5213203435596)) ;
#85950=CARTESIAN_POINT('Origin',(75.7500000000001,218.,30.5213203435596)) ;
#85951=CARTESIAN_POINT('Origin',(75.7500000000001,218.,30.5213203435596)) ;
#85952=CARTESIAN_POINT('Origin',(75.7500000000001,218.,30.1213203435596)) ;
#85953=CARTESIAN_POINT('',(73.5500000000001,218.,30.3213203435596)) ;
#85954=CARTESIAN_POINT('Origin',(73.5500000000001,218.,30.1213203435596)) ;
#85955=CARTESIAN_POINT('Origin',(75.7500000000001,218.,30.3213203435596)) ;
#85956=CARTESIAN_POINT('Origin',(75.7500000000001,218.,30.3213203435596)) ;
#85957=CARTESIAN_POINT('',(78.3500000000001,218.,30.3213203435596)) ;
#85958=CARTESIAN_POINT('Origin',(75.7500000000001,218.,30.3213203435596)) ;
#85959=CARTESIAN_POINT('Origin',(75.7500000000001,218.,30.5213203435596)) ;
#85960=CARTESIAN_POINT('Origin',(78.3500000000001,218.,30.5213203435596)) ;
#85961=CARTESIAN_POINT('Origin',(51.2,257.,30.6213203435596)) ;
#85962=CARTESIAN_POINT('Origin',(55.2649110640674,257.,30.6213203435596)) ;
#85963=CARTESIAN_POINT('Origin',(73.2,257.,30.6213203435596)) ;
#85964=CARTESIAN_POINT('Origin',(77.2649110640674,257.,30.6213203435596)) ;
#85965=CARTESIAN_POINT('Origin',(75.7500000000001,218.,30.6213203435596)) ;
#85966=CARTESIAN_POINT('Origin',(79.8149110640674,218.,30.6213203435596)) ;
#85967=CARTESIAN_POINT('Origin',(73.2,257.,29.6213203435596)) ;
#85968=CARTESIAN_POINT('Origin',(33.6,245.6,19.9213203435596)) ;
#85969=CARTESIAN_POINT('',(33.6,245.,19.9213203435596)) ;
#85970=CARTESIAN_POINT('',(34.2,245.6,19.9213203435596)) ;
#85971=CARTESIAN_POINT('Origin',(26.2,245.,19.9213203435596)) ;
#85972=CARTESIAN_POINT('',(26.8,245.,19.9213203435596)) ;
#85973=CARTESIAN_POINT('Origin',(26.8,245.6,19.9213203435596)) ;
#85974=CARTESIAN_POINT('Origin',(75.5999999999993,225.9,19.9213203435596)) ;
#85975=CARTESIAN_POINT('Origin',(75.1999999999994,230.5,19.9213203435596)) ;
#85976=CARTESIAN_POINT('Origin',(75.5999999999994,230.1,19.9213203435596)) ;
#85977=CARTESIAN_POINT('Origin',(80.199999999999,230.5,19.9213203435596)) ;
#85978=CARTESIAN_POINT('Origin',(80.199999999999,253.5,19.9213203435596)) ;
#85979=CARTESIAN_POINT('Ctrl Pts',(46.8995772828086,264.999999634466,30.7206748684131)) ;
#85980=CARTESIAN_POINT('Ctrl Pts',(46.8996347166691,265.000098160446,30.900346512201)) ;
#85981=CARTESIAN_POINT('Ctrl Pts',(46.8518142718604,264.918063685094,31.2588421307007)) ;
#85982=CARTESIAN_POINT('Ctrl Pts',(46.6177377231473,264.516555192435,31.7637752135733)) ;
#85983=CARTESIAN_POINT('Ctrl Pts',(46.3570192595451,264.069339743442,31.9213203435596)) ;
#85984=CARTESIAN_POINT('Ctrl Pts',(46.2,263.8,31.9213203435596)) ;
#85985=CARTESIAN_POINT('Ctrl Pts',(47.0306190770353,265.00011652697,30.7206035829153)) ;
#85986=CARTESIAN_POINT('Ctrl Pts',(47.0307043719217,265.0002417701,30.9201211188153)) ;
#85987=CARTESIAN_POINT('Ctrl Pts',(46.9596768730597,264.895948135418,31.3129265397466)) ;
#85988=CARTESIAN_POINT('Ctrl Pts',(46.6673261574499,264.467185432906,31.790097128723)) ;
#85989=CARTESIAN_POINT('Ctrl Pts',(46.3757393401946,264.050619662792,31.9213203435596)) ;
#85990=CARTESIAN_POINT('Ctrl Pts',(46.2,263.8,31.9213203435596)) ;
#85991=CARTESIAN_POINT('Ctrl Pts',(47.2915525808353,264.891552580839,30.7205226506387)) ;
#85992=CARTESIAN_POINT('Ctrl Pts',(47.2916923685089,264.891692368513,30.9425726727612)) ;
#85993=CARTESIAN_POINT('Ctrl Pts',(47.175274965989,264.775274965993,31.372780469797)) ;
#85994=CARTESIAN_POINT('Ctrl Pts',(46.7673172266825,264.367317226684,31.8157593328667)) ;
#85995=CARTESIAN_POINT('Ctrl Pts',(46.4131795014931,264.013179501493,31.9213203435596)) ;
#85996=CARTESIAN_POINT('Ctrl Pts',(46.2,263.8,31.9213203435596)) ;
#85997=CARTESIAN_POINT('Ctrl Pts',(47.400116526968,264.630619077042,30.7206035829153)) ;
#85998=CARTESIAN_POINT('Ctrl Pts',(47.4002417700975,264.630704371928,30.9201211188158)) ;
#85999=CARTESIAN_POINT('Ctrl Pts',(47.295948135415,264.559676873064,31.3129265397479)) ;
#86000=CARTESIAN_POINT('Ctrl Pts',(46.8671854329034,264.267326157452,31.7900971287236)) ;
#86001=CARTESIAN_POINT('Ctrl Pts',(46.4506196627917,263.975739340196,31.9213203435596)) ;
#86002=CARTESIAN_POINT('Ctrl Pts',(46.2,263.8,31.9213203435596)) ;
#86003=CARTESIAN_POINT('Ctrl Pts',(47.3999996344655,264.499577282817,30.7206748684131)) ;
#86004=CARTESIAN_POINT('Ctrl Pts',(47.4000981604458,264.499634716678,30.9003465122023)) ;
#86005=CARTESIAN_POINT('Ctrl Pts',(47.3180636850924,264.451814271868,31.2588421307041)) ;
#86006=CARTESIAN_POINT('Ctrl Pts',(46.9165551924319,264.21773772315,31.763775213575)) ;
#86007=CARTESIAN_POINT('Ctrl Pts',(46.4693397434408,263.957019259546,31.9213203435596)) ;
#86008=CARTESIAN_POINT('Ctrl Pts',(46.2,263.8,31.9213203435596)) ;
#86009=CARTESIAN_POINT('Origin',(46.2,263.8,30.7213203435596)) ;
#86010=CARTESIAN_POINT('',(47.4,264.5,30.7213203435596)) ;
#86011=CARTESIAN_POINT('Origin',(46.2,263.8,30.7213203435596)) ;
#86012=CARTESIAN_POINT('Origin',(46.9,264.5,30.7213203435596)) ;
#86013=CARTESIAN_POINT('Ctrl Pts',(55.0000127765018,264.497506774224,30.717524648916)) ;
#86014=CARTESIAN_POINT('Ctrl Pts',(54.99912644432,264.498021883759,30.9874956561826)) ;
#86015=CARTESIAN_POINT('Ctrl Pts',(55.2172274582073,264.371268236017,31.6180363905289)) ;
#86016=CARTESIAN_POINT('Ctrl Pts',(55.8404866413515,264.008965312001,31.9213203435596)) ;
#86017=CARTESIAN_POINT('Ctrl Pts',(56.2,263.8,31.9213203435596)) ;
#86018=CARTESIAN_POINT('Ctrl Pts',(54.9993214128065,264.629240949551,30.7170995183319)) ;
#86019=CARTESIAN_POINT('Ctrl Pts',(54.9981949105548,264.629996957963,31.0173898959233)) ;
#86020=CARTESIAN_POINT('Ctrl Pts',(55.2755991661809,264.443841808721,31.6781435477989)) ;
#86021=CARTESIAN_POINT('Ctrl Pts',(55.8655779824594,264.034056653109,31.9213203435596)) ;
#86022=CARTESIAN_POINT('Ctrl Pts',(56.2,263.8,31.9213203435596)) ;
#86023=CARTESIAN_POINT('Ctrl Pts',(55.1080548223873,264.891945177613,30.7166163696442)) ;
#86024=CARTESIAN_POINT('Ctrl Pts',(55.1068252095724,264.893174790428,31.0513754562231)) ;
#86025=CARTESIAN_POINT('Ctrl Pts',(55.4097601276945,264.590239872305,31.7407074319743)) ;
#86026=CARTESIAN_POINT('Ctrl Pts',(55.9157606646752,264.084239335325,31.9213203435596)) ;
#86027=CARTESIAN_POINT('Ctrl Pts',(56.2,263.8,31.9213203435596)) ;
#86028=CARTESIAN_POINT('Ctrl Pts',(55.3707590504493,265.000678587193,30.7170995183319)) ;
#86029=CARTESIAN_POINT('Ctrl Pts',(55.3700030420373,265.001805089445,31.0173898959233)) ;
#86030=CARTESIAN_POINT('Ctrl Pts',(55.5561581912784,264.724400833819,31.6781435477988)) ;
#86031=CARTESIAN_POINT('Ctrl Pts',(55.965943346891,264.134422017541,31.9213203435596)) ;
#86032=CARTESIAN_POINT('Ctrl Pts',(56.2,263.8,31.9213203435596)) ;
#86033=CARTESIAN_POINT('Ctrl Pts',(55.5024932257763,264.999987223498,30.7175246489159)) ;
#86034=CARTESIAN_POINT('Ctrl Pts',(55.5019781162411,265.00087355568,30.9874956561826)) ;
#86035=CARTESIAN_POINT('Ctrl Pts',(55.6287317639835,264.782772541792,31.6180363905288)) ;
#86036=CARTESIAN_POINT('Ctrl Pts',(55.9910346879988,264.159513358648,31.9213203435596)) ;
#86037=CARTESIAN_POINT('Ctrl Pts',(56.2,263.8,31.9213203435596)) ;
#86038=CARTESIAN_POINT('',(55.,264.5,30.7213203435596)) ;
#86039=CARTESIAN_POINT('',(55.3522605104815,264.294514702219,31.5706363965757)) ;
#86040=CARTESIAN_POINT('Origin',(56.2,263.8,30.7213203435596)) ;
#86041=CARTESIAN_POINT('Origin',(56.2,263.8,30.7213203435596)) ;
#86042=CARTESIAN_POINT('',(55.7054852977724,264.647739489533,31.5706363965612)) ;
#86043=CARTESIAN_POINT('Origin',(56.2,263.8,30.7213203435596)) ;
#86044=CARTESIAN_POINT('Origin',(56.2,263.8,30.7213203435596)) ;
#86045=CARTESIAN_POINT('Origin',(55.5,264.5,30.7213203435596)) ;
#86046=CARTESIAN_POINT('Ctrl Pts',(68.8975058001088,264.999987213392,30.7175231713329)) ;
#86047=CARTESIAN_POINT('Ctrl Pts',(68.8980211176555,265.000873904652,30.9874944556892)) ;
#86048=CARTESIAN_POINT('Ctrl Pts',(68.7712660652602,264.782770188553,31.618033084322)) ;
#86049=CARTESIAN_POINT('Ctrl Pts',(68.4089651270207,264.159513543629,31.9213203435596)) ;
#86050=CARTESIAN_POINT('Ctrl Pts',(68.2,263.8,31.9213203435596)) ;
#86051=CARTESIAN_POINT('Ctrl Pts',(69.0292403053076,265.000678853629,30.7170978723306)) ;
#86052=CARTESIAN_POINT('Ctrl Pts',(69.0299966176013,265.001805816084,31.0173888110261)) ;
#86053=CARTESIAN_POINT('Ctrl Pts',(68.8438397072984,264.72439710198,31.678134090218)) ;
#86054=CARTESIAN_POINT('Ctrl Pts',(68.4340565297887,264.134422140861,31.9213203435596)) ;
#86055=CARTESIAN_POINT('Ctrl Pts',(68.2,263.8,31.9213203435596)) ;
#86056=CARTESIAN_POINT('Ctrl Pts',(69.2919444837221,264.891944483736,30.7166145318953)) ;
#86057=CARTESIAN_POINT('Ctrl Pts',(69.293174578849,264.893174578863,31.0513745401012)) ;
#86058=CARTESIAN_POINT('Ctrl Pts',(68.990239681009,264.590239681019,31.7406867780937)) ;
#86059=CARTESIAN_POINT('Ctrl Pts',(68.4842393353228,264.084239335327,31.9213203435596)) ;
#86060=CARTESIAN_POINT('Ctrl Pts',(68.2,263.8,31.9213203435596)) ;
#86061=CARTESIAN_POINT('Ctrl Pts',(69.400678853621,264.629240305328,30.7170978723306)) ;
#86062=CARTESIAN_POINT('Ctrl Pts',(69.4018058160759,264.629996617621,31.0173888110287)) ;
#86063=CARTESIAN_POINT('Ctrl Pts',(69.12439710197,264.443839707309,31.6781340902227)) ;
#86064=CARTESIAN_POINT('Ctrl Pts',(68.5344221408571,264.034056529793,31.9213203435596)) ;
#86065=CARTESIAN_POINT('Ctrl Pts',(68.2,263.8,31.9213203435596)) ;
#86066=CARTESIAN_POINT('Ctrl Pts',(69.3999872133923,264.497505800138,30.7175231713328)) ;
#86067=CARTESIAN_POINT('Ctrl Pts',(69.4008739046523,264.498021117685,30.9874944556959)) ;
#86068=CARTESIAN_POINT('Ctrl Pts',(69.1827701885397,264.371266065276,31.6180330843354)) ;
#86069=CARTESIAN_POINT('Ctrl Pts',(68.5595135436233,264.008965127026,31.9213203435596)) ;
#86070=CARTESIAN_POINT('Ctrl Pts',(68.2,263.8,31.9213203435596)) ;
#86071=CARTESIAN_POINT('',(68.694428877676,264.64759236173,31.570783225819)) ;
#86072=CARTESIAN_POINT('Origin',(68.2,263.8,30.7213203435596)) ;
#86073=CARTESIAN_POINT('Origin',(68.2,263.8,30.7213203435596)) ;
#86074=CARTESIAN_POINT('',(69.0475923616046,264.294428877603,31.5707832259444)) ;
#86075=CARTESIAN_POINT('Origin',(68.2,263.8,30.7213203435596)) ;
#86076=CARTESIAN_POINT('',(69.4,264.5,30.7213203435596)) ;
#86077=CARTESIAN_POINT('Origin',(68.2,263.8,30.7213203435596)) ;
#86078=CARTESIAN_POINT('Origin',(68.9,264.5,30.7213203435596)) ;
#86079=CARTESIAN_POINT('Ctrl Pts',(77.0000127930585,264.497505178544,30.7175222285172)) ;
#86080=CARTESIAN_POINT('Ctrl Pts',(76.999125872671,264.498020628823,30.9874936896829)) ;
#86081=CARTESIAN_POINT('Ctrl Pts',(77.2172313133203,264.371264679952,31.6180309744835)) ;
#86082=CARTESIAN_POINT('Ctrl Pts',(77.8404863383386,264.008965008988,31.9213203435596)) ;
#86083=CARTESIAN_POINT('Ctrl Pts',(78.2,263.8,31.9213203435596)) ;
#86084=CARTESIAN_POINT('Ctrl Pts',(76.999320976368,264.629239894225,30.7170968220494)) ;
#86085=CARTESIAN_POINT('Ctrl Pts',(76.9981937202562,264.629996400424,31.0173881187927)) ;
#86086=CARTESIAN_POINT('Ctrl Pts',(77.2756052796858,264.44383836622,31.6781280546311)) ;
#86087=CARTESIAN_POINT('Ctrl Pts',(77.8655777804508,264.034056451101,31.9213203435596)) ;
#86088=CARTESIAN_POINT('Ctrl Pts',(78.2,263.8,31.9213203435596)) ;
#86089=CARTESIAN_POINT('Ctrl Pts',(77.1080559582206,264.891944041766,30.7166133592621)) ;
#86090=CARTESIAN_POINT('Ctrl Pts',(77.1068255553296,264.893174444657,31.0513739555782)) ;
#86091=CARTESIAN_POINT('Ctrl Pts',(77.4097604424929,264.590239557496,31.7406735987709)) ;
#86092=CARTESIAN_POINT('Ctrl Pts',(77.9157606646733,264.084239335323,31.9213203435596)) ;
#86093=CARTESIAN_POINT('Ctrl Pts',(78.2,263.8,31.9213203435596)) ;
#86094=CARTESIAN_POINT('Ctrl Pts',(77.370760105756,265.000679023624,30.7170968220493)) ;
#86095=CARTESIAN_POINT('Ctrl Pts',(77.3700035995569,265.001806279736,31.0173881187952)) ;
#86096=CARTESIAN_POINT('Ctrl Pts',(77.5561616337687,264.724394720305,31.6781280546357)) ;
#86097=CARTESIAN_POINT('Ctrl Pts',(77.965943548896,264.134422219546,31.9213203435596)) ;
#86098=CARTESIAN_POINT('Ctrl Pts',(78.2,263.8,31.9213203435596)) ;
#86099=CARTESIAN_POINT('Ctrl Pts',(77.5024948214269,264.999987206942,30.7175222285171)) ;
#86100=CARTESIAN_POINT('Ctrl Pts',(77.5019793711485,265.000874127329,30.9874936896894)) ;
#86101=CARTESIAN_POINT('Ctrl Pts',(77.6287353200318,264.782768686667,31.6180309744965)) ;
#86102=CARTESIAN_POINT('Ctrl Pts',(77.9910349910063,264.159513661656,31.9213203435596)) ;
#86103=CARTESIAN_POINT('Ctrl Pts',(78.2,263.8,31.9213203435596)) ;
#86104=CARTESIAN_POINT('',(77.,264.5,30.7213203435596)) ;
#86105=CARTESIAN_POINT('',(77.3525015634302,264.294374087999,31.5708769337946)) ;
#86106=CARTESIAN_POINT('Origin',(78.2,263.8,30.7213203435596)) ;
#86107=CARTESIAN_POINT('Origin',(78.2,263.8,30.7213203435596)) ;
#86108=CARTESIAN_POINT('Origin',(77.5,264.5,30.7213203435596)) ;
#86109=CARTESIAN_POINT('Origin',(78.2,252.191753592594,30.7213203435596)) ;
#86110=CARTESIAN_POINT('',(77.,263.763591785235,30.7213203435596)) ;
#86111=CARTESIAN_POINT('',(77.,252.191753592594,30.7213203435596)) ;
#86112=CARTESIAN_POINT('Origin',(78.2,263.763591785235,30.7213203435596)) ;
#86113=CARTESIAN_POINT('Ctrl Pts',(76.4995190226377,262.026327156306,31.9213203435596)) ;
#86114=CARTESIAN_POINT('Ctrl Pts',(76.8811596225238,262.026212180825,31.9213203435596)) ;
#86115=CARTESIAN_POINT('Ctrl Pts',(77.5148352095089,262.254066418952,31.9213203435596)) ;
#86116=CARTESIAN_POINT('Ctrl Pts',(78.0836688954258,262.984975488253,31.9213203435596)) ;
#86117=CARTESIAN_POINT('Ctrl Pts',(78.2000733801637,263.504024694381,31.9213203435596)) ;
#86118=CARTESIAN_POINT('Ctrl Pts',(78.1999999305895,263.764083305616,31.9213203435596)) ;
#86119=CARTESIAN_POINT('Ctrl Pts',(76.4996093403379,262.337938596679,31.9213203432719)) ;
#86120=CARTESIAN_POINT('Ctrl Pts',(76.8095855113217,262.337841295896,31.9213207998724)) ;
#86121=CARTESIAN_POINT('Ctrl Pts',(77.3248206408524,262.530669626882,31.9204156081284)) ;
#86122=CARTESIAN_POINT('Ctrl Pts',(77.7690289165673,263.136266572609,31.9210372315204)) ;
#86123=CARTESIAN_POINT('Ctrl Pts',(77.848207800611,263.556750307023,31.9210300573126)) ;
#86124=CARTESIAN_POINT('Ctrl Pts',(77.8409471725199,263.763983467654,31.9213208928997)) ;
#86125=CARTESIAN_POINT('Ctrl Pts',(76.4997657781298,262.879952924587,31.697544092197)) ;
#86126=CARTESIAN_POINT('Ctrl Pts',(76.685613962614,262.879887256888,31.6975487112581)) ;
#86127=CARTESIAN_POINT('Ctrl Pts',(76.9925944092368,263.010027791412,31.6883950616448)) ;
#86128=CARTESIAN_POINT('Ctrl Pts',(77.2228704336,263.397819282277,31.6563868166324)) ;
#86129=CARTESIAN_POINT('Ctrl Pts',(77.238135214489,263.647341999612,31.6322498913161)) ;
#86130=CARTESIAN_POINT('Ctrl Pts',(77.2194335073132,263.763811927863,31.6196189939447)) ;
#86131=CARTESIAN_POINT('Ctrl Pts',(76.4998448149111,263.152594688376,31.1969452376454)) ;
#86132=CARTESIAN_POINT('Ctrl Pts',(76.6229793650612,263.152550698014,31.1969584257997)) ;
#86133=CARTESIAN_POINT('Ctrl Pts',(76.8274272241081,263.23973060012,31.1708228417253)) ;
#86134=CARTESIAN_POINT('Ctrl Pts',(76.9892209015336,263.503877433016,31.0845228152707)) ;
#86135=CARTESIAN_POINT('Ctrl Pts',(77.0082592674544,263.679638279009,31.0219906010643)) ;
#86136=CARTESIAN_POINT('Ctrl Pts',(76.9998598913761,263.763750765635,30.99018357636)) ;
#86137=CARTESIAN_POINT('Ctrl Pts',(76.4998585633068,263.20068211308,30.9680799623059)) ;
#86138=CARTESIAN_POINT('Ctrl Pts',(76.6120841869172,263.200644865691,30.968096329597)) ;
#86139=CARTESIAN_POINT('Ctrl Pts',(76.7984234856098,263.27446038894,30.9356602252213)) ;
#86140=CARTESIAN_POINT('Ctrl Pts',(76.9657383928732,263.511275997684,30.831616819832)) ;
#86141=CARTESIAN_POINT('Ctrl Pts',(77.0000051280261,263.679472135069,30.7577337022785)) ;
#86142=CARTESIAN_POINT('Ctrl Pts',(77.0000001340552,263.763751075536,30.720717075604)) ;
#86143=CARTESIAN_POINT('Origin',(76.5,262.026327083856,30.7213203435596)) ;
#86144=CARTESIAN_POINT('Origin',(76.5,263.763591785235,30.7213203435596)) ;
#86145=CARTESIAN_POINT('Origin',(64.4,262.026327083856,30.7213203435596)) ;
#86146=CARTESIAN_POINT('Origin',(69.9,262.026327083856,30.7213203435596)) ;
#86147=CARTESIAN_POINT('Ctrl Pts',(68.1983125112596,263.765148977383,31.9213190650864)) ;
#86148=CARTESIAN_POINT('Ctrl Pts',(68.1980077983924,263.374417823647,31.9213212039938)) ;
#86149=CARTESIAN_POINT('Ctrl Pts',(68.5095269157522,262.461458547847,31.9213224688896)) ;
#86150=CARTESIAN_POINT('Ctrl Pts',(69.3919168992797,262.024364125748,31.9213193980855)) ;
#86151=CARTESIAN_POINT('Ctrl Pts',(69.9015236996613,262.024862823348,31.9213194015866)) ;
#86152=CARTESIAN_POINT('Ctrl Pts',(68.5579695947186,263.764832436952,31.9218621048563)) ;
#86153=CARTESIAN_POINT('Ctrl Pts',(68.5469047154847,263.45353874313,31.9213904806212)) ;
#86154=CARTESIAN_POINT('Ctrl Pts',(68.7720647452498,262.70680443246,31.9210845767404)) ;
#86155=CARTESIAN_POINT('Ctrl Pts',(69.4873911960094,262.336546050699,31.9217215128341)) ;
#86156=CARTESIAN_POINT('Ctrl Pts',(69.901237377907,262.336968483875,31.9217207866612)) ;
#86157=CARTESIAN_POINT('Ctrl Pts',(69.1805657273697,263.764288546693,31.6200744602099)) ;
#86158=CARTESIAN_POINT('Ctrl Pts',(69.1523633773431,263.589485112743,31.6390141732535)) ;
#86159=CARTESIAN_POINT('Ctrl Pts',(69.2295848925071,263.131551068329,31.6803391920196)) ;
#86160=CARTESIAN_POINT('Ctrl Pts',(69.6527467734552,262.879525187827,31.6979704437927)) ;
#86161=CARTESIAN_POINT('Ctrl Pts',(69.9007414815215,262.879812711463,31.6979503261674)) ;
#86162=CARTESIAN_POINT('Ctrl Pts',(69.4002579350921,263.764094862603,30.9898143483238)) ;
#86163=CARTESIAN_POINT('Ctrl Pts',(69.3875802847056,263.637875419481,31.0375709322432)) ;
#86164=CARTESIAN_POINT('Ctrl Pts',(69.4541887094701,263.320310298445,31.1465777171764)) ;
#86165=CARTESIAN_POINT('Ctrl Pts',(69.7362429697597,263.152507028698,31.196812365578)) ;
#86166=CARTESIAN_POINT('Ctrl Pts',(69.900491089929,263.152698471114,31.1967550496367)) ;
#86167=CARTESIAN_POINT('Ctrl Pts',(69.3999996982701,263.764095954884,30.7202075564157)) ;
#86168=CARTESIAN_POINT('Ctrl Pts',(69.3999369107821,263.63758951881,30.7757813606872)) ;
#86169=CARTESIAN_POINT('Ctrl Pts',(69.4915234368195,263.342047582185,30.9056533534648)) ;
#86170=CARTESIAN_POINT('Ctrl Pts',(69.7507436235131,263.200584779449,30.9678467447103)) ;
#86171=CARTESIAN_POINT('Ctrl Pts',(69.9004476076753,263.200746179747,30.9677757859222)) ;
#86172=CARTESIAN_POINT('',(69.4,263.763591785235,30.7213203435597)) ;
#86173=CARTESIAN_POINT('Origin',(68.2,263.763591785235,30.7213203435596)) ;
#86174=CARTESIAN_POINT('Origin',(69.9,263.763591785235,30.7213203435596)) ;
#86175=CARTESIAN_POINT('Origin',(68.2,251.191753592594,30.7213203435596)) ;
#86176=CARTESIAN_POINT('',(69.4,251.191753592594,30.7213203435596)) ;
#86177=CARTESIAN_POINT('Origin',(66.4499999999999,263.8,30.7213203435596)) ;
#86178=CARTESIAN_POINT('Origin',(56.2,252.191753592594,30.7213203435596)) ;
#86179=CARTESIAN_POINT('',(55.,263.763591785235,30.7213203435596)) ;
#86180=CARTESIAN_POINT('',(55.,252.191753592594,30.7213203435596)) ;
#86181=CARTESIAN_POINT('Origin',(56.2,263.763591785235,30.7213203435596)) ;
#86182=CARTESIAN_POINT('Ctrl Pts',(54.4995191990323,262.026327156252,31.9213203435596)) ;
#86183=CARTESIAN_POINT('Ctrl Pts',(54.8811597389274,262.026212224654,31.9213203435596)) ;
#86184=CARTESIAN_POINT('Ctrl Pts',(55.5148367741968,262.25406310381,31.9213203435596)) ;
#86185=CARTESIAN_POINT('Ctrl Pts',(56.0836704564179,262.98497327714,31.9213203435596)) ;
#86186=CARTESIAN_POINT('Ctrl Pts',(56.2000733522523,263.50402457578,31.9213203435596)) ;
#86187=CARTESIAN_POINT('Ctrl Pts',(56.1999999306414,263.764083125354,31.9213203435596)) ;
#86188=CARTESIAN_POINT('Ctrl Pts',(54.4996094836088,262.337938596633,31.9213203432732)) ;
#86189=CARTESIAN_POINT('Ctrl Pts',(54.8095856066388,262.337841334075,31.9213207980662)) ;
#86190=CARTESIAN_POINT('Ctrl Pts',(55.324820581982,262.530664663494,31.9204188586157)) ;
#86191=CARTESIAN_POINT('Ctrl Pts',(55.7690292246145,263.136262709219,31.9210399847418)) ;
#86192=CARTESIAN_POINT('Ctrl Pts',(55.8482077820982,263.556750212249,31.9210300555789)) ;
#86193=CARTESIAN_POINT('Ctrl Pts',(55.8409471775529,263.763983324007,31.9213208926998)) ;
#86194=CARTESIAN_POINT('Ctrl Pts',(54.4997658640126,262.87995410944,31.6975454235242)) ;
#86195=CARTESIAN_POINT('Ctrl Pts',(54.6856140321838,262.879888467203,31.6975500409814)) ;
#86196=CARTESIAN_POINT('Ctrl Pts',(54.9925945661554,263.010026293502,31.6883962107278)) ;
#86197=CARTESIAN_POINT('Ctrl Pts',(55.222870433538,263.397818932101,31.6563880739499)) ;
#86198=CARTESIAN_POINT('Ctrl Pts',(55.2381328918591,263.647341932731,31.6322519116531)) ;
#86199=CARTESIAN_POINT('Ctrl Pts',(55.2194312038371,263.763811847149,31.6196210183214)) ;
#86200=CARTESIAN_POINT('Ctrl Pts',(54.4998448718075,263.15259463109,31.1969453407673)) ;
#86201=CARTESIAN_POINT('Ctrl Pts',(54.6229794158692,263.152550658295,31.196958524294)) ;
#86202=CARTESIAN_POINT('Ctrl Pts',(54.8274272512656,263.239727731085,31.1708225203607)) ;
#86203=CARTESIAN_POINT('Ctrl Pts',(54.9892211600963,263.503875278608,31.0845224833632)) ;
#86204=CARTESIAN_POINT('Ctrl Pts',(55.0082593119534,263.67963823302,31.0219907412878)) ;
#86205=CARTESIAN_POINT('Ctrl Pts',(54.9998599440985,263.763750707344,30.9901837278691)) ;
#86206=CARTESIAN_POINT('Ctrl Pts',(54.4998586151676,263.200682078159,30.9680801284357)) ;
#86207=CARTESIAN_POINT('Ctrl Pts',(54.6120842290547,263.20064484498,30.9680964894767)) ;
#86208=CARTESIAN_POINT('Ctrl Pts',(54.7984239677902,263.274459292836,30.9356608694408)) ;
#86209=CARTESIAN_POINT('Ctrl Pts',(54.9657388695267,263.511275278549,30.8316173195593)) ;
#86210=CARTESIAN_POINT('Ctrl Pts',(55.0000051257995,263.679472096755,30.7577339109711)) ;
#86211=CARTESIAN_POINT('Ctrl Pts',(55.0000001339559,263.763751017118,30.7207172968552)) ;
#86212=CARTESIAN_POINT('Origin',(54.5,262.026327083856,30.7213203435596)) ;
#86213=CARTESIAN_POINT('Origin',(54.5,263.763591785235,30.7213203435596)) ;
#86214=CARTESIAN_POINT('Origin',(53.4,262.026327083856,30.7213203435596)) ;
#86215=CARTESIAN_POINT('Origin',(47.9,262.026327083856,30.7213203435596)) ;
#86216=CARTESIAN_POINT('Ctrl Pts',(46.1983076282625,263.76515348891,31.9213190576818)) ;
#86217=CARTESIAN_POINT('Ctrl Pts',(46.1980020403729,263.374419766008,31.9213212030712)) ;
#86218=CARTESIAN_POINT('Ctrl Pts',(46.5095143637924,262.461447593742,31.9213224512428)) ;
#86219=CARTESIAN_POINT('Ctrl Pts',(47.3919185200641,262.024358451223,31.9213193926338)) ;
#86220=CARTESIAN_POINT('Ctrl Pts',(47.9015281138921,262.024858587217,31.9213193961311)) ;
#86221=CARTESIAN_POINT('Ctrl Pts',(46.5579664947406,263.764836030645,31.921863668865)) ;
#86222=CARTESIAN_POINT('Ctrl Pts',(46.5469008415638,263.453540510638,31.9213919346374)) ;
#86223=CARTESIAN_POINT('Ctrl Pts',(46.7720552690258,262.706793116683,31.9210902454287)) ;
#86224=CARTESIAN_POINT('Ctrl Pts',(47.4873927052263,262.336542026587,31.9217226657269)) ;
#86225=CARTESIAN_POINT('Ctrl Pts',(47.9012409620629,262.33696567494,31.921721942615)) ;
#86226=CARTESIAN_POINT('Ctrl Pts',(47.1805678274021,263.764290563759,31.6200780451729)) ;
#86227=CARTESIAN_POINT('Ctrl Pts',(47.1523648718258,263.589486462611,31.639017761761)) ;
#86228=CARTESIAN_POINT('Ctrl Pts',(47.229577444136,263.131548511894,31.6803418390727)) ;
#86229=CARTESIAN_POINT('Ctrl Pts',(47.6527479151927,262.879524817036,31.6979732378616)) ;
#86230=CARTESIAN_POINT('Ctrl Pts',(47.9007436285402,262.879813170893,31.6979530617955)) ;
#86231=CARTESIAN_POINT('Ctrl Pts',(47.4002579617035,263.764096318685,30.9898141318404)) ;
#86232=CARTESIAN_POINT('Ctrl Pts',(47.387579941251,263.637876445166,31.0375708922236)) ;
#86233=CARTESIAN_POINT('Ctrl Pts',(47.4541847095435,263.32030586019,31.1465778444696)) ;
#86234=CARTESIAN_POINT('Ctrl Pts',(47.7362438590021,263.152506333287,31.1968127976388)) ;
#86235=CARTESIAN_POINT('Ctrl Pts',(47.9004925115266,263.152698325886,31.1967553153352)) ;
#86236=CARTESIAN_POINT('Ctrl Pts',(47.3999996994773,263.764097414176,30.7202074191205)) ;
#86237=CARTESIAN_POINT('Ctrl Pts',(47.3999365884846,263.637590496111,30.7757814206139)) ;
#86238=CARTESIAN_POINT('Ctrl Pts',(47.4915207311276,263.342045075793,30.9056548931698)) ;
#86239=CARTESIAN_POINT('Ctrl Pts',(47.750744453621,263.200584225821,30.9678473764369)) ;
#86240=CARTESIAN_POINT('Ctrl Pts',(47.9004489033514,263.200746091367,30.9677762131617)) ;
#86241=CARTESIAN_POINT('',(47.4,263.763591785235,30.7213203435596)) ;
#86242=CARTESIAN_POINT('Origin',(46.2,263.763591785235,30.7213203435596)) ;
#86243=CARTESIAN_POINT('Origin',(47.9,263.763591785235,30.7213203435596)) ;
#86244=CARTESIAN_POINT('Origin',(46.2,251.191753592594,30.7213203435596)) ;
#86245=CARTESIAN_POINT('',(47.4,251.191753592594,30.7213203435596)) ;
#86246=CARTESIAN_POINT('Origin',(66.4499999999999,263.8,30.7213203435596)) ;
#86247=CARTESIAN_POINT('Origin',(47.9,265.198823964111,23.9039674938989)) ;
#86248=CARTESIAN_POINT('',(47.4,264.5,27.2233813234278)) ;
#86249=CARTESIAN_POINT('Origin',(47.9,264.5,27.2233813234278)) ;
#86250=CARTESIAN_POINT('',(47.4,265.198823964111,23.9039674938989)) ;
#86251=CARTESIAN_POINT('Origin',(54.5,265.241264282414,23.7023759819625)) ;
#86252=CARTESIAN_POINT('',(55.,264.5,27.2233813234279)) ;
#86253=CARTESIAN_POINT('',(55.,265.241264282414,23.7023759819625)) ;
#86254=CARTESIAN_POINT('Origin',(54.5,264.5,27.2233813234279)) ;
#86255=CARTESIAN_POINT('Origin',(55.,265.,19.9213203435596)) ;
#86256=CARTESIAN_POINT('',(55.,264.5,19.9213203435596)) ;
#86257=CARTESIAN_POINT('Origin',(55.5,264.5,19.9213203435596)) ;
#86258=CARTESIAN_POINT('Origin',(55.5,264.5,27.2233813234279)) ;
#86259=CARTESIAN_POINT('Origin',(68.8999999999999,264.5,19.9213203435596)) ;
#86260=CARTESIAN_POINT('',(69.4,264.5,27.2233813234278)) ;
#86261=CARTESIAN_POINT('',(69.4,264.5,19.9213203435596)) ;
#86262=CARTESIAN_POINT('Origin',(68.8999999999999,264.5,27.2233813234279)) ;
#86263=CARTESIAN_POINT('Origin',(69.4,263.,19.9213203435596)) ;
#86264=CARTESIAN_POINT('',(69.4,265.198823964111,23.9039674938989)) ;
#86265=CARTESIAN_POINT('Origin',(69.9,265.198823964111,23.9039674938989)) ;
#86266=CARTESIAN_POINT('Origin',(69.9,264.5,27.2233813234278)) ;
#86267=CARTESIAN_POINT('Origin',(76.5,265.241264282414,23.7023759819625)) ;
#86268=CARTESIAN_POINT('',(77.,264.5,27.2233813234279)) ;
#86269=CARTESIAN_POINT('',(77.,265.241264282414,23.7023759819625)) ;
#86270=CARTESIAN_POINT('Origin',(76.5,264.5,27.2233813234279)) ;
#86271=CARTESIAN_POINT('Origin',(77.,265.,19.9213203435596)) ;
#86272=CARTESIAN_POINT('',(77.,264.5,19.9213203435596)) ;
#86273=CARTESIAN_POINT('Origin',(77.5,264.5,19.9213203435596)) ;
#86274=CARTESIAN_POINT('Origin',(77.5,264.5,27.2233813234279)) ;
#86275=CARTESIAN_POINT('Origin',(57.9573593128808,239.1,25.9213203435596)) ;
#86276=CARTESIAN_POINT('',(57.9573593128808,239.1,25.9213203435596)) ;
#86277=CARTESIAN_POINT('',(57.9573593128808,239.1,25.9213203435596)) ;
#86278=CARTESIAN_POINT('',(58.9573593128808,239.1,25.9213203435596)) ;
#86279=CARTESIAN_POINT('Origin',(57.9573593128808,241.9,25.9213203435596)) ;
#86280=CARTESIAN_POINT('',(57.9573593128808,238.,25.9213203435596)) ;
#86281=CARTESIAN_POINT('Origin',(58.4573593128808,240.5,25.9213203435596)) ;
#86282=CARTESIAN_POINT('Origin',(28.2,259.5,25.9213203435596)) ;
#86283=CARTESIAN_POINT('',(28.2,259.5,22.9213203435596)) ;
#86284=CARTESIAN_POINT('',(28.2,259.5,25.9213203435596)) ;
#86285=CARTESIAN_POINT('Origin',(28.2,262.3,25.9213203435596)) ;
#86286=CARTESIAN_POINT('Origin',(28.2,263.4,19.9213203435596)) ;
#86287=CARTESIAN_POINT('Origin',(80.199999999999,229.4,25.9213203435596)) ;
#86288=CARTESIAN_POINT('',(80.199999999999,229.4,22.9213203435596)) ;
#86289=CARTESIAN_POINT('',(80.199999999999,229.4,25.9213203435596)) ;
#86290=CARTESIAN_POINT('Origin',(80.199999999999,226.6,25.9213203435596)) ;
#86291=CARTESIAN_POINT('Origin',(80.199999999999,225.5,19.9213203435596)) ;
#86292=CARTESIAN_POINT('Origin',(80.1999999999999,252.4,25.9213203435596)) ;
#86293=CARTESIAN_POINT('',(80.1999999999999,252.4,25.9213203435596)) ;
#86294=CARTESIAN_POINT('Origin',(80.1999999999999,249.6,25.9213203435596)) ;
#86295=CARTESIAN_POINT('Origin',(62.3573593128808,236.,19.9213203435596)) ;
#86296=CARTESIAN_POINT('Origin',(59.6573593128808,230.,19.9213203435596)) ;
#86297=CARTESIAN_POINT('Origin',(74.1999999999999,226.,19.9213203435596)) ;
#86298=CARTESIAN_POINT('Origin',(74.1999999999999,232.,19.9213203435596)) ;
#86299=CARTESIAN_POINT('Origin',(46.2,249.,19.9213203435596)) ;
#86300=CARTESIAN_POINT('Origin',(34.2,249.,19.9213203435596)) ;
#86301=CARTESIAN_POINT('Origin',(47.9,265.198823964111,23.9039674938989)) ;
#86302=CARTESIAN_POINT('Ctrl Pts',(47.9,262.836465365523,26.8731635056431)) ;
#86303=CARTESIAN_POINT('Ctrl Pts',(47.5643828957836,262.836465365523,26.8731635056431)) ;
#86304=CARTESIAN_POINT('Ctrl Pts',(46.9213179685814,263.028957632654,26.9136881934604)) ;
#86305=CARTESIAN_POINT('Ctrl Pts',(46.4879676042577,263.526449023177,27.0184232230439)) ;
#86306=CARTESIAN_POINT('Ctrl Pts',(46.3578850044002,263.800011088028,27.0760152366969)) ;
#86307=CARTESIAN_POINT('Origin',(69.9,265.198823964111,23.9039674938989)) ;
#86308=CARTESIAN_POINT('Ctrl Pts',(69.8999999999999,262.836465365523,26.8731635056431)) ;
#86309=CARTESIAN_POINT('Ctrl Pts',(69.5643828957837,262.836465365523,26.8731635056431)) ;
#86310=CARTESIAN_POINT('Ctrl Pts',(68.9213187664228,263.028958787238,26.9136884365308)) ;
#86311=CARTESIAN_POINT('Ctrl Pts',(68.4879676731616,263.526449111869,27.018423241716)) ;
#86312=CARTESIAN_POINT('Ctrl Pts',(68.3578850163,263.800011090529,27.0760152372235)) ;
#86313=CARTESIAN_POINT('',(68.2,265.198823964111,23.9039674938989)) ;
#86314=CARTESIAN_POINT('Origin',(54.5,265.241264282414,23.7023759819625)) ;
#86315=CARTESIAN_POINT('',(56.2,265.241264282414,23.7023759819625)) ;
#86316=CARTESIAN_POINT('Ctrl Pts',(56.0420937198538,263.800015543961,27.0760161747882)) ;
#86317=CARTESIAN_POINT('Ctrl Pts',(55.9130621935296,263.528796310769,27.0189173888531)) ;
#86318=CARTESIAN_POINT('Ctrl Pts',(55.4812583733538,263.030547215847,26.9140228425536)) ;
#86319=CARTESIAN_POINT('Ctrl Pts',(54.8382263221145,262.836465365523,26.8731635056432)) ;
#86320=CARTESIAN_POINT('Ctrl Pts',(54.5,262.836465365523,26.8731635056432)) ;
#86321=CARTESIAN_POINT('Ctrl Pts',(77.5537622727767,263.802136938942,22.4624560909017)) ;
#86322=CARTESIAN_POINT('Ctrl Pts',(77.6160771412392,263.802537425212,22.6256558820165)) ;
#86323=CARTESIAN_POINT('Ctrl Pts',(77.7667803184966,263.803782273667,23.6750632252419)) ;
#86324=CARTESIAN_POINT('Ctrl Pts',(77.9665329974434,263.843280570403,25.8555842488501)) ;
#86325=CARTESIAN_POINT('Ctrl Pts',(78.0877270051615,263.90548764331,27.0982208272828)) ;
#86326=CARTESIAN_POINT('Ctrl Pts',(77.5161760774539,263.799312868747,22.4167726468286)) ;
#86327=CARTESIAN_POINT('Ctrl Pts',(77.5360130337711,263.788191358363,22.5795333003453)) ;
#86328=CARTESIAN_POINT('Ctrl Pts',(77.5967692029986,263.715444795543,23.6261104468405)) ;
#86329=CARTESIAN_POINT('Ctrl Pts',(77.7986137416006,263.605995170056,25.7988034515835)) ;
#86330=CARTESIAN_POINT('Ctrl Pts',(77.9646212448201,263.590301235021,27.0318657939587)) ;
#86331=CARTESIAN_POINT('Ctrl Pts',(77.4409019362984,263.799793835359,22.326574012864)) ;
#86332=CARTESIAN_POINT('Ctrl Pts',(77.3748831483453,263.771443558149,22.4887490503241)) ;
#86333=CARTESIAN_POINT('Ctrl Pts',(77.2452754678601,263.588475046809,23.5314907130649)) ;
#86334=CARTESIAN_POINT('Ctrl Pts',(77.3522662402912,263.226007627549,25.6938646863724)) ;
#86335=CARTESIAN_POINT('Ctrl Pts',(77.5202253706355,263.042309806729,26.9164991774763)) ;
#86336=CARTESIAN_POINT('Ctrl Pts',(77.3648210667925,263.812301985206,22.2379396633952)) ;
#86337=CARTESIAN_POINT('Ctrl Pts',(77.2112621247156,263.777968352196,22.4010107034791)) ;
#86338=CARTESIAN_POINT('Ctrl Pts',(76.8778016563596,263.557546258392,23.4497540555238)) ;
#86339=CARTESIAN_POINT('Ctrl Pts',(76.7820603106784,263.099191795812,25.6290359143092)) ;
#86340=CARTESIAN_POINT('Ctrl Pts',(76.8382263221145,262.836465365523,26.8731635056432)) ;
#86341=CARTESIAN_POINT('Ctrl Pts',(77.3271465306621,263.821412870453,22.1946628572268)) ;
#86342=CARTESIAN_POINT('Ctrl Pts',(77.1302379764753,263.786866856953,22.3587564213473)) ;
#86343=CARTESIAN_POINT('Ctrl Pts',(76.6959586099435,263.564706082808,23.4140200985382)) ;
#86344=CARTESIAN_POINT('Ctrl Pts',(76.4999999999999,263.102238319793,25.6107419728579)) ;
#86345=CARTESIAN_POINT('Ctrl Pts',(76.5,262.836465365523,26.8731635056432)) ;
#86346=CARTESIAN_POINT('Ctrl Pts',(46.3089246998894,263.914167397861,27.1000481440303)) ;
#86347=CARTESIAN_POINT('Ctrl Pts',(46.398964552187,263.865836783231,26.1667163497985)) ;
#86348=CARTESIAN_POINT('Ctrl Pts',(46.6032252577224,263.805761093415,23.9724961226782)) ;
#86349=CARTESIAN_POINT('Ctrl Pts',(46.7606927309181,263.803165448826,22.6811011432147)) ;
#86350=CARTESIAN_POINT('Ctrl Pts',(46.8451922840736,263.802215511675,22.4637434724043)) ;
#86351=CARTESIAN_POINT('Ctrl Pts',(46.4320964795723,263.592931328567,27.0324194978629)) ;
#86352=CARTESIAN_POINT('Ctrl Pts',(46.5570399219172,263.604010070467,26.1064695432228)) ;
#86353=CARTESIAN_POINT('Ctrl Pts',(46.7855269650946,263.693914392471,23.922291785831)) ;
#86354=CARTESIAN_POINT('Ctrl Pts',(46.8563738086724,263.784563059776,22.6340524722874)) ;
#86355=CARTESIAN_POINT('Ctrl Pts',(46.8834079801304,263.7992846537,22.417292856026)) ;
#86356=CARTESIAN_POINT('Ctrl Pts',(46.8791957179207,263.041566324535,26.9163426549089)) ;
#86357=CARTESIAN_POINT('Ctrl Pts',(47.005410100848,263.179715009613,25.9983019039964)) ;
#86358=CARTESIAN_POINT('Ctrl Pts',(47.1632040825922,263.535554931216,23.8263510090413)) ;
#86359=CARTESIAN_POINT('Ctrl Pts',(47.0468280440546,263.761973579305,22.5426416146634)) ;
#86360=CARTESIAN_POINT('Ctrl Pts',(46.9590496239828,263.799755056779,22.3266718772418)) ;
#86361=CARTESIAN_POINT('Ctrl Pts',(47.5643828957836,262.836465365523,26.8731635056431)) ;
#86362=CARTESIAN_POINT('Ctrl Pts',(47.60623000954,263.033757813591,25.9388062619286)) ;
#86363=CARTESIAN_POINT('Ctrl Pts',(47.5618573951966,263.495689639793,23.7452082892501)) ;
#86364=CARTESIAN_POINT('Ctrl Pts',(47.2403381174637,263.766640803451,22.4548184438463)) ;
#86365=CARTESIAN_POINT('Ctrl Pts',(47.035499525566,263.812365610051,22.2376373441309)) ;
#86366=CARTESIAN_POINT('Ctrl Pts',(47.9,262.836465365523,26.8731635056431)) ;
#86367=CARTESIAN_POINT('Ctrl Pts',(47.9,263.036041279363,25.925177914903)) ;
#86368=CARTESIAN_POINT('Ctrl Pts',(47.7565399119583,263.502185788995,23.7109914941486)) ;
#86369=CARTESIAN_POINT('Ctrl Pts',(47.3349857520721,263.775399470748,22.4132265058195)) ;
#86370=CARTESIAN_POINT('Ctrl Pts',(47.0728917988203,263.821406189075,22.1946945937677)) ;
#86371=CARTESIAN_POINT('Ctrl Pts',(68.3089238972751,263.914169501419,27.1000485868847)) ;
#86372=CARTESIAN_POINT('Ctrl Pts',(68.3989635214134,263.86583849844,26.1667167443968)) ;
#86373=CARTESIAN_POINT('Ctrl Pts',(68.6032220468531,263.805761123684,23.9725059876743)) ;
#86374=CARTESIAN_POINT('Ctrl Pts',(68.7606921054679,263.803165570431,22.6811014507584)) ;
#86375=CARTESIAN_POINT('Ctrl Pts',(68.8451920342653,263.802215530838,22.4637437760421)) ;
#86376=CARTESIAN_POINT('Ctrl Pts',(68.4320954464358,263.59293250129,27.0324197447521)) ;
#86377=CARTESIAN_POINT('Ctrl Pts',(68.5570388859512,263.60401096028,26.1064697725006)) ;
#86378=CARTESIAN_POINT('Ctrl Pts',(68.7855276207896,263.693915243154,23.9223023915977)) ;
#86379=CARTESIAN_POINT('Ctrl Pts',(68.856373384639,263.784563110008,22.6340526757915)) ;
#86380=CARTESIAN_POINT('Ctrl Pts',(68.8834078117171,263.799284652591,22.4172930577749)) ;
#86381=CARTESIAN_POINT('Ctrl Pts',(68.8791958017697,263.041567784116,26.9163429621891)) ;
#86382=CARTESIAN_POINT('Ctrl Pts',(69.0054102786155,263.179716403355,25.998302229438)) ;
#86383=CARTESIAN_POINT('Ctrl Pts',(69.1631998752088,263.535551916632,23.8263609376104)) ;
#86384=CARTESIAN_POINT('Ctrl Pts',(69.0468278287294,263.761973575494,22.5426417126032)) ;
#86385=CARTESIAN_POINT('Ctrl Pts',(68.9590495389693,263.799755044124,22.3266719765335)) ;
#86386=CARTESIAN_POINT('Ctrl Pts',(69.5643828957837,262.836465365523,26.8731635056431)) ;
#86387=CARTESIAN_POINT('Ctrl Pts',(69.6062300095402,263.033757813591,25.9388062619264)) ;
#86388=CARTESIAN_POINT('Ctrl Pts',(69.5618553916678,263.495691690019,23.7452185551853)) ;
#86389=CARTESIAN_POINT('Ctrl Pts',(69.2403381174618,263.766640803452,22.4548184438401)) ;
#86390=CARTESIAN_POINT('Ctrl Pts',(69.0354995255635,263.812365610052,22.2376373441282)) ;
#86391=CARTESIAN_POINT('Ctrl Pts',(69.8999999999999,262.836465365523,26.8731635056431)) ;
#86392=CARTESIAN_POINT('Ctrl Pts',(69.9,263.036041279363,25.9251779149008)) ;
#86393=CARTESIAN_POINT('Ctrl Pts',(69.7565372356489,263.502183882598,23.7110005495361)) ;
#86394=CARTESIAN_POINT('Ctrl Pts',(69.3349857520697,263.77539947075,22.4132265058132)) ;
#86395=CARTESIAN_POINT('Ctrl Pts',(69.0728917988171,263.821406189076,22.194694593765)) ;
#86396=CARTESIAN_POINT('Origin',(68.2,263.,19.9213203435596)) ;
#86397=CARTESIAN_POINT('Ctrl Pts',(55.5537620469059,263.802136922676,22.4624558020398)) ;
#86398=CARTESIAN_POINT('Ctrl Pts',(55.6160766782539,263.80253734094,22.6256555955562)) ;
#86399=CARTESIAN_POINT('Ctrl Pts',(55.7667779370375,263.803782509322,23.6750521597127)) ;
#86400=CARTESIAN_POINT('Ctrl Pts',(55.9665320341884,263.843279207882,25.8555839228286)) ;
#86401=CARTESIAN_POINT('Ctrl Pts',(56.0877262991014,263.905485833697,27.0982204463116)) ;
#86402=CARTESIAN_POINT('Ctrl Pts',(55.5161759288423,263.799312871516,22.4167724460066)) ;
#86403=CARTESIAN_POINT('Ctrl Pts',(55.5360127177972,263.788191328469,22.5795331048077)) ;
#86404=CARTESIAN_POINT('Ctrl Pts',(55.5967692807576,263.715444932713,23.6260989147318)) ;
#86405=CARTESIAN_POINT('Ctrl Pts',(55.7986128632549,263.605994459492,25.798803253818)) ;
#86406=CARTESIAN_POINT('Ctrl Pts',(55.9646203702438,263.59030019996,27.0318655760511)) ;
#86407=CARTESIAN_POINT('Ctrl Pts',(55.4409018736246,263.799793850706,22.326573900578)) ;
#86408=CARTESIAN_POINT('Ctrl Pts',(55.3748830042504,263.771443563708,22.4887489443983)) ;
#86409=CARTESIAN_POINT('Ctrl Pts',(55.2452720253742,263.588478145295,23.5314796807535)) ;
#86410=CARTESIAN_POINT('Ctrl Pts',(55.3522665253084,263.226006301692,25.693864370421)) ;
#86411=CARTESIAN_POINT('Ctrl Pts',(55.5202255476893,263.042308404551,26.9164988822807)) ;
#86412=CARTESIAN_POINT('Ctrl Pts',(55.3648210917583,263.812301990784,22.2379396367372)) ;
#86413=CARTESIAN_POINT('Ctrl Pts',(55.2112621445889,263.777968364114,22.4010106829945)) ;
#86414=CARTESIAN_POINT('Ctrl Pts',(54.8777999382771,263.557545614509,23.449742781627)) ;
#86415=CARTESIAN_POINT('Ctrl Pts',(54.7820603106785,263.099191795812,25.6290359143101)) ;
#86416=CARTESIAN_POINT('Ctrl Pts',(54.8382263221145,262.836465365523,26.8731635056432)) ;
#86417=CARTESIAN_POINT('Ctrl Pts',(55.3271465626755,263.821412876097,22.1946628304122)) ;
#86418=CARTESIAN_POINT('Ctrl Pts',(55.1302380022922,263.786866861796,22.3587563983465)) ;
#86419=CARTESIAN_POINT('Ctrl Pts',(54.6959563997398,263.564708271942,23.4140097001504)) ;
#86420=CARTESIAN_POINT('Ctrl Pts',(54.4999999999999,263.102238319793,25.6107419728589)) ;
#86421=CARTESIAN_POINT('Ctrl Pts',(54.5,262.836465365523,26.8731635056432)) ;
#86422=CARTESIAN_POINT('Origin',(56.2,265.,19.9213203435596)) ;
#86423=CARTESIAN_POINT('Ctrl Pts',(47.4008246626337,264.507291217703,27.3512671439807)) ;
#86424=CARTESIAN_POINT('Ctrl Pts',(47.3989076166213,264.621171941884,26.2435524495949)) ;
#86425=CARTESIAN_POINT('Ctrl Pts',(47.3293899330196,264.805875369694,24.4171429924089)) ;
#86426=CARTESIAN_POINT('Ctrl Pts',(47.1149669351868,264.970247820277,22.7745888050877)) ;
#86427=CARTESIAN_POINT('Ctrl Pts',(46.9644226373298,265.001836362709,22.4577371313621)) ;
#86428=CARTESIAN_POINT('Ctrl Pts',(46.8873229985597,264.999843640625,22.477722172732)) ;
#86429=CARTESIAN_POINT('Ctrl Pts',(47.3909631887125,264.370604282734,27.3224308638185)) ;
#86430=CARTESIAN_POINT('Ctrl Pts',(47.4243488309635,264.501610595782,26.2190423498724)) ;
#86431=CARTESIAN_POINT('Ctrl Pts',(47.385851610773,264.73667771661,24.3962605702668)) ;
#86432=CARTESIAN_POINT('Ctrl Pts',(47.1535711617938,264.958837275192,22.7560844475633)) ;
#86433=CARTESIAN_POINT('Ctrl Pts',(46.9758145805122,265.0024310584,22.4395657325186)) ;
#86434=CARTESIAN_POINT('Ctrl Pts',(46.8850787413281,264.999683369079,22.4595294432364)) ;
#86435=CARTESIAN_POINT('Ctrl Pts',(47.4952139876938,264.097493346775,27.2655157277541)) ;
#86436=CARTESIAN_POINT('Ctrl Pts',(47.5582348223583,264.292430830159,26.170510089975)) ;
#86437=CARTESIAN_POINT('Ctrl Pts',(47.5249447211539,264.631611270102,24.3552106906146)) ;
#86438=CARTESIAN_POINT('Ctrl Pts',(47.228614625003,264.944153638504,22.7198228985961)) ;
#86439=CARTESIAN_POINT('Ctrl Pts',(46.9983903760502,265.005190448574,22.4040660373099)) ;
#86440=CARTESIAN_POINT('Ctrl Pts',(46.8806381671158,265.00134258216,22.4239812708368)) ;
#86441=CARTESIAN_POINT('Ctrl Pts',(47.7673957205814,263.984449147131,27.2432031080418)) ;
#86442=CARTESIAN_POINT('Ctrl Pts',(47.7928204242151,264.216965605649,26.1426034533423)) ;
#86443=CARTESIAN_POINT('Ctrl Pts',(47.6940585839927,264.599716436459,24.3229037323166)) ;
#86444=CARTESIAN_POINT('Ctrl Pts',(47.3047276552285,264.944752851235,22.6850560291216)) ;
#86445=CARTESIAN_POINT('Ctrl Pts',(47.0211912224739,265.011015887813,22.3688906832847)) ;
#86446=CARTESIAN_POINT('Ctrl Pts',(46.8761507816279,265.006835652272,22.3888318545834)) ;
#86447=CARTESIAN_POINT('Ctrl Pts',(47.900839428631,263.984703728653,27.2439881395081)) ;
#86448=CARTESIAN_POINT('Ctrl Pts',(47.9070163405631,264.21777726175,26.1368564584777)) ;
#86449=CARTESIAN_POINT('Ctrl Pts',(47.7764900567607,264.602186299455,24.3109308810781)) ;
#86450=CARTESIAN_POINT('Ctrl Pts',(47.3417200484268,264.947919455522,22.6686907100956)) ;
#86451=CARTESIAN_POINT('Ctrl Pts',(47.0323284790502,265.014618545435,22.3518830915824)) ;
#86452=CARTESIAN_POINT('Ctrl Pts',(46.873959871809,265.010411597039,22.3718653109223)) ;
#86453=CARTESIAN_POINT('Origin',(46.9,264.5,27.2233813234279)) ;
#86454=CARTESIAN_POINT('Ctrl Pts',(55.5255673610189,264.999356809564,22.4862307209618)) ;
#86455=CARTESIAN_POINT('Ctrl Pts',(55.4109671059889,265.005425204665,22.4210492449598)) ;
#86456=CARTESIAN_POINT('Ctrl Pts',(55.1416818286438,264.924461110078,23.2918898343867)) ;
#86457=CARTESIAN_POINT('Ctrl Pts',(55.0024976411188,264.667616273681,25.9804497446043)) ;
#86458=CARTESIAN_POINT('Ctrl Pts',(54.9963300104537,264.515694422742,27.4891456859497)) ;
#86459=CARTESIAN_POINT('Ctrl Pts',(55.5304587903673,264.998833446453,22.4670625659595)) ;
#86460=CARTESIAN_POINT('Ctrl Pts',(55.3940129026723,265.007685061672,22.4019652735408)) ;
#86461=CARTESIAN_POINT('Ctrl Pts',(55.0701232396585,264.889109282959,23.2716945070135)) ;
#86462=CARTESIAN_POINT('Ctrl Pts',(54.9691052398483,264.542596400602,25.9559962065829)) ;
#86463=CARTESIAN_POINT('Ctrl Pts',(55.01870636833,264.370339661709,27.4582800755484)) ;
#86464=CARTESIAN_POINT('Ctrl Pts',(55.5399297326649,265.000117029878,22.4304757432437)) ;
#86465=CARTESIAN_POINT('Ctrl Pts',(55.3610526986339,265.012656016268,22.3655583950824)) ;
#86466=CARTESIAN_POINT('Ctrl Pts',(54.9363638397547,264.844925871569,23.2329126197646)) ;
#86467=CARTESIAN_POINT('Ctrl Pts',(54.823337890213,264.339857688415,25.9080805918787)) ;
#86468=CARTESIAN_POINT('Ctrl Pts',(54.9202367438694,264.076965070082,27.3976744897227)) ;
#86469=CARTESIAN_POINT('Ctrl Pts',(55.5495146369683,265.005673339809,22.3943346542401)) ;
#86470=CARTESIAN_POINT('Ctrl Pts',(55.3276395741456,265.019340477166,22.3293242824278)) ;
#86471=CARTESIAN_POINT('Ctrl Pts',(54.8035926044541,264.836747727878,23.1979076932162)) ;
#86472=CARTESIAN_POINT('Ctrl Pts',(54.5910965086588,264.272804860473,25.8777147035963)) ;
#86473=CARTESIAN_POINT('Ctrl Pts',(54.6354515551578,263.956212815122,27.3754759866893)) ;
#86474=CARTESIAN_POINT('Ctrl Pts',(55.5540753127105,265.009258937202,22.3773405899133)) ;
#86475=CARTESIAN_POINT('Ctrl Pts',(55.3117363898015,265.022976994424,22.3121815465214)) ;
#86476=CARTESIAN_POINT('Ctrl Pts',(54.7405444818452,264.839699472842,23.1827259708804)) ;
#86477=CARTESIAN_POINT('Ctrl Pts',(54.4812488421695,264.273919304648,25.8701523185663)) ;
#86478=CARTESIAN_POINT('Ctrl Pts',(54.4993596409889,263.956681652816,27.3771201355784)) ;
#86479=CARTESIAN_POINT('Ctrl Pts',(77.5126870873055,264.999843389651,22.4777270870555)) ;
#86480=CARTESIAN_POINT('Ctrl Pts',(77.4355856076841,265.001837775216,22.4577244733426)) ;
#86481=CARTESIAN_POINT('Ctrl Pts',(77.2850416233415,264.970250830608,22.774574270844)) ;
#86482=CARTESIAN_POINT('Ctrl Pts',(77.070616045939,264.805880890583,24.4171737852644)) ;
#86483=CARTESIAN_POINT('Ctrl Pts',(77.0010927930105,264.621179637214,26.2436227267522)) ;
#86484=CARTESIAN_POINT('Ctrl Pts',(76.9991739635825,264.507297407404,27.3513716626615)) ;
#86485=CARTESIAN_POINT('Ctrl Pts',(77.5149332535848,264.999682929536,22.4595336213756)) ;
#86486=CARTESIAN_POINT('Ctrl Pts',(77.4241945868893,265.002432970266,22.4395523417571)) ;
#86487=CARTESIAN_POINT('Ctrl Pts',(77.2464340770455,264.958840455122,22.7560694393853)) ;
#86488=CARTESIAN_POINT('Ctrl Pts',(77.014150140122,264.736678453386,24.3962909120826)) ;
#86489=CARTESIAN_POINT('Ctrl Pts',(76.9756554398609,264.5016104682,26.2191114851833)) ;
#86490=CARTESIAN_POINT('Ctrl Pts',(77.0090442725839,264.370603528154,27.3225338245482)) ;
#86491=CARTESIAN_POINT('Ctrl Pts',(77.5193774902576,265.001341919645,22.4239852672336)) ;
#86492=CARTESIAN_POINT('Ctrl Pts',(77.4016209356984,265.005193167249,22.4040525055347)) ;
#86493=CARTESIAN_POINT('Ctrl Pts',(77.1713939672703,264.944156713126,22.7198077925902)) ;
#86494=CARTESIAN_POINT('Ctrl Pts',(76.8750612211273,264.631607422865,24.3552406151253)) ;
#86495=CARTESIAN_POINT('Ctrl Pts',(76.8417685764965,264.292425394558,26.1705787621317)) ;
#86496=CARTESIAN_POINT('Ctrl Pts',(76.904797000281,264.097484288593,27.2656173880932)) ;
#86497=CARTESIAN_POINT('Ctrl Pts',(77.523868555885,265.006834920525,22.3888356841188)) ;
#86498=CARTESIAN_POINT('Ctrl Pts',(77.3788224880676,265.011018690996,22.3688769443209)) ;
#86499=CARTESIAN_POINT('Ctrl Pts',(77.0952809873972,264.944758364116,22.6850409999854)) ;
#86500=CARTESIAN_POINT('Ctrl Pts',(76.7059440140755,264.599714552233,24.3229338911505)) ;
#86501=CARTESIAN_POINT('Ctrl Pts',(76.6071833141231,264.216953764414,26.1426713565531)) ;
#86502=CARTESIAN_POINT('Ctrl Pts',(76.6326153072635,263.984431556749,27.2433041953422)) ;
#86503=CARTESIAN_POINT('Ctrl Pts',(77.5260611861056,265.010410675423,22.3718696861525)) ;
#86504=CARTESIAN_POINT('Ctrl Pts',(77.3676867570225,265.014621321342,22.3518699016325)) ;
#86505=CARTESIAN_POINT('Ctrl Pts',(77.0582908870455,264.947922650659,22.6686755732325)) ;
#86506=CARTESIAN_POINT('Ctrl Pts',(76.623515455463,264.602180068614,24.3109603652938)) ;
#86507=CARTESIAN_POINT('Ctrl Pts',(76.4929898959272,264.217763018292,26.1369243071539)) ;
#86508=CARTESIAN_POINT('Ctrl Pts',(76.4991742481055,263.984682447818,27.2440890311872)) ;
#86509=CARTESIAN_POINT('Ctrl Pts',(69.4008257028231,264.507295904801,27.3513462902868)) ;
#86510=CARTESIAN_POINT('Ctrl Pts',(69.3989073063844,264.621177769096,26.2436056666157)) ;
#86511=CARTESIAN_POINT('Ctrl Pts',(69.3293854049881,264.805879550229,24.4171663113135)) ;
#86512=CARTESIAN_POINT('Ctrl Pts',(69.1149604545227,264.970250099837,22.7745777990922)) ;
#86513=CARTESIAN_POINT('Ctrl Pts',(68.9644163937797,265.001837432337,22.4577275461148)) ;
#86514=CARTESIAN_POINT('Ctrl Pts',(68.8873153610441,264.999843450594,22.4777258938723)) ;
#86515=CARTESIAN_POINT('Ctrl Pts',(69.3909575385873,264.370603711185,27.3225088303552)) ;
#86516=CARTESIAN_POINT('Ctrl Pts',(69.4243455968175,264.501610499055,26.2190947022126)) ;
#86517=CARTESIAN_POINT('Ctrl Pts',(69.3858502849074,264.736678274293,24.3962835477298)) ;
#86518=CARTESIAN_POINT('Ctrl Pts',(69.1535671948623,264.958839683308,22.7560730826454)) ;
#86519=CARTESIAN_POINT('Ctrl Pts',(68.9758076385222,265.002432506156,22.4395555924098)) ;
#86520=CARTESIAN_POINT('Ctrl Pts',(68.8850696582037,264.999683036264,22.4595326069041)) ;
#86521=CARTESIAN_POINT('Ctrl Pts',(69.4952056691767,264.097486489153,27.2655927099579)) ;
#86522=CARTESIAN_POINT('Ctrl Pts',(69.5582322508228,264.292426715909,26.1705620920024)) ;
#86523=CARTESIAN_POINT('Ctrl Pts',(69.5249402193863,264.63160835578,24.3552333518857)) ;
#86524=CARTESIAN_POINT('Ctrl Pts',(69.2286081188304,264.944155966591,22.7198114595033)) ;
#86525=CARTESIAN_POINT('Ctrl Pts',(68.9983818102557,265.005192507295,22.4040557903944)) ;
#86526=CARTESIAN_POINT('Ctrl Pts',(68.8806263106136,265.001342080515,22.4239842968519)) ;
#86527=CARTESIAN_POINT('Ctrl Pts',(69.7673873702777,263.98443582666,27.24327965592)) ;
#86528=CARTESIAN_POINT('Ctrl Pts',(69.7928175937792,264.21695663877,26.1426548726517)) ;
#86529=CARTESIAN_POINT('Ctrl Pts',(69.6940566161564,264.599715009964,24.3229265712649)) ;
#86530=CARTESIAN_POINT('Ctrl Pts',(69.3047211111121,264.944757025772,22.6850446482569)) ;
#86531=CARTESIAN_POINT('Ctrl Pts',(69.0211808402246,265.011018010547,22.3688802794475)) ;
#86532=CARTESIAN_POINT('Ctrl Pts',(68.8761361383546,265.006835098209,22.3888347542145)) ;
#86533=CARTESIAN_POINT('Ctrl Pts',(69.9008290727288,263.984687613801,27.2440645392984)) ;
#86534=CARTESIAN_POINT('Ctrl Pts',(69.9070116186382,264.217766475947,26.1369078365147)) ;
#86535=CARTESIAN_POINT('Ctrl Pts',(69.7764858821136,264.602181580875,24.3109532089491)) ;
#86536=CARTESIAN_POINT('Ctrl Pts',(69.3417117681599,264.947921875006,22.6686792476652)) ;
#86537=CARTESIAN_POINT('Ctrl Pts',(69.0323169416041,265.014620647502,22.3518731034479)) ;
#86538=CARTESIAN_POINT('Ctrl Pts',(68.8739439257557,265.01041089921,22.3718686237511)) ;
#86539=CARTESIAN_POINT('Origin',(46.9,264.5,19.9213203435596)) ;
#86540=CARTESIAN_POINT('',(47.4,264.5,19.9213203435596)) ;
#86541=CARTESIAN_POINT('Origin',(47.4,263.,19.9213203435596)) ;
#117128=UNCERTAINTY_MEASURE_WITH_UNIT(LENGTH_MEASURE(0.01),#117171,
'DISTANCE_ACCURACY_VALUE',
'Maximum model space distance between geometric entities at asserted c
onnectivities') ;
#117147=UNCERTAINTY_MEASURE_WITH_UNIT(LENGTH_MEASURE(0.01),#117171,
'DISTANCE_ACCURACY_VALUE',
'Maximum model space distance between geometric entities at asserted c
onnectivities') ;
#117151=(
GEOMETRIC_REPRESENTATION_CONTEXT(3)
GLOBAL_UNCERTAINTY_ASSIGNED_CONTEXT((#117128))
GLOBAL_UNIT_ASSIGNED_CONTEXT((#117171,#117173,#117174))
REPRESENTATION_CONTEXT('','3D')
) ;
#117170=(
GEOMETRIC_REPRESENTATION_CONTEXT(3)
GLOBAL_UNCERTAINTY_ASSIGNED_CONTEXT((#117147))
GLOBAL_UNIT_ASSIGNED_CONTEXT((#117171,#117173,#117174))
REPRESENTATION_CONTEXT('','3D')
) ;
#117171=(
LENGTH_UNIT()
NAMED_UNIT(*)
SI_UNIT(.MILLI.,.METRE.)
) ;
#117173=(
NAMED_UNIT(*)
PLANE_ANGLE_UNIT()
SI_UNIT($,.RADIAN.)
) ;
#117174=(
NAMED_UNIT(*)
SI_UNIT($,.STERADIAN.)
SOLID_ANGLE_UNIT()
) ;
#117178=SHAPE_DEFINITION_REPRESENTATION(#117200,#117243) ;
#117200=PRODUCT_DEFINITION_SHAPE('',$,#117266) ;
#117243=SHAPE_REPRESENTATION('',(#50164),#117151) ;
#117262=PRODUCT_DEFINITION_CONTEXT('part definition',#117330,'design') ;
#117266=PRODUCT_DEFINITION('Base_Plate','Base_Plate',#117288,#117262) ;
#117288=PRODUCT_DEFINITION_FORMATION('',$,#117335) ;
#117330=APPLICATION_CONTEXT(
'Core Data for Automotive Mechanical Design Process') ;
#117331=PRODUCT_CONTEXT('part definition',#117330,'mechanical') ;
#117335=PRODUCT('Base_Plate','Base_Plate',$,(#117331)) ;
#117355=PRESENTATION_STYLE_ASSIGNMENT((#117357)) ;
#117357=SURFACE_STYLE_USAGE(.BOTH.,#117359) ;
#117359=SURFACE_SIDE_STYLE('',(#117361)) ;
#117361=SURFACE_STYLE_FILL_AREA(#117363) ;
#117363=FILL_AREA_STYLE('Opaque(160,160,160)',(#117365)) ;
#117365=FILL_AREA_STYLE_COLOUR('Opaque(160,160,160)',#117367) ;
#117367=COLOUR_RGB('Opaque(160,160,160)', 0.09019608, 0.27058824, 0.51372549) ;
ENDSEC;
END-ISO-10303-21;
